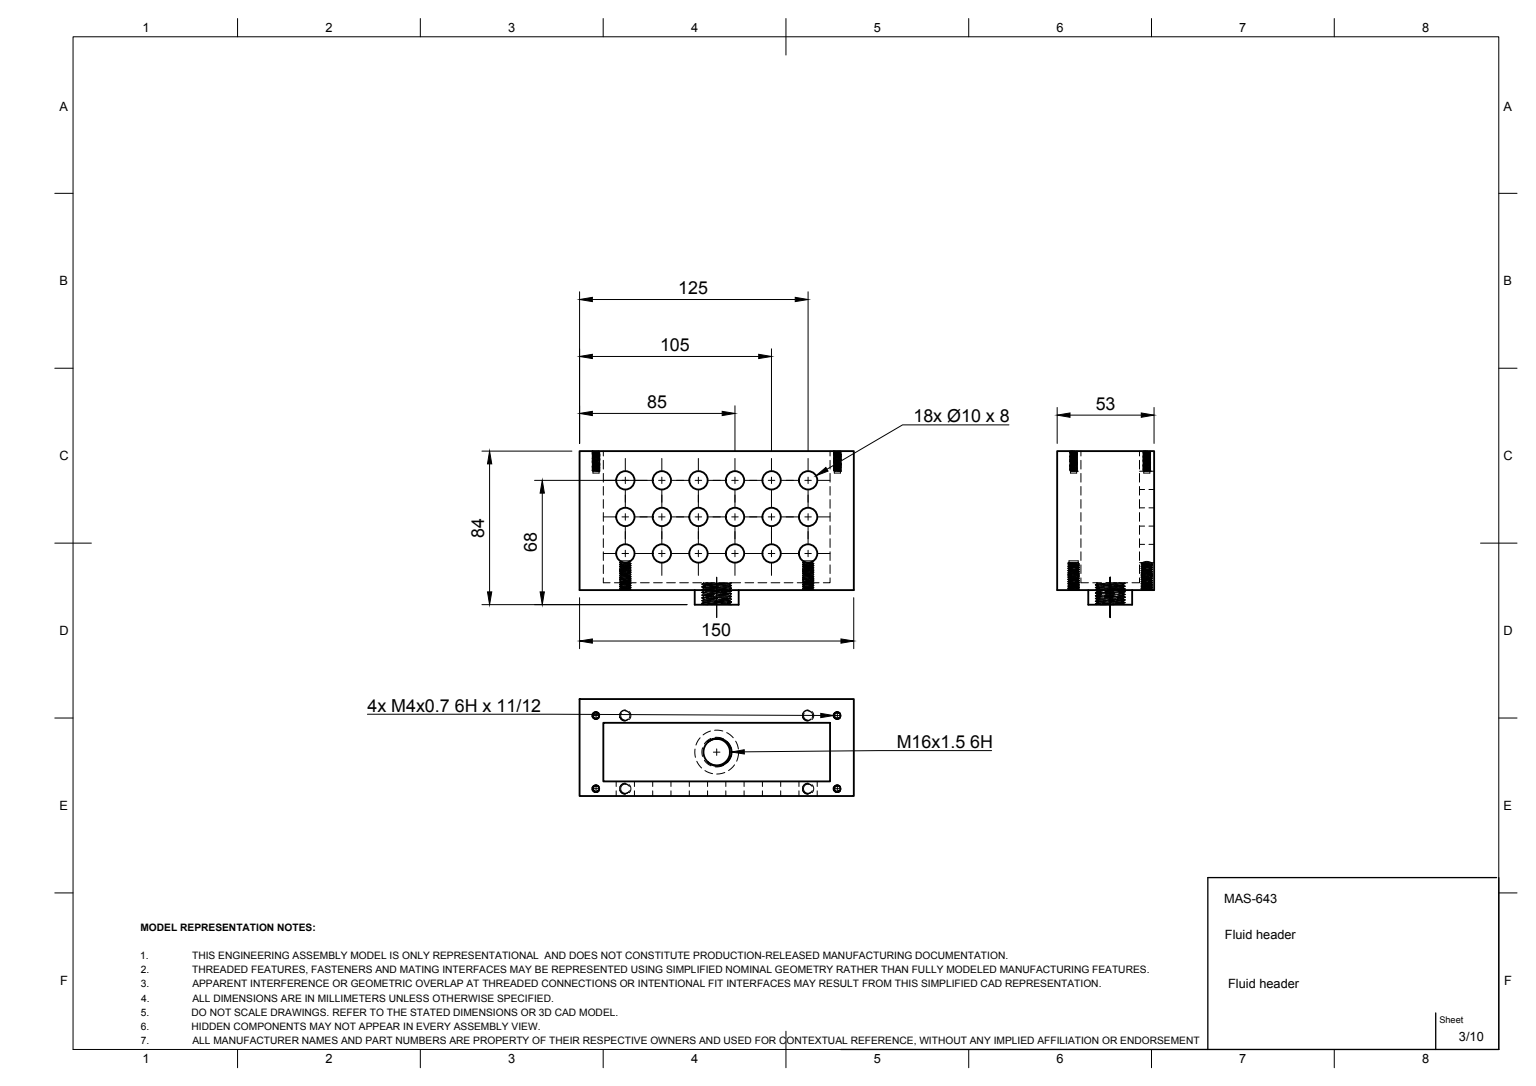
ISO-10303-21;
HEADER;
/* Generated by software containing ST-Developer
 * from STEP Tools, Inc. (www.steptools.com) 
 */

FILE_DESCRIPTION(
/* description */ ('Independent eighteen-tube parallel-flow evaporator geometry. Repeated
 machined headers and gasketed service covers, eighteen copper tubes, 
twenty-nine punched fins, threaded hose connections and bolted mountin
g feet. Native editable features and instanced parts. Braze details, w
orking fluid, pressure and thermal ratings require engineering selecti
on.'),
/* implementation_level */ '2;1');

FILE_NAME(
/* name */ 'Fluid header.step',
/* time_stamp */ '2026-11-08T20:53:59-08:00',
/* author */ (''),
/* organization */ (''),
/* preprocessor_version */ 'ST-DEVELOPER v20.2',
/* originating_system */ 'Autodesk Translation Framework v15.17.0.0',
/* authorisation */ '');

FILE_SCHEMA (('AUTOMOTIVE_DESIGN { 1 0 10303 214 3 1 1 }'));
ENDSEC;

DATA;
#10=MECHANICAL_DESIGN_GEOMETRIC_PRESENTATION_REPRESENTATION('',(#333),#42620);
#313=SHAPE_REPRESENTATION_RELATIONSHIP('SRR','None',#42723,#323);
#323=ADVANCED_BREP_SHAPE_REPRESENTATION('',(#343),#42610);
#333=STYLED_ITEM('',(#42782),#343);
#343=MANIFOLD_SOLID_BREP('Body1',#10383);
#353=FACE_BOUND('',#1411,.T.);
#354=FACE_BOUND('',#1415,.T.);
#355=FACE_BOUND('',#1416,.T.);
#356=FACE_BOUND('',#1417,.T.);
#357=FACE_BOUND('',#1418,.T.);
#358=FACE_BOUND('',#1419,.T.);
#359=FACE_BOUND('',#1492,.T.);
#360=FACE_BOUND('',#1493,.T.);
#361=FACE_BOUND('',#1494,.T.);
#362=FACE_BOUND('',#1495,.T.);
#363=FACE_BOUND('',#1496,.T.);
#364=FACE_BOUND('',#1497,.T.);
#365=FACE_BOUND('',#1498,.T.);
#366=FACE_BOUND('',#1499,.T.);
#367=FACE_BOUND('',#1500,.T.);
#368=FACE_BOUND('',#1501,.T.);
#369=FACE_BOUND('',#1502,.T.);
#370=FACE_BOUND('',#1503,.T.);
#371=FACE_BOUND('',#1504,.T.);
#372=FACE_BOUND('',#1505,.T.);
#373=FACE_BOUND('',#1506,.T.);
#374=FACE_BOUND('',#1507,.T.);
#375=FACE_BOUND('',#1508,.T.);
#376=FACE_BOUND('',#1509,.T.);
#377=FACE_BOUND('',#1513,.T.);
#378=FACE_BOUND('',#1516,.T.);
#379=FACE_BOUND('',#1517,.T.);
#380=FACE_BOUND('',#1518,.T.);
#381=FACE_BOUND('',#1519,.T.);
#382=FACE_BOUND('',#1520,.T.);
#383=FACE_BOUND('',#1521,.T.);
#384=FACE_BOUND('',#1522,.T.);
#385=FACE_BOUND('',#1523,.T.);
#386=FACE_BOUND('',#1524,.T.);
#387=FACE_BOUND('',#1525,.T.);
#388=FACE_BOUND('',#1526,.T.);
#389=FACE_BOUND('',#1527,.T.);
#390=FACE_BOUND('',#1528,.T.);
#391=FACE_BOUND('',#1529,.T.);
#392=FACE_BOUND('',#1530,.T.);
#393=FACE_BOUND('',#1531,.T.);
#394=FACE_BOUND('',#1532,.T.);
#395=FACE_BOUND('',#1533,.T.);
#396=FACE_BOUND('',#1537,.T.);
#397=FACE_BOUND('',#1538,.T.);
#398=FACE_BOUND('',#1539,.T.);
#399=FACE_BOUND('',#1540,.T.);
#400=FACE_BOUND('',#1541,.T.);
#487=PLANE('',#10813);
#488=PLANE('',#10818);
#489=PLANE('',#10819);
#490=PLANE('',#10822);
#491=PLANE('',#10825);
#492=PLANE('',#10826);
#493=PLANE('',#10828);
#494=PLANE('',#10831);
#495=PLANE('',#10832);
#496=PLANE('',#10834);
#497=PLANE('',#10838);
#498=PLANE('',#10839);
#499=PLANE('',#10841);
#500=PLANE('',#10844);
#501=PLANE('',#10847);
#502=PLANE('',#10850);
#503=PLANE('',#10853);
#504=PLANE('',#10854);
#505=PLANE('',#10855);
#506=PLANE('',#10856);
#507=PLANE('',#10911);
#508=PLANE('',#10912);
#509=PLANE('',#10913);
#510=PLANE('',#10914);
#511=PLANE('',#10915);
#512=PLANE('',#10916);
#513=PLANE('',#10917);
#514=PLANE('',#10918);
#515=PLANE('',#10919);
#516=PLANE('',#10920);
#579=B_SPLINE_SURFACE_WITH_KNOTS('',3,3,((#23222,#23223,#23224,#23225,#23226,
#23227,#23228,#23229,#23230,#23231,#23232,#23233,#23234,#23235,#23236,#23237,
#23238,#23239,#23240,#23241,#23242,#23243,#23244,#23245,#23246,#23247,#23248,
#23249,#23250,#23251,#23252,#23253,#23254,#23255,#23256,#23257,#23258,#23259,
#23260,#23261,#23262,#23263,#23264,#23265,#23266,#23267,#23268,#23269,#23270,
#23271,#23272,#23273,#23274,#23275,#23276,#23277,#23278,#23279,#23280,#23281,
#23282,#23283,#23284,#23285,#23286,#23287,#23288,#23289,#23290,#23291,#23292,
#23293,#23294,#23295,#23296,#23297,#23298,#23299,#23300,#23301,#23302,#23303,
#23304,#23305,#23306,#23307,#23308,#23309,#23310,#23311,#23312,#23313,#23314,
#23315,#23316,#23317,#23318,#23319,#23320,#23321,#23322,#23323,#23324,#23325,
#23326,#23327,#23328,#23329,#23330),(#23331,#23332,#23333,#23334,#23335,
#23336,#23337,#23338,#23339,#23340,#23341,#23342,#23343,#23344,#23345,#23346,
#23347,#23348,#23349,#23350,#23351,#23352,#23353,#23354,#23355,#23356,#23357,
#23358,#23359,#23360,#23361,#23362,#23363,#23364,#23365,#23366,#23367,#23368,
#23369,#23370,#23371,#23372,#23373,#23374,#23375,#23376,#23377,#23378,#23379,
#23380,#23381,#23382,#23383,#23384,#23385,#23386,#23387,#23388,#23389,#23390,
#23391,#23392,#23393,#23394,#23395,#23396,#23397,#23398,#23399,#23400,#23401,
#23402,#23403,#23404,#23405,#23406,#23407,#23408,#23409,#23410,#23411,#23412,
#23413,#23414,#23415,#23416,#23417,#23418,#23419,#23420,#23421,#23422,#23423,
#23424,#23425,#23426,#23427,#23428,#23429,#23430,#23431,#23432,#23433,#23434,
#23435,#23436,#23437,#23438,#23439),(#23440,#23441,#23442,#23443,#23444,
#23445,#23446,#23447,#23448,#23449,#23450,#23451,#23452,#23453,#23454,#23455,
#23456,#23457,#23458,#23459,#23460,#23461,#23462,#23463,#23464,#23465,#23466,
#23467,#23468,#23469,#23470,#23471,#23472,#23473,#23474,#23475,#23476,#23477,
#23478,#23479,#23480,#23481,#23482,#23483,#23484,#23485,#23486,#23487,#23488,
#23489,#23490,#23491,#23492,#23493,#23494,#23495,#23496,#23497,#23498,#23499,
#23500,#23501,#23502,#23503,#23504,#23505,#23506,#23507,#23508,#23509,#23510,
#23511,#23512,#23513,#23514,#23515,#23516,#23517,#23518,#23519,#23520,#23521,
#23522,#23523,#23524,#23525,#23526,#23527,#23528,#23529,#23530,#23531,#23532,
#23533,#23534,#23535,#23536,#23537,#23538,#23539,#23540,#23541,#23542,#23543,
#23544,#23545,#23546,#23547,#23548),(#23549,#23550,#23551,#23552,#23553,
#23554,#23555,#23556,#23557,#23558,#23559,#23560,#23561,#23562,#23563,#23564,
#23565,#23566,#23567,#23568,#23569,#23570,#23571,#23572,#23573,#23574,#23575,
#23576,#23577,#23578,#23579,#23580,#23581,#23582,#23583,#23584,#23585,#23586,
#23587,#23588,#23589,#23590,#23591,#23592,#23593,#23594,#23595,#23596,#23597,
#23598,#23599,#23600,#23601,#23602,#23603,#23604,#23605,#23606,#23607,#23608,
#23609,#23610,#23611,#23612,#23613,#23614,#23615,#23616,#23617,#23618,#23619,
#23620,#23621,#23622,#23623,#23624,#23625,#23626,#23627,#23628,#23629,#23630,
#23631,#23632,#23633,#23634,#23635,#23636,#23637,#23638,#23639,#23640,#23641,
#23642,#23643,#23644,#23645,#23646,#23647,#23648,#23649,#23650,#23651,#23652,
#23653,#23654,#23655,#23656,#23657)),.UNSPECIFIED.,.F.,.F.,.F.,(4,4),(4,
1,1,1,1,1,1,1,1,1,1,1,1,1,1,1,1,1,1,1,1,1,1,1,1,1,1,1,1,1,1,1,1,1,1,1,1,
1,1,1,1,1,1,1,1,1,1,1,1,1,1,1,1,1,1,1,1,1,1,1,1,1,1,1,1,1,1,1,1,1,1,1,1,
1,1,1,1,1,1,1,1,1,1,1,1,1,1,1,1,1,1,1,1,1,1,1,1,1,1,1,1,1,1,1,1,1,4),(0.,
0.0968216401431001),(11.8468968665462,12.3402299811373,12.8335630957283,
13.3268962103193,13.8202293249104,14.3135624395014,14.8068955540925,15.3002286686835,
15.7935617832746,16.2868948978656,16.7802280124566,17.2735611270477,17.7668942416387,
18.2602273562298,18.7535604708208,19.2468935854119,19.7402267000029,20.2335598145939,
20.726892929185,21.220226043776,21.7135591583671,22.2068922729581,22.7002253875492,
23.1935585021402,23.6868916167312,24.1802247313223,24.6735578459133,25.1668909605044,
25.6602240750954,26.1535571896865,26.6468903042775,27.1402234188686,27.6335565334596,
28.1268896480506,28.6202227626417,29.1135558772327,29.6068889918238,30.1002221064148,
30.5935552210059,31.0868883355969,31.5802214501879,32.073554564779,32.56688767937,
33.0602207939611,33.5535539085521,34.0468870231432,34.5402201377342,35.0335532523252,
35.5268863669163,36.0202194815073,36.5135525960984,37.0068857106894,37.5002188252805,
37.9935519398715,38.4868850544625,38.9802181690536,39.4735512836446,39.9668843982357,
40.4602175128267,40.9535506274178,41.4468837420088,41.9402168565998,42.4335499711909,
42.9268830857819,43.420216200373,43.913549314964,44.4068824295551,44.9002155441461,
45.3935486587371,45.8868817733282,46.3802148879192,46.8735480025103,47.3668811171013,
47.8602142316924,48.3535473462834,48.8468804608745,49.3402135754655,49.8335466900565,
50.3268798046476,50.8202129192386,51.3135460338297,51.8068791484207,52.3002122630117,
52.7935453776028,53.2868784921938,53.7802116067849,54.2735447213759,54.766877835967,
55.260210950558,55.7535440651491,56.2468771797401,56.7402102943311,57.2335434089222,
57.7268765235132,58.2202096381043,58.7135427526953,59.2068758672864,59.7002089818774,
60.1935420964684,60.6868752110595,61.1802083256505,61.6735414402416,62.1668745548326,
62.6602076694237,63.1535407840147,63.6468738986057,64.1402070131968),
 .UNSPECIFIED.);
#580=B_SPLINE_SURFACE_WITH_KNOTS('',3,3,((#23931,#23932,#23933,#23934,#23935,
#23936,#23937,#23938,#23939,#23940,#23941,#23942,#23943,#23944,#23945,#23946,
#23947,#23948,#23949,#23950,#23951,#23952,#23953,#23954,#23955,#23956,#23957,
#23958,#23959,#23960,#23961,#23962,#23963,#23964,#23965,#23966,#23967,#23968,
#23969,#23970,#23971,#23972,#23973,#23974,#23975,#23976,#23977,#23978,#23979,
#23980,#23981,#23982,#23983,#23984,#23985,#23986,#23987,#23988,#23989,#23990,
#23991,#23992,#23993,#23994,#23995,#23996,#23997,#23998,#23999,#24000,#24001,
#24002,#24003,#24004,#24005,#24006,#24007,#24008,#24009,#24010,#24011,#24012,
#24013,#24014,#24015,#24016,#24017,#24018,#24019,#24020,#24021,#24022,#24023,
#24024,#24025,#24026,#24027,#24028,#24029,#24030,#24031,#24032,#24033,#24034,
#24035,#24036,#24037,#24038,#24039),(#24040,#24041,#24042,#24043,#24044,
#24045,#24046,#24047,#24048,#24049,#24050,#24051,#24052,#24053,#24054,#24055,
#24056,#24057,#24058,#24059,#24060,#24061,#24062,#24063,#24064,#24065,#24066,
#24067,#24068,#24069,#24070,#24071,#24072,#24073,#24074,#24075,#24076,#24077,
#24078,#24079,#24080,#24081,#24082,#24083,#24084,#24085,#24086,#24087,#24088,
#24089,#24090,#24091,#24092,#24093,#24094,#24095,#24096,#24097,#24098,#24099,
#24100,#24101,#24102,#24103,#24104,#24105,#24106,#24107,#24108,#24109,#24110,
#24111,#24112,#24113,#24114,#24115,#24116,#24117,#24118,#24119,#24120,#24121,
#24122,#24123,#24124,#24125,#24126,#24127,#24128,#24129,#24130,#24131,#24132,
#24133,#24134,#24135,#24136,#24137,#24138,#24139,#24140,#24141,#24142,#24143,
#24144,#24145,#24146,#24147,#24148),(#24149,#24150,#24151,#24152,#24153,
#24154,#24155,#24156,#24157,#24158,#24159,#24160,#24161,#24162,#24163,#24164,
#24165,#24166,#24167,#24168,#24169,#24170,#24171,#24172,#24173,#24174,#24175,
#24176,#24177,#24178,#24179,#24180,#24181,#24182,#24183,#24184,#24185,#24186,
#24187,#24188,#24189,#24190,#24191,#24192,#24193,#24194,#24195,#24196,#24197,
#24198,#24199,#24200,#24201,#24202,#24203,#24204,#24205,#24206,#24207,#24208,
#24209,#24210,#24211,#24212,#24213,#24214,#24215,#24216,#24217,#24218,#24219,
#24220,#24221,#24222,#24223,#24224,#24225,#24226,#24227,#24228,#24229,#24230,
#24231,#24232,#24233,#24234,#24235,#24236,#24237,#24238,#24239,#24240,#24241,
#24242,#24243,#24244,#24245,#24246,#24247,#24248,#24249,#24250,#24251,#24252,
#24253,#24254,#24255,#24256,#24257),(#24258,#24259,#24260,#24261,#24262,
#24263,#24264,#24265,#24266,#24267,#24268,#24269,#24270,#24271,#24272,#24273,
#24274,#24275,#24276,#24277,#24278,#24279,#24280,#24281,#24282,#24283,#24284,
#24285,#24286,#24287,#24288,#24289,#24290,#24291,#24292,#24293,#24294,#24295,
#24296,#24297,#24298,#24299,#24300,#24301,#24302,#24303,#24304,#24305,#24306,
#24307,#24308,#24309,#24310,#24311,#24312,#24313,#24314,#24315,#24316,#24317,
#24318,#24319,#24320,#24321,#24322,#24323,#24324,#24325,#24326,#24327,#24328,
#24329,#24330,#24331,#24332,#24333,#24334,#24335,#24336,#24337,#24338,#24339,
#24340,#24341,#24342,#24343,#24344,#24345,#24346,#24347,#24348,#24349,#24350,
#24351,#24352,#24353,#24354,#24355,#24356,#24357,#24358,#24359,#24360,#24361,
#24362,#24363,#24364,#24365,#24366)),.UNSPECIFIED.,.F.,.F.,.F.,(4,4),(4,
1,1,1,1,1,1,1,1,1,1,1,1,1,1,1,1,1,1,1,1,1,1,1,1,1,1,1,1,1,1,1,1,1,1,1,1,
1,1,1,1,1,1,1,1,1,1,1,1,1,1,1,1,1,1,1,1,1,1,1,1,1,1,1,1,1,1,1,1,1,1,1,1,
1,1,1,1,1,1,1,1,1,1,1,1,1,1,1,1,1,1,1,1,1,1,1,1,1,1,1,1,1,1,1,1,1,4),(0.,
0.0968216401431001),(14.399609326548,14.892942441139,15.3862755557301,15.8796086703211,
16.3729417849122,16.8662748995032,17.3596080140942,17.8529411286853,18.3462742432763,
18.8396073578674,19.3329404724584,19.8262735870495,20.3196067016405,20.8129398162316,
21.3062729308226,21.7996060454136,22.2929391600047,22.7862722745957,23.2796053891868,
23.7729385037778,24.2662716183689,24.7596047329599,25.2529378475509,25.746270962142,
26.239604076733,26.7329371913241,27.2262703059151,27.7196034205062,28.2129365350972,
28.7062696496882,29.1996027642793,29.6929358788703,30.1862689934614,30.6796021080524,
31.1729352226435,31.6662683372345,32.1596014518255,32.6529345664166,33.1462676810076,
33.6396007955987,34.1329339101897,34.6262670247808,35.1196001393718,35.6129332539629,
36.1062663685539,36.5995994831449,37.092932597736,37.586265712327,38.0795988269181,
38.5729319415091,39.0662650561001,39.5595981706912,40.0529312852822,40.5462643998733,
41.0395975144643,41.5329306290554,42.0262637436464,42.5195968582374,43.0129299728285,
43.5062630874195,43.9995962020106,44.4929293166016,44.9862624311927,45.4795955457837,
45.9729286603748,46.4662617749658,46.9595948895568,47.4529280041479,47.9462611187389,
48.43959423333,48.932927347921,49.4262604625121,49.9195935771031,50.4129266916941,
50.9062598062852,51.3995929208762,51.8929260354673,52.3862591500583,52.8795922646494,
53.3729253792404,53.8662584938314,54.3595916084225,54.8529247230135,55.3462578376046,
55.8395909521956,56.3329240667867,56.8262571813777,57.3195902959688,57.8129234105598,
58.3062565251508,58.7995896397419,59.2929227543329,59.786255868924,60.279588983515,
60.7729220981061,61.2662552126971,61.7595883272881,62.2529214418792,62.7462545564702,
63.2395876710613,63.7329207856523,64.2262539002434,64.7195870148344,65.2129201294254,
65.7062532440165,66.1995863586075,66.6929194731986),.UNSPECIFIED.);
#581=B_SPLINE_SURFACE_WITH_KNOTS('',3,3,((#25611,#25612,#25613,#25614,#25615,
#25616,#25617,#25618,#25619,#25620,#25621,#25622,#25623,#25624,#25625,#25626,
#25627,#25628,#25629,#25630,#25631,#25632,#25633,#25634,#25635,#25636,#25637,
#25638,#25639,#25640,#25641,#25642,#25643,#25644,#25645,#25646,#25647,#25648,
#25649,#25650,#25651,#25652,#25653,#25654,#25655,#25656,#25657,#25658,#25659,
#25660,#25661,#25662,#25663,#25664,#25665,#25666,#25667,#25668,#25669,#25670,
#25671,#25672,#25673,#25674,#25675,#25676,#25677,#25678,#25679,#25680,#25681,
#25682,#25683,#25684,#25685,#25686,#25687,#25688,#25689,#25690,#25691,#25692,
#25693,#25694,#25695,#25696,#25697,#25698,#25699,#25700,#25701,#25702,#25703,
#25704,#25705,#25706,#25707,#25708,#25709,#25710),(#25711,#25712,#25713,
#25714,#25715,#25716,#25717,#25718,#25719,#25720,#25721,#25722,#25723,#25724,
#25725,#25726,#25727,#25728,#25729,#25730,#25731,#25732,#25733,#25734,#25735,
#25736,#25737,#25738,#25739,#25740,#25741,#25742,#25743,#25744,#25745,#25746,
#25747,#25748,#25749,#25750,#25751,#25752,#25753,#25754,#25755,#25756,#25757,
#25758,#25759,#25760,#25761,#25762,#25763,#25764,#25765,#25766,#25767,#25768,
#25769,#25770,#25771,#25772,#25773,#25774,#25775,#25776,#25777,#25778,#25779,
#25780,#25781,#25782,#25783,#25784,#25785,#25786,#25787,#25788,#25789,#25790,
#25791,#25792,#25793,#25794,#25795,#25796,#25797,#25798,#25799,#25800,#25801,
#25802,#25803,#25804,#25805,#25806,#25807,#25808,#25809,#25810),(#25811,
#25812,#25813,#25814,#25815,#25816,#25817,#25818,#25819,#25820,#25821,#25822,
#25823,#25824,#25825,#25826,#25827,#25828,#25829,#25830,#25831,#25832,#25833,
#25834,#25835,#25836,#25837,#25838,#25839,#25840,#25841,#25842,#25843,#25844,
#25845,#25846,#25847,#25848,#25849,#25850,#25851,#25852,#25853,#25854,#25855,
#25856,#25857,#25858,#25859,#25860,#25861,#25862,#25863,#25864,#25865,#25866,
#25867,#25868,#25869,#25870,#25871,#25872,#25873,#25874,#25875,#25876,#25877,
#25878,#25879,#25880,#25881,#25882,#25883,#25884,#25885,#25886,#25887,#25888,
#25889,#25890,#25891,#25892,#25893,#25894,#25895,#25896,#25897,#25898,#25899,
#25900,#25901,#25902,#25903,#25904,#25905,#25906,#25907,#25908,#25909,#25910),
(#25911,#25912,#25913,#25914,#25915,#25916,#25917,#25918,#25919,#25920,
#25921,#25922,#25923,#25924,#25925,#25926,#25927,#25928,#25929,#25930,#25931,
#25932,#25933,#25934,#25935,#25936,#25937,#25938,#25939,#25940,#25941,#25942,
#25943,#25944,#25945,#25946,#25947,#25948,#25949,#25950,#25951,#25952,#25953,
#25954,#25955,#25956,#25957,#25958,#25959,#25960,#25961,#25962,#25963,#25964,
#25965,#25966,#25967,#25968,#25969,#25970,#25971,#25972,#25973,#25974,#25975,
#25976,#25977,#25978,#25979,#25980,#25981,#25982,#25983,#25984,#25985,#25986,
#25987,#25988,#25989,#25990,#25991,#25992,#25993,#25994,#25995,#25996,#25997,
#25998,#25999,#26000,#26001,#26002,#26003,#26004,#26005,#26006,#26007,#26008,
#26009,#26010)),.UNSPECIFIED.,.F.,.F.,.F.,(4,4),(4,1,1,1,1,1,1,1,1,1,1,
1,1,1,1,1,1,1,1,1,1,1,1,1,1,1,1,1,1,1,1,1,1,1,1,1,1,1,1,1,1,1,1,1,1,1,1,
1,1,1,1,1,1,1,1,1,1,1,1,1,1,1,1,1,1,1,1,1,1,1,1,1,1,1,1,1,1,1,1,1,1,1,1,
1,1,1,1,1,1,1,1,1,1,1,1,1,1,4),(0.,0.0642013499338866),(11.8589888623077,
12.8514087025214,13.843828542735,14.8362483829486,15.8286682231623,16.8210880633759,
17.8135079035895,18.8059277438032,19.7983475840168,20.7907674242304,21.7831872644441,
22.7756071046577,23.7680269448713,24.7604467850849,25.7528666252986,26.7452864655122,
27.7377063057258,28.7301261459395,29.7225459861531,30.7149658263667,31.7073856665804,
32.699805506794,33.6922253470076,34.6846451872213,35.6770650274349,36.6694848676485,
37.6619047078622,38.6543245480758,39.6467443882894,40.639164228503,41.6315840687167,
42.6240039089303,43.6164237491439,44.6088435893576,45.6012634295712,46.5936832697848,
47.5861031099985,48.5785229502121,49.5709427904257,50.5633626306394,51.555782470853,
52.5482023110666,53.5406221512803,54.5330419914939,55.5254618317075,56.5178816719212,
57.5103015121348,58.5027213523484,59.4951411925621,60.4875610327757,61.4799808729893,
62.4724007132029,63.4648205534166,64.4572403936302,65.4496602338438,66.4420800740575,
67.4344999142711,68.4269197544847,69.4193395946984,70.411759434912,71.4041792751256,
72.3965991153393,73.3890189555529,74.3814387957665,75.3738586359802,76.3662784761938,
77.3586983164074,78.3511181566211,79.3435379968347,80.3359578370483,81.328377677262,
82.3207975174756,83.3132173576892,84.3056371979029,85.2980570381165,86.2904768783301,
87.2828967185437,88.2753165587574,89.267736398971,90.2601562391846,91.2525760793983,
92.2449959196119,93.2374157598255,94.2298356000392,95.2222554402528,96.2146752804664,
97.2070951206801,98.1995149608937,99.1919348011073,100.184354641321,101.176774481535,
102.169194321748,103.161614161962,104.154034002175,105.146453842389,106.138873682603,
107.131293522816,108.12371336303),.UNSPECIFIED.);
#582=B_SPLINE_SURFACE_WITH_KNOTS('',3,3,((#26036,#26037,#26038,#26039,#26040,
#26041,#26042,#26043,#26044,#26045,#26046,#26047,#26048,#26049,#26050,#26051,
#26052,#26053,#26054,#26055,#26056,#26057,#26058,#26059,#26060,#26061,#26062,
#26063,#26064,#26065,#26066,#26067,#26068,#26069,#26070,#26071,#26072,#26073,
#26074,#26075,#26076,#26077,#26078,#26079,#26080,#26081,#26082,#26083,#26084,
#26085,#26086,#26087,#26088,#26089,#26090,#26091,#26092,#26093,#26094,#26095,
#26096,#26097,#26098,#26099,#26100,#26101,#26102,#26103,#26104,#26105,#26106,
#26107,#26108,#26109,#26110,#26111,#26112,#26113,#26114,#26115,#26116,#26117,
#26118,#26119,#26120,#26121,#26122,#26123,#26124,#26125,#26126,#26127,#26128,
#26129,#26130,#26131,#26132,#26133,#26134,#26135),(#26136,#26137,#26138,
#26139,#26140,#26141,#26142,#26143,#26144,#26145,#26146,#26147,#26148,#26149,
#26150,#26151,#26152,#26153,#26154,#26155,#26156,#26157,#26158,#26159,#26160,
#26161,#26162,#26163,#26164,#26165,#26166,#26167,#26168,#26169,#26170,#26171,
#26172,#26173,#26174,#26175,#26176,#26177,#26178,#26179,#26180,#26181,#26182,
#26183,#26184,#26185,#26186,#26187,#26188,#26189,#26190,#26191,#26192,#26193,
#26194,#26195,#26196,#26197,#26198,#26199,#26200,#26201,#26202,#26203,#26204,
#26205,#26206,#26207,#26208,#26209,#26210,#26211,#26212,#26213,#26214,#26215,
#26216,#26217,#26218,#26219,#26220,#26221,#26222,#26223,#26224,#26225,#26226,
#26227,#26228,#26229,#26230,#26231,#26232,#26233,#26234,#26235),(#26236,
#26237,#26238,#26239,#26240,#26241,#26242,#26243,#26244,#26245,#26246,#26247,
#26248,#26249,#26250,#26251,#26252,#26253,#26254,#26255,#26256,#26257,#26258,
#26259,#26260,#26261,#26262,#26263,#26264,#26265,#26266,#26267,#26268,#26269,
#26270,#26271,#26272,#26273,#26274,#26275,#26276,#26277,#26278,#26279,#26280,
#26281,#26282,#26283,#26284,#26285,#26286,#26287,#26288,#26289,#26290,#26291,
#26292,#26293,#26294,#26295,#26296,#26297,#26298,#26299,#26300,#26301,#26302,
#26303,#26304,#26305,#26306,#26307,#26308,#26309,#26310,#26311,#26312,#26313,
#26314,#26315,#26316,#26317,#26318,#26319,#26320,#26321,#26322,#26323,#26324,
#26325,#26326,#26327,#26328,#26329,#26330,#26331,#26332,#26333,#26334,#26335),
(#26336,#26337,#26338,#26339,#26340,#26341,#26342,#26343,#26344,#26345,
#26346,#26347,#26348,#26349,#26350,#26351,#26352,#26353,#26354,#26355,#26356,
#26357,#26358,#26359,#26360,#26361,#26362,#26363,#26364,#26365,#26366,#26367,
#26368,#26369,#26370,#26371,#26372,#26373,#26374,#26375,#26376,#26377,#26378,
#26379,#26380,#26381,#26382,#26383,#26384,#26385,#26386,#26387,#26388,#26389,
#26390,#26391,#26392,#26393,#26394,#26395,#26396,#26397,#26398,#26399,#26400,
#26401,#26402,#26403,#26404,#26405,#26406,#26407,#26408,#26409,#26410,#26411,
#26412,#26413,#26414,#26415,#26416,#26417,#26418,#26419,#26420,#26421,#26422,
#26423,#26424,#26425,#26426,#26427,#26428,#26429,#26430,#26431,#26432,#26433,
#26434,#26435)),.UNSPECIFIED.,.F.,.F.,.F.,(4,4),(4,1,1,1,1,1,1,1,1,1,1,
1,1,1,1,1,1,1,1,1,1,1,1,1,1,1,1,1,1,1,1,1,1,1,1,1,1,1,1,1,1,1,1,1,1,1,1,
1,1,1,1,1,1,1,1,1,1,1,1,1,1,1,1,1,1,1,1,1,1,1,1,1,1,1,1,1,1,1,1,1,1,1,1,
1,1,1,1,1,1,1,1,1,1,1,1,1,1,4),(0.,0.0642013499338862),(14.3984001269718,
15.3908199671854,16.383239807399,17.3756596476127,18.3680794878263,19.3604993280399,
20.3529191682536,21.3453390084672,22.3377588486808,23.3301786888945,24.3225985291081,
25.3150183693217,26.3074382095353,27.299858049749,28.2922778899626,29.2846977301762,
30.2771175703899,31.2695374106035,32.2619572508171,33.2543770910308,34.2467969312444,
35.239216771458,36.2316366116717,37.2240564518853,38.2164762920989,39.2088961323126,
40.2013159725262,41.1937358127398,42.1861556529534,43.1785754931671,44.1709953333807,
45.1634151735943,46.155835013808,47.1482548540216,48.1406746942352,49.1330945344489,
50.1255143746625,51.1179342148761,52.1103540550898,53.1027738953034,54.095193735517,
55.0876135757306,56.0800334159443,57.0724532561579,58.0648730963715,59.0572929365852,
60.0497127767988,61.0421326170124,62.0345524572261,63.0269722974397,64.0193921376533,
65.011811977867,66.0042318180806,66.9966516582942,67.9890714985079,68.9814913387215,
69.9739111789351,70.9663310191488,71.9587508593624,72.951170699576,73.9435905397896,
74.9360103800033,75.9284302202169,76.9208500604305,77.9132699006442,78.9056897408578,
79.8981095810714,80.8905294212851,81.8829492614987,82.8753691017123,83.867788941926,
84.8602087821396,85.8526286223532,86.8450484625669,87.8374683027805,88.8298881429941,
89.8223079832078,90.8147278234214,91.807147663635,92.7995675038486,93.7919873440623,
94.7844071842759,95.7768270244895,96.7692468647032,97.7616667049168,98.7540865451304,
99.7465063853441,100.738926225558,101.731346065771,102.723765905985,103.716185746199,
104.708605586412,105.701025426626,106.693445266839,107.685865107053,108.678284947267,
109.67070478748,110.663124627694),.UNSPECIFIED.);
#583=B_SPLINE_SURFACE_WITH_KNOTS('',3,3,((#26670,#26671,#26672,#26673,#26674,
#26675,#26676,#26677,#26678,#26679,#26680,#26681,#26682,#26683,#26684,#26685,
#26686,#26687,#26688,#26689,#26690,#26691,#26692,#26693,#26694,#26695,#26696,
#26697,#26698,#26699,#26700,#26701,#26702,#26703,#26704,#26705,#26706,#26707,
#26708,#26709,#26710,#26711,#26712,#26713,#26714,#26715,#26716,#26717,#26718,
#26719,#26720,#26721,#26722,#26723,#26724,#26725,#26726,#26727,#26728,#26729,
#26730,#26731,#26732,#26733,#26734,#26735,#26736,#26737,#26738,#26739,#26740,
#26741,#26742,#26743,#26744,#26745,#26746,#26747,#26748,#26749,#26750,#26751,
#26752,#26753,#26754,#26755,#26756,#26757,#26758,#26759,#26760,#26761,#26762,
#26763,#26764,#26765,#26766,#26767,#26768,#26769),(#26770,#26771,#26772,
#26773,#26774,#26775,#26776,#26777,#26778,#26779,#26780,#26781,#26782,#26783,
#26784,#26785,#26786,#26787,#26788,#26789,#26790,#26791,#26792,#26793,#26794,
#26795,#26796,#26797,#26798,#26799,#26800,#26801,#26802,#26803,#26804,#26805,
#26806,#26807,#26808,#26809,#26810,#26811,#26812,#26813,#26814,#26815,#26816,
#26817,#26818,#26819,#26820,#26821,#26822,#26823,#26824,#26825,#26826,#26827,
#26828,#26829,#26830,#26831,#26832,#26833,#26834,#26835,#26836,#26837,#26838,
#26839,#26840,#26841,#26842,#26843,#26844,#26845,#26846,#26847,#26848,#26849,
#26850,#26851,#26852,#26853,#26854,#26855,#26856,#26857,#26858,#26859,#26860,
#26861,#26862,#26863,#26864,#26865,#26866,#26867,#26868,#26869),(#26870,
#26871,#26872,#26873,#26874,#26875,#26876,#26877,#26878,#26879,#26880,#26881,
#26882,#26883,#26884,#26885,#26886,#26887,#26888,#26889,#26890,#26891,#26892,
#26893,#26894,#26895,#26896,#26897,#26898,#26899,#26900,#26901,#26902,#26903,
#26904,#26905,#26906,#26907,#26908,#26909,#26910,#26911,#26912,#26913,#26914,
#26915,#26916,#26917,#26918,#26919,#26920,#26921,#26922,#26923,#26924,#26925,
#26926,#26927,#26928,#26929,#26930,#26931,#26932,#26933,#26934,#26935,#26936,
#26937,#26938,#26939,#26940,#26941,#26942,#26943,#26944,#26945,#26946,#26947,
#26948,#26949,#26950,#26951,#26952,#26953,#26954,#26955,#26956,#26957,#26958,
#26959,#26960,#26961,#26962,#26963,#26964,#26965,#26966,#26967,#26968,#26969),
(#26970,#26971,#26972,#26973,#26974,#26975,#26976,#26977,#26978,#26979,
#26980,#26981,#26982,#26983,#26984,#26985,#26986,#26987,#26988,#26989,#26990,
#26991,#26992,#26993,#26994,#26995,#26996,#26997,#26998,#26999,#27000,#27001,
#27002,#27003,#27004,#27005,#27006,#27007,#27008,#27009,#27010,#27011,#27012,
#27013,#27014,#27015,#27016,#27017,#27018,#27019,#27020,#27021,#27022,#27023,
#27024,#27025,#27026,#27027,#27028,#27029,#27030,#27031,#27032,#27033,#27034,
#27035,#27036,#27037,#27038,#27039,#27040,#27041,#27042,#27043,#27044,#27045,
#27046,#27047,#27048,#27049,#27050,#27051,#27052,#27053,#27054,#27055,#27056,
#27057,#27058,#27059,#27060,#27061,#27062,#27063,#27064,#27065,#27066,#27067,
#27068,#27069)),.UNSPECIFIED.,.F.,.F.,.F.,(4,4),(4,1,1,1,1,1,1,1,1,1,1,
1,1,1,1,1,1,1,1,1,1,1,1,1,1,1,1,1,1,1,1,1,1,1,1,1,1,1,1,1,1,1,1,1,1,1,1,
1,1,1,1,1,1,1,1,1,1,1,1,1,1,1,1,1,1,1,1,1,1,1,1,1,1,1,1,1,1,1,1,1,1,1,1,
1,1,1,1,1,1,1,1,1,1,1,1,1,1,4),(0.,0.0642013499338866),(11.8589888623077,
12.8514087025214,13.843828542735,14.8362483829486,15.8286682231623,16.8210880633759,
17.8135079035895,18.8059277438032,19.7983475840168,20.7907674242304,21.7831872644441,
22.7756071046577,23.7680269448713,24.7604467850849,25.7528666252986,26.7452864655122,
27.7377063057258,28.7301261459395,29.7225459861531,30.7149658263667,31.7073856665804,
32.699805506794,33.6922253470076,34.6846451872213,35.6770650274349,36.6694848676485,
37.6619047078622,38.6543245480758,39.6467443882894,40.639164228503,41.6315840687167,
42.6240039089303,43.6164237491439,44.6088435893576,45.6012634295712,46.5936832697848,
47.5861031099985,48.5785229502121,49.5709427904257,50.5633626306394,51.555782470853,
52.5482023110666,53.5406221512803,54.5330419914939,55.5254618317075,56.5178816719212,
57.5103015121348,58.5027213523484,59.4951411925621,60.4875610327757,61.4799808729893,
62.4724007132029,63.4648205534166,64.4572403936302,65.4496602338438,66.4420800740575,
67.4344999142711,68.4269197544847,69.4193395946984,70.411759434912,71.4041792751256,
72.3965991153393,73.3890189555529,74.3814387957665,75.3738586359802,76.3662784761938,
77.3586983164074,78.3511181566211,79.3435379968347,80.3359578370483,81.328377677262,
82.3207975174756,83.3132173576892,84.3056371979029,85.2980570381165,86.2904768783301,
87.2828967185437,88.2753165587574,89.267736398971,90.2601562391846,91.2525760793983,
92.2449959196119,93.2374157598255,94.2298356000392,95.2222554402528,96.2146752804664,
97.2070951206801,98.1995149608937,99.1919348011073,100.184354641321,101.176774481535,
102.169194321748,103.161614161962,104.154034002175,105.146453842389,106.138873682603,
107.131293522816,108.12371336303),.UNSPECIFIED.);
#584=B_SPLINE_SURFACE_WITH_KNOTS('',3,3,((#27095,#27096,#27097,#27098,#27099,
#27100,#27101,#27102,#27103,#27104,#27105,#27106,#27107,#27108,#27109,#27110,
#27111,#27112,#27113,#27114,#27115,#27116,#27117,#27118,#27119,#27120,#27121,
#27122,#27123,#27124,#27125,#27126,#27127,#27128,#27129,#27130,#27131,#27132,
#27133,#27134,#27135,#27136,#27137,#27138,#27139,#27140,#27141,#27142,#27143,
#27144,#27145,#27146,#27147,#27148,#27149,#27150,#27151,#27152,#27153,#27154,
#27155,#27156,#27157,#27158,#27159,#27160,#27161,#27162,#27163,#27164,#27165,
#27166,#27167,#27168,#27169,#27170,#27171,#27172,#27173,#27174,#27175,#27176,
#27177,#27178,#27179,#27180,#27181,#27182,#27183,#27184,#27185,#27186,#27187,
#27188,#27189,#27190,#27191,#27192,#27193,#27194),(#27195,#27196,#27197,
#27198,#27199,#27200,#27201,#27202,#27203,#27204,#27205,#27206,#27207,#27208,
#27209,#27210,#27211,#27212,#27213,#27214,#27215,#27216,#27217,#27218,#27219,
#27220,#27221,#27222,#27223,#27224,#27225,#27226,#27227,#27228,#27229,#27230,
#27231,#27232,#27233,#27234,#27235,#27236,#27237,#27238,#27239,#27240,#27241,
#27242,#27243,#27244,#27245,#27246,#27247,#27248,#27249,#27250,#27251,#27252,
#27253,#27254,#27255,#27256,#27257,#27258,#27259,#27260,#27261,#27262,#27263,
#27264,#27265,#27266,#27267,#27268,#27269,#27270,#27271,#27272,#27273,#27274,
#27275,#27276,#27277,#27278,#27279,#27280,#27281,#27282,#27283,#27284,#27285,
#27286,#27287,#27288,#27289,#27290,#27291,#27292,#27293,#27294),(#27295,
#27296,#27297,#27298,#27299,#27300,#27301,#27302,#27303,#27304,#27305,#27306,
#27307,#27308,#27309,#27310,#27311,#27312,#27313,#27314,#27315,#27316,#27317,
#27318,#27319,#27320,#27321,#27322,#27323,#27324,#27325,#27326,#27327,#27328,
#27329,#27330,#27331,#27332,#27333,#27334,#27335,#27336,#27337,#27338,#27339,
#27340,#27341,#27342,#27343,#27344,#27345,#27346,#27347,#27348,#27349,#27350,
#27351,#27352,#27353,#27354,#27355,#27356,#27357,#27358,#27359,#27360,#27361,
#27362,#27363,#27364,#27365,#27366,#27367,#27368,#27369,#27370,#27371,#27372,
#27373,#27374,#27375,#27376,#27377,#27378,#27379,#27380,#27381,#27382,#27383,
#27384,#27385,#27386,#27387,#27388,#27389,#27390,#27391,#27392,#27393,#27394),
(#27395,#27396,#27397,#27398,#27399,#27400,#27401,#27402,#27403,#27404,
#27405,#27406,#27407,#27408,#27409,#27410,#27411,#27412,#27413,#27414,#27415,
#27416,#27417,#27418,#27419,#27420,#27421,#27422,#27423,#27424,#27425,#27426,
#27427,#27428,#27429,#27430,#27431,#27432,#27433,#27434,#27435,#27436,#27437,
#27438,#27439,#27440,#27441,#27442,#27443,#27444,#27445,#27446,#27447,#27448,
#27449,#27450,#27451,#27452,#27453,#27454,#27455,#27456,#27457,#27458,#27459,
#27460,#27461,#27462,#27463,#27464,#27465,#27466,#27467,#27468,#27469,#27470,
#27471,#27472,#27473,#27474,#27475,#27476,#27477,#27478,#27479,#27480,#27481,
#27482,#27483,#27484,#27485,#27486,#27487,#27488,#27489,#27490,#27491,#27492,
#27493,#27494)),.UNSPECIFIED.,.F.,.F.,.F.,(4,4),(4,1,1,1,1,1,1,1,1,1,1,
1,1,1,1,1,1,1,1,1,1,1,1,1,1,1,1,1,1,1,1,1,1,1,1,1,1,1,1,1,1,1,1,1,1,1,1,
1,1,1,1,1,1,1,1,1,1,1,1,1,1,1,1,1,1,1,1,1,1,1,1,1,1,1,1,1,1,1,1,1,1,1,1,
1,1,1,1,1,1,1,1,1,1,1,1,1,1,4),(0.,0.0642013499338862),(14.3984001269718,
15.3908199671854,16.383239807399,17.3756596476127,18.3680794878263,19.3604993280399,
20.3529191682536,21.3453390084672,22.3377588486808,23.3301786888945,24.3225985291081,
25.3150183693217,26.3074382095353,27.299858049749,28.2922778899626,29.2846977301762,
30.2771175703899,31.2695374106035,32.2619572508171,33.2543770910308,34.2467969312444,
35.239216771458,36.2316366116717,37.2240564518853,38.2164762920989,39.2088961323126,
40.2013159725262,41.1937358127398,42.1861556529534,43.1785754931671,44.1709953333807,
45.1634151735943,46.155835013808,47.1482548540216,48.1406746942352,49.1330945344489,
50.1255143746625,51.1179342148761,52.1103540550898,53.1027738953034,54.095193735517,
55.0876135757306,56.0800334159443,57.0724532561579,58.0648730963715,59.0572929365852,
60.0497127767988,61.0421326170124,62.0345524572261,63.0269722974397,64.0193921376533,
65.011811977867,66.0042318180806,66.9966516582942,67.9890714985079,68.9814913387215,
69.9739111789351,70.9663310191488,71.9587508593624,72.951170699576,73.9435905397896,
74.9360103800033,75.9284302202169,76.9208500604305,77.9132699006442,78.9056897408578,
79.8981095810714,80.8905294212851,81.8829492614987,82.8753691017123,83.867788941926,
84.8602087821396,85.8526286223532,86.8450484625669,87.8374683027805,88.8298881429941,
89.8223079832078,90.8147278234214,91.807147663635,92.7995675038486,93.7919873440623,
94.7844071842759,95.7768270244895,96.7692468647032,97.7616667049168,98.7540865451304,
99.7465063853441,100.738926225558,101.731346065771,102.723765905985,103.716185746199,
104.708605586412,105.701025426626,106.693445266839,107.685865107053,108.678284947267,
109.67070478748,110.663124627694),.UNSPECIFIED.);
#585=B_SPLINE_SURFACE_WITH_KNOTS('',3,3,((#27743,#27744,#27745,#27746,#27747,
#27748,#27749,#27750,#27751,#27752,#27753,#27754,#27755,#27756,#27757,#27758,
#27759,#27760,#27761,#27762,#27763,#27764,#27765,#27766,#27767,#27768,#27769,
#27770,#27771,#27772,#27773,#27774,#27775,#27776,#27777,#27778,#27779,#27780,
#27781,#27782,#27783,#27784,#27785,#27786,#27787,#27788,#27789,#27790,#27791,
#27792,#27793,#27794,#27795,#27796,#27797,#27798,#27799,#27800,#27801,#27802,
#27803,#27804,#27805,#27806,#27807,#27808,#27809,#27810,#27811,#27812,#27813,
#27814,#27815,#27816,#27817,#27818,#27819,#27820,#27821,#27822,#27823,#27824,
#27825,#27826,#27827,#27828,#27829,#27830,#27831,#27832,#27833,#27834,#27835,
#27836,#27837,#27838,#27839,#27840,#27841,#27842),(#27843,#27844,#27845,
#27846,#27847,#27848,#27849,#27850,#27851,#27852,#27853,#27854,#27855,#27856,
#27857,#27858,#27859,#27860,#27861,#27862,#27863,#27864,#27865,#27866,#27867,
#27868,#27869,#27870,#27871,#27872,#27873,#27874,#27875,#27876,#27877,#27878,
#27879,#27880,#27881,#27882,#27883,#27884,#27885,#27886,#27887,#27888,#27889,
#27890,#27891,#27892,#27893,#27894,#27895,#27896,#27897,#27898,#27899,#27900,
#27901,#27902,#27903,#27904,#27905,#27906,#27907,#27908,#27909,#27910,#27911,
#27912,#27913,#27914,#27915,#27916,#27917,#27918,#27919,#27920,#27921,#27922,
#27923,#27924,#27925,#27926,#27927,#27928,#27929,#27930,#27931,#27932,#27933,
#27934,#27935,#27936,#27937,#27938,#27939,#27940,#27941,#27942),(#27943,
#27944,#27945,#27946,#27947,#27948,#27949,#27950,#27951,#27952,#27953,#27954,
#27955,#27956,#27957,#27958,#27959,#27960,#27961,#27962,#27963,#27964,#27965,
#27966,#27967,#27968,#27969,#27970,#27971,#27972,#27973,#27974,#27975,#27976,
#27977,#27978,#27979,#27980,#27981,#27982,#27983,#27984,#27985,#27986,#27987,
#27988,#27989,#27990,#27991,#27992,#27993,#27994,#27995,#27996,#27997,#27998,
#27999,#28000,#28001,#28002,#28003,#28004,#28005,#28006,#28007,#28008,#28009,
#28010,#28011,#28012,#28013,#28014,#28015,#28016,#28017,#28018,#28019,#28020,
#28021,#28022,#28023,#28024,#28025,#28026,#28027,#28028,#28029,#28030,#28031,
#28032,#28033,#28034,#28035,#28036,#28037,#28038,#28039,#28040,#28041,#28042),
(#28043,#28044,#28045,#28046,#28047,#28048,#28049,#28050,#28051,#28052,
#28053,#28054,#28055,#28056,#28057,#28058,#28059,#28060,#28061,#28062,#28063,
#28064,#28065,#28066,#28067,#28068,#28069,#28070,#28071,#28072,#28073,#28074,
#28075,#28076,#28077,#28078,#28079,#28080,#28081,#28082,#28083,#28084,#28085,
#28086,#28087,#28088,#28089,#28090,#28091,#28092,#28093,#28094,#28095,#28096,
#28097,#28098,#28099,#28100,#28101,#28102,#28103,#28104,#28105,#28106,#28107,
#28108,#28109,#28110,#28111,#28112,#28113,#28114,#28115,#28116,#28117,#28118,
#28119,#28120,#28121,#28122,#28123,#28124,#28125,#28126,#28127,#28128,#28129,
#28130,#28131,#28132,#28133,#28134,#28135,#28136,#28137,#28138,#28139,#28140,
#28141,#28142)),.UNSPECIFIED.,.F.,.F.,.F.,(4,4),(4,1,1,1,1,1,1,1,1,1,1,
1,1,1,1,1,1,1,1,1,1,1,1,1,1,1,1,1,1,1,1,1,1,1,1,1,1,1,1,1,1,1,1,1,1,1,1,
1,1,1,1,1,1,1,1,1,1,1,1,1,1,1,1,1,1,1,1,1,1,1,1,1,1,1,1,1,1,1,1,1,1,1,1,
1,1,1,1,1,1,1,1,1,1,1,1,1,1,4),(0.,0.0642013499338866),(11.8589888623077,
12.8514087025214,13.843828542735,14.8362483829486,15.8286682231623,16.8210880633759,
17.8135079035895,18.8059277438032,19.7983475840168,20.7907674242304,21.7831872644441,
22.7756071046577,23.7680269448713,24.7604467850849,25.7528666252986,26.7452864655122,
27.7377063057258,28.7301261459395,29.7225459861531,30.7149658263667,31.7073856665804,
32.699805506794,33.6922253470076,34.6846451872213,35.6770650274349,36.6694848676485,
37.6619047078622,38.6543245480758,39.6467443882894,40.639164228503,41.6315840687167,
42.6240039089303,43.6164237491439,44.6088435893576,45.6012634295712,46.5936832697848,
47.5861031099985,48.5785229502121,49.5709427904257,50.5633626306394,51.555782470853,
52.5482023110666,53.5406221512803,54.5330419914939,55.5254618317075,56.5178816719212,
57.5103015121348,58.5027213523484,59.4951411925621,60.4875610327757,61.4799808729893,
62.4724007132029,63.4648205534166,64.4572403936302,65.4496602338438,66.4420800740575,
67.4344999142711,68.4269197544847,69.4193395946984,70.411759434912,71.4041792751256,
72.3965991153393,73.3890189555529,74.3814387957665,75.3738586359802,76.3662784761938,
77.3586983164074,78.3511181566211,79.3435379968347,80.3359578370483,81.328377677262,
82.3207975174756,83.3132173576892,84.3056371979029,85.2980570381165,86.2904768783301,
87.2828967185437,88.2753165587574,89.267736398971,90.2601562391846,91.2525760793983,
92.2449959196119,93.2374157598255,94.2298356000392,95.2222554402528,96.2146752804664,
97.2070951206801,98.1995149608937,99.1919348011073,100.184354641321,101.176774481535,
102.169194321748,103.161614161962,104.154034002175,105.146453842389,106.138873682603,
107.131293522816,108.12371336303),.UNSPECIFIED.);
#586=B_SPLINE_SURFACE_WITH_KNOTS('',3,3,((#28168,#28169,#28170,#28171,#28172,
#28173,#28174,#28175,#28176,#28177,#28178,#28179,#28180,#28181,#28182,#28183,
#28184,#28185,#28186,#28187,#28188,#28189,#28190,#28191,#28192,#28193,#28194,
#28195,#28196,#28197,#28198,#28199,#28200,#28201,#28202,#28203,#28204,#28205,
#28206,#28207,#28208,#28209,#28210,#28211,#28212,#28213,#28214,#28215,#28216,
#28217,#28218,#28219,#28220,#28221,#28222,#28223,#28224,#28225,#28226,#28227,
#28228,#28229,#28230,#28231,#28232,#28233,#28234,#28235,#28236,#28237,#28238,
#28239,#28240,#28241,#28242,#28243,#28244,#28245,#28246,#28247,#28248,#28249,
#28250,#28251,#28252,#28253,#28254,#28255,#28256,#28257,#28258,#28259,#28260,
#28261,#28262,#28263,#28264,#28265,#28266,#28267),(#28268,#28269,#28270,
#28271,#28272,#28273,#28274,#28275,#28276,#28277,#28278,#28279,#28280,#28281,
#28282,#28283,#28284,#28285,#28286,#28287,#28288,#28289,#28290,#28291,#28292,
#28293,#28294,#28295,#28296,#28297,#28298,#28299,#28300,#28301,#28302,#28303,
#28304,#28305,#28306,#28307,#28308,#28309,#28310,#28311,#28312,#28313,#28314,
#28315,#28316,#28317,#28318,#28319,#28320,#28321,#28322,#28323,#28324,#28325,
#28326,#28327,#28328,#28329,#28330,#28331,#28332,#28333,#28334,#28335,#28336,
#28337,#28338,#28339,#28340,#28341,#28342,#28343,#28344,#28345,#28346,#28347,
#28348,#28349,#28350,#28351,#28352,#28353,#28354,#28355,#28356,#28357,#28358,
#28359,#28360,#28361,#28362,#28363,#28364,#28365,#28366,#28367),(#28368,
#28369,#28370,#28371,#28372,#28373,#28374,#28375,#28376,#28377,#28378,#28379,
#28380,#28381,#28382,#28383,#28384,#28385,#28386,#28387,#28388,#28389,#28390,
#28391,#28392,#28393,#28394,#28395,#28396,#28397,#28398,#28399,#28400,#28401,
#28402,#28403,#28404,#28405,#28406,#28407,#28408,#28409,#28410,#28411,#28412,
#28413,#28414,#28415,#28416,#28417,#28418,#28419,#28420,#28421,#28422,#28423,
#28424,#28425,#28426,#28427,#28428,#28429,#28430,#28431,#28432,#28433,#28434,
#28435,#28436,#28437,#28438,#28439,#28440,#28441,#28442,#28443,#28444,#28445,
#28446,#28447,#28448,#28449,#28450,#28451,#28452,#28453,#28454,#28455,#28456,
#28457,#28458,#28459,#28460,#28461,#28462,#28463,#28464,#28465,#28466,#28467),
(#28468,#28469,#28470,#28471,#28472,#28473,#28474,#28475,#28476,#28477,
#28478,#28479,#28480,#28481,#28482,#28483,#28484,#28485,#28486,#28487,#28488,
#28489,#28490,#28491,#28492,#28493,#28494,#28495,#28496,#28497,#28498,#28499,
#28500,#28501,#28502,#28503,#28504,#28505,#28506,#28507,#28508,#28509,#28510,
#28511,#28512,#28513,#28514,#28515,#28516,#28517,#28518,#28519,#28520,#28521,
#28522,#28523,#28524,#28525,#28526,#28527,#28528,#28529,#28530,#28531,#28532,
#28533,#28534,#28535,#28536,#28537,#28538,#28539,#28540,#28541,#28542,#28543,
#28544,#28545,#28546,#28547,#28548,#28549,#28550,#28551,#28552,#28553,#28554,
#28555,#28556,#28557,#28558,#28559,#28560,#28561,#28562,#28563,#28564,#28565,
#28566,#28567)),.UNSPECIFIED.,.F.,.F.,.F.,(4,4),(4,1,1,1,1,1,1,1,1,1,1,
1,1,1,1,1,1,1,1,1,1,1,1,1,1,1,1,1,1,1,1,1,1,1,1,1,1,1,1,1,1,1,1,1,1,1,1,
1,1,1,1,1,1,1,1,1,1,1,1,1,1,1,1,1,1,1,1,1,1,1,1,1,1,1,1,1,1,1,1,1,1,1,1,
1,1,1,1,1,1,1,1,1,1,1,1,1,1,4),(0.,0.0642013499338862),(14.3984001269718,
15.3908199671854,16.383239807399,17.3756596476127,18.3680794878263,19.3604993280399,
20.3529191682536,21.3453390084672,22.3377588486808,23.3301786888945,24.3225985291081,
25.3150183693217,26.3074382095353,27.299858049749,28.2922778899626,29.2846977301762,
30.2771175703899,31.2695374106035,32.2619572508171,33.2543770910308,34.2467969312444,
35.239216771458,36.2316366116717,37.2240564518853,38.2164762920989,39.2088961323126,
40.2013159725262,41.1937358127398,42.1861556529534,43.1785754931671,44.1709953333807,
45.1634151735943,46.155835013808,47.1482548540216,48.1406746942352,49.1330945344489,
50.1255143746625,51.1179342148761,52.1103540550898,53.1027738953034,54.095193735517,
55.0876135757306,56.0800334159443,57.0724532561579,58.0648730963715,59.0572929365852,
60.0497127767988,61.0421326170124,62.0345524572261,63.0269722974397,64.0193921376533,
65.011811977867,66.0042318180806,66.9966516582942,67.9890714985079,68.9814913387215,
69.9739111789351,70.9663310191488,71.9587508593624,72.951170699576,73.9435905397896,
74.9360103800033,75.9284302202169,76.9208500604305,77.9132699006442,78.9056897408578,
79.8981095810714,80.8905294212851,81.8829492614987,82.8753691017123,83.867788941926,
84.8602087821396,85.8526286223532,86.8450484625669,87.8374683027805,88.8298881429941,
89.8223079832078,90.8147278234214,91.807147663635,92.7995675038486,93.7919873440623,
94.7844071842759,95.7768270244895,96.7692468647032,97.7616667049168,98.7540865451304,
99.7465063853441,100.738926225558,101.731346065771,102.723765905985,103.716185746199,
104.708605586412,105.701025426626,106.693445266839,107.685865107053,108.678284947267,
109.67070478748,110.663124627694),.UNSPECIFIED.);
#587=B_SPLINE_SURFACE_WITH_KNOTS('',3,3,((#28837,#28838,#28839,#28840,#28841,
#28842,#28843,#28844,#28845,#28846,#28847,#28848,#28849,#28850,#28851,#28852,
#28853,#28854,#28855,#28856,#28857,#28858,#28859,#28860,#28861,#28862,#28863,
#28864,#28865,#28866,#28867,#28868,#28869,#28870,#28871,#28872,#28873,#28874,
#28875,#28876,#28877,#28878,#28879,#28880,#28881,#28882,#28883,#28884,#28885,
#28886,#28887,#28888,#28889,#28890,#28891,#28892,#28893,#28894,#28895,#28896,
#28897,#28898,#28899,#28900,#28901,#28902,#28903,#28904,#28905,#28906,#28907,
#28908,#28909,#28910,#28911,#28912,#28913,#28914,#28915,#28916,#28917,#28918,
#28919,#28920,#28921,#28922,#28923,#28924,#28925,#28926,#28927,#28928,#28929,
#28930,#28931,#28932,#28933,#28934,#28935,#28936),(#28937,#28938,#28939,
#28940,#28941,#28942,#28943,#28944,#28945,#28946,#28947,#28948,#28949,#28950,
#28951,#28952,#28953,#28954,#28955,#28956,#28957,#28958,#28959,#28960,#28961,
#28962,#28963,#28964,#28965,#28966,#28967,#28968,#28969,#28970,#28971,#28972,
#28973,#28974,#28975,#28976,#28977,#28978,#28979,#28980,#28981,#28982,#28983,
#28984,#28985,#28986,#28987,#28988,#28989,#28990,#28991,#28992,#28993,#28994,
#28995,#28996,#28997,#28998,#28999,#29000,#29001,#29002,#29003,#29004,#29005,
#29006,#29007,#29008,#29009,#29010,#29011,#29012,#29013,#29014,#29015,#29016,
#29017,#29018,#29019,#29020,#29021,#29022,#29023,#29024,#29025,#29026,#29027,
#29028,#29029,#29030,#29031,#29032,#29033,#29034,#29035,#29036),(#29037,
#29038,#29039,#29040,#29041,#29042,#29043,#29044,#29045,#29046,#29047,#29048,
#29049,#29050,#29051,#29052,#29053,#29054,#29055,#29056,#29057,#29058,#29059,
#29060,#29061,#29062,#29063,#29064,#29065,#29066,#29067,#29068,#29069,#29070,
#29071,#29072,#29073,#29074,#29075,#29076,#29077,#29078,#29079,#29080,#29081,
#29082,#29083,#29084,#29085,#29086,#29087,#29088,#29089,#29090,#29091,#29092,
#29093,#29094,#29095,#29096,#29097,#29098,#29099,#29100,#29101,#29102,#29103,
#29104,#29105,#29106,#29107,#29108,#29109,#29110,#29111,#29112,#29113,#29114,
#29115,#29116,#29117,#29118,#29119,#29120,#29121,#29122,#29123,#29124,#29125,
#29126,#29127,#29128,#29129,#29130,#29131,#29132,#29133,#29134,#29135,#29136),
(#29137,#29138,#29139,#29140,#29141,#29142,#29143,#29144,#29145,#29146,
#29147,#29148,#29149,#29150,#29151,#29152,#29153,#29154,#29155,#29156,#29157,
#29158,#29159,#29160,#29161,#29162,#29163,#29164,#29165,#29166,#29167,#29168,
#29169,#29170,#29171,#29172,#29173,#29174,#29175,#29176,#29177,#29178,#29179,
#29180,#29181,#29182,#29183,#29184,#29185,#29186,#29187,#29188,#29189,#29190,
#29191,#29192,#29193,#29194,#29195,#29196,#29197,#29198,#29199,#29200,#29201,
#29202,#29203,#29204,#29205,#29206,#29207,#29208,#29209,#29210,#29211,#29212,
#29213,#29214,#29215,#29216,#29217,#29218,#29219,#29220,#29221,#29222,#29223,
#29224,#29225,#29226,#29227,#29228,#29229,#29230,#29231,#29232,#29233,#29234,
#29235,#29236)),.UNSPECIFIED.,.F.,.F.,.F.,(4,4),(4,1,1,1,1,1,1,1,1,1,1,
1,1,1,1,1,1,1,1,1,1,1,1,1,1,1,1,1,1,1,1,1,1,1,1,1,1,1,1,1,1,1,1,1,1,1,1,
1,1,1,1,1,1,1,1,1,1,1,1,1,1,1,1,1,1,1,1,1,1,1,1,1,1,1,1,1,1,1,1,1,1,1,1,
1,1,1,1,1,1,1,1,1,1,1,1,1,1,4),(0.,0.0642013499338866),(11.8589888623077,
12.8514087025214,13.843828542735,14.8362483829486,15.8286682231623,16.8210880633759,
17.8135079035895,18.8059277438032,19.7983475840168,20.7907674242304,21.7831872644441,
22.7756071046577,23.7680269448713,24.7604467850849,25.7528666252986,26.7452864655122,
27.7377063057258,28.7301261459395,29.7225459861531,30.7149658263667,31.7073856665804,
32.699805506794,33.6922253470076,34.6846451872213,35.6770650274349,36.6694848676485,
37.6619047078622,38.6543245480758,39.6467443882894,40.639164228503,41.6315840687167,
42.6240039089303,43.6164237491439,44.6088435893576,45.6012634295712,46.5936832697848,
47.5861031099985,48.5785229502121,49.5709427904257,50.5633626306394,51.555782470853,
52.5482023110666,53.5406221512803,54.5330419914939,55.5254618317075,56.5178816719212,
57.5103015121348,58.5027213523484,59.4951411925621,60.4875610327757,61.4799808729893,
62.4724007132029,63.4648205534166,64.4572403936302,65.4496602338438,66.4420800740575,
67.4344999142711,68.4269197544847,69.4193395946984,70.411759434912,71.4041792751256,
72.3965991153393,73.3890189555529,74.3814387957665,75.3738586359802,76.3662784761938,
77.3586983164074,78.3511181566211,79.3435379968347,80.3359578370483,81.328377677262,
82.3207975174756,83.3132173576892,84.3056371979029,85.2980570381165,86.2904768783301,
87.2828967185437,88.2753165587574,89.267736398971,90.2601562391846,91.2525760793983,
92.2449959196119,93.2374157598255,94.2298356000392,95.2222554402528,96.2146752804664,
97.2070951206801,98.1995149608937,99.1919348011073,100.184354641321,101.176774481535,
102.169194321748,103.161614161962,104.154034002175,105.146453842389,106.138873682603,
107.131293522816,108.12371336303),.UNSPECIFIED.);
#588=B_SPLINE_SURFACE_WITH_KNOTS('',3,3,((#29262,#29263,#29264,#29265,#29266,
#29267,#29268,#29269,#29270,#29271,#29272,#29273,#29274,#29275,#29276,#29277,
#29278,#29279,#29280,#29281,#29282,#29283,#29284,#29285,#29286,#29287,#29288,
#29289,#29290,#29291,#29292,#29293,#29294,#29295,#29296,#29297,#29298,#29299,
#29300,#29301,#29302,#29303,#29304,#29305,#29306,#29307,#29308,#29309,#29310,
#29311,#29312,#29313,#29314,#29315,#29316,#29317,#29318,#29319,#29320,#29321,
#29322,#29323,#29324,#29325,#29326,#29327,#29328,#29329,#29330,#29331,#29332,
#29333,#29334,#29335,#29336,#29337,#29338,#29339,#29340,#29341,#29342,#29343,
#29344,#29345,#29346,#29347,#29348,#29349,#29350,#29351,#29352,#29353,#29354,
#29355,#29356,#29357,#29358,#29359,#29360,#29361),(#29362,#29363,#29364,
#29365,#29366,#29367,#29368,#29369,#29370,#29371,#29372,#29373,#29374,#29375,
#29376,#29377,#29378,#29379,#29380,#29381,#29382,#29383,#29384,#29385,#29386,
#29387,#29388,#29389,#29390,#29391,#29392,#29393,#29394,#29395,#29396,#29397,
#29398,#29399,#29400,#29401,#29402,#29403,#29404,#29405,#29406,#29407,#29408,
#29409,#29410,#29411,#29412,#29413,#29414,#29415,#29416,#29417,#29418,#29419,
#29420,#29421,#29422,#29423,#29424,#29425,#29426,#29427,#29428,#29429,#29430,
#29431,#29432,#29433,#29434,#29435,#29436,#29437,#29438,#29439,#29440,#29441,
#29442,#29443,#29444,#29445,#29446,#29447,#29448,#29449,#29450,#29451,#29452,
#29453,#29454,#29455,#29456,#29457,#29458,#29459,#29460,#29461),(#29462,
#29463,#29464,#29465,#29466,#29467,#29468,#29469,#29470,#29471,#29472,#29473,
#29474,#29475,#29476,#29477,#29478,#29479,#29480,#29481,#29482,#29483,#29484,
#29485,#29486,#29487,#29488,#29489,#29490,#29491,#29492,#29493,#29494,#29495,
#29496,#29497,#29498,#29499,#29500,#29501,#29502,#29503,#29504,#29505,#29506,
#29507,#29508,#29509,#29510,#29511,#29512,#29513,#29514,#29515,#29516,#29517,
#29518,#29519,#29520,#29521,#29522,#29523,#29524,#29525,#29526,#29527,#29528,
#29529,#29530,#29531,#29532,#29533,#29534,#29535,#29536,#29537,#29538,#29539,
#29540,#29541,#29542,#29543,#29544,#29545,#29546,#29547,#29548,#29549,#29550,
#29551,#29552,#29553,#29554,#29555,#29556,#29557,#29558,#29559,#29560,#29561),
(#29562,#29563,#29564,#29565,#29566,#29567,#29568,#29569,#29570,#29571,
#29572,#29573,#29574,#29575,#29576,#29577,#29578,#29579,#29580,#29581,#29582,
#29583,#29584,#29585,#29586,#29587,#29588,#29589,#29590,#29591,#29592,#29593,
#29594,#29595,#29596,#29597,#29598,#29599,#29600,#29601,#29602,#29603,#29604,
#29605,#29606,#29607,#29608,#29609,#29610,#29611,#29612,#29613,#29614,#29615,
#29616,#29617,#29618,#29619,#29620,#29621,#29622,#29623,#29624,#29625,#29626,
#29627,#29628,#29629,#29630,#29631,#29632,#29633,#29634,#29635,#29636,#29637,
#29638,#29639,#29640,#29641,#29642,#29643,#29644,#29645,#29646,#29647,#29648,
#29649,#29650,#29651,#29652,#29653,#29654,#29655,#29656,#29657,#29658,#29659,
#29660,#29661)),.UNSPECIFIED.,.F.,.F.,.F.,(4,4),(4,1,1,1,1,1,1,1,1,1,1,
1,1,1,1,1,1,1,1,1,1,1,1,1,1,1,1,1,1,1,1,1,1,1,1,1,1,1,1,1,1,1,1,1,1,1,1,
1,1,1,1,1,1,1,1,1,1,1,1,1,1,1,1,1,1,1,1,1,1,1,1,1,1,1,1,1,1,1,1,1,1,1,1,
1,1,1,1,1,1,1,1,1,1,1,1,1,1,4),(0.,0.0642013499338862),(14.3984001269718,
15.3908199671854,16.383239807399,17.3756596476127,18.3680794878263,19.3604993280399,
20.3529191682536,21.3453390084672,22.3377588486808,23.3301786888945,24.3225985291081,
25.3150183693217,26.3074382095353,27.299858049749,28.2922778899626,29.2846977301762,
30.2771175703899,31.2695374106035,32.2619572508171,33.2543770910308,34.2467969312444,
35.239216771458,36.2316366116717,37.2240564518853,38.2164762920989,39.2088961323126,
40.2013159725262,41.1937358127398,42.1861556529534,43.1785754931671,44.1709953333807,
45.1634151735943,46.155835013808,47.1482548540216,48.1406746942352,49.1330945344489,
50.1255143746625,51.1179342148761,52.1103540550898,53.1027738953034,54.095193735517,
55.0876135757306,56.0800334159443,57.0724532561579,58.0648730963715,59.0572929365852,
60.0497127767988,61.0421326170124,62.0345524572261,63.0269722974397,64.0193921376533,
65.011811977867,66.0042318180806,66.9966516582942,67.9890714985079,68.9814913387215,
69.9739111789351,70.9663310191488,71.9587508593624,72.951170699576,73.9435905397896,
74.9360103800033,75.9284302202169,76.9208500604305,77.9132699006442,78.9056897408578,
79.8981095810714,80.8905294212851,81.8829492614987,82.8753691017123,83.867788941926,
84.8602087821396,85.8526286223532,86.8450484625669,87.8374683027805,88.8298881429941,
89.8223079832078,90.8147278234214,91.807147663635,92.7995675038486,93.7919873440623,
94.7844071842759,95.7768270244895,96.7692468647032,97.7616667049168,98.7540865451304,
99.7465063853441,100.738926225558,101.731346065771,102.723765905985,103.716185746199,
104.708605586412,105.701025426626,106.693445266839,107.685865107053,108.678284947267,
109.67070478748,110.663124627694),.UNSPECIFIED.);
#589=B_SPLINE_SURFACE_WITH_KNOTS('',3,3,((#29906,#29907,#29908,#29909,#29910,
#29911,#29912,#29913,#29914,#29915,#29916,#29917,#29918,#29919,#29920,#29921,
#29922,#29923,#29924,#29925,#29926,#29927,#29928,#29929,#29930,#29931,#29932,
#29933,#29934,#29935,#29936,#29937,#29938,#29939,#29940,#29941,#29942,#29943,
#29944,#29945,#29946,#29947,#29948,#29949,#29950,#29951,#29952,#29953,#29954,
#29955,#29956,#29957,#29958,#29959,#29960,#29961,#29962,#29963,#29964,#29965,
#29966,#29967,#29968,#29969,#29970,#29971,#29972,#29973,#29974,#29975,#29976,
#29977,#29978,#29979,#29980,#29981,#29982,#29983,#29984,#29985,#29986,#29987,
#29988,#29989,#29990,#29991,#29992,#29993,#29994,#29995,#29996,#29997,#29998,
#29999,#30000,#30001,#30002,#30003,#30004,#30005,#30006,#30007,#30008,#30009),
(#30010,#30011,#30012,#30013,#30014,#30015,#30016,#30017,#30018,#30019,
#30020,#30021,#30022,#30023,#30024,#30025,#30026,#30027,#30028,#30029,#30030,
#30031,#30032,#30033,#30034,#30035,#30036,#30037,#30038,#30039,#30040,#30041,
#30042,#30043,#30044,#30045,#30046,#30047,#30048,#30049,#30050,#30051,#30052,
#30053,#30054,#30055,#30056,#30057,#30058,#30059,#30060,#30061,#30062,#30063,
#30064,#30065,#30066,#30067,#30068,#30069,#30070,#30071,#30072,#30073,#30074,
#30075,#30076,#30077,#30078,#30079,#30080,#30081,#30082,#30083,#30084,#30085,
#30086,#30087,#30088,#30089,#30090,#30091,#30092,#30093,#30094,#30095,#30096,
#30097,#30098,#30099,#30100,#30101,#30102,#30103,#30104,#30105,#30106,#30107,
#30108,#30109,#30110,#30111,#30112,#30113),(#30114,#30115,#30116,#30117,
#30118,#30119,#30120,#30121,#30122,#30123,#30124,#30125,#30126,#30127,#30128,
#30129,#30130,#30131,#30132,#30133,#30134,#30135,#30136,#30137,#30138,#30139,
#30140,#30141,#30142,#30143,#30144,#30145,#30146,#30147,#30148,#30149,#30150,
#30151,#30152,#30153,#30154,#30155,#30156,#30157,#30158,#30159,#30160,#30161,
#30162,#30163,#30164,#30165,#30166,#30167,#30168,#30169,#30170,#30171,#30172,
#30173,#30174,#30175,#30176,#30177,#30178,#30179,#30180,#30181,#30182,#30183,
#30184,#30185,#30186,#30187,#30188,#30189,#30190,#30191,#30192,#30193,#30194,
#30195,#30196,#30197,#30198,#30199,#30200,#30201,#30202,#30203,#30204,#30205,
#30206,#30207,#30208,#30209,#30210,#30211,#30212,#30213,#30214,#30215,#30216,
#30217),(#30218,#30219,#30220,#30221,#30222,#30223,#30224,#30225,#30226,
#30227,#30228,#30229,#30230,#30231,#30232,#30233,#30234,#30235,#30236,#30237,
#30238,#30239,#30240,#30241,#30242,#30243,#30244,#30245,#30246,#30247,#30248,
#30249,#30250,#30251,#30252,#30253,#30254,#30255,#30256,#30257,#30258,#30259,
#30260,#30261,#30262,#30263,#30264,#30265,#30266,#30267,#30268,#30269,#30270,
#30271,#30272,#30273,#30274,#30275,#30276,#30277,#30278,#30279,#30280,#30281,
#30282,#30283,#30284,#30285,#30286,#30287,#30288,#30289,#30290,#30291,#30292,
#30293,#30294,#30295,#30296,#30297,#30298,#30299,#30300,#30301,#30302,#30303,
#30304,#30305,#30306,#30307,#30308,#30309,#30310,#30311,#30312,#30313,#30314,
#30315,#30316,#30317,#30318,#30319,#30320,#30321)),.UNSPECIFIED.,.F.,.F.,
 .F.,(4,4),(4,1,1,1,1,1,1,1,1,1,1,1,1,1,1,1,1,1,1,1,1,1,1,1,1,1,1,1,1,1,
1,1,1,1,1,1,1,1,1,1,1,1,1,1,1,1,1,1,1,1,1,1,1,1,1,1,1,1,1,1,1,1,1,1,1,1,
1,1,1,1,1,1,1,1,1,1,1,1,1,1,1,1,1,1,1,1,1,1,1,1,1,1,1,1,1,1,1,1,1,1,1,4),
(0.,0.0448889834294935),(11.8615800042566,12.8591085386932,13.8566370731298,
14.8541656075664,15.851694142003,16.8492226764396,17.8467512108762,18.8442797453128,
19.8418082797494,20.839336814186,21.8368653486226,22.8343938830591,23.8319224174958,
24.8294509519324,25.8269794863689,26.8245080208056,27.8220365552421,28.8195650896787,
29.8170936241154,30.8146221585519,31.8121506929885,32.8096792274251,33.8072077618617,
34.8047362962984,35.8022648307349,36.7997933651715,37.7973218996081,38.7948504340447,
39.7923789684813,40.7899075029179,41.7874360373545,42.7849645717911,43.7824931062277,
44.7800216406643,45.7775501751009,46.7750787095375,47.7726072439741,48.7701357784107,
49.7676643128473,50.7651928472839,51.7627213817205,52.7602499161571,53.7577784505937,
54.7553069850303,55.7528355194669,56.7503640539035,57.7478925883401,58.7454211227767,
59.7429496572133,60.7404781916499,61.7380067260865,62.7355352605231,63.7330637949597,
64.7305923293963,65.7281208638329,66.7256493982695,67.7231779327061,68.7207064671427,
69.7182350015793,70.7157635360159,71.7132920704525,72.7108206048891,73.7083491393257,
74.7058776737623,75.7034062081989,76.7009347426355,77.6984632770721,78.6959918115087,
79.6935203459453,80.6910488803819,81.6885774148185,82.6861059492551,83.6836344836917,
84.6811630181283,85.6786915525649,86.6762200870015,87.6737486214381,88.6712771558747,
89.6688056903113,90.6663342247479,91.6638627591845,92.6613912936211,93.6589198280577,
94.6564483624943,95.6539768969309,96.6515054313675,97.6490339658041,98.6465625002407,
99.6440910346773,100.641619569114,101.639148103551,102.636676637987,103.634205172424,
104.63173370686,105.629262241297,106.626790775734,107.62431931017,108.621847844607,
109.619376379043,110.61690491348,111.614433447917,112.611961982353),
 .UNSPECIFIED.);
#590=B_SPLINE_SURFACE_WITH_KNOTS('',3,3,((#30429,#30430,#30431,#30432,#30433,
#30434,#30435,#30436,#30437,#30438,#30439,#30440,#30441,#30442,#30443,#30444,
#30445,#30446,#30447,#30448,#30449,#30450,#30451,#30452,#30453,#30454,#30455,
#30456,#30457,#30458,#30459,#30460,#30461,#30462,#30463,#30464,#30465,#30466,
#30467,#30468,#30469,#30470,#30471,#30472,#30473,#30474,#30475,#30476,#30477,
#30478,#30479,#30480,#30481,#30482,#30483,#30484,#30485,#30486,#30487,#30488,
#30489,#30490,#30491,#30492,#30493,#30494,#30495,#30496,#30497,#30498,#30499,
#30500,#30501,#30502,#30503,#30504,#30505,#30506,#30507,#30508,#30509,#30510,
#30511,#30512,#30513,#30514,#30515,#30516,#30517,#30518,#30519,#30520,#30521,
#30522,#30523,#30524,#30525,#30526,#30527,#30528,#30529,#30530,#30531,#30532),
(#30533,#30534,#30535,#30536,#30537,#30538,#30539,#30540,#30541,#30542,
#30543,#30544,#30545,#30546,#30547,#30548,#30549,#30550,#30551,#30552,#30553,
#30554,#30555,#30556,#30557,#30558,#30559,#30560,#30561,#30562,#30563,#30564,
#30565,#30566,#30567,#30568,#30569,#30570,#30571,#30572,#30573,#30574,#30575,
#30576,#30577,#30578,#30579,#30580,#30581,#30582,#30583,#30584,#30585,#30586,
#30587,#30588,#30589,#30590,#30591,#30592,#30593,#30594,#30595,#30596,#30597,
#30598,#30599,#30600,#30601,#30602,#30603,#30604,#30605,#30606,#30607,#30608,
#30609,#30610,#30611,#30612,#30613,#30614,#30615,#30616,#30617,#30618,#30619,
#30620,#30621,#30622,#30623,#30624,#30625,#30626,#30627,#30628,#30629,#30630,
#30631,#30632,#30633,#30634,#30635,#30636),(#30637,#30638,#30639,#30640,
#30641,#30642,#30643,#30644,#30645,#30646,#30647,#30648,#30649,#30650,#30651,
#30652,#30653,#30654,#30655,#30656,#30657,#30658,#30659,#30660,#30661,#30662,
#30663,#30664,#30665,#30666,#30667,#30668,#30669,#30670,#30671,#30672,#30673,
#30674,#30675,#30676,#30677,#30678,#30679,#30680,#30681,#30682,#30683,#30684,
#30685,#30686,#30687,#30688,#30689,#30690,#30691,#30692,#30693,#30694,#30695,
#30696,#30697,#30698,#30699,#30700,#30701,#30702,#30703,#30704,#30705,#30706,
#30707,#30708,#30709,#30710,#30711,#30712,#30713,#30714,#30715,#30716,#30717,
#30718,#30719,#30720,#30721,#30722,#30723,#30724,#30725,#30726,#30727,#30728,
#30729,#30730,#30731,#30732,#30733,#30734,#30735,#30736,#30737,#30738,#30739,
#30740),(#30741,#30742,#30743,#30744,#30745,#30746,#30747,#30748,#30749,
#30750,#30751,#30752,#30753,#30754,#30755,#30756,#30757,#30758,#30759,#30760,
#30761,#30762,#30763,#30764,#30765,#30766,#30767,#30768,#30769,#30770,#30771,
#30772,#30773,#30774,#30775,#30776,#30777,#30778,#30779,#30780,#30781,#30782,
#30783,#30784,#30785,#30786,#30787,#30788,#30789,#30790,#30791,#30792,#30793,
#30794,#30795,#30796,#30797,#30798,#30799,#30800,#30801,#30802,#30803,#30804,
#30805,#30806,#30807,#30808,#30809,#30810,#30811,#30812,#30813,#30814,#30815,
#30816,#30817,#30818,#30819,#30820,#30821,#30822,#30823,#30824,#30825,#30826,
#30827,#30828,#30829,#30830,#30831,#30832,#30833,#30834,#30835,#30836,#30837,
#30838,#30839,#30840,#30841,#30842,#30843,#30844)),.UNSPECIFIED.,.F.,.F.,
 .F.,(4,4),(4,1,1,1,1,1,1,1,1,1,1,1,1,1,1,1,1,1,1,1,1,1,1,1,1,1,1,1,1,1,
1,1,1,1,1,1,1,1,1,1,1,1,1,1,1,1,1,1,1,1,1,1,1,1,1,1,1,1,1,1,1,1,1,1,1,1,
1,1,1,1,1,1,1,1,1,1,1,1,1,1,1,1,1,1,1,1,1,1,1,1,1,1,1,1,1,1,1,1,1,1,1,4),
(0.,0.0448889834294935),(14.3981410127768,15.3956695472134,16.39319808165,
17.3907266160866,18.3882551505232,19.3857836849598,20.3833122193964,21.380840753833,
22.3783692882696,23.3758978227062,24.3734263571428,25.3709548915794,26.368483426016,
27.3660119604526,28.3635404948892,29.3610690293258,30.3585975637624,31.356126098199,
32.3536546326356,33.3511831670722,34.3487117015088,35.3462402359454,36.343768770382,
37.3412973048186,38.3388258392552,39.3363543736918,40.3338829081284,41.331411442565,
42.3289399770016,43.3264685114382,44.3239970458748,45.3215255803114,46.319054114748,
47.3165826491846,48.3141111836212,49.3116397180578,50.3091682524944,51.306696786931,
52.3042253213676,53.3017538558042,54.2992823902408,55.2968109246774,56.294339459114,
57.2918679935506,58.2893965279872,59.2869250624238,60.2844535968604,61.281982131297,
62.2795106657336,63.2770392001702,64.2745677346068,65.2720962690434,66.26962480348,
67.2671533379166,68.2646818723532,69.2622104067898,70.2597389412264,71.257267475663,
72.2547960100996,73.2523245445362,74.2498530789728,75.2473816134094,76.244910147846,
77.2424386822826,78.2399672167192,79.2374957511558,80.2350242855924,81.232552820029,
82.2300813544656,83.2276098889022,84.2251384233388,85.2226669577754,86.220195492212,
87.2177240266486,88.2152525610852,89.2127810955218,90.2103096299584,91.207838164395,
92.2053666988316,93.2028952332682,94.2004237677048,95.1979523021414,96.195480836578,
97.1930093710146,98.1905379054512,99.1880664398878,100.185594974324,101.183123508761,
102.180652043198,103.178180577634,104.175709112071,105.173237646507,106.170766180944,
107.168294715381,108.165823249817,109.163351784254,110.16088031869,111.158408853127,
112.155937387564,113.153465922,114.150994456437,115.148522990873),
 .UNSPECIFIED.);
#591=B_SPLINE_SURFACE_WITH_KNOTS('',3,3,((#31149,#31150,#31151,#31152,#31153,
#31154,#31155,#31156,#31157,#31158,#31159,#31160,#31161,#31162,#31163,#31164,
#31165,#31166,#31167,#31168,#31169,#31170,#31171,#31172,#31173,#31174,#31175,
#31176,#31177,#31178,#31179,#31180,#31181,#31182,#31183,#31184,#31185,#31186,
#31187,#31188,#31189,#31190,#31191,#31192,#31193,#31194,#31195,#31196,#31197,
#31198,#31199,#31200,#31201,#31202,#31203,#31204,#31205,#31206,#31207,#31208,
#31209,#31210,#31211,#31212,#31213,#31214,#31215,#31216,#31217,#31218,#31219,
#31220,#31221,#31222,#31223,#31224,#31225,#31226,#31227,#31228,#31229,#31230,
#31231,#31232,#31233,#31234,#31235,#31236,#31237,#31238,#31239,#31240,#31241,
#31242,#31243,#31244,#31245,#31246,#31247,#31248,#31249,#31250,#31251,#31252),
(#31253,#31254,#31255,#31256,#31257,#31258,#31259,#31260,#31261,#31262,
#31263,#31264,#31265,#31266,#31267,#31268,#31269,#31270,#31271,#31272,#31273,
#31274,#31275,#31276,#31277,#31278,#31279,#31280,#31281,#31282,#31283,#31284,
#31285,#31286,#31287,#31288,#31289,#31290,#31291,#31292,#31293,#31294,#31295,
#31296,#31297,#31298,#31299,#31300,#31301,#31302,#31303,#31304,#31305,#31306,
#31307,#31308,#31309,#31310,#31311,#31312,#31313,#31314,#31315,#31316,#31317,
#31318,#31319,#31320,#31321,#31322,#31323,#31324,#31325,#31326,#31327,#31328,
#31329,#31330,#31331,#31332,#31333,#31334,#31335,#31336,#31337,#31338,#31339,
#31340,#31341,#31342,#31343,#31344,#31345,#31346,#31347,#31348,#31349,#31350,
#31351,#31352,#31353,#31354,#31355,#31356),(#31357,#31358,#31359,#31360,
#31361,#31362,#31363,#31364,#31365,#31366,#31367,#31368,#31369,#31370,#31371,
#31372,#31373,#31374,#31375,#31376,#31377,#31378,#31379,#31380,#31381,#31382,
#31383,#31384,#31385,#31386,#31387,#31388,#31389,#31390,#31391,#31392,#31393,
#31394,#31395,#31396,#31397,#31398,#31399,#31400,#31401,#31402,#31403,#31404,
#31405,#31406,#31407,#31408,#31409,#31410,#31411,#31412,#31413,#31414,#31415,
#31416,#31417,#31418,#31419,#31420,#31421,#31422,#31423,#31424,#31425,#31426,
#31427,#31428,#31429,#31430,#31431,#31432,#31433,#31434,#31435,#31436,#31437,
#31438,#31439,#31440,#31441,#31442,#31443,#31444,#31445,#31446,#31447,#31448,
#31449,#31450,#31451,#31452,#31453,#31454,#31455,#31456,#31457,#31458,#31459,
#31460),(#31461,#31462,#31463,#31464,#31465,#31466,#31467,#31468,#31469,
#31470,#31471,#31472,#31473,#31474,#31475,#31476,#31477,#31478,#31479,#31480,
#31481,#31482,#31483,#31484,#31485,#31486,#31487,#31488,#31489,#31490,#31491,
#31492,#31493,#31494,#31495,#31496,#31497,#31498,#31499,#31500,#31501,#31502,
#31503,#31504,#31505,#31506,#31507,#31508,#31509,#31510,#31511,#31512,#31513,
#31514,#31515,#31516,#31517,#31518,#31519,#31520,#31521,#31522,#31523,#31524,
#31525,#31526,#31527,#31528,#31529,#31530,#31531,#31532,#31533,#31534,#31535,
#31536,#31537,#31538,#31539,#31540,#31541,#31542,#31543,#31544,#31545,#31546,
#31547,#31548,#31549,#31550,#31551,#31552,#31553,#31554,#31555,#31556,#31557,
#31558,#31559,#31560,#31561,#31562,#31563,#31564)),.UNSPECIFIED.,.F.,.F.,
 .F.,(4,4),(4,1,1,1,1,1,1,1,1,1,1,1,1,1,1,1,1,1,1,1,1,1,1,1,1,1,1,1,1,1,
1,1,1,1,1,1,1,1,1,1,1,1,1,1,1,1,1,1,1,1,1,1,1,1,1,1,1,1,1,1,1,1,1,1,1,1,
1,1,1,1,1,1,1,1,1,1,1,1,1,1,1,1,1,1,1,1,1,1,1,1,1,1,1,1,1,1,1,1,1,1,1,4),
(0.,0.0448889834294935),(11.8615800042566,12.8591085386932,13.8566370731298,
14.8541656075664,15.851694142003,16.8492226764396,17.8467512108762,18.8442797453128,
19.8418082797494,20.839336814186,21.8368653486226,22.8343938830592,23.8319224174958,
24.8294509519324,25.826979486369,26.8245080208056,27.8220365552422,28.8195650896788,
29.8170936241154,30.814622158552,31.8121506929886,32.8096792274252,33.8072077618618,
34.8047362962984,35.802264830735,36.7997933651716,37.7973218996082,38.7948504340448,
39.7923789684814,40.789907502918,41.7874360373546,42.7849645717912,43.7824931062278,
44.7800216406644,45.777550175101,46.7750787095376,47.7726072439742,48.7701357784108,
49.7676643128474,50.765192847284,51.7627213817206,52.7602499161572,53.7577784505938,
54.7553069850304,55.752835519467,56.7503640539036,57.7478925883402,58.7454211227768,
59.7429496572134,60.74047819165,61.7380067260866,62.7355352605232,63.7330637949598,
64.7305923293964,65.728120863833,66.7256493982696,67.7231779327062,68.7207064671428,
69.7182350015794,70.715763536016,71.7132920704526,72.7108206048892,73.7083491393258,
74.7058776737624,75.703406208199,76.7009347426356,77.6984632770722,78.6959918115088,
79.6935203459454,80.691048880382,81.6885774148186,82.6861059492552,83.6836344836918,
84.6811630181284,85.678691552565,86.6762200870016,87.6737486214382,88.6712771558748,
89.6688056903114,90.666334224748,91.6638627591846,92.6613912936212,93.6589198280578,
94.6564483624944,95.653976896931,96.6515054313676,97.6490339658042,98.6465625002408,
99.6440910346774,100.641619569114,101.639148103551,102.636676637987,103.634205172424,
104.63173370686,105.629262241297,106.626790775734,107.62431931017,108.621847844607,
109.619376379043,110.61690491348,111.614433447917,112.611961982353),
 .UNSPECIFIED.);
#592=B_SPLINE_SURFACE_WITH_KNOTS('',3,3,((#31672,#31673,#31674,#31675,#31676,
#31677,#31678,#31679,#31680,#31681,#31682,#31683,#31684,#31685,#31686,#31687,
#31688,#31689,#31690,#31691,#31692,#31693,#31694,#31695,#31696,#31697,#31698,
#31699,#31700,#31701,#31702,#31703,#31704,#31705,#31706,#31707,#31708,#31709,
#31710,#31711,#31712,#31713,#31714,#31715,#31716,#31717,#31718,#31719,#31720,
#31721,#31722,#31723,#31724,#31725,#31726,#31727,#31728,#31729,#31730,#31731,
#31732,#31733,#31734,#31735,#31736,#31737,#31738,#31739,#31740,#31741,#31742,
#31743,#31744,#31745,#31746,#31747,#31748,#31749,#31750,#31751,#31752,#31753,
#31754,#31755,#31756,#31757,#31758,#31759,#31760,#31761,#31762,#31763,#31764,
#31765,#31766,#31767,#31768,#31769,#31770,#31771,#31772,#31773,#31774,#31775),
(#31776,#31777,#31778,#31779,#31780,#31781,#31782,#31783,#31784,#31785,
#31786,#31787,#31788,#31789,#31790,#31791,#31792,#31793,#31794,#31795,#31796,
#31797,#31798,#31799,#31800,#31801,#31802,#31803,#31804,#31805,#31806,#31807,
#31808,#31809,#31810,#31811,#31812,#31813,#31814,#31815,#31816,#31817,#31818,
#31819,#31820,#31821,#31822,#31823,#31824,#31825,#31826,#31827,#31828,#31829,
#31830,#31831,#31832,#31833,#31834,#31835,#31836,#31837,#31838,#31839,#31840,
#31841,#31842,#31843,#31844,#31845,#31846,#31847,#31848,#31849,#31850,#31851,
#31852,#31853,#31854,#31855,#31856,#31857,#31858,#31859,#31860,#31861,#31862,
#31863,#31864,#31865,#31866,#31867,#31868,#31869,#31870,#31871,#31872,#31873,
#31874,#31875,#31876,#31877,#31878,#31879),(#31880,#31881,#31882,#31883,
#31884,#31885,#31886,#31887,#31888,#31889,#31890,#31891,#31892,#31893,#31894,
#31895,#31896,#31897,#31898,#31899,#31900,#31901,#31902,#31903,#31904,#31905,
#31906,#31907,#31908,#31909,#31910,#31911,#31912,#31913,#31914,#31915,#31916,
#31917,#31918,#31919,#31920,#31921,#31922,#31923,#31924,#31925,#31926,#31927,
#31928,#31929,#31930,#31931,#31932,#31933,#31934,#31935,#31936,#31937,#31938,
#31939,#31940,#31941,#31942,#31943,#31944,#31945,#31946,#31947,#31948,#31949,
#31950,#31951,#31952,#31953,#31954,#31955,#31956,#31957,#31958,#31959,#31960,
#31961,#31962,#31963,#31964,#31965,#31966,#31967,#31968,#31969,#31970,#31971,
#31972,#31973,#31974,#31975,#31976,#31977,#31978,#31979,#31980,#31981,#31982,
#31983),(#31984,#31985,#31986,#31987,#31988,#31989,#31990,#31991,#31992,
#31993,#31994,#31995,#31996,#31997,#31998,#31999,#32000,#32001,#32002,#32003,
#32004,#32005,#32006,#32007,#32008,#32009,#32010,#32011,#32012,#32013,#32014,
#32015,#32016,#32017,#32018,#32019,#32020,#32021,#32022,#32023,#32024,#32025,
#32026,#32027,#32028,#32029,#32030,#32031,#32032,#32033,#32034,#32035,#32036,
#32037,#32038,#32039,#32040,#32041,#32042,#32043,#32044,#32045,#32046,#32047,
#32048,#32049,#32050,#32051,#32052,#32053,#32054,#32055,#32056,#32057,#32058,
#32059,#32060,#32061,#32062,#32063,#32064,#32065,#32066,#32067,#32068,#32069,
#32070,#32071,#32072,#32073,#32074,#32075,#32076,#32077,#32078,#32079,#32080,
#32081,#32082,#32083,#32084,#32085,#32086,#32087)),.UNSPECIFIED.,.F.,.F.,
 .F.,(4,4),(4,1,1,1,1,1,1,1,1,1,1,1,1,1,1,1,1,1,1,1,1,1,1,1,1,1,1,1,1,1,
1,1,1,1,1,1,1,1,1,1,1,1,1,1,1,1,1,1,1,1,1,1,1,1,1,1,1,1,1,1,1,1,1,1,1,1,
1,1,1,1,1,1,1,1,1,1,1,1,1,1,1,1,1,1,1,1,1,1,1,1,1,1,1,1,1,1,1,1,1,1,1,4),
(0.,0.0448889834294935),(14.3981410127769,15.3956695472135,16.3931980816501,
17.3907266160867,18.3882551505233,19.3857836849599,20.3833122193965,21.3808407538331,
22.3783692882697,23.3758978227063,24.3734263571429,25.3709548915795,26.3684834260161,
27.3660119604527,28.3635404948893,29.3610690293259,30.3585975637625,31.3561260981991,
32.3536546326357,33.3511831670723,34.3487117015089,35.3462402359455,36.3437687703821,
37.3412973048187,38.3388258392553,39.3363543736919,40.3338829081285,41.3314114425651,
42.3289399770017,43.3264685114383,44.3239970458749,45.3215255803115,46.3190541147481,
47.3165826491847,48.3141111836213,49.3116397180578,50.3091682524944,51.3066967869311,
52.3042253213677,53.3017538558043,54.2992823902408,55.2968109246774,56.294339459114,
57.2918679935507,58.2893965279873,59.2869250624238,60.2844535968604,61.281982131297,
62.2795106657336,63.2770392001703,64.2745677346068,65.2720962690434,66.26962480348,
67.2671533379166,68.2646818723533,69.2622104067898,70.2597389412264,71.257267475663,
72.2547960100996,73.2523245445362,74.2498530789728,75.2473816134094,76.244910147846,
77.2424386822826,78.2399672167192,79.2374957511558,80.2350242855924,81.232552820029,
82.2300813544656,83.2276098889022,84.2251384233388,85.2226669577754,86.220195492212,
87.2177240266486,88.2152525610852,89.2127810955218,90.2103096299584,91.207838164395,
92.2053666988316,93.2028952332682,94.2004237677048,95.1979523021414,96.195480836578,
97.1930093710146,98.1905379054512,99.1880664398878,100.185594974324,101.183123508761,
102.180652043198,103.178180577634,104.175709112071,105.173237646507,106.170766180944,
107.168294715381,108.165823249817,109.163351784254,110.16088031869,111.158408853127,
112.155937387564,113.153465922,114.150994456437,115.148522990873),
 .UNSPECIFIED.);
#593=B_SPLINE_SURFACE_WITH_KNOTS('',3,3,((#32392,#32393,#32394,#32395,#32396,
#32397,#32398,#32399,#32400,#32401,#32402,#32403,#32404,#32405,#32406,#32407,
#32408,#32409,#32410,#32411,#32412,#32413,#32414,#32415,#32416,#32417,#32418,
#32419,#32420,#32421,#32422,#32423,#32424,#32425,#32426,#32427,#32428,#32429,
#32430,#32431,#32432,#32433,#32434,#32435,#32436,#32437,#32438,#32439,#32440,
#32441,#32442,#32443,#32444,#32445,#32446,#32447,#32448,#32449,#32450,#32451,
#32452,#32453,#32454,#32455,#32456,#32457,#32458,#32459,#32460,#32461,#32462,
#32463,#32464,#32465,#32466,#32467,#32468,#32469,#32470,#32471,#32472,#32473,
#32474,#32475,#32476,#32477,#32478,#32479,#32480,#32481,#32482,#32483,#32484,
#32485,#32486,#32487,#32488,#32489,#32490,#32491,#32492,#32493,#32494,#32495),
(#32496,#32497,#32498,#32499,#32500,#32501,#32502,#32503,#32504,#32505,
#32506,#32507,#32508,#32509,#32510,#32511,#32512,#32513,#32514,#32515,#32516,
#32517,#32518,#32519,#32520,#32521,#32522,#32523,#32524,#32525,#32526,#32527,
#32528,#32529,#32530,#32531,#32532,#32533,#32534,#32535,#32536,#32537,#32538,
#32539,#32540,#32541,#32542,#32543,#32544,#32545,#32546,#32547,#32548,#32549,
#32550,#32551,#32552,#32553,#32554,#32555,#32556,#32557,#32558,#32559,#32560,
#32561,#32562,#32563,#32564,#32565,#32566,#32567,#32568,#32569,#32570,#32571,
#32572,#32573,#32574,#32575,#32576,#32577,#32578,#32579,#32580,#32581,#32582,
#32583,#32584,#32585,#32586,#32587,#32588,#32589,#32590,#32591,#32592,#32593,
#32594,#32595,#32596,#32597,#32598,#32599),(#32600,#32601,#32602,#32603,
#32604,#32605,#32606,#32607,#32608,#32609,#32610,#32611,#32612,#32613,#32614,
#32615,#32616,#32617,#32618,#32619,#32620,#32621,#32622,#32623,#32624,#32625,
#32626,#32627,#32628,#32629,#32630,#32631,#32632,#32633,#32634,#32635,#32636,
#32637,#32638,#32639,#32640,#32641,#32642,#32643,#32644,#32645,#32646,#32647,
#32648,#32649,#32650,#32651,#32652,#32653,#32654,#32655,#32656,#32657,#32658,
#32659,#32660,#32661,#32662,#32663,#32664,#32665,#32666,#32667,#32668,#32669,
#32670,#32671,#32672,#32673,#32674,#32675,#32676,#32677,#32678,#32679,#32680,
#32681,#32682,#32683,#32684,#32685,#32686,#32687,#32688,#32689,#32690,#32691,
#32692,#32693,#32694,#32695,#32696,#32697,#32698,#32699,#32700,#32701,#32702,
#32703),(#32704,#32705,#32706,#32707,#32708,#32709,#32710,#32711,#32712,
#32713,#32714,#32715,#32716,#32717,#32718,#32719,#32720,#32721,#32722,#32723,
#32724,#32725,#32726,#32727,#32728,#32729,#32730,#32731,#32732,#32733,#32734,
#32735,#32736,#32737,#32738,#32739,#32740,#32741,#32742,#32743,#32744,#32745,
#32746,#32747,#32748,#32749,#32750,#32751,#32752,#32753,#32754,#32755,#32756,
#32757,#32758,#32759,#32760,#32761,#32762,#32763,#32764,#32765,#32766,#32767,
#32768,#32769,#32770,#32771,#32772,#32773,#32774,#32775,#32776,#32777,#32778,
#32779,#32780,#32781,#32782,#32783,#32784,#32785,#32786,#32787,#32788,#32789,
#32790,#32791,#32792,#32793,#32794,#32795,#32796,#32797,#32798,#32799,#32800,
#32801,#32802,#32803,#32804,#32805,#32806,#32807)),.UNSPECIFIED.,.F.,.F.,
 .F.,(4,4),(4,1,1,1,1,1,1,1,1,1,1,1,1,1,1,1,1,1,1,1,1,1,1,1,1,1,1,1,1,1,
1,1,1,1,1,1,1,1,1,1,1,1,1,1,1,1,1,1,1,1,1,1,1,1,1,1,1,1,1,1,1,1,1,1,1,1,
1,1,1,1,1,1,1,1,1,1,1,1,1,1,1,1,1,1,1,1,1,1,1,1,1,1,1,1,1,1,1,1,1,1,1,4),
(0.,0.0448889834294935),(11.8615800042566,12.8591085386932,13.8566370731298,
14.8541656075664,15.851694142003,16.8492226764396,17.8467512108762,18.8442797453128,
19.8418082797494,20.839336814186,21.8368653486226,22.8343938830592,23.8319224174958,
24.8294509519324,25.826979486369,26.8245080208056,27.8220365552422,28.8195650896788,
29.8170936241154,30.814622158552,31.8121506929886,32.8096792274252,33.8072077618618,
34.8047362962984,35.802264830735,36.7997933651716,37.7973218996082,38.7948504340448,
39.7923789684814,40.789907502918,41.7874360373546,42.7849645717912,43.7824931062278,
44.7800216406644,45.777550175101,46.7750787095376,47.7726072439742,48.7701357784108,
49.7676643128474,50.765192847284,51.7627213817206,52.7602499161572,53.7577784505938,
54.7553069850304,55.752835519467,56.7503640539036,57.7478925883402,58.7454211227768,
59.7429496572134,60.74047819165,61.7380067260866,62.7355352605232,63.7330637949598,
64.7305923293964,65.728120863833,66.7256493982696,67.7231779327062,68.7207064671428,
69.7182350015794,70.715763536016,71.7132920704526,72.7108206048892,73.7083491393258,
74.7058776737624,75.703406208199,76.7009347426356,77.6984632770722,78.6959918115088,
79.6935203459454,80.691048880382,81.6885774148186,82.6861059492552,83.6836344836918,
84.6811630181284,85.678691552565,86.6762200870016,87.6737486214382,88.6712771558748,
89.6688056903114,90.666334224748,91.6638627591846,92.6613912936212,93.6589198280578,
94.6564483624944,95.653976896931,96.6515054313676,97.6490339658042,98.6465625002408,
99.6440910346774,100.641619569114,101.639148103551,102.636676637987,103.634205172424,
104.63173370686,105.629262241297,106.626790775734,107.62431931017,108.621847844607,
109.619376379043,110.61690491348,111.614433447917,112.611961982353),
 .UNSPECIFIED.);
#594=B_SPLINE_SURFACE_WITH_KNOTS('',3,3,((#32915,#32916,#32917,#32918,#32919,
#32920,#32921,#32922,#32923,#32924,#32925,#32926,#32927,#32928,#32929,#32930,
#32931,#32932,#32933,#32934,#32935,#32936,#32937,#32938,#32939,#32940,#32941,
#32942,#32943,#32944,#32945,#32946,#32947,#32948,#32949,#32950,#32951,#32952,
#32953,#32954,#32955,#32956,#32957,#32958,#32959,#32960,#32961,#32962,#32963,
#32964,#32965,#32966,#32967,#32968,#32969,#32970,#32971,#32972,#32973,#32974,
#32975,#32976,#32977,#32978,#32979,#32980,#32981,#32982,#32983,#32984,#32985,
#32986,#32987,#32988,#32989,#32990,#32991,#32992,#32993,#32994,#32995,#32996,
#32997,#32998,#32999,#33000,#33001,#33002,#33003,#33004,#33005,#33006,#33007,
#33008,#33009,#33010,#33011,#33012,#33013,#33014,#33015,#33016,#33017,#33018),
(#33019,#33020,#33021,#33022,#33023,#33024,#33025,#33026,#33027,#33028,
#33029,#33030,#33031,#33032,#33033,#33034,#33035,#33036,#33037,#33038,#33039,
#33040,#33041,#33042,#33043,#33044,#33045,#33046,#33047,#33048,#33049,#33050,
#33051,#33052,#33053,#33054,#33055,#33056,#33057,#33058,#33059,#33060,#33061,
#33062,#33063,#33064,#33065,#33066,#33067,#33068,#33069,#33070,#33071,#33072,
#33073,#33074,#33075,#33076,#33077,#33078,#33079,#33080,#33081,#33082,#33083,
#33084,#33085,#33086,#33087,#33088,#33089,#33090,#33091,#33092,#33093,#33094,
#33095,#33096,#33097,#33098,#33099,#33100,#33101,#33102,#33103,#33104,#33105,
#33106,#33107,#33108,#33109,#33110,#33111,#33112,#33113,#33114,#33115,#33116,
#33117,#33118,#33119,#33120,#33121,#33122),(#33123,#33124,#33125,#33126,
#33127,#33128,#33129,#33130,#33131,#33132,#33133,#33134,#33135,#33136,#33137,
#33138,#33139,#33140,#33141,#33142,#33143,#33144,#33145,#33146,#33147,#33148,
#33149,#33150,#33151,#33152,#33153,#33154,#33155,#33156,#33157,#33158,#33159,
#33160,#33161,#33162,#33163,#33164,#33165,#33166,#33167,#33168,#33169,#33170,
#33171,#33172,#33173,#33174,#33175,#33176,#33177,#33178,#33179,#33180,#33181,
#33182,#33183,#33184,#33185,#33186,#33187,#33188,#33189,#33190,#33191,#33192,
#33193,#33194,#33195,#33196,#33197,#33198,#33199,#33200,#33201,#33202,#33203,
#33204,#33205,#33206,#33207,#33208,#33209,#33210,#33211,#33212,#33213,#33214,
#33215,#33216,#33217,#33218,#33219,#33220,#33221,#33222,#33223,#33224,#33225,
#33226),(#33227,#33228,#33229,#33230,#33231,#33232,#33233,#33234,#33235,
#33236,#33237,#33238,#33239,#33240,#33241,#33242,#33243,#33244,#33245,#33246,
#33247,#33248,#33249,#33250,#33251,#33252,#33253,#33254,#33255,#33256,#33257,
#33258,#33259,#33260,#33261,#33262,#33263,#33264,#33265,#33266,#33267,#33268,
#33269,#33270,#33271,#33272,#33273,#33274,#33275,#33276,#33277,#33278,#33279,
#33280,#33281,#33282,#33283,#33284,#33285,#33286,#33287,#33288,#33289,#33290,
#33291,#33292,#33293,#33294,#33295,#33296,#33297,#33298,#33299,#33300,#33301,
#33302,#33303,#33304,#33305,#33306,#33307,#33308,#33309,#33310,#33311,#33312,
#33313,#33314,#33315,#33316,#33317,#33318,#33319,#33320,#33321,#33322,#33323,
#33324,#33325,#33326,#33327,#33328,#33329,#33330)),.UNSPECIFIED.,.F.,.F.,
 .F.,(4,4),(4,1,1,1,1,1,1,1,1,1,1,1,1,1,1,1,1,1,1,1,1,1,1,1,1,1,1,1,1,1,
1,1,1,1,1,1,1,1,1,1,1,1,1,1,1,1,1,1,1,1,1,1,1,1,1,1,1,1,1,1,1,1,1,1,1,1,
1,1,1,1,1,1,1,1,1,1,1,1,1,1,1,1,1,1,1,1,1,1,1,1,1,1,1,1,1,1,1,1,1,1,1,4),
(0.,0.0448889834294935),(14.3981410127769,15.3956695472135,16.3931980816501,
17.3907266160867,18.3882551505233,19.3857836849599,20.3833122193965,21.3808407538331,
22.3783692882697,23.3758978227063,24.3734263571429,25.3709548915795,26.3684834260161,
27.3660119604527,28.3635404948893,29.3610690293259,30.3585975637625,31.3561260981991,
32.3536546326357,33.3511831670723,34.3487117015089,35.3462402359455,36.3437687703821,
37.3412973048187,38.3388258392553,39.3363543736919,40.3338829081285,41.3314114425651,
42.3289399770017,43.3264685114383,44.3239970458749,45.3215255803115,46.3190541147481,
47.3165826491847,48.3141111836213,49.3116397180579,50.3091682524945,51.3066967869311,
52.3042253213677,53.3017538558043,54.2992823902409,55.2968109246775,56.2943394591141,
57.2918679935507,58.2893965279873,59.2869250624239,60.2844535968605,61.2819821312971,
62.2795106657337,63.2770392001703,64.2745677346069,65.2720962690435,66.2696248034801,
67.2671533379167,68.2646818723533,69.2622104067899,70.2597389412265,71.2572674756631,
72.2547960100997,73.2523245445363,74.2498530789729,75.2473816134095,76.2449101478461,
77.2424386822827,78.2399672167193,79.2374957511559,80.2350242855925,81.2325528200291,
82.2300813544657,83.2276098889023,84.2251384233389,85.2226669577755,86.2201954922121,
87.2177240266487,88.2152525610853,89.2127810955219,90.2103096299585,91.2078381643951,
92.2053666988317,93.2028952332683,94.2004237677049,95.1979523021415,96.1954808365781,
97.1930093710147,98.1905379054513,99.1880664398879,100.185594974324,101.183123508761,
102.180652043198,103.178180577634,104.175709112071,105.173237646507,106.170766180944,
107.168294715381,108.165823249817,109.163351784254,110.16088031869,111.158408853127,
112.155937387564,113.153465922,114.150994456437,115.148522990873),
 .UNSPECIFIED.);
#595=B_SPLINE_SURFACE_WITH_KNOTS('',3,3,((#33635,#33636,#33637,#33638,#33639,
#33640,#33641,#33642,#33643,#33644,#33645,#33646,#33647,#33648,#33649,#33650,
#33651,#33652,#33653,#33654,#33655,#33656,#33657,#33658,#33659,#33660,#33661,
#33662,#33663,#33664,#33665,#33666,#33667,#33668,#33669,#33670,#33671,#33672,
#33673,#33674,#33675,#33676,#33677,#33678,#33679,#33680,#33681,#33682,#33683,
#33684,#33685,#33686,#33687,#33688,#33689,#33690,#33691,#33692,#33693,#33694,
#33695,#33696,#33697,#33698,#33699,#33700,#33701,#33702,#33703,#33704,#33705,
#33706,#33707,#33708,#33709,#33710,#33711,#33712,#33713,#33714,#33715,#33716,
#33717,#33718,#33719,#33720,#33721,#33722,#33723,#33724,#33725,#33726,#33727,
#33728,#33729,#33730,#33731,#33732,#33733,#33734,#33735,#33736,#33737,#33738),
(#33739,#33740,#33741,#33742,#33743,#33744,#33745,#33746,#33747,#33748,
#33749,#33750,#33751,#33752,#33753,#33754,#33755,#33756,#33757,#33758,#33759,
#33760,#33761,#33762,#33763,#33764,#33765,#33766,#33767,#33768,#33769,#33770,
#33771,#33772,#33773,#33774,#33775,#33776,#33777,#33778,#33779,#33780,#33781,
#33782,#33783,#33784,#33785,#33786,#33787,#33788,#33789,#33790,#33791,#33792,
#33793,#33794,#33795,#33796,#33797,#33798,#33799,#33800,#33801,#33802,#33803,
#33804,#33805,#33806,#33807,#33808,#33809,#33810,#33811,#33812,#33813,#33814,
#33815,#33816,#33817,#33818,#33819,#33820,#33821,#33822,#33823,#33824,#33825,
#33826,#33827,#33828,#33829,#33830,#33831,#33832,#33833,#33834,#33835,#33836,
#33837,#33838,#33839,#33840,#33841,#33842),(#33843,#33844,#33845,#33846,
#33847,#33848,#33849,#33850,#33851,#33852,#33853,#33854,#33855,#33856,#33857,
#33858,#33859,#33860,#33861,#33862,#33863,#33864,#33865,#33866,#33867,#33868,
#33869,#33870,#33871,#33872,#33873,#33874,#33875,#33876,#33877,#33878,#33879,
#33880,#33881,#33882,#33883,#33884,#33885,#33886,#33887,#33888,#33889,#33890,
#33891,#33892,#33893,#33894,#33895,#33896,#33897,#33898,#33899,#33900,#33901,
#33902,#33903,#33904,#33905,#33906,#33907,#33908,#33909,#33910,#33911,#33912,
#33913,#33914,#33915,#33916,#33917,#33918,#33919,#33920,#33921,#33922,#33923,
#33924,#33925,#33926,#33927,#33928,#33929,#33930,#33931,#33932,#33933,#33934,
#33935,#33936,#33937,#33938,#33939,#33940,#33941,#33942,#33943,#33944,#33945,
#33946),(#33947,#33948,#33949,#33950,#33951,#33952,#33953,#33954,#33955,
#33956,#33957,#33958,#33959,#33960,#33961,#33962,#33963,#33964,#33965,#33966,
#33967,#33968,#33969,#33970,#33971,#33972,#33973,#33974,#33975,#33976,#33977,
#33978,#33979,#33980,#33981,#33982,#33983,#33984,#33985,#33986,#33987,#33988,
#33989,#33990,#33991,#33992,#33993,#33994,#33995,#33996,#33997,#33998,#33999,
#34000,#34001,#34002,#34003,#34004,#34005,#34006,#34007,#34008,#34009,#34010,
#34011,#34012,#34013,#34014,#34015,#34016,#34017,#34018,#34019,#34020,#34021,
#34022,#34023,#34024,#34025,#34026,#34027,#34028,#34029,#34030,#34031,#34032,
#34033,#34034,#34035,#34036,#34037,#34038,#34039,#34040,#34041,#34042,#34043,
#34044,#34045,#34046,#34047,#34048,#34049,#34050)),.UNSPECIFIED.,.F.,.F.,
 .F.,(4,4),(4,1,1,1,1,1,1,1,1,1,1,1,1,1,1,1,1,1,1,1,1,1,1,1,1,1,1,1,1,1,
1,1,1,1,1,1,1,1,1,1,1,1,1,1,1,1,1,1,1,1,1,1,1,1,1,1,1,1,1,1,1,1,1,1,1,1,
1,1,1,1,1,1,1,1,1,1,1,1,1,1,1,1,1,1,1,1,1,1,1,1,1,1,1,1,1,1,1,1,1,1,1,4),
(0.,0.0448889834294935),(11.8615800042566,12.8591085386932,13.8566370731298,
14.8541656075664,15.851694142003,16.8492226764396,17.8467512108762,18.8442797453128,
19.8418082797494,20.839336814186,21.8368653486226,22.8343938830592,23.8319224174958,
24.8294509519324,25.826979486369,26.8245080208056,27.8220365552422,28.8195650896788,
29.8170936241154,30.814622158552,31.8121506929886,32.8096792274252,33.8072077618618,
34.8047362962984,35.802264830735,36.7997933651716,37.7973218996082,38.7948504340448,
39.7923789684814,40.789907502918,41.7874360373546,42.7849645717912,43.7824931062278,
44.7800216406644,45.777550175101,46.7750787095376,47.7726072439742,48.7701357784108,
49.7676643128474,50.765192847284,51.7627213817206,52.7602499161572,53.7577784505938,
54.7553069850304,55.752835519467,56.7503640539036,57.7478925883402,58.7454211227768,
59.7429496572134,60.74047819165,61.7380067260866,62.7355352605232,63.7330637949598,
64.7305923293964,65.728120863833,66.7256493982696,67.7231779327062,68.7207064671428,
69.7182350015794,70.715763536016,71.7132920704526,72.7108206048892,73.7083491393258,
74.7058776737624,75.703406208199,76.7009347426356,77.6984632770722,78.6959918115088,
79.6935203459454,80.691048880382,81.6885774148186,82.6861059492552,83.6836344836918,
84.6811630181284,85.678691552565,86.6762200870016,87.6737486214382,88.6712771558748,
89.6688056903114,90.666334224748,91.6638627591846,92.6613912936212,93.6589198280578,
94.6564483624944,95.653976896931,96.6515054313676,97.6490339658042,98.6465625002408,
99.6440910346774,100.641619569114,101.639148103551,102.636676637987,103.634205172424,
104.63173370686,105.629262241297,106.626790775734,107.62431931017,108.621847844607,
109.619376379043,110.61690491348,111.614433447917,112.611961982353),
 .UNSPECIFIED.);
#596=B_SPLINE_SURFACE_WITH_KNOTS('',3,3,((#34158,#34159,#34160,#34161,#34162,
#34163,#34164,#34165,#34166,#34167,#34168,#34169,#34170,#34171,#34172,#34173,
#34174,#34175,#34176,#34177,#34178,#34179,#34180,#34181,#34182,#34183,#34184,
#34185,#34186,#34187,#34188,#34189,#34190,#34191,#34192,#34193,#34194,#34195,
#34196,#34197,#34198,#34199,#34200,#34201,#34202,#34203,#34204,#34205,#34206,
#34207,#34208,#34209,#34210,#34211,#34212,#34213,#34214,#34215,#34216,#34217,
#34218,#34219,#34220,#34221,#34222,#34223,#34224,#34225,#34226,#34227,#34228,
#34229,#34230,#34231,#34232,#34233,#34234,#34235,#34236,#34237,#34238,#34239,
#34240,#34241,#34242,#34243,#34244,#34245,#34246,#34247,#34248,#34249,#34250,
#34251,#34252,#34253,#34254,#34255,#34256,#34257,#34258,#34259,#34260,#34261),
(#34262,#34263,#34264,#34265,#34266,#34267,#34268,#34269,#34270,#34271,
#34272,#34273,#34274,#34275,#34276,#34277,#34278,#34279,#34280,#34281,#34282,
#34283,#34284,#34285,#34286,#34287,#34288,#34289,#34290,#34291,#34292,#34293,
#34294,#34295,#34296,#34297,#34298,#34299,#34300,#34301,#34302,#34303,#34304,
#34305,#34306,#34307,#34308,#34309,#34310,#34311,#34312,#34313,#34314,#34315,
#34316,#34317,#34318,#34319,#34320,#34321,#34322,#34323,#34324,#34325,#34326,
#34327,#34328,#34329,#34330,#34331,#34332,#34333,#34334,#34335,#34336,#34337,
#34338,#34339,#34340,#34341,#34342,#34343,#34344,#34345,#34346,#34347,#34348,
#34349,#34350,#34351,#34352,#34353,#34354,#34355,#34356,#34357,#34358,#34359,
#34360,#34361,#34362,#34363,#34364,#34365),(#34366,#34367,#34368,#34369,
#34370,#34371,#34372,#34373,#34374,#34375,#34376,#34377,#34378,#34379,#34380,
#34381,#34382,#34383,#34384,#34385,#34386,#34387,#34388,#34389,#34390,#34391,
#34392,#34393,#34394,#34395,#34396,#34397,#34398,#34399,#34400,#34401,#34402,
#34403,#34404,#34405,#34406,#34407,#34408,#34409,#34410,#34411,#34412,#34413,
#34414,#34415,#34416,#34417,#34418,#34419,#34420,#34421,#34422,#34423,#34424,
#34425,#34426,#34427,#34428,#34429,#34430,#34431,#34432,#34433,#34434,#34435,
#34436,#34437,#34438,#34439,#34440,#34441,#34442,#34443,#34444,#34445,#34446,
#34447,#34448,#34449,#34450,#34451,#34452,#34453,#34454,#34455,#34456,#34457,
#34458,#34459,#34460,#34461,#34462,#34463,#34464,#34465,#34466,#34467,#34468,
#34469),(#34470,#34471,#34472,#34473,#34474,#34475,#34476,#34477,#34478,
#34479,#34480,#34481,#34482,#34483,#34484,#34485,#34486,#34487,#34488,#34489,
#34490,#34491,#34492,#34493,#34494,#34495,#34496,#34497,#34498,#34499,#34500,
#34501,#34502,#34503,#34504,#34505,#34506,#34507,#34508,#34509,#34510,#34511,
#34512,#34513,#34514,#34515,#34516,#34517,#34518,#34519,#34520,#34521,#34522,
#34523,#34524,#34525,#34526,#34527,#34528,#34529,#34530,#34531,#34532,#34533,
#34534,#34535,#34536,#34537,#34538,#34539,#34540,#34541,#34542,#34543,#34544,
#34545,#34546,#34547,#34548,#34549,#34550,#34551,#34552,#34553,#34554,#34555,
#34556,#34557,#34558,#34559,#34560,#34561,#34562,#34563,#34564,#34565,#34566,
#34567,#34568,#34569,#34570,#34571,#34572,#34573)),.UNSPECIFIED.,.F.,.F.,
 .F.,(4,4),(4,1,1,1,1,1,1,1,1,1,1,1,1,1,1,1,1,1,1,1,1,1,1,1,1,1,1,1,1,1,
1,1,1,1,1,1,1,1,1,1,1,1,1,1,1,1,1,1,1,1,1,1,1,1,1,1,1,1,1,1,1,1,1,1,1,1,
1,1,1,1,1,1,1,1,1,1,1,1,1,1,1,1,1,1,1,1,1,1,1,1,1,1,1,1,1,1,1,1,1,1,1,4),
(0.,0.0448889834294935),(14.3981410127769,15.3956695472135,16.3931980816501,
17.3907266160867,18.3882551505233,19.3857836849599,20.3833122193965,21.3808407538331,
22.3783692882697,23.3758978227063,24.3734263571429,25.3709548915795,26.3684834260161,
27.3660119604527,28.3635404948893,29.3610690293259,30.3585975637625,31.3561260981991,
32.3536546326357,33.3511831670723,34.3487117015089,35.3462402359455,36.3437687703821,
37.3412973048187,38.3388258392553,39.3363543736919,40.3338829081285,41.3314114425651,
42.3289399770017,43.3264685114383,44.3239970458749,45.3215255803115,46.3190541147481,
47.3165826491847,48.3141111836213,49.3116397180578,50.3091682524944,51.3066967869311,
52.3042253213677,53.3017538558043,54.2992823902408,55.2968109246774,56.294339459114,
57.2918679935507,58.2893965279873,59.2869250624238,60.2844535968604,61.281982131297,
62.2795106657336,63.2770392001703,64.2745677346068,65.2720962690434,66.26962480348,
67.2671533379166,68.2646818723533,69.2622104067898,70.2597389412264,71.257267475663,
72.2547960100996,73.2523245445362,74.2498530789728,75.2473816134094,76.244910147846,
77.2424386822826,78.2399672167192,79.2374957511558,80.2350242855924,81.232552820029,
82.2300813544656,83.2276098889022,84.2251384233388,85.2226669577754,86.220195492212,
87.2177240266486,88.2152525610852,89.2127810955218,90.2103096299584,91.207838164395,
92.2053666988316,93.2028952332682,94.2004237677048,95.1979523021414,96.195480836578,
97.1930093710146,98.1905379054512,99.1880664398878,100.185594974324,101.183123508761,
102.180652043198,103.178180577634,104.175709112071,105.173237646507,106.170766180944,
107.168294715381,108.165823249817,109.163351784254,110.16088031869,111.158408853127,
112.155937387564,113.153465922,114.150994456437,115.148522990873),
 .UNSPECIFIED.);
#603=FACE_OUTER_BOUND('',#1147,.T.);
#604=FACE_OUTER_BOUND('',#1148,.T.);
#605=FACE_OUTER_BOUND('',#1149,.T.);
#606=FACE_OUTER_BOUND('',#1150,.T.);
#607=FACE_OUTER_BOUND('',#1151,.T.);
#608=FACE_OUTER_BOUND('',#1152,.T.);
#609=FACE_OUTER_BOUND('',#1153,.T.);
#610=FACE_OUTER_BOUND('',#1154,.T.);
#611=FACE_OUTER_BOUND('',#1155,.T.);
#612=FACE_OUTER_BOUND('',#1156,.T.);
#613=FACE_OUTER_BOUND('',#1157,.T.);
#614=FACE_OUTER_BOUND('',#1158,.T.);
#615=FACE_OUTER_BOUND('',#1159,.T.);
#616=FACE_OUTER_BOUND('',#1160,.T.);
#617=FACE_OUTER_BOUND('',#1161,.T.);
#618=FACE_OUTER_BOUND('',#1162,.T.);
#619=FACE_OUTER_BOUND('',#1163,.T.);
#620=FACE_OUTER_BOUND('',#1164,.T.);
#621=FACE_OUTER_BOUND('',#1165,.T.);
#622=FACE_OUTER_BOUND('',#1166,.T.);
#623=FACE_OUTER_BOUND('',#1167,.T.);
#624=FACE_OUTER_BOUND('',#1168,.T.);
#625=FACE_OUTER_BOUND('',#1169,.T.);
#626=FACE_OUTER_BOUND('',#1170,.T.);
#627=FACE_OUTER_BOUND('',#1171,.T.);
#628=FACE_OUTER_BOUND('',#1172,.T.);
#629=FACE_OUTER_BOUND('',#1173,.T.);
#630=FACE_OUTER_BOUND('',#1174,.T.);
#631=FACE_OUTER_BOUND('',#1175,.T.);
#632=FACE_OUTER_BOUND('',#1176,.T.);
#633=FACE_OUTER_BOUND('',#1177,.T.);
#634=FACE_OUTER_BOUND('',#1178,.T.);
#635=FACE_OUTER_BOUND('',#1179,.T.);
#636=FACE_OUTER_BOUND('',#1180,.T.);
#637=FACE_OUTER_BOUND('',#1181,.T.);
#638=FACE_OUTER_BOUND('',#1182,.T.);
#639=FACE_OUTER_BOUND('',#1183,.T.);
#640=FACE_OUTER_BOUND('',#1184,.T.);
#641=FACE_OUTER_BOUND('',#1185,.T.);
#642=FACE_OUTER_BOUND('',#1186,.T.);
#643=FACE_OUTER_BOUND('',#1187,.T.);
#644=FACE_OUTER_BOUND('',#1188,.T.);
#645=FACE_OUTER_BOUND('',#1189,.T.);
#646=FACE_OUTER_BOUND('',#1190,.T.);
#647=FACE_OUTER_BOUND('',#1191,.T.);
#648=FACE_OUTER_BOUND('',#1192,.T.);
#649=FACE_OUTER_BOUND('',#1193,.T.);
#650=FACE_OUTER_BOUND('',#1194,.T.);
#651=FACE_OUTER_BOUND('',#1195,.T.);
#652=FACE_OUTER_BOUND('',#1196,.T.);
#653=FACE_OUTER_BOUND('',#1197,.T.);
#654=FACE_OUTER_BOUND('',#1198,.T.);
#655=FACE_OUTER_BOUND('',#1199,.T.);
#656=FACE_OUTER_BOUND('',#1200,.T.);
#657=FACE_OUTER_BOUND('',#1201,.T.);
#658=FACE_OUTER_BOUND('',#1202,.T.);
#659=FACE_OUTER_BOUND('',#1203,.T.);
#660=FACE_OUTER_BOUND('',#1204,.T.);
#661=FACE_OUTER_BOUND('',#1205,.T.);
#662=FACE_OUTER_BOUND('',#1206,.T.);
#663=FACE_OUTER_BOUND('',#1207,.T.);
#664=FACE_OUTER_BOUND('',#1208,.T.);
#665=FACE_OUTER_BOUND('',#1209,.T.);
#666=FACE_OUTER_BOUND('',#1210,.T.);
#667=FACE_OUTER_BOUND('',#1211,.T.);
#668=FACE_OUTER_BOUND('',#1212,.T.);
#669=FACE_OUTER_BOUND('',#1213,.T.);
#670=FACE_OUTER_BOUND('',#1214,.T.);
#671=FACE_OUTER_BOUND('',#1215,.T.);
#672=FACE_OUTER_BOUND('',#1216,.T.);
#673=FACE_OUTER_BOUND('',#1217,.T.);
#674=FACE_OUTER_BOUND('',#1218,.T.);
#675=FACE_OUTER_BOUND('',#1219,.T.);
#676=FACE_OUTER_BOUND('',#1220,.T.);
#677=FACE_OUTER_BOUND('',#1221,.T.);
#678=FACE_OUTER_BOUND('',#1222,.T.);
#679=FACE_OUTER_BOUND('',#1223,.T.);
#680=FACE_OUTER_BOUND('',#1224,.T.);
#681=FACE_OUTER_BOUND('',#1225,.T.);
#682=FACE_OUTER_BOUND('',#1226,.T.);
#683=FACE_OUTER_BOUND('',#1227,.T.);
#684=FACE_OUTER_BOUND('',#1228,.T.);
#685=FACE_OUTER_BOUND('',#1229,.T.);
#686=FACE_OUTER_BOUND('',#1230,.T.);
#687=FACE_OUTER_BOUND('',#1231,.T.);
#688=FACE_OUTER_BOUND('',#1232,.T.);
#689=FACE_OUTER_BOUND('',#1233,.T.);
#690=FACE_OUTER_BOUND('',#1234,.T.);
#691=FACE_OUTER_BOUND('',#1235,.T.);
#692=FACE_OUTER_BOUND('',#1236,.T.);
#693=FACE_OUTER_BOUND('',#1237,.T.);
#694=FACE_OUTER_BOUND('',#1238,.T.);
#695=FACE_OUTER_BOUND('',#1239,.T.);
#696=FACE_OUTER_BOUND('',#1240,.T.);
#697=FACE_OUTER_BOUND('',#1241,.T.);
#698=FACE_OUTER_BOUND('',#1242,.T.);
#699=FACE_OUTER_BOUND('',#1243,.T.);
#700=FACE_OUTER_BOUND('',#1244,.T.);
#701=FACE_OUTER_BOUND('',#1245,.T.);
#702=FACE_OUTER_BOUND('',#1246,.T.);
#703=FACE_OUTER_BOUND('',#1247,.T.);
#704=FACE_OUTER_BOUND('',#1248,.T.);
#705=FACE_OUTER_BOUND('',#1249,.T.);
#706=FACE_OUTER_BOUND('',#1250,.T.);
#707=FACE_OUTER_BOUND('',#1251,.T.);
#708=FACE_OUTER_BOUND('',#1252,.T.);
#709=FACE_OUTER_BOUND('',#1253,.T.);
#710=FACE_OUTER_BOUND('',#1254,.T.);
#711=FACE_OUTER_BOUND('',#1255,.T.);
#712=FACE_OUTER_BOUND('',#1256,.T.);
#713=FACE_OUTER_BOUND('',#1257,.T.);
#714=FACE_OUTER_BOUND('',#1258,.T.);
#715=FACE_OUTER_BOUND('',#1259,.T.);
#716=FACE_OUTER_BOUND('',#1260,.T.);
#717=FACE_OUTER_BOUND('',#1261,.T.);
#718=FACE_OUTER_BOUND('',#1262,.T.);
#719=FACE_OUTER_BOUND('',#1263,.T.);
#720=FACE_OUTER_BOUND('',#1264,.T.);
#721=FACE_OUTER_BOUND('',#1265,.T.);
#722=FACE_OUTER_BOUND('',#1266,.T.);
#723=FACE_OUTER_BOUND('',#1267,.T.);
#724=FACE_OUTER_BOUND('',#1268,.T.);
#725=FACE_OUTER_BOUND('',#1269,.T.);
#726=FACE_OUTER_BOUND('',#1270,.T.);
#727=FACE_OUTER_BOUND('',#1271,.T.);
#728=FACE_OUTER_BOUND('',#1272,.T.);
#729=FACE_OUTER_BOUND('',#1273,.T.);
#730=FACE_OUTER_BOUND('',#1274,.T.);
#731=FACE_OUTER_BOUND('',#1275,.T.);
#732=FACE_OUTER_BOUND('',#1276,.T.);
#733=FACE_OUTER_BOUND('',#1277,.T.);
#734=FACE_OUTER_BOUND('',#1278,.T.);
#735=FACE_OUTER_BOUND('',#1279,.T.);
#736=FACE_OUTER_BOUND('',#1280,.T.);
#737=FACE_OUTER_BOUND('',#1281,.T.);
#738=FACE_OUTER_BOUND('',#1282,.T.);
#739=FACE_OUTER_BOUND('',#1283,.T.);
#740=FACE_OUTER_BOUND('',#1284,.T.);
#741=FACE_OUTER_BOUND('',#1285,.T.);
#742=FACE_OUTER_BOUND('',#1286,.T.);
#743=FACE_OUTER_BOUND('',#1287,.T.);
#744=FACE_OUTER_BOUND('',#1288,.T.);
#745=FACE_OUTER_BOUND('',#1289,.T.);
#746=FACE_OUTER_BOUND('',#1290,.T.);
#747=FACE_OUTER_BOUND('',#1291,.T.);
#748=FACE_OUTER_BOUND('',#1292,.T.);
#749=FACE_OUTER_BOUND('',#1293,.T.);
#750=FACE_OUTER_BOUND('',#1294,.T.);
#751=FACE_OUTER_BOUND('',#1295,.T.);
#752=FACE_OUTER_BOUND('',#1296,.T.);
#753=FACE_OUTER_BOUND('',#1297,.T.);
#754=FACE_OUTER_BOUND('',#1298,.T.);
#755=FACE_OUTER_BOUND('',#1299,.T.);
#756=FACE_OUTER_BOUND('',#1300,.T.);
#757=FACE_OUTER_BOUND('',#1301,.T.);
#758=FACE_OUTER_BOUND('',#1302,.T.);
#759=FACE_OUTER_BOUND('',#1303,.T.);
#760=FACE_OUTER_BOUND('',#1304,.T.);
#761=FACE_OUTER_BOUND('',#1305,.T.);
#762=FACE_OUTER_BOUND('',#1306,.T.);
#763=FACE_OUTER_BOUND('',#1307,.T.);
#764=FACE_OUTER_BOUND('',#1308,.T.);
#765=FACE_OUTER_BOUND('',#1309,.T.);
#766=FACE_OUTER_BOUND('',#1310,.T.);
#767=FACE_OUTER_BOUND('',#1311,.T.);
#768=FACE_OUTER_BOUND('',#1312,.T.);
#769=FACE_OUTER_BOUND('',#1313,.T.);
#770=FACE_OUTER_BOUND('',#1314,.T.);
#771=FACE_OUTER_BOUND('',#1315,.T.);
#772=FACE_OUTER_BOUND('',#1316,.T.);
#773=FACE_OUTER_BOUND('',#1317,.T.);
#774=FACE_OUTER_BOUND('',#1318,.T.);
#775=FACE_OUTER_BOUND('',#1319,.T.);
#776=FACE_OUTER_BOUND('',#1320,.T.);
#777=FACE_OUTER_BOUND('',#1321,.T.);
#778=FACE_OUTER_BOUND('',#1322,.T.);
#779=FACE_OUTER_BOUND('',#1323,.T.);
#780=FACE_OUTER_BOUND('',#1324,.T.);
#781=FACE_OUTER_BOUND('',#1325,.T.);
#782=FACE_OUTER_BOUND('',#1326,.T.);
#783=FACE_OUTER_BOUND('',#1327,.T.);
#784=FACE_OUTER_BOUND('',#1328,.T.);
#785=FACE_OUTER_BOUND('',#1329,.T.);
#786=FACE_OUTER_BOUND('',#1330,.T.);
#787=FACE_OUTER_BOUND('',#1331,.T.);
#788=FACE_OUTER_BOUND('',#1332,.T.);
#789=FACE_OUTER_BOUND('',#1333,.T.);
#790=FACE_OUTER_BOUND('',#1334,.T.);
#791=FACE_OUTER_BOUND('',#1335,.T.);
#792=FACE_OUTER_BOUND('',#1336,.T.);
#793=FACE_OUTER_BOUND('',#1337,.T.);
#794=FACE_OUTER_BOUND('',#1338,.T.);
#795=FACE_OUTER_BOUND('',#1339,.T.);
#796=FACE_OUTER_BOUND('',#1340,.T.);
#797=FACE_OUTER_BOUND('',#1341,.T.);
#798=FACE_OUTER_BOUND('',#1342,.T.);
#799=FACE_OUTER_BOUND('',#1343,.T.);
#800=FACE_OUTER_BOUND('',#1344,.T.);
#801=FACE_OUTER_BOUND('',#1345,.T.);
#802=FACE_OUTER_BOUND('',#1346,.T.);
#803=FACE_OUTER_BOUND('',#1347,.T.);
#804=FACE_OUTER_BOUND('',#1348,.T.);
#805=FACE_OUTER_BOUND('',#1349,.T.);
#806=FACE_OUTER_BOUND('',#1350,.T.);
#807=FACE_OUTER_BOUND('',#1351,.T.);
#808=FACE_OUTER_BOUND('',#1352,.T.);
#809=FACE_OUTER_BOUND('',#1353,.T.);
#810=FACE_OUTER_BOUND('',#1354,.T.);
#811=FACE_OUTER_BOUND('',#1355,.T.);
#812=FACE_OUTER_BOUND('',#1356,.T.);
#813=FACE_OUTER_BOUND('',#1357,.T.);
#814=FACE_OUTER_BOUND('',#1358,.T.);
#815=FACE_OUTER_BOUND('',#1359,.T.);
#816=FACE_OUTER_BOUND('',#1360,.T.);
#817=FACE_OUTER_BOUND('',#1361,.T.);
#818=FACE_OUTER_BOUND('',#1362,.T.);
#819=FACE_OUTER_BOUND('',#1363,.T.);
#820=FACE_OUTER_BOUND('',#1364,.T.);
#821=FACE_OUTER_BOUND('',#1365,.T.);
#822=FACE_OUTER_BOUND('',#1366,.T.);
#823=FACE_OUTER_BOUND('',#1367,.T.);
#824=FACE_OUTER_BOUND('',#1368,.T.);
#825=FACE_OUTER_BOUND('',#1369,.T.);
#826=FACE_OUTER_BOUND('',#1370,.T.);
#827=FACE_OUTER_BOUND('',#1371,.T.);
#828=FACE_OUTER_BOUND('',#1372,.T.);
#829=FACE_OUTER_BOUND('',#1373,.T.);
#830=FACE_OUTER_BOUND('',#1374,.T.);
#831=FACE_OUTER_BOUND('',#1375,.T.);
#832=FACE_OUTER_BOUND('',#1376,.T.);
#833=FACE_OUTER_BOUND('',#1377,.T.);
#834=FACE_OUTER_BOUND('',#1378,.T.);
#835=FACE_OUTER_BOUND('',#1379,.T.);
#836=FACE_OUTER_BOUND('',#1380,.T.);
#837=FACE_OUTER_BOUND('',#1381,.T.);
#838=FACE_OUTER_BOUND('',#1382,.T.);
#839=FACE_OUTER_BOUND('',#1383,.T.);
#840=FACE_OUTER_BOUND('',#1384,.T.);
#841=FACE_OUTER_BOUND('',#1385,.T.);
#842=FACE_OUTER_BOUND('',#1386,.T.);
#843=FACE_OUTER_BOUND('',#1387,.T.);
#844=FACE_OUTER_BOUND('',#1388,.T.);
#845=FACE_OUTER_BOUND('',#1389,.T.);
#846=FACE_OUTER_BOUND('',#1390,.T.);
#847=FACE_OUTER_BOUND('',#1391,.T.);
#848=FACE_OUTER_BOUND('',#1392,.T.);
#849=FACE_OUTER_BOUND('',#1393,.T.);
#850=FACE_OUTER_BOUND('',#1394,.T.);
#851=FACE_OUTER_BOUND('',#1395,.T.);
#852=FACE_OUTER_BOUND('',#1396,.T.);
#853=FACE_OUTER_BOUND('',#1397,.T.);
#854=FACE_OUTER_BOUND('',#1398,.T.);
#855=FACE_OUTER_BOUND('',#1399,.T.);
#856=FACE_OUTER_BOUND('',#1400,.T.);
#857=FACE_OUTER_BOUND('',#1401,.T.);
#858=FACE_OUTER_BOUND('',#1402,.T.);
#859=FACE_OUTER_BOUND('',#1403,.T.);
#860=FACE_OUTER_BOUND('',#1404,.T.);
#861=FACE_OUTER_BOUND('',#1405,.T.);
#862=FACE_OUTER_BOUND('',#1406,.T.);
#863=FACE_OUTER_BOUND('',#1407,.T.);
#864=FACE_OUTER_BOUND('',#1408,.T.);
#865=FACE_OUTER_BOUND('',#1409,.T.);
#866=FACE_OUTER_BOUND('',#1410,.T.);
#867=FACE_OUTER_BOUND('',#1412,.T.);
#868=FACE_OUTER_BOUND('',#1413,.T.);
#869=FACE_OUTER_BOUND('',#1414,.T.);
#870=FACE_OUTER_BOUND('',#1420,.T.);
#871=FACE_OUTER_BOUND('',#1421,.T.);
#872=FACE_OUTER_BOUND('',#1422,.T.);
#873=FACE_OUTER_BOUND('',#1423,.T.);
#874=FACE_OUTER_BOUND('',#1424,.T.);
#875=FACE_OUTER_BOUND('',#1425,.T.);
#876=FACE_OUTER_BOUND('',#1426,.T.);
#877=FACE_OUTER_BOUND('',#1427,.T.);
#878=FACE_OUTER_BOUND('',#1428,.T.);
#879=FACE_OUTER_BOUND('',#1429,.T.);
#880=FACE_OUTER_BOUND('',#1430,.T.);
#881=FACE_OUTER_BOUND('',#1431,.T.);
#882=FACE_OUTER_BOUND('',#1432,.T.);
#883=FACE_OUTER_BOUND('',#1433,.T.);
#884=FACE_OUTER_BOUND('',#1434,.T.);
#885=FACE_OUTER_BOUND('',#1435,.T.);
#886=FACE_OUTER_BOUND('',#1436,.T.);
#887=FACE_OUTER_BOUND('',#1437,.T.);
#888=FACE_OUTER_BOUND('',#1438,.T.);
#889=FACE_OUTER_BOUND('',#1439,.T.);
#890=FACE_OUTER_BOUND('',#1440,.T.);
#891=FACE_OUTER_BOUND('',#1441,.T.);
#892=FACE_OUTER_BOUND('',#1442,.T.);
#893=FACE_OUTER_BOUND('',#1443,.T.);
#894=FACE_OUTER_BOUND('',#1444,.T.);
#895=FACE_OUTER_BOUND('',#1445,.T.);
#896=FACE_OUTER_BOUND('',#1446,.T.);
#897=FACE_OUTER_BOUND('',#1447,.T.);
#898=FACE_OUTER_BOUND('',#1448,.T.);
#899=FACE_OUTER_BOUND('',#1449,.T.);
#900=FACE_OUTER_BOUND('',#1450,.T.);
#901=FACE_OUTER_BOUND('',#1451,.T.);
#902=FACE_OUTER_BOUND('',#1452,.T.);
#903=FACE_OUTER_BOUND('',#1453,.T.);
#904=FACE_OUTER_BOUND('',#1454,.T.);
#905=FACE_OUTER_BOUND('',#1455,.T.);
#906=FACE_OUTER_BOUND('',#1456,.T.);
#907=FACE_OUTER_BOUND('',#1457,.T.);
#908=FACE_OUTER_BOUND('',#1458,.T.);
#909=FACE_OUTER_BOUND('',#1459,.T.);
#910=FACE_OUTER_BOUND('',#1460,.T.);
#911=FACE_OUTER_BOUND('',#1461,.T.);
#912=FACE_OUTER_BOUND('',#1462,.T.);
#913=FACE_OUTER_BOUND('',#1463,.T.);
#914=FACE_OUTER_BOUND('',#1464,.T.);
#915=FACE_OUTER_BOUND('',#1465,.T.);
#916=FACE_OUTER_BOUND('',#1466,.T.);
#917=FACE_OUTER_BOUND('',#1467,.T.);
#918=FACE_OUTER_BOUND('',#1468,.T.);
#919=FACE_OUTER_BOUND('',#1469,.T.);
#920=FACE_OUTER_BOUND('',#1470,.T.);
#921=FACE_OUTER_BOUND('',#1471,.T.);
#922=FACE_OUTER_BOUND('',#1472,.T.);
#923=FACE_OUTER_BOUND('',#1473,.T.);
#924=FACE_OUTER_BOUND('',#1474,.T.);
#925=FACE_OUTER_BOUND('',#1475,.T.);
#926=FACE_OUTER_BOUND('',#1476,.T.);
#927=FACE_OUTER_BOUND('',#1477,.T.);
#928=FACE_OUTER_BOUND('',#1478,.T.);
#929=FACE_OUTER_BOUND('',#1479,.T.);
#930=FACE_OUTER_BOUND('',#1480,.T.);
#931=FACE_OUTER_BOUND('',#1481,.T.);
#932=FACE_OUTER_BOUND('',#1482,.T.);
#933=FACE_OUTER_BOUND('',#1483,.T.);
#934=FACE_OUTER_BOUND('',#1484,.T.);
#935=FACE_OUTER_BOUND('',#1485,.T.);
#936=FACE_OUTER_BOUND('',#1486,.T.);
#937=FACE_OUTER_BOUND('',#1487,.T.);
#938=FACE_OUTER_BOUND('',#1488,.T.);
#939=FACE_OUTER_BOUND('',#1489,.T.);
#940=FACE_OUTER_BOUND('',#1490,.T.);
#941=FACE_OUTER_BOUND('',#1491,.T.);
#942=FACE_OUTER_BOUND('',#1510,.T.);
#943=FACE_OUTER_BOUND('',#1511,.T.);
#944=FACE_OUTER_BOUND('',#1512,.T.);
#945=FACE_OUTER_BOUND('',#1514,.T.);
#946=FACE_OUTER_BOUND('',#1515,.T.);
#947=FACE_OUTER_BOUND('',#1534,.T.);
#948=FACE_OUTER_BOUND('',#1535,.T.);
#949=FACE_OUTER_BOUND('',#1536,.T.);
#1147=EDGE_LOOP('',(#6389,#6390,#6391,#6392,#6393,#6394,#6395,#6396));
#1148=EDGE_LOOP('',(#6397,#6398,#6399,#6400));
#1149=EDGE_LOOP('',(#6401,#6402,#6403,#6404));
#1150=EDGE_LOOP('',(#6405,#6406,#6407,#6408));
#1151=EDGE_LOOP('',(#6409,#6410,#6411,#6412));
#1152=EDGE_LOOP('',(#6413,#6414,#6415,#6416));
#1153=EDGE_LOOP('',(#6417,#6418,#6419,#6420));
#1154=EDGE_LOOP('',(#6421,#6422,#6423,#6424));
#1155=EDGE_LOOP('',(#6425,#6426,#6427,#6428));
#1156=EDGE_LOOP('',(#6429,#6430,#6431,#6432));
#1157=EDGE_LOOP('',(#6433,#6434,#6435,#6436));
#1158=EDGE_LOOP('',(#6437,#6438,#6439,#6440));
#1159=EDGE_LOOP('',(#6441,#6442,#6443,#6444));
#1160=EDGE_LOOP('',(#6445,#6446,#6447,#6448));
#1161=EDGE_LOOP('',(#6449,#6450,#6451,#6452));
#1162=EDGE_LOOP('',(#6453,#6454,#6455,#6456));
#1163=EDGE_LOOP('',(#6457,#6458,#6459,#6460));
#1164=EDGE_LOOP('',(#6461,#6462,#6463,#6464));
#1165=EDGE_LOOP('',(#6465,#6466,#6467,#6468));
#1166=EDGE_LOOP('',(#6469,#6470,#6471,#6472));
#1167=EDGE_LOOP('',(#6473,#6474,#6475,#6476));
#1168=EDGE_LOOP('',(#6477,#6478,#6479,#6480));
#1169=EDGE_LOOP('',(#6481,#6482,#6483,#6484));
#1170=EDGE_LOOP('',(#6485,#6486,#6487,#6488));
#1171=EDGE_LOOP('',(#6489,#6490,#6491,#6492));
#1172=EDGE_LOOP('',(#6493,#6494,#6495,#6496));
#1173=EDGE_LOOP('',(#6497,#6498,#6499,#6500));
#1174=EDGE_LOOP('',(#6501,#6502,#6503,#6504));
#1175=EDGE_LOOP('',(#6505,#6506,#6507,#6508));
#1176=EDGE_LOOP('',(#6509,#6510,#6511,#6512));
#1177=EDGE_LOOP('',(#6513,#6514,#6515,#6516));
#1178=EDGE_LOOP('',(#6517,#6518,#6519,#6520,#6521,#6522,#6523,#6524));
#1179=EDGE_LOOP('',(#6525,#6526,#6527,#6528));
#1180=EDGE_LOOP('',(#6529,#6530,#6531,#6532));
#1181=EDGE_LOOP('',(#6533,#6534,#6535,#6536));
#1182=EDGE_LOOP('',(#6537,#6538,#6539,#6540));
#1183=EDGE_LOOP('',(#6541,#6542,#6543,#6544));
#1184=EDGE_LOOP('',(#6545,#6546,#6547,#6548));
#1185=EDGE_LOOP('',(#6549,#6550,#6551,#6552));
#1186=EDGE_LOOP('',(#6553,#6554,#6555,#6556));
#1187=EDGE_LOOP('',(#6557,#6558,#6559,#6560));
#1188=EDGE_LOOP('',(#6561,#6562,#6563,#6564));
#1189=EDGE_LOOP('',(#6565,#6566,#6567,#6568));
#1190=EDGE_LOOP('',(#6569,#6570,#6571,#6572));
#1191=EDGE_LOOP('',(#6573,#6574,#6575,#6576));
#1192=EDGE_LOOP('',(#6577,#6578,#6579,#6580));
#1193=EDGE_LOOP('',(#6581,#6582,#6583,#6584));
#1194=EDGE_LOOP('',(#6585,#6586,#6587,#6588));
#1195=EDGE_LOOP('',(#6589,#6590,#6591,#6592));
#1196=EDGE_LOOP('',(#6593,#6594,#6595,#6596));
#1197=EDGE_LOOP('',(#6597,#6598,#6599,#6600));
#1198=EDGE_LOOP('',(#6601,#6602,#6603,#6604));
#1199=EDGE_LOOP('',(#6605,#6606,#6607,#6608));
#1200=EDGE_LOOP('',(#6609,#6610,#6611,#6612));
#1201=EDGE_LOOP('',(#6613,#6614,#6615,#6616));
#1202=EDGE_LOOP('',(#6617,#6618,#6619,#6620));
#1203=EDGE_LOOP('',(#6621,#6622,#6623,#6624));
#1204=EDGE_LOOP('',(#6625,#6626,#6627,#6628));
#1205=EDGE_LOOP('',(#6629,#6630,#6631,#6632));
#1206=EDGE_LOOP('',(#6633,#6634,#6635,#6636));
#1207=EDGE_LOOP('',(#6637,#6638,#6639,#6640));
#1208=EDGE_LOOP('',(#6641,#6642,#6643,#6644));
#1209=EDGE_LOOP('',(#6645,#6646,#6647,#6648,#6649,#6650,#6651,#6652));
#1210=EDGE_LOOP('',(#6653,#6654,#6655,#6656));
#1211=EDGE_LOOP('',(#6657,#6658,#6659,#6660));
#1212=EDGE_LOOP('',(#6661,#6662,#6663,#6664));
#1213=EDGE_LOOP('',(#6665,#6666,#6667,#6668));
#1214=EDGE_LOOP('',(#6669,#6670,#6671,#6672));
#1215=EDGE_LOOP('',(#6673,#6674,#6675,#6676));
#1216=EDGE_LOOP('',(#6677,#6678,#6679,#6680));
#1217=EDGE_LOOP('',(#6681,#6682,#6683,#6684));
#1218=EDGE_LOOP('',(#6685,#6686,#6687,#6688));
#1219=EDGE_LOOP('',(#6689,#6690,#6691,#6692));
#1220=EDGE_LOOP('',(#6693,#6694,#6695,#6696));
#1221=EDGE_LOOP('',(#6697,#6698,#6699,#6700));
#1222=EDGE_LOOP('',(#6701,#6702,#6703,#6704));
#1223=EDGE_LOOP('',(#6705,#6706,#6707,#6708));
#1224=EDGE_LOOP('',(#6709,#6710,#6711,#6712));
#1225=EDGE_LOOP('',(#6713,#6714,#6715,#6716));
#1226=EDGE_LOOP('',(#6717,#6718,#6719,#6720));
#1227=EDGE_LOOP('',(#6721,#6722,#6723,#6724));
#1228=EDGE_LOOP('',(#6725,#6726,#6727,#6728));
#1229=EDGE_LOOP('',(#6729,#6730,#6731,#6732));
#1230=EDGE_LOOP('',(#6733,#6734,#6735,#6736));
#1231=EDGE_LOOP('',(#6737,#6738,#6739,#6740));
#1232=EDGE_LOOP('',(#6741,#6742,#6743,#6744));
#1233=EDGE_LOOP('',(#6745,#6746,#6747,#6748));
#1234=EDGE_LOOP('',(#6749,#6750,#6751,#6752));
#1235=EDGE_LOOP('',(#6753,#6754,#6755,#6756));
#1236=EDGE_LOOP('',(#6757,#6758,#6759,#6760));
#1237=EDGE_LOOP('',(#6761,#6762,#6763,#6764));
#1238=EDGE_LOOP('',(#6765,#6766,#6767,#6768));
#1239=EDGE_LOOP('',(#6769,#6770,#6771,#6772));
#1240=EDGE_LOOP('',(#6773,#6774,#6775,#6776,#6777,#6778,#6779,#6780));
#1241=EDGE_LOOP('',(#6781,#6782,#6783,#6784));
#1242=EDGE_LOOP('',(#6785,#6786,#6787,#6788));
#1243=EDGE_LOOP('',(#6789,#6790,#6791,#6792));
#1244=EDGE_LOOP('',(#6793,#6794,#6795,#6796));
#1245=EDGE_LOOP('',(#6797,#6798,#6799,#6800));
#1246=EDGE_LOOP('',(#6801,#6802,#6803,#6804));
#1247=EDGE_LOOP('',(#6805,#6806,#6807,#6808));
#1248=EDGE_LOOP('',(#6809,#6810,#6811,#6812));
#1249=EDGE_LOOP('',(#6813,#6814,#6815,#6816));
#1250=EDGE_LOOP('',(#6817,#6818,#6819,#6820));
#1251=EDGE_LOOP('',(#6821,#6822,#6823,#6824));
#1252=EDGE_LOOP('',(#6825,#6826,#6827,#6828));
#1253=EDGE_LOOP('',(#6829,#6830,#6831,#6832));
#1254=EDGE_LOOP('',(#6833,#6834,#6835,#6836));
#1255=EDGE_LOOP('',(#6837,#6838,#6839,#6840));
#1256=EDGE_LOOP('',(#6841,#6842,#6843,#6844));
#1257=EDGE_LOOP('',(#6845,#6846,#6847,#6848));
#1258=EDGE_LOOP('',(#6849,#6850,#6851,#6852));
#1259=EDGE_LOOP('',(#6853,#6854,#6855,#6856));
#1260=EDGE_LOOP('',(#6857,#6858,#6859,#6860));
#1261=EDGE_LOOP('',(#6861,#6862,#6863,#6864));
#1262=EDGE_LOOP('',(#6865,#6866,#6867,#6868));
#1263=EDGE_LOOP('',(#6869,#6870,#6871,#6872));
#1264=EDGE_LOOP('',(#6873,#6874,#6875,#6876));
#1265=EDGE_LOOP('',(#6877,#6878,#6879,#6880));
#1266=EDGE_LOOP('',(#6881,#6882,#6883,#6884));
#1267=EDGE_LOOP('',(#6885,#6886,#6887,#6888));
#1268=EDGE_LOOP('',(#6889,#6890,#6891,#6892));
#1269=EDGE_LOOP('',(#6893,#6894,#6895,#6896));
#1270=EDGE_LOOP('',(#6897,#6898,#6899,#6900));
#1271=EDGE_LOOP('',(#6901,#6902,#6903,#6904,#6905,#6906));
#1272=EDGE_LOOP('',(#6907,#6908,#6909,#6910));
#1273=EDGE_LOOP('',(#6911,#6912,#6913,#6914));
#1274=EDGE_LOOP('',(#6915,#6916,#6917,#6918));
#1275=EDGE_LOOP('',(#6919,#6920,#6921,#6922));
#1276=EDGE_LOOP('',(#6923,#6924,#6925,#6926));
#1277=EDGE_LOOP('',(#6927,#6928,#6929,#6930));
#1278=EDGE_LOOP('',(#6931,#6932,#6933,#6934));
#1279=EDGE_LOOP('',(#6935,#6936,#6937,#6938));
#1280=EDGE_LOOP('',(#6939,#6940,#6941,#6942));
#1281=EDGE_LOOP('',(#6943,#6944,#6945,#6946));
#1282=EDGE_LOOP('',(#6947,#6948,#6949,#6950));
#1283=EDGE_LOOP('',(#6951,#6952,#6953,#6954));
#1284=EDGE_LOOP('',(#6955,#6956,#6957,#6958));
#1285=EDGE_LOOP('',(#6959,#6960,#6961,#6962));
#1286=EDGE_LOOP('',(#6963,#6964,#6965,#6966,#6967,#6968));
#1287=EDGE_LOOP('',(#6969,#6970,#6971,#6972));
#1288=EDGE_LOOP('',(#6973,#6974,#6975,#6976));
#1289=EDGE_LOOP('',(#6977,#6978,#6979,#6980));
#1290=EDGE_LOOP('',(#6981,#6982,#6983,#6984));
#1291=EDGE_LOOP('',(#6985,#6986,#6987,#6988));
#1292=EDGE_LOOP('',(#6989,#6990,#6991,#6992));
#1293=EDGE_LOOP('',(#6993,#6994,#6995,#6996));
#1294=EDGE_LOOP('',(#6997,#6998,#6999,#7000));
#1295=EDGE_LOOP('',(#7001,#7002,#7003,#7004));
#1296=EDGE_LOOP('',(#7005,#7006,#7007,#7008));
#1297=EDGE_LOOP('',(#7009,#7010,#7011,#7012));
#1298=EDGE_LOOP('',(#7013,#7014,#7015,#7016));
#1299=EDGE_LOOP('',(#7017,#7018,#7019,#7020));
#1300=EDGE_LOOP('',(#7021,#7022,#7023,#7024));
#1301=EDGE_LOOP('',(#7025,#7026,#7027,#7028));
#1302=EDGE_LOOP('',(#7029,#7030,#7031,#7032));
#1303=EDGE_LOOP('',(#7033,#7034,#7035,#7036));
#1304=EDGE_LOOP('',(#7037,#7038,#7039,#7040));
#1305=EDGE_LOOP('',(#7041,#7042,#7043,#7044));
#1306=EDGE_LOOP('',(#7045,#7046,#7047,#7048));
#1307=EDGE_LOOP('',(#7049,#7050,#7051,#7052));
#1308=EDGE_LOOP('',(#7053,#7054,#7055,#7056));
#1309=EDGE_LOOP('',(#7057,#7058,#7059,#7060));
#1310=EDGE_LOOP('',(#7061,#7062,#7063,#7064));
#1311=EDGE_LOOP('',(#7065,#7066,#7067,#7068));
#1312=EDGE_LOOP('',(#7069,#7070,#7071,#7072));
#1313=EDGE_LOOP('',(#7073,#7074,#7075,#7076));
#1314=EDGE_LOOP('',(#7077,#7078,#7079,#7080));
#1315=EDGE_LOOP('',(#7081,#7082,#7083,#7084));
#1316=EDGE_LOOP('',(#7085,#7086,#7087,#7088));
#1317=EDGE_LOOP('',(#7089,#7090,#7091,#7092));
#1318=EDGE_LOOP('',(#7093,#7094,#7095,#7096));
#1319=EDGE_LOOP('',(#7097,#7098,#7099,#7100));
#1320=EDGE_LOOP('',(#7101,#7102,#7103,#7104));
#1321=EDGE_LOOP('',(#7105,#7106,#7107,#7108));
#1322=EDGE_LOOP('',(#7109,#7110,#7111,#7112));
#1323=EDGE_LOOP('',(#7113,#7114,#7115,#7116));
#1324=EDGE_LOOP('',(#7117,#7118,#7119,#7120));
#1325=EDGE_LOOP('',(#7121,#7122,#7123,#7124));
#1326=EDGE_LOOP('',(#7125,#7126,#7127,#7128));
#1327=EDGE_LOOP('',(#7129,#7130,#7131,#7132));
#1328=EDGE_LOOP('',(#7133,#7134,#7135,#7136));
#1329=EDGE_LOOP('',(#7137,#7138,#7139,#7140));
#1330=EDGE_LOOP('',(#7141,#7142,#7143,#7144));
#1331=EDGE_LOOP('',(#7145,#7146,#7147,#7148,#7149,#7150,#7151,#7152));
#1332=EDGE_LOOP('',(#7153,#7154,#7155,#7156));
#1333=EDGE_LOOP('',(#7157,#7158,#7159,#7160));
#1334=EDGE_LOOP('',(#7161,#7162,#7163,#7164));
#1335=EDGE_LOOP('',(#7165,#7166,#7167,#7168));
#1336=EDGE_LOOP('',(#7169,#7170,#7171,#7172));
#1337=EDGE_LOOP('',(#7173,#7174,#7175,#7176));
#1338=EDGE_LOOP('',(#7177,#7178,#7179,#7180));
#1339=EDGE_LOOP('',(#7181,#7182,#7183,#7184));
#1340=EDGE_LOOP('',(#7185,#7186,#7187,#7188));
#1341=EDGE_LOOP('',(#7189,#7190,#7191,#7192));
#1342=EDGE_LOOP('',(#7193,#7194,#7195,#7196));
#1343=EDGE_LOOP('',(#7197,#7198,#7199,#7200));
#1344=EDGE_LOOP('',(#7201,#7202,#7203,#7204));
#1345=EDGE_LOOP('',(#7205,#7206,#7207,#7208));
#1346=EDGE_LOOP('',(#7209,#7210,#7211,#7212));
#1347=EDGE_LOOP('',(#7213,#7214,#7215,#7216));
#1348=EDGE_LOOP('',(#7217,#7218,#7219,#7220));
#1349=EDGE_LOOP('',(#7221,#7222,#7223,#7224));
#1350=EDGE_LOOP('',(#7225,#7226,#7227,#7228));
#1351=EDGE_LOOP('',(#7229,#7230,#7231,#7232));
#1352=EDGE_LOOP('',(#7233,#7234,#7235,#7236));
#1353=EDGE_LOOP('',(#7237,#7238,#7239,#7240));
#1354=EDGE_LOOP('',(#7241,#7242,#7243,#7244));
#1355=EDGE_LOOP('',(#7245,#7246,#7247,#7248));
#1356=EDGE_LOOP('',(#7249,#7250,#7251,#7252));
#1357=EDGE_LOOP('',(#7253,#7254,#7255,#7256));
#1358=EDGE_LOOP('',(#7257,#7258,#7259,#7260));
#1359=EDGE_LOOP('',(#7261,#7262,#7263,#7264));
#1360=EDGE_LOOP('',(#7265,#7266,#7267,#7268));
#1361=EDGE_LOOP('',(#7269,#7270,#7271,#7272,#7273,#7274,#7275,#7276));
#1362=EDGE_LOOP('',(#7277,#7278,#7279,#7280));
#1363=EDGE_LOOP('',(#7281,#7282,#7283,#7284));
#1364=EDGE_LOOP('',(#7285,#7286,#7287,#7288));
#1365=EDGE_LOOP('',(#7289,#7290,#7291,#7292));
#1366=EDGE_LOOP('',(#7293,#7294,#7295,#7296));
#1367=EDGE_LOOP('',(#7297,#7298,#7299,#7300));
#1368=EDGE_LOOP('',(#7301,#7302,#7303,#7304));
#1369=EDGE_LOOP('',(#7305,#7306,#7307,#7308));
#1370=EDGE_LOOP('',(#7309,#7310,#7311,#7312));
#1371=EDGE_LOOP('',(#7313,#7314,#7315,#7316));
#1372=EDGE_LOOP('',(#7317,#7318,#7319,#7320));
#1373=EDGE_LOOP('',(#7321,#7322,#7323,#7324));
#1374=EDGE_LOOP('',(#7325,#7326,#7327,#7328));
#1375=EDGE_LOOP('',(#7329,#7330,#7331,#7332));
#1376=EDGE_LOOP('',(#7333,#7334,#7335,#7336));
#1377=EDGE_LOOP('',(#7337,#7338,#7339,#7340));
#1378=EDGE_LOOP('',(#7341,#7342,#7343,#7344));
#1379=EDGE_LOOP('',(#7345,#7346,#7347,#7348));
#1380=EDGE_LOOP('',(#7349,#7350,#7351,#7352));
#1381=EDGE_LOOP('',(#7353,#7354,#7355,#7356));
#1382=EDGE_LOOP('',(#7357,#7358,#7359,#7360));
#1383=EDGE_LOOP('',(#7361,#7362,#7363,#7364));
#1384=EDGE_LOOP('',(#7365,#7366,#7367,#7368));
#1385=EDGE_LOOP('',(#7369,#7370,#7371,#7372));
#1386=EDGE_LOOP('',(#7373,#7374,#7375,#7376));
#1387=EDGE_LOOP('',(#7377,#7378,#7379,#7380));
#1388=EDGE_LOOP('',(#7381,#7382,#7383,#7384));
#1389=EDGE_LOOP('',(#7385,#7386,#7387,#7388));
#1390=EDGE_LOOP('',(#7389,#7390,#7391,#7392));
#1391=EDGE_LOOP('',(#7393,#7394,#7395,#7396));
#1392=EDGE_LOOP('',(#7397,#7398,#7399,#7400));
#1393=EDGE_LOOP('',(#7401,#7402,#7403,#7404));
#1394=EDGE_LOOP('',(#7405,#7406,#7407,#7408));
#1395=EDGE_LOOP('',(#7409,#7410,#7411,#7412));
#1396=EDGE_LOOP('',(#7413,#7414,#7415,#7416));
#1397=EDGE_LOOP('',(#7417,#7418,#7419,#7420));
#1398=EDGE_LOOP('',(#7421,#7422,#7423,#7424));
#1399=EDGE_LOOP('',(#7425,#7426,#7427,#7428));
#1400=EDGE_LOOP('',(#7429,#7430,#7431,#7432));
#1401=EDGE_LOOP('',(#7433,#7434,#7435,#7436));
#1402=EDGE_LOOP('',(#7437,#7438,#7439,#7440));
#1403=EDGE_LOOP('',(#7441,#7442,#7443,#7444));
#1404=EDGE_LOOP('',(#7445,#7446,#7447,#7448));
#1405=EDGE_LOOP('',(#7449,#7450,#7451,#7452));
#1406=EDGE_LOOP('',(#7453,#7454,#7455,#7456));
#1407=EDGE_LOOP('',(#7457,#7458,#7459,#7460));
#1408=EDGE_LOOP('',(#7461,#7462,#7463,#7464,#7465,#7466,#7467,#7468,#7469,
#7470,#7471,#7472,#7473,#7474,#7475,#7476,#7477,#7478,#7479,#7480));
#1409=EDGE_LOOP('',(#7481,#7482,#7483,#7484,#7485,#7486,#7487,#7488,#7489,
#7490,#7491,#7492,#7493,#7494,#7495,#7496,#7497,#7498,#7499,#7500));
#1410=EDGE_LOOP('',(#7501));
#1411=EDGE_LOOP('',(#7502,#7503,#7504,#7505));
#1412=EDGE_LOOP('',(#7506,#7507,#7508,#7509));
#1413=EDGE_LOOP('',(#7510,#7511,#7512,#7513));
#1414=EDGE_LOOP('',(#7514,#7515,#7516,#7517));
#1415=EDGE_LOOP('',(#7518,#7519,#7520,#7521));
#1416=EDGE_LOOP('',(#7522,#7523,#7524,#7525));
#1417=EDGE_LOOP('',(#7526,#7527,#7528,#7529));
#1418=EDGE_LOOP('',(#7530,#7531,#7532,#7533));
#1419=EDGE_LOOP('',(#7534));
#1420=EDGE_LOOP('',(#7535,#7536,#7537,#7538,#7539));
#1421=EDGE_LOOP('',(#7540,#7541,#7542,#7543));
#1422=EDGE_LOOP('',(#7544,#7545,#7546,#7547,#7548,#7549,#7550,#7551,#7552,
#7553,#7554,#7555,#7556,#7557,#7558,#7559,#7560,#7561,#7562,#7563,#7564,
#7565,#7566,#7567,#7568,#7569,#7570,#7571,#7572,#7573,#7574,#7575,#7576,
#7577));
#1423=EDGE_LOOP('',(#7578,#7579,#7580,#7581,#7582,#7583,#7584,#7585,#7586,
#7587,#7588,#7589,#7590,#7591,#7592,#7593,#7594,#7595,#7596,#7597,#7598,
#7599,#7600,#7601,#7602,#7603,#7604,#7605,#7606,#7607,#7608,#7609,#7610,
#7611));
#1424=EDGE_LOOP('',(#7612,#7613,#7614,#7615));
#1425=EDGE_LOOP('',(#7616,#7617,#7618,#7619,#7620));
#1426=EDGE_LOOP('',(#7621,#7622,#7623,#7624));
#1427=EDGE_LOOP('',(#7625,#7626,#7627,#7628,#7629,#7630,#7631,#7632,#7633,
#7634,#7635,#7636,#7637,#7638,#7639,#7640,#7641,#7642,#7643,#7644,#7645,
#7646,#7647,#7648,#7649,#7650,#7651,#7652,#7653,#7654,#7655,#7656,#7657,
#7658));
#1428=EDGE_LOOP('',(#7659,#7660,#7661,#7662,#7663,#7664,#7665,#7666,#7667,
#7668,#7669,#7670,#7671,#7672,#7673,#7674,#7675,#7676,#7677,#7678,#7679,
#7680,#7681,#7682,#7683,#7684,#7685,#7686,#7687,#7688,#7689,#7690,#7691,
#7692));
#1429=EDGE_LOOP('',(#7693,#7694,#7695,#7696));
#1430=EDGE_LOOP('',(#7697,#7698,#7699));
#1431=EDGE_LOOP('',(#7700,#7701,#7702,#7703,#7704,#7705));
#1432=EDGE_LOOP('',(#7706,#7707,#7708));
#1433=EDGE_LOOP('',(#7709,#7710,#7711,#7712));
#1434=EDGE_LOOP('',(#7713,#7714,#7715,#7716,#7717,#7718,#7719,#7720,#7721,
#7722,#7723,#7724,#7725,#7726,#7727,#7728,#7729,#7730,#7731,#7732,#7733,
#7734,#7735,#7736,#7737,#7738,#7739,#7740,#7741,#7742,#7743,#7744,#7745,
#7746,#7747));
#1435=EDGE_LOOP('',(#7748,#7749,#7750,#7751,#7752,#7753,#7754,#7755,#7756,
#7757,#7758,#7759,#7760,#7761,#7762,#7763,#7764,#7765,#7766,#7767,#7768,
#7769,#7770,#7771,#7772,#7773,#7774,#7775,#7776,#7777,#7778,#7779,#7780,
#7781,#7782));
#1436=EDGE_LOOP('',(#7783,#7784,#7785));
#1437=EDGE_LOOP('',(#7786,#7787,#7788));
#1438=EDGE_LOOP('',(#7789,#7790,#7791,#7792,#7793,#7794));
#1439=EDGE_LOOP('',(#7795,#7796,#7797));
#1440=EDGE_LOOP('',(#7798,#7799,#7800,#7801));
#1441=EDGE_LOOP('',(#7802,#7803,#7804,#7805,#7806,#7807,#7808,#7809,#7810,
#7811,#7812,#7813,#7814,#7815,#7816,#7817,#7818,#7819,#7820,#7821,#7822,
#7823,#7824,#7825,#7826,#7827,#7828,#7829,#7830,#7831,#7832,#7833,#7834,
#7835,#7836));
#1442=EDGE_LOOP('',(#7837,#7838,#7839,#7840,#7841,#7842,#7843,#7844,#7845,
#7846,#7847,#7848,#7849,#7850,#7851,#7852,#7853,#7854,#7855,#7856,#7857,
#7858,#7859,#7860,#7861,#7862,#7863,#7864,#7865,#7866,#7867,#7868,#7869,
#7870,#7871));
#1443=EDGE_LOOP('',(#7872,#7873,#7874));
#1444=EDGE_LOOP('',(#7875,#7876,#7877,#7878));
#1445=EDGE_LOOP('',(#7879));
#1446=EDGE_LOOP('',(#7880));
#1447=EDGE_LOOP('',(#7881,#7882,#7883,#7884));
#1448=EDGE_LOOP('',(#7885,#7886,#7887,#7888));
#1449=EDGE_LOOP('',(#7889,#7890,#7891,#7892));
#1450=EDGE_LOOP('',(#7893,#7894,#7895,#7896,#7897,#7898,#7899,#7900,#7901,
#7902,#7903,#7904,#7905,#7906,#7907,#7908,#7909,#7910,#7911,#7912,#7913,
#7914,#7915,#7916,#7917,#7918,#7919,#7920,#7921,#7922,#7923,#7924,#7925,
#7926,#7927,#7928));
#1451=EDGE_LOOP('',(#7929,#7930,#7931,#7932,#7933,#7934,#7935,#7936,#7937,
#7938,#7939,#7940,#7941,#7942,#7943,#7944,#7945,#7946,#7947,#7948,#7949,
#7950,#7951,#7952,#7953,#7954,#7955,#7956,#7957,#7958,#7959,#7960,#7961,
#7962,#7963));
#1452=EDGE_LOOP('',(#7964,#7965,#7966,#7967));
#1453=EDGE_LOOP('',(#7968,#7969,#7970,#7971));
#1454=EDGE_LOOP('',(#7972,#7973,#7974,#7975));
#1455=EDGE_LOOP('',(#7976,#7977,#7978,#7979,#7980,#7981,#7982,#7983,#7984,
#7985,#7986,#7987,#7988,#7989,#7990,#7991,#7992,#7993,#7994,#7995,#7996,
#7997,#7998,#7999,#8000,#8001,#8002,#8003,#8004,#8005,#8006,#8007,#8008,
#8009,#8010,#8011));
#1456=EDGE_LOOP('',(#8012,#8013,#8014,#8015,#8016,#8017,#8018,#8019,#8020,
#8021,#8022,#8023,#8024,#8025,#8026,#8027,#8028,#8029,#8030,#8031,#8032,
#8033,#8034,#8035,#8036,#8037,#8038,#8039,#8040,#8041,#8042,#8043,#8044,
#8045,#8046));
#1457=EDGE_LOOP('',(#8047,#8048,#8049,#8050));
#1458=EDGE_LOOP('',(#8051,#8052,#8053,#8054));
#1459=EDGE_LOOP('',(#8055,#8056,#8057,#8058));
#1460=EDGE_LOOP('',(#8059,#8060,#8061,#8062,#8063,#8064,#8065,#8066,#8067,
#8068,#8069,#8070,#8071,#8072,#8073,#8074,#8075,#8076,#8077,#8078,#8079,
#8080,#8081,#8082,#8083,#8084,#8085,#8086,#8087,#8088,#8089,#8090,#8091,
#8092,#8093,#8094));
#1461=EDGE_LOOP('',(#8095,#8096,#8097,#8098,#8099,#8100,#8101,#8102,#8103,
#8104,#8105,#8106,#8107,#8108,#8109,#8110,#8111,#8112,#8113,#8114,#8115,
#8116,#8117,#8118,#8119,#8120,#8121,#8122,#8123,#8124,#8125,#8126,#8127,
#8128,#8129));
#1462=EDGE_LOOP('',(#8130,#8131,#8132,#8133));
#1463=EDGE_LOOP('',(#8134,#8135,#8136,#8137));
#1464=EDGE_LOOP('',(#8138,#8139,#8140,#8141));
#1465=EDGE_LOOP('',(#8142,#8143,#8144,#8145,#8146,#8147,#8148,#8149,#8150,
#8151,#8152,#8153,#8154,#8155,#8156,#8157,#8158,#8159,#8160,#8161,#8162,
#8163,#8164,#8165,#8166,#8167,#8168,#8169,#8170,#8171,#8172,#8173,#8174,
#8175,#8176,#8177));
#1466=EDGE_LOOP('',(#8178,#8179,#8180,#8181,#8182,#8183,#8184,#8185,#8186,
#8187,#8188,#8189,#8190,#8191,#8192,#8193,#8194,#8195,#8196,#8197,#8198,
#8199,#8200,#8201,#8202,#8203,#8204,#8205,#8206,#8207,#8208,#8209,#8210,
#8211,#8212));
#1467=EDGE_LOOP('',(#8213,#8214,#8215,#8216));
#1468=EDGE_LOOP('',(#8217));
#1469=EDGE_LOOP('',(#8218));
#1470=EDGE_LOOP('',(#8219));
#1471=EDGE_LOOP('',(#8220));
#1472=EDGE_LOOP('',(#8221,#8222,#8223,#8224));
#1473=EDGE_LOOP('',(#8225,#8226,#8227,#8228));
#1474=EDGE_LOOP('',(#8229,#8230,#8231,#8232));
#1475=EDGE_LOOP('',(#8233,#8234,#8235,#8236));
#1476=EDGE_LOOP('',(#8237,#8238,#8239,#8240));
#1477=EDGE_LOOP('',(#8241,#8242,#8243,#8244));
#1478=EDGE_LOOP('',(#8245,#8246,#8247,#8248));
#1479=EDGE_LOOP('',(#8249,#8250,#8251,#8252));
#1480=EDGE_LOOP('',(#8253,#8254,#8255,#8256,#8257,#8258,#8259,#8260,#8261,
#8262,#8263,#8264,#8265));
#1481=EDGE_LOOP('',(#8266,#8267,#8268,#8269));
#1482=EDGE_LOOP('',(#8270,#8271,#8272,#8273));
#1483=EDGE_LOOP('',(#8274,#8275,#8276,#8277));
#1484=EDGE_LOOP('',(#8278,#8279,#8280,#8281));
#1485=EDGE_LOOP('',(#8282,#8283,#8284,#8285));
#1486=EDGE_LOOP('',(#8286,#8287,#8288,#8289));
#1487=EDGE_LOOP('',(#8290,#8291,#8292,#8293));
#1488=EDGE_LOOP('',(#8294,#8295,#8296,#8297,#8298,#8299,#8300,#8301,#8302,
#8303,#8304,#8305,#8306));
#1489=EDGE_LOOP('',(#8307,#8308,#8309,#8310));
#1490=EDGE_LOOP('',(#8311,#8312,#8313,#8314));
#1491=EDGE_LOOP('',(#8315,#8316,#8317,#8318));
#1492=EDGE_LOOP('',(#8319));
#1493=EDGE_LOOP('',(#8320));
#1494=EDGE_LOOP('',(#8321));
#1495=EDGE_LOOP('',(#8322));
#1496=EDGE_LOOP('',(#8323));
#1497=EDGE_LOOP('',(#8324));
#1498=EDGE_LOOP('',(#8325));
#1499=EDGE_LOOP('',(#8326));
#1500=EDGE_LOOP('',(#8327));
#1501=EDGE_LOOP('',(#8328));
#1502=EDGE_LOOP('',(#8329));
#1503=EDGE_LOOP('',(#8330));
#1504=EDGE_LOOP('',(#8331));
#1505=EDGE_LOOP('',(#8332));
#1506=EDGE_LOOP('',(#8333));
#1507=EDGE_LOOP('',(#8334));
#1508=EDGE_LOOP('',(#8335));
#1509=EDGE_LOOP('',(#8336));
#1510=EDGE_LOOP('',(#8337,#8338,#8339,#8340));
#1511=EDGE_LOOP('',(#8341,#8342,#8343,#8344));
#1512=EDGE_LOOP('',(#8345,#8346,#8347,#8348));
#1513=EDGE_LOOP('',(#8349,#8350,#8351,#8352));
#1514=EDGE_LOOP('',(#8353,#8354,#8355,#8356));
#1515=EDGE_LOOP('',(#8357,#8358,#8359,#8360));
#1516=EDGE_LOOP('',(#8361));
#1517=EDGE_LOOP('',(#8362));
#1518=EDGE_LOOP('',(#8363));
#1519=EDGE_LOOP('',(#8364));
#1520=EDGE_LOOP('',(#8365));
#1521=EDGE_LOOP('',(#8366));
#1522=EDGE_LOOP('',(#8367));
#1523=EDGE_LOOP('',(#8368));
#1524=EDGE_LOOP('',(#8369));
#1525=EDGE_LOOP('',(#8370));
#1526=EDGE_LOOP('',(#8371));
#1527=EDGE_LOOP('',(#8372));
#1528=EDGE_LOOP('',(#8373));
#1529=EDGE_LOOP('',(#8374));
#1530=EDGE_LOOP('',(#8375));
#1531=EDGE_LOOP('',(#8376));
#1532=EDGE_LOOP('',(#8377));
#1533=EDGE_LOOP('',(#8378));
#1534=EDGE_LOOP('',(#8379,#8380,#8381,#8382));
#1535=EDGE_LOOP('',(#8383,#8384,#8385,#8386));
#1536=EDGE_LOOP('',(#8387,#8388,#8389,#8390));
#1537=EDGE_LOOP('',(#8391,#8392,#8393,#8394));
#1538=EDGE_LOOP('',(#8395,#8396,#8397,#8398));
#1539=EDGE_LOOP('',(#8399,#8400,#8401,#8402));
#1540=EDGE_LOOP('',(#8403,#8404,#8405,#8406));
#1541=EDGE_LOOP('',(#8407,#8408,#8409,#8410));
#1825=CIRCLE('',#10507,1.666);
#1826=CIRCLE('',#10508,1.666);
#1827=CIRCLE('',#10523,1.666);
#1828=CIRCLE('',#10525,2.05475000000001);
#1829=CIRCLE('',#10541,2.05475000000001);
#1830=CIRCLE('',#10543,1.666);
#1831=CIRCLE('',#10544,1.666);
#1832=CIRCLE('',#10559,1.666);
#1833=CIRCLE('',#10561,2.05475);
#1834=CIRCLE('',#10577,2.05475);
#1835=CIRCLE('',#10579,1.666);
#1836=CIRCLE('',#10580,1.666);
#1837=CIRCLE('',#10595,1.666);
#1838=CIRCLE('',#10597,2.05475000000001);
#1839=CIRCLE('',#10613,2.05475000000001);
#1840=CIRCLE('',#10615,1.666);
#1841=CIRCLE('',#10616,1.666);
#1842=CIRCLE('',#10631,1.666);
#1843=CIRCLE('',#10633,2.05475);
#1844=CIRCLE('',#10649,2.05475);
#1845=CIRCLE('',#10651,2.5175);
#1846=CIRCLE('',#10652,2.5175);
#1847=CIRCLE('',#10667,2.5175);
#1848=CIRCLE('',#10669,2.5175);
#1849=CIRCLE('',#10670,2.5175);
#1850=CIRCLE('',#10685,2.5175);
#1851=CIRCLE('',#10687,3.0735);
#1852=CIRCLE('',#10702,3.0735);
#1853=CIRCLE('',#10704,3.0735);
#1854=CIRCLE('',#10719,3.0735);
#1855=CIRCLE('',#10721,2.5175);
#1856=CIRCLE('',#10722,2.5175);
#1857=CIRCLE('',#10723,2.5175);
#1858=CIRCLE('',#10738,2.5175);
#1859=CIRCLE('',#10740,3.0735);
#1860=CIRCLE('',#10755,3.0735);
#1861=CIRCLE('',#10757,2.5175);
#1862=CIRCLE('',#10758,2.5175);
#1863=CIRCLE('',#10759,2.5175);
#1864=CIRCLE('',#10774,2.5175);
#1865=CIRCLE('',#10776,3.0735);
#1866=CIRCLE('',#10791,3.0735);
#1867=CIRCLE('',#10793,7.263);
#1868=CIRCLE('',#10801,7.263);
#1869=CIRCLE('',#10803,8.1015);
#1870=CIRCLE('',#10811,8.1015);
#1871=CIRCLE('',#10814,12.);
#1872=CIRCLE('',#10817,12.);
#1873=CIRCLE('',#10827,2.5175);
#1874=CIRCLE('',#10833,2.5175);
#1875=CIRCLE('',#10858,5.);
#1876=CIRCLE('',#10859,5.);
#1877=CIRCLE('',#10861,5.);
#1878=CIRCLE('',#10862,5.);
#1879=CIRCLE('',#10864,5.);
#1880=CIRCLE('',#10865,5.);
#1881=CIRCLE('',#10867,5.);
#1882=CIRCLE('',#10868,5.);
#1883=CIRCLE('',#10870,5.);
#1884=CIRCLE('',#10871,5.);
#1885=CIRCLE('',#10873,5.);
#1886=CIRCLE('',#10874,5.);
#1887=CIRCLE('',#10876,5.);
#1888=CIRCLE('',#10877,5.);
#1889=CIRCLE('',#10879,5.);
#1890=CIRCLE('',#10880,5.);
#1891=CIRCLE('',#10882,5.);
#1892=CIRCLE('',#10883,5.);
#1893=CIRCLE('',#10885,5.);
#1894=CIRCLE('',#10886,5.);
#1895=CIRCLE('',#10888,5.);
#1896=CIRCLE('',#10889,5.);
#1897=CIRCLE('',#10891,5.);
#1898=CIRCLE('',#10892,5.);
#1899=CIRCLE('',#10894,5.);
#1900=CIRCLE('',#10895,5.);
#1901=CIRCLE('',#10897,5.);
#1902=CIRCLE('',#10898,5.);
#1903=CIRCLE('',#10900,5.);
#1904=CIRCLE('',#10901,5.);
#1905=CIRCLE('',#10903,5.);
#1906=CIRCLE('',#10904,5.);
#1907=CIRCLE('',#10906,5.);
#1908=CIRCLE('',#10907,5.);
#1909=CIRCLE('',#10909,5.);
#1910=CIRCLE('',#10910,5.);
#2021=B_SPLINE_CURVE_WITH_KNOTS('',3,(#13455,#13456,#13457,#13458,#13459,
#13460,#13461,#13462,#13463,#13464,#13465,#13466,#13467,#13468,#13469,#13470,
#13471,#13472,#13473),.UNSPECIFIED.,.F.,.F.,(4,3,3,3,3,3,4),(95.5576018628658,
95.7627393059135,96.7602678403502,97.7577963747867,98.7553249092233,99.75285344366,
100.750381978097),.UNSPECIFIED.);
#2022=B_SPLINE_CURVE_WITH_KNOTS('',3,(#13477,#13478,#13479,#13480),
 .UNSPECIFIED.,.F.,.F.,(4,4),(-98.735769112822,-98.0941628713862),
 .UNSPECIFIED.);
#2023=B_SPLINE_CURVE_WITH_KNOTS('',3,(#13484,#13485,#13486,#13487,#13488,
#13489,#13490,#13491,#13492,#13493,#13494,#13495,#13496,#13497,#13498,#13499,
#13500,#13501,#13502,#13503,#13504,#13505),.UNSPECIFIED.,.F.,.F.,(4,3,3,
3,3,3,3,4),(-98.0941628713862,-97.7577963747868,-96.7602678403502,-95.7627393059136,
-94.765210771477,-93.7676822370404,-92.7701537026038,-91.8109775642066),
 .UNSPECIFIED.);
#2024=B_SPLINE_CURVE_WITH_KNOTS('',3,(#13510,#13511,#13512,#13513,#13514,
#13515,#13516,#13517,#13518,#13519,#13520,#13521,#13522,#13523,#13524,#13525,
#13526,#13527,#13528,#13529,#13530,#13531),.UNSPECIFIED.,.F.,.F.,(4,3,3,
3,3,3,3,4),(89.2744165556862,89.777568099294,90.7750966337306,91.7726251681672,
92.7701537026037,93.7676822370404,94.7652107714769,95.5576018628658),
 .UNSPECIFIED.);
#2025=B_SPLINE_CURVE_WITH_KNOTS('',3,(#13532,#13533,#13534,#13535,#13536,
#13537,#13538,#13539,#13540,#13541,#13542,#13543,#13544,#13545,#13546,#13547,
#13548,#13549,#13550,#13551,#13552,#13553,#13554,#13555,#13556),
 .UNSPECIFIED.,.F.,.F.,(4,3,3,3,3,3,3,3,4),(-91.8109775642066,-91.7726251681672,
-90.7750966337306,-89.777568099294,-88.7800395648574,-87.7825110304208,
-86.7849824959842,-85.7874539615476,-85.527792257027),.UNSPECIFIED.);
#2026=B_SPLINE_CURVE_WITH_KNOTS('',3,(#13561,#13562,#13563,#13564,#13565,
#13566,#13567,#13568,#13569,#13570,#13571,#13572,#13573,#13574,#13575,#13576,
#13577,#13578,#13579,#13580,#13581,#13582),.UNSPECIFIED.,.F.,.F.,(4,3,3,
3,3,3,3,4),(82.9912312485066,83.7923968926744,84.789925427111,85.7874539615476,
86.7849824959842,87.7825110304208,88.7800395648573,89.2744165556862),
 .UNSPECIFIED.);
#2027=B_SPLINE_CURVE_WITH_KNOTS('',3,(#13583,#13584,#13585,#13586,#13587,
#13588,#13589,#13590,#13591,#13592,#13593,#13594,#13595,#13596,#13597,#13598,
#13599,#13600,#13601,#13602,#13603,#13604),.UNSPECIFIED.,.F.,.F.,(4,3,3,
3,3,3,3,4),(-85.527792257027,-84.789925427111,-83.7923968926744,-82.7948683582378,
-81.7973398238012,-80.7998112893646,-79.802282754928,-79.2446069498474),
 .UNSPECIFIED.);
#2028=B_SPLINE_CURVE_WITH_KNOTS('',3,(#13609,#13610,#13611,#13612,#13613,
#13614,#13615,#13616,#13617,#13618,#13619,#13620,#13621,#13622,#13623,#13624,
#13625,#13626,#13627,#13628,#13629,#13630,#13631,#13632,#13633),
 .UNSPECIFIED.,.F.,.F.,(4,3,3,3,3,3,3,3,4),(76.7080459413271,76.8096971516182,
77.8072256860548,78.8047542204914,79.802282754928,80.7998112893646,81.7973398238012,
82.7948683582378,82.9912312485066),.UNSPECIFIED.);
#2029=B_SPLINE_CURVE_WITH_KNOTS('',3,(#13634,#13635,#13636,#13637,#13638,
#13639,#13640,#13641,#13642,#13643,#13644,#13645,#13646,#13647,#13648,#13649,
#13650,#13651,#13652,#13653,#13654,#13655),.UNSPECIFIED.,.F.,.F.,(4,3,3,
3,3,3,3,4),(-79.2446069498474,-78.8047542204914,-77.8072256860548,-76.8096971516182,
-75.8121686171816,-74.814640082745,-73.8171115483084,-72.9614216426678),
 .UNSPECIFIED.);
#2030=B_SPLINE_CURVE_WITH_KNOTS('',3,(#13660,#13661,#13662,#13663,#13664,
#13665,#13666,#13667,#13668,#13669,#13670,#13671,#13672,#13673,#13674,#13675,
#13676,#13677,#13678,#13679,#13680,#13681),.UNSPECIFIED.,.F.,.F.,(4,3,3,
3,3,3,3,4),(70.4248606341475,70.8245259449986,71.8220544794352,72.8195830138718,
73.8171115483084,74.814640082745,75.8121686171816,76.7080459413271),
 .UNSPECIFIED.);
#2031=B_SPLINE_CURVE_WITH_KNOTS('',3,(#13682,#13683,#13684,#13685,#13686,
#13687,#13688,#13689,#13690,#13691,#13692,#13693,#13694,#13695,#13696,#13697,
#13698,#13699,#13700,#13701,#13702,#13703,#13704,#13705,#13706),
 .UNSPECIFIED.,.F.,.F.,(4,3,3,3,3,3,3,3,4),(-72.9614216426678,-72.8195830138718,
-71.8220544794352,-70.8245259449986,-69.826997410562,-68.8294688761254,
-67.8319403416888,-66.8344118072522,-66.6782363354882),.UNSPECIFIED.);
#2032=B_SPLINE_CURVE_WITH_KNOTS('',3,(#13711,#13712,#13713,#13714,#13715,
#13716,#13717,#13718,#13719,#13720,#13721,#13722,#13723,#13724,#13725,#13726,
#13727,#13728,#13729,#13730,#13731,#13732),.UNSPECIFIED.,.F.,.F.,(4,3,3,
3,3,3,3,4),(64.1416753269678,64.839354738379,65.8368832728156,66.8344118072522,
67.8319403416888,68.8294688761254,69.826997410562,70.4248606341475),
 .UNSPECIFIED.);
#2033=B_SPLINE_CURVE_WITH_KNOTS('',3,(#13733,#13734,#13735,#13736,#13737,
#13738,#13739,#13740,#13741,#13742,#13743,#13744,#13745,#13746,#13747,#13748,
#13749,#13750,#13751,#13752,#13753,#13754),.UNSPECIFIED.,.F.,.F.,(4,3,3,
3,3,3,3,4),(-66.6782363354882,-65.8368832728156,-64.839354738379,-63.8418262039424,
-62.8442976695058,-61.8467691350692,-60.8492406006326,-60.3950510283086),
 .UNSPECIFIED.);
#2034=B_SPLINE_CURVE_WITH_KNOTS('',3,(#13759,#13760,#13761,#13762,#13763,
#13764,#13765,#13766,#13767,#13768,#13769,#13770,#13771,#13772,#13773,#13774,
#13775,#13776,#13777,#13778,#13779,#13780),.UNSPECIFIED.,.F.,.F.,(4,3,3,
3,3,3,3,4),(57.8584900197883,58.8541835317594,59.851712066196,60.8492406006326,
61.8467691350692,62.8442976695058,63.8418262039424,64.1416753269678),
 .UNSPECIFIED.);
#2035=B_SPLINE_CURVE_WITH_KNOTS('',3,(#13781,#13782,#13783,#13784,#13785,
#13786,#13787,#13788,#13789,#13790,#13791,#13792,#13793,#13794,#13795,#13796,
#13797,#13798,#13799,#13800,#13801,#13802),.UNSPECIFIED.,.F.,.F.,(4,3,3,
3,3,3,3,4),(-60.3950510283086,-59.851712066196,-58.8541835317594,-57.8566549973228,
-56.8591264628862,-55.8615979284496,-54.864069394013,-54.111865721129),
 .UNSPECIFIED.);
#2036=B_SPLINE_CURVE_WITH_KNOTS('',3,(#13807,#13808,#13809,#13810,#13811,
#13812,#13813,#13814,#13815,#13816,#13817,#13818,#13819,#13820,#13821,#13822,
#13823,#13824,#13825,#13826,#13827,#13828),.UNSPECIFIED.,.F.,.F.,(4,3,3,
3,3,3,3,4),(51.5753047126087,51.8714837907032,52.8690123251398,53.8665408595764,
54.864069394013,55.8615979284496,56.8591264628862,57.8584900197883),
 .UNSPECIFIED.);
#2037=B_SPLINE_CURVE_WITH_KNOTS('',3,(#13829,#13830,#13831,#13832,#13833,
#13834,#13835,#13836,#13837,#13838,#13839,#13840,#13841,#13842,#13843,#13844,
#13845,#13846,#13847,#13848,#13849,#13850,#13851,#13852,#13853),
 .UNSPECIFIED.,.F.,.F.,(4,3,3,3,3,3,3,3,4),(-54.111865721129,-53.8665408595764,
-52.8690123251398,-51.8714837907032,-50.8739552562666,-49.87642672183,-48.8788981873934,
-47.8813696529568,-47.8286804139494),.UNSPECIFIED.);
#2038=B_SPLINE_CURVE_WITH_KNOTS('',3,(#13858,#13859,#13860,#13861,#13862,
#13863,#13864,#13865,#13866,#13867,#13868,#13869,#13870,#13871,#13872,#13873,
#13874,#13875,#13876,#13877,#13878,#13879),.UNSPECIFIED.,.F.,.F.,(4,3,3,
3,3,3,3,4),(45.2921194054291,45.8863125840836,46.8838411185202,47.8813696529568,
48.8788981873934,49.87642672183,50.8739552562666,51.5753047126087),
 .UNSPECIFIED.);
#2039=B_SPLINE_CURVE_WITH_KNOTS('',3,(#13880,#13881,#13882,#13883,#13884,
#13885,#13886,#13887,#13888,#13889,#13890,#13891,#13892,#13893,#13894,#13895,
#13896,#13897,#13898,#13899,#13900,#13901),.UNSPECIFIED.,.F.,.F.,(4,3,3,
3,3,3,3,4),(-47.8286804139494,-46.8838411185202,-45.8863125840836,-44.888784049647,
-43.8912555152104,-42.8937269807738,-41.8961984463372,-41.5454951067698),
 .UNSPECIFIED.);
#2040=B_SPLINE_CURVE_WITH_KNOTS('',3,(#13906,#13907,#13908,#13909,#13910,
#13911,#13912,#13913,#13914,#13915,#13916,#13917,#13918,#13919,#13920,#13921,
#13922,#13923,#13924,#13925,#13926,#13927),.UNSPECIFIED.,.F.,.F.,(4,3,3,
3,3,3,3,4),(39.0089340982495,39.901141377464,40.8986699119006,41.8961984463372,
42.8937269807738,43.8912555152104,44.888784049647,45.2921194054291),
 .UNSPECIFIED.);
#2041=B_SPLINE_CURVE_WITH_KNOTS('',3,(#13928,#13929,#13930,#13931,#13932,
#13933,#13934,#13935,#13936,#13937,#13938,#13939,#13940,#13941,#13942,#13943,
#13944,#13945,#13946,#13947,#13948,#13949),.UNSPECIFIED.,.F.,.F.,(4,3,3,
3,3,3,3,4),(-41.5454951067698,-40.8986699119006,-39.901141377464,-38.9036128430274,
-37.9060843085908,-36.9085557741542,-35.9110272397176,-35.2623097995902),
 .UNSPECIFIED.);
#2042=B_SPLINE_CURVE_WITH_KNOTS('',3,(#13954,#13955,#13956,#13957,#13958,
#13959,#13960,#13961,#13962,#13963,#13964,#13965,#13966,#13967,#13968,#13969,
#13970,#13971,#13972,#13973,#13974,#13975,#13976,#13977,#13978),
 .UNSPECIFIED.,.F.,.F.,(4,3,3,3,3,3,3,3,4),(32.7257487910699,32.9184416364078,
33.9159701708444,34.913498705281,35.9110272397176,36.9085557741542,37.9060843085908,
38.9036128430274,39.0089340982495),.UNSPECIFIED.);
#2043=B_SPLINE_CURVE_WITH_KNOTS('',3,(#13979,#13980,#13981,#13982,#13983,
#13984,#13985,#13986,#13987,#13988,#13989,#13990,#13991,#13992,#13993,#13994,
#13995,#13996,#13997,#13998,#13999,#14000),.UNSPECIFIED.,.F.,.F.,(4,3,3,
3,3,3,3,4),(-35.2623097995902,-34.913498705281,-33.9159701708444,-32.9184416364078,
-31.9209131019712,-30.9233845675346,-29.925856033098,-28.9791244924106),
 .UNSPECIFIED.);
#2044=B_SPLINE_CURVE_WITH_KNOTS('',3,(#14005,#14006,#14007,#14008,#14009,
#14010,#14011,#14012,#14013,#14014,#14015,#14016,#14017,#14018,#14019,#14020,
#14021,#14022,#14023,#14024,#14025,#14026),.UNSPECIFIED.,.F.,.F.,(4,3,3,
3,3,3,3,4),(26.4425634838903,26.9332704297882,27.9307989642248,28.9283274986614,
29.925856033098,30.9233845675346,31.9209131019712,32.7257487910699),
 .UNSPECIFIED.);
#2045=B_SPLINE_CURVE_WITH_KNOTS('',3,(#14027,#14028,#14029,#14030,#14031,
#14032,#14033,#14034,#14035,#14036,#14037,#14038,#14039,#14040,#14041,#14042,
#14043,#14044,#14045,#14046,#14047,#14048,#14049,#14050,#14051),
 .UNSPECIFIED.,.F.,.F.,(4,3,3,3,3,3,3,3,4),(-28.9791244924106,-28.9283274986614,
-27.9307989642248,-26.9332704297882,-25.9357418953516,-24.938213360915,
-23.9406848264784,-22.9431562920418,-22.6959391852311),.UNSPECIFIED.);
#2046=B_SPLINE_CURVE_WITH_KNOTS('',3,(#14056,#14057,#14058,#14059,#14060,
#14061,#14062,#14063,#14064,#14065,#14066,#14067,#14068,#14069,#14070,#14071,
#14072,#14073,#14074,#14075,#14076,#14077),.UNSPECIFIED.,.F.,.F.,(4,3,3,
3,3,3,3,4),(20.1593781767107,20.9480992231686,21.9456277576052,22.9431562920418,
23.9406848264784,24.938213360915,25.9357418953516,26.4425634838903),
 .UNSPECIFIED.);
#2047=B_SPLINE_CURVE_WITH_KNOTS('',3,(#14078,#14079,#14080,#14081,#14082,
#14083,#14084,#14085,#14086,#14087,#14088,#14089,#14090,#14091,#14092,#14093,
#14094,#14095,#14096,#14097,#14098,#14099),.UNSPECIFIED.,.F.,.F.,(4,3,3,
3,3,3,3,4),(-22.6959391852311,-21.9456277576052,-20.9480992231686,-19.950570688732,
-18.9530421542954,-17.9555136198588,-16.9579850854222,-16.4127538780515),
 .UNSPECIFIED.);
#2048=B_SPLINE_CURVE_WITH_KNOTS('',3,(#14104,#14105,#14106,#14107,#14108,
#14109,#14110,#14111,#14112,#14113,#14114,#14115,#14116,#14117,#14118,#14119,
#14120,#14121,#14122,#14123,#14124,#14125,#14126,#14127,#14128),
 .UNSPECIFIED.,.F.,.F.,(4,3,3,3,3,3,3,3,4),(13.8761928695311,13.9653994821124,
14.962928016549,15.9604565509856,16.9579850854222,17.9555136198588,18.9530421542954,
19.950570688732,20.1593781767107),.UNSPECIFIED.);
#2049=B_SPLINE_CURVE_WITH_KNOTS('',3,(#14129,#14130,#14131,#14132,#14133,
#14134,#14135,#14136,#14137,#14138,#14139,#14140,#14141,#14142,#14143,#14144,
#14145,#14146,#14147,#14148,#14149,#14150),.UNSPECIFIED.,.F.,.F.,(4,3,3,
3,3,3,3,4),(-16.4127538780515,-15.9604565509856,-14.962928016549,-13.9653994821124,
-12.9678709476758,-11.9703424132392,-10.9728138788026,-10.1295685708719),
 .UNSPECIFIED.);
#2050=B_SPLINE_CURVE_WITH_KNOTS('',3,(#14156,#14157,#14158,#14159,#14160,
#14161,#14162,#14163,#14164,#14165,#14166,#14167,#14168),.UNSPECIFIED.,
 .F.,.F.,(4,3,3,3,4),(-3.8463832636923,-2.9925856033098,-1.9950570688732,
-0.997528534436598,0.),.UNSPECIFIED.);
#2051=B_SPLINE_CURVE_WITH_KNOTS('',3,(#14171,#14172,#14173,#14174,#14175,
#14176,#14177,#14178,#14179,#14180,#14181,#14182,#14183,#14184,#14185,#14186,
#14187,#14188,#14189),.UNSPECIFIED.,.F.,.F.,(4,3,3,3,3,3,4),(2.01461286527445,
2.9925856033098,3.9901141377464,4.987642672183,5.9851712066196,6.9826997410562,
7.59300756235153),.UNSPECIFIED.);
#2052=B_SPLINE_CURVE_WITH_KNOTS('',3,(#14195,#14196,#14197,#14198,#14199,
#14200),.UNSPECIFIED.,.F.,.F.,(4,1,1,4),(109.955742875643,110.61690491348,
111.614433447917,112.611961982353),.UNSPECIFIED.);
#2053=B_SPLINE_CURVE_WITH_KNOTS('',3,(#14203,#14204,#14205,#14206,#14207,
#14208,#14209),.UNSPECIFIED.,.F.,.F.,(4,1,1,1,4),(109.955742875643,110.16088031869,
111.158408853127,112.155937387564,113.133910125599),.UNSPECIFIED.);
#2054=B_SPLINE_CURVE_WITH_KNOTS('',3,(#14214,#14215,#14216,#14217,#14218,
#14219,#14220,#14221,#14222,#14223),.UNSPECIFIED.,.F.,.F.,(4,1,1,1,1,1,
1,4),(103.672557568463,104.63173370686,105.629262241297,106.626790775734,
107.62431931017,108.621847844607,109.619376379043,109.955742875643),
 .UNSPECIFIED.);
#2055=B_SPLINE_CURVE_WITH_KNOTS('',3,(#14224,#14225,#14226,#14227,#14228,
#14229,#14230,#14231,#14232,#14233),.UNSPECIFIED.,.F.,.F.,(4,1,1,1,1,1,
1,4),(103.672557568463,104.175709112071,105.173237646507,106.170766180944,
107.168294715381,108.165823249817,109.163351784254,109.955742875643),
 .UNSPECIFIED.);
#2056=B_SPLINE_CURVE_WITH_KNOTS('',3,(#14238,#14239,#14240,#14241,#14242,
#14243,#14244,#14245,#14246,#14247,#14248),.UNSPECIFIED.,.F.,.F.,(4,1,1,
1,1,1,1,1,4),(97.3893722612836,97.6490339658042,98.6465625002408,99.6440910346774,
100.641619569114,101.639148103551,102.636676637987,103.634205172424,103.672557568463),
 .UNSPECIFIED.);
#2057=B_SPLINE_CURVE_WITH_KNOTS('',3,(#14249,#14250,#14251,#14252,#14253,
#14254,#14255,#14256,#14257,#14258),.UNSPECIFIED.,.F.,.F.,(4,1,1,1,1,1,
1,4),(97.3893722612836,98.1905379054512,99.1880664398878,100.185594974324,
101.183123508761,102.180652043198,103.178180577634,103.672557568463),
 .UNSPECIFIED.);
#2058=B_SPLINE_CURVE_WITH_KNOTS('',3,(#14263,#14264,#14265,#14266,#14267,
#14268,#14269,#14270,#14271,#14272),.UNSPECIFIED.,.F.,.F.,(4,1,1,1,1,1,
1,4),(91.106186954104,91.6638627591846,92.6613912936212,93.6589198280578,
94.6564483624944,95.653976896931,96.6515054313676,97.3893722612836),
 .UNSPECIFIED.);
#2059=B_SPLINE_CURVE_WITH_KNOTS('',3,(#14273,#14274,#14275,#14276,#14277,
#14278,#14279,#14280,#14281,#14282,#14283),.UNSPECIFIED.,.F.,.F.,(4,1,1,
1,1,1,1,1,4),(91.106186954104,91.207838164395,92.2053666988316,93.2028952332682,
94.2004237677048,95.1979523021414,96.195480836578,97.1930093710146,97.3893722612836),
 .UNSPECIFIED.);
#2060=B_SPLINE_CURVE_WITH_KNOTS('',3,(#14288,#14289,#14290,#14291,#14292,
#14293,#14294,#14295,#14296,#14297),.UNSPECIFIED.,.F.,.F.,(4,1,1,1,1,1,
1,4),(84.8230016469244,85.678691552565,86.6762200870016,87.6737486214382,
88.6712771558748,89.6688056903114,90.666334224748,91.106186954104),
 .UNSPECIFIED.);
#2061=B_SPLINE_CURVE_WITH_KNOTS('',3,(#14298,#14299,#14300,#14301,#14302,
#14303,#14304,#14305,#14306,#14307),.UNSPECIFIED.,.F.,.F.,(4,1,1,1,1,1,
1,4),(84.8230016469244,85.2226669577754,86.220195492212,87.2177240266486,
88.2152525610852,89.2127810955218,90.2103096299584,91.106186954104),
 .UNSPECIFIED.);
#2062=B_SPLINE_CURVE_WITH_KNOTS('',3,(#14312,#14313,#14314,#14315,#14316,
#14317,#14318,#14319,#14320,#14321,#14322),.UNSPECIFIED.,.F.,.F.,(4,1,1,
1,1,1,1,1,4),(78.5398163397448,78.6959918115088,79.6935203459454,80.691048880382,
81.6885774148186,82.6861059492552,83.6836344836918,84.6811630181284,84.8230016469244),
 .UNSPECIFIED.);
#2063=B_SPLINE_CURVE_WITH_KNOTS('',3,(#14323,#14324,#14325,#14326,#14327,
#14328,#14329,#14330,#14331,#14332),.UNSPECIFIED.,.F.,.F.,(4,1,1,1,1,1,
1,4),(78.5398163397448,79.2374957511558,80.2350242855924,81.232552820029,
82.2300813544656,83.2276098889022,84.2251384233388,84.8230016469244),
 .UNSPECIFIED.);
#2064=B_SPLINE_CURVE_WITH_KNOTS('',3,(#14337,#14338,#14339,#14340,#14341,
#14342,#14343,#14344,#14345,#14346),.UNSPECIFIED.,.F.,.F.,(4,1,1,1,1,1,
1,4),(72.2566310325652,72.7108206048892,73.7083491393258,74.7058776737624,
75.703406208199,76.7009347426356,77.6984632770722,78.5398163397448),
 .UNSPECIFIED.);
#2065=B_SPLINE_CURVE_WITH_KNOTS('',3,(#14347,#14348,#14349,#14350,#14351,
#14352,#14353,#14354,#14355,#14356),.UNSPECIFIED.,.F.,.F.,(4,1,1,1,1,1,
1,4),(72.2566310325652,73.2523245445362,74.2498530789728,75.2473816134094,
76.244910147846,77.2424386822826,78.2399672167192,78.5398163397448),
 .UNSPECIFIED.);
#2066=B_SPLINE_CURVE_WITH_KNOTS('',3,(#14361,#14362,#14363,#14364,#14365,
#14366,#14367,#14368,#14369,#14370),.UNSPECIFIED.,.F.,.F.,(4,1,1,1,1,1,
1,4),(65.9734457253856,66.7256493982696,67.7231779327062,68.7207064671428,
69.7182350015794,70.715763536016,71.7132920704526,72.2566310325652),
 .UNSPECIFIED.);
#2067=B_SPLINE_CURVE_WITH_KNOTS('',3,(#14371,#14372,#14373,#14374,#14375,
#14376,#14377,#14378,#14379,#14380,#14381),.UNSPECIFIED.,.F.,.F.,(4,1,1,
1,1,1,1,1,4),(65.9734457253856,66.26962480348,67.2671533379166,68.2646818723533,
69.2622104067898,70.2597389412264,71.257267475663,72.2547960100996,72.2566310325652),
 .UNSPECIFIED.);
#2068=B_SPLINE_CURVE_WITH_KNOTS('',3,(#14386,#14387,#14388,#14389,#14390,
#14391,#14392,#14393,#14394,#14395,#14396),.UNSPECIFIED.,.F.,.F.,(4,1,1,
1,1,1,1,1,4),(59.690260418206,59.7429496572134,60.74047819165,61.7380067260866,
62.7355352605232,63.7330637949598,64.7305923293964,65.728120863833,65.9734457253856),
 .UNSPECIFIED.);
#2069=B_SPLINE_CURVE_WITH_KNOTS('',3,(#14397,#14398,#14399,#14400,#14401,
#14402,#14403,#14404,#14405,#14406),.UNSPECIFIED.,.F.,.F.,(4,1,1,1,1,1,
1,4),(59.690260418206,60.2844535968604,61.281982131297,62.2795106657336,
63.2770392001703,64.2745677346068,65.2720962690434,65.9734457253856),
 .UNSPECIFIED.);
#2070=B_SPLINE_CURVE_WITH_KNOTS('',3,(#14411,#14412,#14413,#14414,#14415,
#14416,#14417,#14418,#14419,#14420),.UNSPECIFIED.,.F.,.F.,(4,1,1,1,1,1,
1,4),(53.4070751110264,53.7577784505938,54.7553069850304,55.752835519467,
56.7503640539036,57.7478925883402,58.7454211227768,59.690260418206),
 .UNSPECIFIED.);
#2071=B_SPLINE_CURVE_WITH_KNOTS('',3,(#14421,#14422,#14423,#14424,#14425,
#14426,#14427,#14428,#14429,#14430),.UNSPECIFIED.,.F.,.F.,(4,1,1,1,1,1,
1,4),(53.4070751110264,54.2992823902408,55.2968109246774,56.294339459114,
57.2918679935507,58.2893965279873,59.2869250624238,59.690260418206),
 .UNSPECIFIED.);
#2072=B_SPLINE_CURVE_WITH_KNOTS('',3,(#14435,#14436,#14437,#14438,#14439,
#14440,#14441,#14442,#14443,#14444),.UNSPECIFIED.,.F.,.F.,(4,1,1,1,1,1,
1,4),(47.1238898038469,47.7726072439742,48.7701357784108,49.7676643128474,
50.765192847284,51.7627213817206,52.7602499161572,53.4070751110264),
 .UNSPECIFIED.);
#2073=B_SPLINE_CURVE_WITH_KNOTS('',3,(#14445,#14446,#14447,#14448,#14449,
#14450,#14451,#14452,#14453,#14454,#14455),.UNSPECIFIED.,.F.,.F.,(4,1,1,
1,1,1,1,1,4),(47.1238898038469,47.3165826491847,48.3141111836213,49.3116397180578,
50.3091682524944,51.3066967869311,52.3042253213677,53.3017538558043,53.4070751110264),
 .UNSPECIFIED.);
#2074=B_SPLINE_CURVE_WITH_KNOTS('',3,(#14460,#14461,#14462,#14463,#14464,
#14465,#14466,#14467,#14468,#14469),.UNSPECIFIED.,.F.,.F.,(4,1,1,1,1,1,
1,4),(40.8407044966673,41.7874360373546,42.7849645717912,43.7824931062278,
44.7800216406644,45.777550175101,46.7750787095376,47.1238898038469),
 .UNSPECIFIED.);
#2075=B_SPLINE_CURVE_WITH_KNOTS('',3,(#14470,#14471,#14472,#14473,#14474,
#14475,#14476,#14477,#14478,#14479),.UNSPECIFIED.,.F.,.F.,(4,1,1,1,1,1,
1,4),(40.8407044966673,41.3314114425651,42.3289399770017,43.3264685114383,
44.3239970458749,45.3215255803115,46.3190541147481,47.1238898038469),
 .UNSPECIFIED.);
#2076=B_SPLINE_CURVE_WITH_KNOTS('',3,(#14484,#14485,#14486,#14487,#14488,
#14489,#14490,#14491,#14492,#14493,#14494),.UNSPECIFIED.,.F.,.F.,(4,1,1,
1,1,1,1,1,4),(34.5575191894876,34.8047362962984,35.802264830735,36.7997933651716,
37.7973218996082,38.7948504340448,39.7923789684814,40.789907502918,40.8407044966673),
 .UNSPECIFIED.);
#2077=B_SPLINE_CURVE_WITH_KNOTS('',3,(#14495,#14496,#14497,#14498,#14499,
#14500,#14501,#14502,#14503,#14504),.UNSPECIFIED.,.F.,.F.,(4,1,1,1,1,1,
1,4),(34.5575191894876,35.3462402359455,36.3437687703821,37.3412973048187,
38.3388258392553,39.3363543736919,40.3338829081285,40.8407044966673),
 .UNSPECIFIED.);
#2078=B_SPLINE_CURVE_WITH_KNOTS('',3,(#14509,#14510,#14511,#14512,#14513,
#14514,#14515,#14516,#14517,#14518),.UNSPECIFIED.,.F.,.F.,(4,1,1,1,1,1,
1,4),(28.2743338823081,28.8195650896788,29.8170936241154,30.814622158552,
31.8121506929886,32.8096792274252,33.8072077618618,34.5575191894876),
 .UNSPECIFIED.);
#2079=B_SPLINE_CURVE_WITH_KNOTS('',3,(#14519,#14520,#14521,#14522,#14523,
#14524,#14525,#14526,#14527,#14528,#14529),.UNSPECIFIED.,.F.,.F.,(4,1,1,
1,1,1,1,1,4),(28.2743338823081,28.3635404948893,29.3610690293259,30.3585975637625,
31.3561260981991,32.3536546326357,33.3511831670723,34.3487117015089,34.5575191894876),
 .UNSPECIFIED.);
#2080=B_SPLINE_CURVE_WITH_KNOTS('',3,(#14534,#14535,#14536,#14537,#14538,
#14539,#14540,#14541,#14542,#14543),.UNSPECIFIED.,.F.,.F.,(4,1,1,1,1,1,
1,4),(21.9911485751285,22.8343938830592,23.8319224174958,24.8294509519324,
25.826979486369,26.8245080208056,27.8220365552422,28.2743338823081),
 .UNSPECIFIED.);
#2081=B_SPLINE_CURVE_WITH_KNOTS('',3,(#14544,#14545,#14546,#14547,#14548,
#14549,#14550,#14551,#14552,#14553),.UNSPECIFIED.,.F.,.F.,(4,1,1,1,1,1,
1,4),(21.9911485751285,22.3783692882697,23.3758978227063,24.3734263571429,
25.3709548915795,26.3684834260161,27.3660119604527,28.2743338823081),
 .UNSPECIFIED.);
#2082=B_SPLINE_CURVE_WITH_KNOTS('',3,(#14559,#14560,#14561,#14562,#14563),
 .UNSPECIFIED.,.F.,.F.,(4,1,4),(14.3981410127769,15.3956695472135,15.7079632679489),
 .UNSPECIFIED.);
#2083=B_SPLINE_CURVE_WITH_KNOTS('',3,(#14566,#14567,#14568,#14569,#14570),
 .UNSPECIFIED.,.F.,.F.,(4,1,4),(13.8761928695311,14.8541656075664,15.7079632679489),
 .UNSPECIFIED.);
#2084=B_SPLINE_CURVE_WITH_KNOTS('',3,(#14576,#14577,#14578,#14579,#14580,
#14581,#14582,#14583,#14584,#14585,#14586,#14587,#14588,#14589,#14590,#14591,
#14592,#14593,#14594),.UNSPECIFIED.,.F.,.F.,(4,3,3,3,3,3,4),(95.5576018628658,
95.7627393059136,96.7602678403502,97.7577963747868,98.7553249092234,99.75285344366,
100.750381978097),.UNSPECIFIED.);
#2085=B_SPLINE_CURVE_WITH_KNOTS('',3,(#14598,#14599,#14600,#14601),
 .UNSPECIFIED.,.F.,.F.,(4,4),(-98.735769112822,-98.0941628713861),
 .UNSPECIFIED.);
#2086=B_SPLINE_CURVE_WITH_KNOTS('',3,(#14605,#14606,#14607,#14608,#14609,
#14610,#14611,#14612,#14613,#14614,#14615,#14616,#14617,#14618,#14619,#14620,
#14621,#14622,#14623,#14624,#14625,#14626),.UNSPECIFIED.,.F.,.F.,(4,3,3,
3,3,3,3,4),(-98.0941628713861,-97.7577963747867,-96.7602678403501,-95.7627393059135,
-94.7652107714769,-93.7676822370404,-92.7701537026037,-91.8109775642065),
 .UNSPECIFIED.);
#2087=B_SPLINE_CURVE_WITH_KNOTS('',3,(#14631,#14632,#14633,#14634,#14635,
#14636,#14637,#14638,#14639,#14640,#14641,#14642,#14643,#14644,#14645,#14646,
#14647,#14648,#14649,#14650,#14651,#14652),.UNSPECIFIED.,.F.,.F.,(4,3,3,
3,3,3,3,4),(89.2744165556862,89.777568099294,90.7750966337306,91.7726251681672,
92.7701537026038,93.7676822370404,94.765210771477,95.5576018628658),
 .UNSPECIFIED.);
#2088=B_SPLINE_CURVE_WITH_KNOTS('',3,(#14653,#14654,#14655,#14656,#14657,
#14658,#14659,#14660,#14661,#14662,#14663,#14664,#14665,#14666,#14667,#14668,
#14669,#14670,#14671,#14672,#14673,#14674,#14675,#14676,#14677),
 .UNSPECIFIED.,.F.,.F.,(4,3,3,3,3,3,3,3,4),(-91.8109775642065,-91.7726251681671,
-90.7750966337306,-89.7775680992939,-88.7800395648573,-87.7825110304207,
-86.7849824959842,-85.7874539615475,-85.527792257027),.UNSPECIFIED.);
#2089=B_SPLINE_CURVE_WITH_KNOTS('',3,(#14682,#14683,#14684,#14685,#14686,
#14687,#14688,#14689,#14690,#14691,#14692,#14693,#14694,#14695,#14696,#14697,
#14698,#14699,#14700,#14701,#14702,#14703),.UNSPECIFIED.,.F.,.F.,(4,3,3,
3,3,3,3,4),(82.9912312485066,83.7923968926744,84.789925427111,85.7874539615476,
86.7849824959842,87.7825110304208,88.7800395648574,89.2744165556862),
 .UNSPECIFIED.);
#2090=B_SPLINE_CURVE_WITH_KNOTS('',3,(#14704,#14705,#14706,#14707,#14708,
#14709,#14710,#14711,#14712,#14713,#14714,#14715,#14716,#14717,#14718,#14719,
#14720,#14721,#14722,#14723,#14724,#14725),.UNSPECIFIED.,.F.,.F.,(4,3,3,
3,3,3,3,4),(-85.527792257027,-84.7899254271109,-83.7923968926744,-82.7948683582377,
-81.7973398238012,-80.7998112893646,-79.802282754928,-79.2446069498474),
 .UNSPECIFIED.);
#2091=B_SPLINE_CURVE_WITH_KNOTS('',3,(#14730,#14731,#14732,#14733,#14734,
#14735,#14736,#14737,#14738,#14739,#14740,#14741,#14742,#14743,#14744,#14745,
#14746,#14747,#14748,#14749,#14750,#14751,#14752,#14753,#14754),
 .UNSPECIFIED.,.F.,.F.,(4,3,3,3,3,3,3,3,4),(76.708045941327,76.8096971516182,
77.8072256860548,78.8047542204914,79.802282754928,80.7998112893646,81.7973398238012,
82.7948683582378,82.9912312485066),.UNSPECIFIED.);
#2092=B_SPLINE_CURVE_WITH_KNOTS('',3,(#14755,#14756,#14757,#14758,#14759,
#14760,#14761,#14762,#14763,#14764,#14765,#14766,#14767,#14768,#14769,#14770,
#14771,#14772,#14773,#14774,#14775,#14776),.UNSPECIFIED.,.F.,.F.,(4,3,3,
3,3,3,3,4),(-79.2446069498474,-78.8047542204914,-77.8072256860548,-76.8096971516182,
-75.8121686171816,-74.814640082745,-73.8171115483084,-72.9614216426678),
 .UNSPECIFIED.);
#2093=B_SPLINE_CURVE_WITH_KNOTS('',3,(#14781,#14782,#14783,#14784,#14785,
#14786,#14787,#14788,#14789,#14790,#14791,#14792,#14793,#14794,#14795,#14796,
#14797,#14798,#14799,#14800,#14801,#14802),.UNSPECIFIED.,.F.,.F.,(4,3,3,
3,3,3,3,4),(70.4248606341474,70.8245259449986,71.8220544794352,72.8195830138718,
73.8171115483084,74.814640082745,75.8121686171816,76.708045941327),
 .UNSPECIFIED.);
#2094=B_SPLINE_CURVE_WITH_KNOTS('',3,(#14803,#14804,#14805,#14806,#14807,
#14808,#14809,#14810,#14811,#14812,#14813,#14814,#14815,#14816,#14817,#14818,
#14819,#14820,#14821,#14822,#14823,#14824,#14825,#14826,#14827),
 .UNSPECIFIED.,.F.,.F.,(4,3,3,3,3,3,3,3,4),(-72.9614216426678,-72.8195830138717,
-71.8220544794352,-70.8245259449986,-69.826997410562,-68.8294688761254,
-67.8319403416887,-66.8344118072522,-66.6782363354882),.UNSPECIFIED.);
#2095=B_SPLINE_CURVE_WITH_KNOTS('',3,(#14832,#14833,#14834,#14835,#14836,
#14837,#14838,#14839,#14840,#14841,#14842,#14843,#14844,#14845,#14846,#14847,
#14848,#14849,#14850,#14851,#14852,#14853),.UNSPECIFIED.,.F.,.F.,(4,3,3,
3,3,3,3,4),(64.1416753269678,64.839354738379,65.8368832728156,66.8344118072522,
67.8319403416888,68.8294688761254,69.826997410562,70.4248606341474),
 .UNSPECIFIED.);
#2096=B_SPLINE_CURVE_WITH_KNOTS('',3,(#14854,#14855,#14856,#14857,#14858,
#14859,#14860,#14861,#14862,#14863,#14864,#14865,#14866,#14867,#14868,#14869,
#14870,#14871,#14872,#14873,#14874,#14875),.UNSPECIFIED.,.F.,.F.,(4,3,3,
3,3,3,3,4),(-66.6782363354882,-65.8368832728156,-64.839354738379,-63.8418262039424,
-62.8442976695058,-61.8467691350692,-60.8492406006326,-60.3950510283086),
 .UNSPECIFIED.);
#2097=B_SPLINE_CURVE_WITH_KNOTS('',3,(#14880,#14881,#14882,#14883,#14884,
#14885,#14886,#14887,#14888,#14889,#14890,#14891,#14892,#14893,#14894,#14895,
#14896,#14897,#14898,#14899,#14900,#14901),.UNSPECIFIED.,.F.,.F.,(4,3,3,
3,3,3,3,4),(57.8584900197882,58.8541835317594,59.851712066196,60.8492406006326,
61.8467691350692,62.8442976695058,63.8418262039424,64.1416753269678),
 .UNSPECIFIED.);
#2098=B_SPLINE_CURVE_WITH_KNOTS('',3,(#14902,#14903,#14904,#14905,#14906,
#14907,#14908,#14909,#14910,#14911,#14912,#14913,#14914,#14915,#14916,#14917,
#14918,#14919,#14920,#14921,#14922,#14923),.UNSPECIFIED.,.F.,.F.,(4,3,3,
3,3,3,3,4),(-60.3950510283086,-59.851712066196,-58.8541835317594,-57.8566549973228,
-56.8591264628862,-55.8615979284496,-54.864069394013,-54.111865721129),
 .UNSPECIFIED.);
#2099=B_SPLINE_CURVE_WITH_KNOTS('',3,(#14928,#14929,#14930,#14931,#14932,
#14933,#14934,#14935,#14936,#14937,#14938,#14939,#14940,#14941,#14942,#14943,
#14944,#14945,#14946,#14947,#14948,#14949),.UNSPECIFIED.,.F.,.F.,(4,3,3,
3,3,3,3,4),(51.5753047126086,51.8714837907032,52.8690123251398,53.8665408595764,
54.864069394013,55.8615979284496,56.8591264628862,57.8584900197882),
 .UNSPECIFIED.);
#2100=B_SPLINE_CURVE_WITH_KNOTS('',3,(#14950,#14951,#14952,#14953,#14954,
#14955,#14956,#14957,#14958,#14959,#14960,#14961,#14962,#14963,#14964,#14965,
#14966,#14967,#14968,#14969,#14970,#14971,#14972,#14973,#14974),
 .UNSPECIFIED.,.F.,.F.,(4,3,3,3,3,3,3,3,4),(-54.111865721129,-53.8665408595764,
-52.8690123251398,-51.8714837907032,-50.8739552562666,-49.87642672183,-48.8788981873934,
-47.8813696529568,-47.8286804139494),.UNSPECIFIED.);
#2101=B_SPLINE_CURVE_WITH_KNOTS('',3,(#14979,#14980,#14981,#14982,#14983,
#14984,#14985,#14986,#14987,#14988,#14989,#14990,#14991,#14992,#14993,#14994,
#14995,#14996,#14997,#14998,#14999,#15000),.UNSPECIFIED.,.F.,.F.,(4,3,3,
3,3,3,3,4),(45.292119405429,45.8863125840836,46.8838411185202,47.8813696529568,
48.8788981873934,49.87642672183,50.8739552562666,51.5753047126086),
 .UNSPECIFIED.);
#2102=B_SPLINE_CURVE_WITH_KNOTS('',3,(#15001,#15002,#15003,#15004,#15005,
#15006,#15007,#15008,#15009,#15010,#15011,#15012,#15013,#15014,#15015,#15016,
#15017,#15018,#15019,#15020,#15021,#15022),.UNSPECIFIED.,.F.,.F.,(4,3,3,
3,3,3,3,4),(-47.8286804139494,-46.8838411185202,-45.8863125840836,-44.888784049647,
-43.8912555152104,-42.8937269807738,-41.8961984463372,-41.5454951067698),
 .UNSPECIFIED.);
#2103=B_SPLINE_CURVE_WITH_KNOTS('',3,(#15027,#15028,#15029,#15030,#15031,
#15032,#15033,#15034,#15035,#15036,#15037,#15038,#15039,#15040,#15041,#15042,
#15043,#15044,#15045,#15046,#15047,#15048),.UNSPECIFIED.,.F.,.F.,(4,3,3,
3,3,3,3,4),(39.0089340982494,39.901141377464,40.8986699119006,41.8961984463372,
42.8937269807738,43.8912555152104,44.888784049647,45.292119405429),
 .UNSPECIFIED.);
#2104=B_SPLINE_CURVE_WITH_KNOTS('',3,(#15049,#15050,#15051,#15052,#15053,
#15054,#15055,#15056,#15057,#15058,#15059,#15060,#15061,#15062,#15063,#15064,
#15065,#15066,#15067,#15068,#15069,#15070),.UNSPECIFIED.,.F.,.F.,(4,3,3,
3,3,3,3,4),(-41.5454951067698,-40.8986699119006,-39.901141377464,-38.9036128430274,
-37.9060843085908,-36.9085557741542,-35.9110272397176,-35.2623097995902),
 .UNSPECIFIED.);
#2105=B_SPLINE_CURVE_WITH_KNOTS('',3,(#15075,#15076,#15077,#15078,#15079,
#15080,#15081,#15082,#15083,#15084,#15085,#15086,#15087,#15088,#15089,#15090,
#15091,#15092,#15093,#15094,#15095,#15096,#15097,#15098,#15099),
 .UNSPECIFIED.,.F.,.F.,(4,3,3,3,3,3,3,3,4),(32.7257487910699,32.9184416364078,
33.9159701708444,34.913498705281,35.9110272397176,36.9085557741542,37.9060843085908,
38.9036128430274,39.0089340982494),.UNSPECIFIED.);
#2106=B_SPLINE_CURVE_WITH_KNOTS('',3,(#15100,#15101,#15102,#15103,#15104,
#15105,#15106,#15107,#15108,#15109,#15110,#15111,#15112,#15113,#15114,#15115,
#15116,#15117,#15118,#15119,#15120,#15121),.UNSPECIFIED.,.F.,.F.,(4,3,3,
3,3,3,3,4),(-35.2623097995902,-34.913498705281,-33.9159701708444,-32.9184416364078,
-31.9209131019712,-30.9233845675346,-29.925856033098,-28.9791244924106),
 .UNSPECIFIED.);
#2107=B_SPLINE_CURVE_WITH_KNOTS('',3,(#15126,#15127,#15128,#15129,#15130,
#15131,#15132,#15133,#15134,#15135,#15136,#15137,#15138,#15139,#15140,#15141,
#15142,#15143,#15144,#15145,#15146,#15147),.UNSPECIFIED.,.F.,.F.,(4,3,3,
3,3,3,3,4),(26.4425634838902,26.9332704297882,27.9307989642248,28.9283274986614,
29.925856033098,30.9233845675346,31.9209131019712,32.7257487910699),
 .UNSPECIFIED.);
#2108=B_SPLINE_CURVE_WITH_KNOTS('',3,(#15148,#15149,#15150,#15151,#15152,
#15153,#15154,#15155,#15156,#15157,#15158,#15159,#15160,#15161,#15162,#15163,
#15164,#15165,#15166,#15167,#15168,#15169,#15170,#15171,#15172),
 .UNSPECIFIED.,.F.,.F.,(4,3,3,3,3,3,3,3,4),(-28.9791244924106,-28.9283274986614,
-27.9307989642248,-26.9332704297882,-25.9357418953516,-24.938213360915,
-23.9406848264784,-22.9431562920418,-22.695939185231),.UNSPECIFIED.);
#2109=B_SPLINE_CURVE_WITH_KNOTS('',3,(#15177,#15178,#15179,#15180,#15181,
#15182,#15183,#15184,#15185,#15186,#15187,#15188,#15189,#15190,#15191,#15192,
#15193,#15194,#15195,#15196,#15197,#15198),.UNSPECIFIED.,.F.,.F.,(4,3,3,
3,3,3,3,4),(20.1593781767107,20.9480992231686,21.9456277576052,22.9431562920418,
23.9406848264784,24.938213360915,25.9357418953516,26.4425634838902),
 .UNSPECIFIED.);
#2110=B_SPLINE_CURVE_WITH_KNOTS('',3,(#15199,#15200,#15201,#15202,#15203,
#15204,#15205,#15206,#15207,#15208,#15209,#15210,#15211,#15212,#15213,#15214,
#15215,#15216,#15217,#15218,#15219,#15220),.UNSPECIFIED.,.F.,.F.,(4,3,3,
3,3,3,3,4),(-22.695939185231,-21.9456277576052,-20.9480992231686,-19.950570688732,
-18.9530421542954,-17.9555136198588,-16.9579850854222,-16.4127538780514),
 .UNSPECIFIED.);
#2111=B_SPLINE_CURVE_WITH_KNOTS('',3,(#15225,#15226,#15227,#15228,#15229,
#15230,#15231,#15232,#15233,#15234,#15235,#15236,#15237,#15238,#15239,#15240,
#15241,#15242,#15243,#15244,#15245,#15246,#15247,#15248,#15249),
 .UNSPECIFIED.,.F.,.F.,(4,3,3,3,3,3,3,3,4),(13.8761928695311,13.9653994821124,
14.962928016549,15.9604565509856,16.9579850854222,17.9555136198588,18.9530421542954,
19.950570688732,20.1593781767107),.UNSPECIFIED.);
#2112=B_SPLINE_CURVE_WITH_KNOTS('',3,(#15250,#15251,#15252,#15253,#15254,
#15255,#15256,#15257,#15258,#15259,#15260,#15261,#15262,#15263,#15264,#15265,
#15266,#15267,#15268,#15269,#15270,#15271),.UNSPECIFIED.,.F.,.F.,(4,3,3,
3,3,3,3,4),(-16.4127538780514,-15.9604565509856,-14.962928016549,-13.9653994821124,
-12.9678709476758,-11.9703424132392,-10.9728138788026,-10.1295685708719),
 .UNSPECIFIED.);
#2113=B_SPLINE_CURVE_WITH_KNOTS('',3,(#15277,#15278,#15279,#15280,#15281,
#15282,#15283,#15284,#15285,#15286,#15287,#15288,#15289),.UNSPECIFIED.,
 .F.,.F.,(4,3,3,3,4),(-3.84638326369226,-2.9925856033098,-1.9950570688732,
-0.997528534436601,0.),.UNSPECIFIED.);
#2114=B_SPLINE_CURVE_WITH_KNOTS('',3,(#15292,#15293,#15294,#15295,#15296,
#15297,#15298,#15299,#15300,#15301,#15302,#15303,#15304,#15305,#15306,#15307,
#15308,#15309,#15310),.UNSPECIFIED.,.F.,.F.,(4,3,3,3,3,3,4),(2.01461286527449,
2.9925856033098,3.9901141377464,4.987642672183,5.9851712066196,6.9826997410562,
7.59300756235149),.UNSPECIFIED.);
#2115=B_SPLINE_CURVE_WITH_KNOTS('',3,(#15316,#15317,#15318,#15319,#15320,
#15321),.UNSPECIFIED.,.F.,.F.,(4,1,1,4),(109.955742875643,110.61690491348,
111.614433447917,112.611961982353),.UNSPECIFIED.);
#2116=B_SPLINE_CURVE_WITH_KNOTS('',3,(#15324,#15325,#15326,#15327,#15328,
#15329,#15330),.UNSPECIFIED.,.F.,.F.,(4,1,1,1,4),(109.955742875643,110.16088031869,
111.158408853127,112.155937387564,113.133910125599),.UNSPECIFIED.);
#2117=B_SPLINE_CURVE_WITH_KNOTS('',3,(#15335,#15336,#15337,#15338,#15339,
#15340,#15341,#15342,#15343,#15344),.UNSPECIFIED.,.F.,.F.,(4,1,1,1,1,1,
1,4),(103.672557568463,104.63173370686,105.629262241297,106.626790775734,
107.62431931017,108.621847844607,109.619376379043,109.955742875643),
 .UNSPECIFIED.);
#2118=B_SPLINE_CURVE_WITH_KNOTS('',3,(#15345,#15346,#15347,#15348,#15349,
#15350,#15351,#15352,#15353,#15354),.UNSPECIFIED.,.F.,.F.,(4,1,1,1,1,1,
1,4),(103.672557568463,104.175709112071,105.173237646507,106.170766180944,
107.168294715381,108.165823249817,109.163351784254,109.955742875643),
 .UNSPECIFIED.);
#2119=B_SPLINE_CURVE_WITH_KNOTS('',3,(#15359,#15360,#15361,#15362,#15363,
#15364,#15365,#15366,#15367,#15368,#15369),.UNSPECIFIED.,.F.,.F.,(4,1,1,
1,1,1,1,1,4),(97.3893722612835,97.6490339658042,98.6465625002408,99.6440910346774,
100.641619569114,101.639148103551,102.636676637987,103.634205172424,103.672557568463),
 .UNSPECIFIED.);
#2120=B_SPLINE_CURVE_WITH_KNOTS('',3,(#15370,#15371,#15372,#15373,#15374,
#15375,#15376,#15377,#15378,#15379),.UNSPECIFIED.,.F.,.F.,(4,1,1,1,1,1,
1,4),(97.3893722612835,98.1905379054513,99.1880664398879,100.185594974324,
101.183123508761,102.180652043198,103.178180577634,103.672557568463),
 .UNSPECIFIED.);
#2121=B_SPLINE_CURVE_WITH_KNOTS('',3,(#15384,#15385,#15386,#15387,#15388,
#15389,#15390,#15391,#15392,#15393),.UNSPECIFIED.,.F.,.F.,(4,1,1,1,1,1,
1,4),(91.106186954104,91.6638627591846,92.6613912936212,93.6589198280578,
94.6564483624944,95.653976896931,96.6515054313676,97.3893722612835),
 .UNSPECIFIED.);
#2122=B_SPLINE_CURVE_WITH_KNOTS('',3,(#15394,#15395,#15396,#15397,#15398,
#15399,#15400,#15401,#15402,#15403,#15404),.UNSPECIFIED.,.F.,.F.,(4,1,1,
1,1,1,1,1,4),(91.106186954104,91.2078381643951,92.2053666988317,93.2028952332683,
94.2004237677049,95.1979523021415,96.1954808365781,97.1930093710147,97.3893722612835),
 .UNSPECIFIED.);
#2123=B_SPLINE_CURVE_WITH_KNOTS('',3,(#15409,#15410,#15411,#15412,#15413,
#15414,#15415,#15416,#15417,#15418),.UNSPECIFIED.,.F.,.F.,(4,1,1,1,1,1,
1,4),(84.8230016469244,85.678691552565,86.6762200870016,87.6737486214382,
88.6712771558748,89.6688056903114,90.666334224748,91.106186954104),
 .UNSPECIFIED.);
#2124=B_SPLINE_CURVE_WITH_KNOTS('',3,(#15419,#15420,#15421,#15422,#15423,
#15424,#15425,#15426,#15427,#15428),.UNSPECIFIED.,.F.,.F.,(4,1,1,1,1,1,
1,4),(84.8230016469244,85.2226669577755,86.2201954922121,87.2177240266487,
88.2152525610853,89.2127810955219,90.2103096299585,91.106186954104),
 .UNSPECIFIED.);
#2125=B_SPLINE_CURVE_WITH_KNOTS('',3,(#15433,#15434,#15435,#15436,#15437,
#15438,#15439,#15440,#15441,#15442,#15443),.UNSPECIFIED.,.F.,.F.,(4,1,1,
1,1,1,1,1,4),(78.5398163397448,78.6959918115088,79.6935203459454,80.691048880382,
81.6885774148186,82.6861059492552,83.6836344836918,84.6811630181284,84.8230016469244),
 .UNSPECIFIED.);
#2126=B_SPLINE_CURVE_WITH_KNOTS('',3,(#15444,#15445,#15446,#15447,#15448,
#15449,#15450,#15451,#15452,#15453),.UNSPECIFIED.,.F.,.F.,(4,1,1,1,1,1,
1,4),(78.5398163397448,79.2374957511559,80.2350242855925,81.2325528200291,
82.2300813544657,83.2276098889023,84.2251384233389,84.8230016469244),
 .UNSPECIFIED.);
#2127=B_SPLINE_CURVE_WITH_KNOTS('',3,(#15458,#15459,#15460,#15461,#15462,
#15463,#15464,#15465,#15466,#15467),.UNSPECIFIED.,.F.,.F.,(4,1,1,1,1,1,
1,4),(72.2566310325652,72.7108206048892,73.7083491393258,74.7058776737624,
75.703406208199,76.7009347426356,77.6984632770722,78.5398163397448),
 .UNSPECIFIED.);
#2128=B_SPLINE_CURVE_WITH_KNOTS('',3,(#15468,#15469,#15470,#15471,#15472,
#15473,#15474,#15475,#15476,#15477),.UNSPECIFIED.,.F.,.F.,(4,1,1,1,1,1,
1,4),(72.2566310325652,73.2523245445363,74.2498530789729,75.2473816134095,
76.2449101478461,77.2424386822827,78.2399672167193,78.5398163397448),
 .UNSPECIFIED.);
#2129=B_SPLINE_CURVE_WITH_KNOTS('',3,(#15482,#15483,#15484,#15485,#15486,
#15487,#15488,#15489,#15490,#15491),.UNSPECIFIED.,.F.,.F.,(4,1,1,1,1,1,
1,4),(65.9734457253856,66.7256493982696,67.7231779327062,68.7207064671428,
69.7182350015794,70.715763536016,71.7132920704526,72.2566310325652),
 .UNSPECIFIED.);
#2130=B_SPLINE_CURVE_WITH_KNOTS('',3,(#15492,#15493,#15494,#15495,#15496,
#15497,#15498,#15499,#15500,#15501,#15502),.UNSPECIFIED.,.F.,.F.,(4,1,1,
1,1,1,1,1,4),(65.9734457253856,66.2696248034801,67.2671533379167,68.2646818723533,
69.2622104067899,70.2597389412265,71.2572674756631,72.2547960100997,72.2566310325652),
 .UNSPECIFIED.);
#2131=B_SPLINE_CURVE_WITH_KNOTS('',3,(#15507,#15508,#15509,#15510,#15511,
#15512,#15513,#15514,#15515,#15516,#15517),.UNSPECIFIED.,.F.,.F.,(4,1,1,
1,1,1,1,1,4),(59.690260418206,59.7429496572134,60.74047819165,61.7380067260866,
62.7355352605232,63.7330637949598,64.7305923293964,65.728120863833,65.9734457253856),
 .UNSPECIFIED.);
#2132=B_SPLINE_CURVE_WITH_KNOTS('',3,(#15518,#15519,#15520,#15521,#15522,
#15523,#15524,#15525,#15526,#15527),.UNSPECIFIED.,.F.,.F.,(4,1,1,1,1,1,
1,4),(59.690260418206,60.2844535968605,61.2819821312971,62.2795106657337,
63.2770392001703,64.2745677346069,65.2720962690435,65.9734457253856),
 .UNSPECIFIED.);
#2133=B_SPLINE_CURVE_WITH_KNOTS('',3,(#15532,#15533,#15534,#15535,#15536,
#15537,#15538,#15539,#15540,#15541),.UNSPECIFIED.,.F.,.F.,(4,1,1,1,1,1,
1,4),(53.4070751110264,53.7577784505938,54.7553069850304,55.752835519467,
56.7503640539036,57.7478925883402,58.7454211227768,59.690260418206),
 .UNSPECIFIED.);
#2134=B_SPLINE_CURVE_WITH_KNOTS('',3,(#15542,#15543,#15544,#15545,#15546,
#15547,#15548,#15549,#15550,#15551),.UNSPECIFIED.,.F.,.F.,(4,1,1,1,1,1,
1,4),(53.4070751110264,54.2992823902409,55.2968109246775,56.2943394591141,
57.2918679935507,58.2893965279873,59.2869250624239,59.690260418206),
 .UNSPECIFIED.);
#2135=B_SPLINE_CURVE_WITH_KNOTS('',3,(#15556,#15557,#15558,#15559,#15560,
#15561,#15562,#15563,#15564,#15565),.UNSPECIFIED.,.F.,.F.,(4,1,1,1,1,1,
1,4),(47.1238898038468,47.7726072439742,48.7701357784108,49.7676643128474,
50.765192847284,51.7627213817206,52.7602499161572,53.4070751110264),
 .UNSPECIFIED.);
#2136=B_SPLINE_CURVE_WITH_KNOTS('',3,(#15566,#15567,#15568,#15569,#15570,
#15571,#15572,#15573,#15574,#15575,#15576),.UNSPECIFIED.,.F.,.F.,(4,1,1,
1,1,1,1,1,4),(47.1238898038468,47.3165826491847,48.3141111836213,49.3116397180579,
50.3091682524945,51.3066967869311,52.3042253213677,53.3017538558043,53.4070751110264),
 .UNSPECIFIED.);
#2137=B_SPLINE_CURVE_WITH_KNOTS('',3,(#15581,#15582,#15583,#15584,#15585,
#15586,#15587,#15588,#15589,#15590),.UNSPECIFIED.,.F.,.F.,(4,1,1,1,1,1,
1,4),(40.8407044966673,41.7874360373546,42.7849645717912,43.7824931062278,
44.7800216406644,45.777550175101,46.7750787095376,47.1238898038468),
 .UNSPECIFIED.);
#2138=B_SPLINE_CURVE_WITH_KNOTS('',3,(#15591,#15592,#15593,#15594,#15595,
#15596,#15597,#15598,#15599,#15600),.UNSPECIFIED.,.F.,.F.,(4,1,1,1,1,1,
1,4),(40.8407044966673,41.3314114425651,42.3289399770017,43.3264685114383,
44.3239970458749,45.3215255803115,46.3190541147481,47.1238898038468),
 .UNSPECIFIED.);
#2139=B_SPLINE_CURVE_WITH_KNOTS('',3,(#15605,#15606,#15607,#15608,#15609,
#15610,#15611,#15612,#15613,#15614,#15615),.UNSPECIFIED.,.F.,.F.,(4,1,1,
1,1,1,1,1,4),(34.5575191894876,34.8047362962984,35.802264830735,36.7997933651716,
37.7973218996082,38.7948504340448,39.7923789684814,40.789907502918,40.8407044966673),
 .UNSPECIFIED.);
#2140=B_SPLINE_CURVE_WITH_KNOTS('',3,(#15616,#15617,#15618,#15619,#15620,
#15621,#15622,#15623,#15624,#15625),.UNSPECIFIED.,.F.,.F.,(4,1,1,1,1,1,
1,4),(34.5575191894876,35.3462402359455,36.3437687703821,37.3412973048187,
38.3388258392553,39.3363543736919,40.3338829081285,40.8407044966673),
 .UNSPECIFIED.);
#2141=B_SPLINE_CURVE_WITH_KNOTS('',3,(#15630,#15631,#15632,#15633,#15634,
#15635,#15636,#15637,#15638,#15639),.UNSPECIFIED.,.F.,.F.,(4,1,1,1,1,1,
1,4),(28.2743338823081,28.8195650896788,29.8170936241154,30.814622158552,
31.8121506929886,32.8096792274252,33.8072077618618,34.5575191894876),
 .UNSPECIFIED.);
#2142=B_SPLINE_CURVE_WITH_KNOTS('',3,(#15640,#15641,#15642,#15643,#15644,
#15645,#15646,#15647,#15648,#15649,#15650),.UNSPECIFIED.,.F.,.F.,(4,1,1,
1,1,1,1,1,4),(28.2743338823081,28.3635404948893,29.3610690293259,30.3585975637625,
31.3561260981991,32.3536546326357,33.3511831670723,34.3487117015089,34.5575191894876),
 .UNSPECIFIED.);
#2143=B_SPLINE_CURVE_WITH_KNOTS('',3,(#15655,#15656,#15657,#15658,#15659,
#15660,#15661,#15662,#15663,#15664),.UNSPECIFIED.,.F.,.F.,(4,1,1,1,1,1,
1,4),(21.9911485751284,22.8343938830592,23.8319224174958,24.8294509519324,
25.826979486369,26.8245080208056,27.8220365552422,28.2743338823081),
 .UNSPECIFIED.);
#2144=B_SPLINE_CURVE_WITH_KNOTS('',3,(#15665,#15666,#15667,#15668,#15669,
#15670,#15671,#15672,#15673,#15674),.UNSPECIFIED.,.F.,.F.,(4,1,1,1,1,1,
1,4),(21.9911485751284,22.3783692882697,23.3758978227063,24.3734263571429,
25.3709548915795,26.3684834260161,27.3660119604527,28.2743338823081),
 .UNSPECIFIED.);
#2145=B_SPLINE_CURVE_WITH_KNOTS('',3,(#15680,#15681,#15682,#15683,#15684),
 .UNSPECIFIED.,.F.,.F.,(4,1,4),(14.3981410127769,15.3956695472135,15.7079632679489),
 .UNSPECIFIED.);
#2146=B_SPLINE_CURVE_WITH_KNOTS('',3,(#15687,#15688,#15689,#15690,#15691),
 .UNSPECIFIED.,.F.,.F.,(4,1,4),(13.8761928695311,14.8541656075664,15.7079632679489),
 .UNSPECIFIED.);
#2147=B_SPLINE_CURVE_WITH_KNOTS('',3,(#15697,#15698,#15699,#15700,#15701,
#15702,#15703,#15704,#15705,#15706,#15707,#15708,#15709,#15710,#15711,#15712,
#15713,#15714,#15715),.UNSPECIFIED.,.F.,.F.,(4,3,3,3,3,3,4),(95.5576018628658,
95.7627393059135,96.7602678403502,97.7577963747867,98.7553249092234,99.75285344366,
100.750381978096),.UNSPECIFIED.);
#2148=B_SPLINE_CURVE_WITH_KNOTS('',3,(#15719,#15720,#15721,#15722),
 .UNSPECIFIED.,.F.,.F.,(4,4),(-98.735769112822,-98.0941628713861),
 .UNSPECIFIED.);
#2149=B_SPLINE_CURVE_WITH_KNOTS('',3,(#15726,#15727,#15728,#15729,#15730,
#15731,#15732,#15733,#15734,#15735,#15736,#15737,#15738,#15739,#15740,#15741,
#15742,#15743,#15744,#15745,#15746,#15747),.UNSPECIFIED.,.F.,.F.,(4,3,3,
3,3,3,3,4),(-98.0941628713861,-97.7577963747868,-96.7602678403502,-95.7627393059136,
-94.765210771477,-93.7676822370404,-92.7701537026038,-91.8109775642066),
 .UNSPECIFIED.);
#2150=B_SPLINE_CURVE_WITH_KNOTS('',3,(#15752,#15753,#15754,#15755,#15756,
#15757,#15758,#15759,#15760,#15761,#15762,#15763,#15764,#15765,#15766,#15767,
#15768,#15769,#15770,#15771,#15772,#15773),.UNSPECIFIED.,.F.,.F.,(4,3,3,
3,3,3,3,4),(89.2744165556862,89.777568099294,90.7750966337306,91.7726251681672,
92.7701537026037,93.7676822370404,94.7652107714769,95.5576018628658),
 .UNSPECIFIED.);
#2151=B_SPLINE_CURVE_WITH_KNOTS('',3,(#15774,#15775,#15776,#15777,#15778,
#15779,#15780,#15781,#15782,#15783,#15784,#15785,#15786,#15787,#15788,#15789,
#15790,#15791,#15792,#15793,#15794,#15795,#15796,#15797,#15798),
 .UNSPECIFIED.,.F.,.F.,(4,3,3,3,3,3,3,3,4),(-91.8109775642066,-91.7726251681672,
-90.7750966337306,-89.777568099294,-88.7800395648574,-87.7825110304208,
-86.7849824959842,-85.7874539615476,-85.527792257027),.UNSPECIFIED.);
#2152=B_SPLINE_CURVE_WITH_KNOTS('',3,(#15803,#15804,#15805,#15806,#15807,
#15808,#15809,#15810,#15811,#15812,#15813,#15814,#15815,#15816,#15817,#15818,
#15819,#15820,#15821,#15822,#15823,#15824),.UNSPECIFIED.,.F.,.F.,(4,3,3,
3,3,3,3,4),(82.9912312485066,83.7923968926744,84.789925427111,85.7874539615476,
86.7849824959842,87.7825110304208,88.7800395648573,89.2744165556862),
 .UNSPECIFIED.);
#2153=B_SPLINE_CURVE_WITH_KNOTS('',3,(#15825,#15826,#15827,#15828,#15829,
#15830,#15831,#15832,#15833,#15834,#15835,#15836,#15837,#15838,#15839,#15840,
#15841,#15842,#15843,#15844,#15845,#15846),.UNSPECIFIED.,.F.,.F.,(4,3,3,
3,3,3,3,4),(-85.527792257027,-84.789925427111,-83.7923968926744,-82.7948683582378,
-81.7973398238012,-80.7998112893646,-79.802282754928,-79.2446069498474),
 .UNSPECIFIED.);
#2154=B_SPLINE_CURVE_WITH_KNOTS('',3,(#15851,#15852,#15853,#15854,#15855,
#15856,#15857,#15858,#15859,#15860,#15861,#15862,#15863,#15864,#15865,#15866,
#15867,#15868,#15869,#15870,#15871,#15872,#15873,#15874,#15875),
 .UNSPECIFIED.,.F.,.F.,(4,3,3,3,3,3,3,3,4),(76.708045941327,76.8096971516182,
77.8072256860548,78.8047542204914,79.802282754928,80.7998112893646,81.7973398238012,
82.7948683582378,82.9912312485066),.UNSPECIFIED.);
#2155=B_SPLINE_CURVE_WITH_KNOTS('',3,(#15876,#15877,#15878,#15879,#15880,
#15881,#15882,#15883,#15884,#15885,#15886,#15887,#15888,#15889,#15890,#15891,
#15892,#15893,#15894,#15895,#15896,#15897),.UNSPECIFIED.,.F.,.F.,(4,3,3,
3,3,3,3,4),(-79.2446069498474,-78.8047542204914,-77.8072256860548,-76.8096971516182,
-75.8121686171816,-74.814640082745,-73.8171115483084,-72.9614216426678),
 .UNSPECIFIED.);
#2156=B_SPLINE_CURVE_WITH_KNOTS('',3,(#15902,#15903,#15904,#15905,#15906,
#15907,#15908,#15909,#15910,#15911,#15912,#15913,#15914,#15915,#15916,#15917,
#15918,#15919,#15920,#15921,#15922,#15923),.UNSPECIFIED.,.F.,.F.,(4,3,3,
3,3,3,3,4),(70.4248606341474,70.8245259449986,71.8220544794352,72.8195830138718,
73.8171115483084,74.814640082745,75.8121686171816,76.708045941327),
 .UNSPECIFIED.);
#2157=B_SPLINE_CURVE_WITH_KNOTS('',3,(#15924,#15925,#15926,#15927,#15928,
#15929,#15930,#15931,#15932,#15933,#15934,#15935,#15936,#15937,#15938,#15939,
#15940,#15941,#15942,#15943,#15944,#15945,#15946,#15947,#15948),
 .UNSPECIFIED.,.F.,.F.,(4,3,3,3,3,3,3,3,4),(-72.9614216426678,-72.8195830138718,
-71.8220544794352,-70.8245259449986,-69.826997410562,-68.8294688761254,
-67.8319403416888,-66.8344118072522,-66.6782363354882),.UNSPECIFIED.);
#2158=B_SPLINE_CURVE_WITH_KNOTS('',3,(#15953,#15954,#15955,#15956,#15957,
#15958,#15959,#15960,#15961,#15962,#15963,#15964,#15965,#15966,#15967,#15968,
#15969,#15970,#15971,#15972,#15973,#15974),.UNSPECIFIED.,.F.,.F.,(4,3,3,
3,3,3,3,4),(64.1416753269678,64.839354738379,65.8368832728156,66.8344118072522,
67.8319403416888,68.8294688761254,69.826997410562,70.4248606341474),
 .UNSPECIFIED.);
#2159=B_SPLINE_CURVE_WITH_KNOTS('',3,(#15975,#15976,#15977,#15978,#15979,
#15980,#15981,#15982,#15983,#15984,#15985,#15986,#15987,#15988,#15989,#15990,
#15991,#15992,#15993,#15994,#15995,#15996),.UNSPECIFIED.,.F.,.F.,(4,3,3,
3,3,3,3,4),(-66.6782363354882,-65.8368832728156,-64.839354738379,-63.8418262039424,
-62.8442976695058,-61.8467691350692,-60.8492406006326,-60.3950510283086),
 .UNSPECIFIED.);
#2160=B_SPLINE_CURVE_WITH_KNOTS('',3,(#16001,#16002,#16003,#16004,#16005,
#16006,#16007,#16008,#16009,#16010,#16011,#16012,#16013,#16014,#16015,#16016,
#16017,#16018,#16019,#16020,#16021,#16022),.UNSPECIFIED.,.F.,.F.,(4,3,3,
3,3,3,3,4),(57.8584900197883,58.8541835317594,59.851712066196,60.8492406006326,
61.8467691350692,62.8442976695058,63.8418262039424,64.1416753269678),
 .UNSPECIFIED.);
#2161=B_SPLINE_CURVE_WITH_KNOTS('',3,(#16023,#16024,#16025,#16026,#16027,
#16028,#16029,#16030,#16031,#16032,#16033,#16034,#16035,#16036,#16037,#16038,
#16039,#16040,#16041,#16042,#16043,#16044),.UNSPECIFIED.,.F.,.F.,(4,3,3,
3,3,3,3,4),(-60.3950510283086,-59.851712066196,-58.8541835317594,-57.8566549973228,
-56.8591264628862,-55.8615979284496,-54.864069394013,-54.111865721129),
 .UNSPECIFIED.);
#2162=B_SPLINE_CURVE_WITH_KNOTS('',3,(#16049,#16050,#16051,#16052,#16053,
#16054,#16055,#16056,#16057,#16058,#16059,#16060,#16061,#16062,#16063,#16064,
#16065,#16066,#16067,#16068,#16069,#16070),.UNSPECIFIED.,.F.,.F.,(4,3,3,
3,3,3,3,4),(51.5753047126087,51.8714837907032,52.8690123251398,53.8665408595764,
54.864069394013,55.8615979284496,56.8591264628862,57.8584900197883),
 .UNSPECIFIED.);
#2163=B_SPLINE_CURVE_WITH_KNOTS('',3,(#16071,#16072,#16073,#16074,#16075,
#16076,#16077,#16078,#16079,#16080,#16081,#16082,#16083,#16084,#16085,#16086,
#16087,#16088,#16089,#16090,#16091,#16092,#16093,#16094,#16095),
 .UNSPECIFIED.,.F.,.F.,(4,3,3,3,3,3,3,3,4),(-54.111865721129,-53.8665408595764,
-52.8690123251398,-51.8714837907032,-50.8739552562666,-49.87642672183,-48.8788981873934,
-47.8813696529568,-47.8286804139494),.UNSPECIFIED.);
#2164=B_SPLINE_CURVE_WITH_KNOTS('',3,(#16100,#16101,#16102,#16103,#16104,
#16105,#16106,#16107,#16108,#16109,#16110,#16111,#16112,#16113,#16114,#16115,
#16116,#16117,#16118,#16119,#16120,#16121),.UNSPECIFIED.,.F.,.F.,(4,3,3,
3,3,3,3,4),(45.292119405429,45.8863125840836,46.8838411185202,47.8813696529568,
48.8788981873934,49.87642672183,50.8739552562666,51.5753047126087),
 .UNSPECIFIED.);
#2165=B_SPLINE_CURVE_WITH_KNOTS('',3,(#16122,#16123,#16124,#16125,#16126,
#16127,#16128,#16129,#16130,#16131,#16132,#16133,#16134,#16135,#16136,#16137,
#16138,#16139,#16140,#16141,#16142,#16143),.UNSPECIFIED.,.F.,.F.,(4,3,3,
3,3,3,3,4),(-47.8286804139494,-46.8838411185202,-45.8863125840836,-44.888784049647,
-43.8912555152104,-42.8937269807738,-41.8961984463372,-41.5454951067698),
 .UNSPECIFIED.);
#2166=B_SPLINE_CURVE_WITH_KNOTS('',3,(#16148,#16149,#16150,#16151,#16152,
#16153,#16154,#16155,#16156,#16157,#16158,#16159,#16160,#16161,#16162,#16163,
#16164,#16165,#16166,#16167,#16168,#16169),.UNSPECIFIED.,.F.,.F.,(4,3,3,
3,3,3,3,4),(39.0089340982495,39.901141377464,40.8986699119006,41.8961984463372,
42.8937269807738,43.8912555152104,44.888784049647,45.292119405429),
 .UNSPECIFIED.);
#2167=B_SPLINE_CURVE_WITH_KNOTS('',3,(#16170,#16171,#16172,#16173,#16174,
#16175,#16176,#16177,#16178,#16179,#16180,#16181,#16182,#16183,#16184,#16185,
#16186,#16187,#16188,#16189,#16190,#16191),.UNSPECIFIED.,.F.,.F.,(4,3,3,
3,3,3,3,4),(-41.5454951067698,-40.8986699119006,-39.901141377464,-38.9036128430274,
-37.9060843085908,-36.9085557741542,-35.9110272397176,-35.2623097995902),
 .UNSPECIFIED.);
#2168=B_SPLINE_CURVE_WITH_KNOTS('',3,(#16196,#16197,#16198,#16199,#16200,
#16201,#16202,#16203,#16204,#16205,#16206,#16207,#16208,#16209,#16210,#16211,
#16212,#16213,#16214,#16215,#16216,#16217,#16218,#16219,#16220),
 .UNSPECIFIED.,.F.,.F.,(4,3,3,3,3,3,3,3,4),(32.7257487910699,32.9184416364078,
33.9159701708444,34.913498705281,35.9110272397176,36.9085557741542,37.9060843085908,
38.9036128430274,39.0089340982495),.UNSPECIFIED.);
#2169=B_SPLINE_CURVE_WITH_KNOTS('',3,(#16221,#16222,#16223,#16224,#16225,
#16226,#16227,#16228,#16229,#16230,#16231,#16232,#16233,#16234,#16235,#16236,
#16237,#16238,#16239,#16240,#16241,#16242),.UNSPECIFIED.,.F.,.F.,(4,3,3,
3,3,3,3,4),(-35.2623097995902,-34.913498705281,-33.9159701708444,-32.9184416364078,
-31.9209131019712,-30.9233845675346,-29.925856033098,-28.9791244924106),
 .UNSPECIFIED.);
#2170=B_SPLINE_CURVE_WITH_KNOTS('',3,(#16247,#16248,#16249,#16250,#16251,
#16252,#16253,#16254,#16255,#16256,#16257,#16258,#16259,#16260,#16261,#16262,
#16263,#16264,#16265,#16266,#16267,#16268),.UNSPECIFIED.,.F.,.F.,(4,3,3,
3,3,3,3,4),(26.4425634838903,26.9332704297882,27.9307989642248,28.9283274986614,
29.925856033098,30.9233845675346,31.9209131019712,32.7257487910699),
 .UNSPECIFIED.);
#2171=B_SPLINE_CURVE_WITH_KNOTS('',3,(#16269,#16270,#16271,#16272,#16273,
#16274,#16275,#16276,#16277,#16278,#16279,#16280,#16281,#16282,#16283,#16284,
#16285,#16286,#16287,#16288,#16289,#16290,#16291,#16292,#16293),
 .UNSPECIFIED.,.F.,.F.,(4,3,3,3,3,3,3,3,4),(-28.9791244924106,-28.9283274986614,
-27.9307989642248,-26.9332704297882,-25.9357418953516,-24.938213360915,
-23.9406848264784,-22.9431562920418,-22.6959391852311),.UNSPECIFIED.);
#2172=B_SPLINE_CURVE_WITH_KNOTS('',3,(#16298,#16299,#16300,#16301,#16302,
#16303,#16304,#16305,#16306,#16307,#16308,#16309,#16310,#16311,#16312,#16313,
#16314,#16315,#16316,#16317,#16318,#16319),.UNSPECIFIED.,.F.,.F.,(4,3,3,
3,3,3,3,4),(20.1593781767107,20.9480992231686,21.9456277576052,22.9431562920418,
23.9406848264784,24.938213360915,25.9357418953516,26.4425634838903),
 .UNSPECIFIED.);
#2173=B_SPLINE_CURVE_WITH_KNOTS('',3,(#16320,#16321,#16322,#16323,#16324,
#16325,#16326,#16327,#16328,#16329,#16330,#16331,#16332,#16333,#16334,#16335,
#16336,#16337,#16338,#16339,#16340,#16341),.UNSPECIFIED.,.F.,.F.,(4,3,3,
3,3,3,3,4),(-22.6959391852311,-21.9456277576052,-20.9480992231686,-19.950570688732,
-18.9530421542954,-17.9555136198588,-16.9579850854222,-16.4127538780514),
 .UNSPECIFIED.);
#2174=B_SPLINE_CURVE_WITH_KNOTS('',3,(#16346,#16347,#16348,#16349,#16350,
#16351,#16352,#16353,#16354,#16355,#16356,#16357,#16358,#16359,#16360,#16361,
#16362,#16363,#16364,#16365,#16366,#16367,#16368,#16369,#16370),
 .UNSPECIFIED.,.F.,.F.,(4,3,3,3,3,3,3,3,4),(13.8761928695311,13.9653994821124,
14.962928016549,15.9604565509856,16.9579850854222,17.9555136198588,18.9530421542954,
19.950570688732,20.1593781767107),.UNSPECIFIED.);
#2175=B_SPLINE_CURVE_WITH_KNOTS('',3,(#16371,#16372,#16373,#16374,#16375,
#16376,#16377,#16378,#16379,#16380,#16381,#16382,#16383,#16384,#16385,#16386,
#16387,#16388,#16389,#16390,#16391,#16392),.UNSPECIFIED.,.F.,.F.,(4,3,3,
3,3,3,3,4),(-16.4127538780514,-15.9604565509856,-14.962928016549,-13.9653994821124,
-12.9678709476758,-11.9703424132392,-10.9728138788026,-10.1295685708719),
 .UNSPECIFIED.);
#2176=B_SPLINE_CURVE_WITH_KNOTS('',3,(#16398,#16399,#16400,#16401,#16402,
#16403,#16404,#16405,#16406,#16407,#16408,#16409,#16410),.UNSPECIFIED.,
 .F.,.F.,(4,3,3,3,4),(-3.8463832636923,-2.9925856033098,-1.9950570688732,
-0.997528534436595,0.),.UNSPECIFIED.);
#2177=B_SPLINE_CURVE_WITH_KNOTS('',3,(#16413,#16414,#16415,#16416,#16417,
#16418,#16419,#16420,#16421,#16422,#16423,#16424,#16425,#16426,#16427,#16428,
#16429,#16430,#16431),.UNSPECIFIED.,.F.,.F.,(4,3,3,3,3,3,4),(2.01461286527449,
2.9925856033098,3.9901141377464,4.98764267218299,5.98517120661959,6.98269974105619,
7.59300756235153),.UNSPECIFIED.);
#2178=B_SPLINE_CURVE_WITH_KNOTS('',3,(#16437,#16438,#16439,#16440,#16441,
#16442),.UNSPECIFIED.,.F.,.F.,(4,1,1,4),(109.955742875643,110.61690491348,
111.614433447917,112.611961982353),.UNSPECIFIED.);
#2179=B_SPLINE_CURVE_WITH_KNOTS('',3,(#16445,#16446,#16447,#16448,#16449,
#16450,#16451),.UNSPECIFIED.,.F.,.F.,(4,1,1,1,4),(109.955742875643,110.16088031869,
111.158408853127,112.155937387564,113.133910125599),.UNSPECIFIED.);
#2180=B_SPLINE_CURVE_WITH_KNOTS('',3,(#16456,#16457,#16458,#16459,#16460,
#16461,#16462,#16463,#16464,#16465),.UNSPECIFIED.,.F.,.F.,(4,1,1,1,1,1,
1,4),(103.672557568463,104.63173370686,105.629262241297,106.626790775734,
107.62431931017,108.621847844607,109.619376379043,109.955742875643),
 .UNSPECIFIED.);
#2181=B_SPLINE_CURVE_WITH_KNOTS('',3,(#16466,#16467,#16468,#16469,#16470,
#16471,#16472,#16473,#16474,#16475),.UNSPECIFIED.,.F.,.F.,(4,1,1,1,1,1,
1,4),(103.672557568463,104.175709112071,105.173237646507,106.170766180944,
107.168294715381,108.165823249817,109.163351784254,109.955742875643),
 .UNSPECIFIED.);
#2182=B_SPLINE_CURVE_WITH_KNOTS('',3,(#16480,#16481,#16482,#16483,#16484,
#16485,#16486,#16487,#16488,#16489,#16490),.UNSPECIFIED.,.F.,.F.,(4,1,1,
1,1,1,1,1,4),(97.3893722612836,97.6490339658042,98.6465625002408,99.6440910346774,
100.641619569114,101.639148103551,102.636676637987,103.634205172424,103.672557568463),
 .UNSPECIFIED.);
#2183=B_SPLINE_CURVE_WITH_KNOTS('',3,(#16491,#16492,#16493,#16494,#16495,
#16496,#16497,#16498,#16499,#16500),.UNSPECIFIED.,.F.,.F.,(4,1,1,1,1,1,
1,4),(97.3893722612836,98.1905379054512,99.1880664398878,100.185594974324,
101.183123508761,102.180652043198,103.178180577634,103.672557568463),
 .UNSPECIFIED.);
#2184=B_SPLINE_CURVE_WITH_KNOTS('',3,(#16505,#16506,#16507,#16508,#16509,
#16510,#16511,#16512,#16513,#16514),.UNSPECIFIED.,.F.,.F.,(4,1,1,1,1,1,
1,4),(91.106186954104,91.6638627591846,92.6613912936212,93.6589198280578,
94.6564483624944,95.653976896931,96.6515054313676,97.3893722612836),
 .UNSPECIFIED.);
#2185=B_SPLINE_CURVE_WITH_KNOTS('',3,(#16515,#16516,#16517,#16518,#16519,
#16520,#16521,#16522,#16523,#16524,#16525),.UNSPECIFIED.,.F.,.F.,(4,1,1,
1,1,1,1,1,4),(91.106186954104,91.207838164395,92.2053666988316,93.2028952332682,
94.2004237677048,95.1979523021414,96.195480836578,97.1930093710146,97.3893722612836),
 .UNSPECIFIED.);
#2186=B_SPLINE_CURVE_WITH_KNOTS('',3,(#16530,#16531,#16532,#16533,#16534,
#16535,#16536,#16537,#16538,#16539),.UNSPECIFIED.,.F.,.F.,(4,1,1,1,1,1,
1,4),(84.8230016469244,85.678691552565,86.6762200870016,87.6737486214382,
88.6712771558748,89.6688056903114,90.666334224748,91.106186954104),
 .UNSPECIFIED.);
#2187=B_SPLINE_CURVE_WITH_KNOTS('',3,(#16540,#16541,#16542,#16543,#16544,
#16545,#16546,#16547,#16548,#16549),.UNSPECIFIED.,.F.,.F.,(4,1,1,1,1,1,
1,4),(84.8230016469244,85.2226669577754,86.220195492212,87.2177240266486,
88.2152525610852,89.2127810955218,90.2103096299584,91.106186954104),
 .UNSPECIFIED.);
#2188=B_SPLINE_CURVE_WITH_KNOTS('',3,(#16554,#16555,#16556,#16557,#16558,
#16559,#16560,#16561,#16562,#16563,#16564),.UNSPECIFIED.,.F.,.F.,(4,1,1,
1,1,1,1,1,4),(78.5398163397448,78.6959918115088,79.6935203459454,80.691048880382,
81.6885774148186,82.6861059492552,83.6836344836918,84.6811630181284,84.8230016469244),
 .UNSPECIFIED.);
#2189=B_SPLINE_CURVE_WITH_KNOTS('',3,(#16565,#16566,#16567,#16568,#16569,
#16570,#16571,#16572,#16573,#16574),.UNSPECIFIED.,.F.,.F.,(4,1,1,1,1,1,
1,4),(78.5398163397448,79.2374957511558,80.2350242855924,81.232552820029,
82.2300813544656,83.2276098889022,84.2251384233388,84.8230016469244),
 .UNSPECIFIED.);
#2190=B_SPLINE_CURVE_WITH_KNOTS('',3,(#16579,#16580,#16581,#16582,#16583,
#16584,#16585,#16586,#16587,#16588),.UNSPECIFIED.,.F.,.F.,(4,1,1,1,1,1,
1,4),(72.2566310325652,72.7108206048892,73.7083491393258,74.7058776737624,
75.703406208199,76.7009347426356,77.6984632770722,78.5398163397448),
 .UNSPECIFIED.);
#2191=B_SPLINE_CURVE_WITH_KNOTS('',3,(#16589,#16590,#16591,#16592,#16593,
#16594,#16595,#16596,#16597,#16598),.UNSPECIFIED.,.F.,.F.,(4,1,1,1,1,1,
1,4),(72.2566310325652,73.2523245445362,74.2498530789728,75.2473816134094,
76.244910147846,77.2424386822826,78.2399672167192,78.5398163397448),
 .UNSPECIFIED.);
#2192=B_SPLINE_CURVE_WITH_KNOTS('',3,(#16603,#16604,#16605,#16606,#16607,
#16608,#16609,#16610,#16611,#16612),.UNSPECIFIED.,.F.,.F.,(4,1,1,1,1,1,
1,4),(65.9734457253856,66.7256493982696,67.7231779327062,68.7207064671428,
69.7182350015794,70.715763536016,71.7132920704526,72.2566310325652),
 .UNSPECIFIED.);
#2193=B_SPLINE_CURVE_WITH_KNOTS('',3,(#16613,#16614,#16615,#16616,#16617,
#16618,#16619,#16620,#16621,#16622,#16623),.UNSPECIFIED.,.F.,.F.,(4,1,1,
1,1,1,1,1,4),(65.9734457253856,66.26962480348,67.2671533379166,68.2646818723533,
69.2622104067898,70.2597389412264,71.257267475663,72.2547960100996,72.2566310325652),
 .UNSPECIFIED.);
#2194=B_SPLINE_CURVE_WITH_KNOTS('',3,(#16628,#16629,#16630,#16631,#16632,
#16633,#16634,#16635,#16636,#16637,#16638),.UNSPECIFIED.,.F.,.F.,(4,1,1,
1,1,1,1,1,4),(59.690260418206,59.7429496572134,60.74047819165,61.7380067260866,
62.7355352605232,63.7330637949598,64.7305923293964,65.728120863833,65.9734457253856),
 .UNSPECIFIED.);
#2195=B_SPLINE_CURVE_WITH_KNOTS('',3,(#16639,#16640,#16641,#16642,#16643,
#16644,#16645,#16646,#16647,#16648),.UNSPECIFIED.,.F.,.F.,(4,1,1,1,1,1,
1,4),(59.690260418206,60.2844535968604,61.281982131297,62.2795106657336,
63.2770392001703,64.2745677346068,65.2720962690434,65.9734457253856),
 .UNSPECIFIED.);
#2196=B_SPLINE_CURVE_WITH_KNOTS('',3,(#16653,#16654,#16655,#16656,#16657,
#16658,#16659,#16660,#16661,#16662),.UNSPECIFIED.,.F.,.F.,(4,1,1,1,1,1,
1,4),(53.4070751110264,53.7577784505938,54.7553069850304,55.752835519467,
56.7503640539036,57.7478925883402,58.7454211227768,59.690260418206),
 .UNSPECIFIED.);
#2197=B_SPLINE_CURVE_WITH_KNOTS('',3,(#16663,#16664,#16665,#16666,#16667,
#16668,#16669,#16670,#16671,#16672),.UNSPECIFIED.,.F.,.F.,(4,1,1,1,1,1,
1,4),(53.4070751110264,54.2992823902408,55.2968109246774,56.294339459114,
57.2918679935507,58.2893965279873,59.2869250624238,59.690260418206),
 .UNSPECIFIED.);
#2198=B_SPLINE_CURVE_WITH_KNOTS('',3,(#16677,#16678,#16679,#16680,#16681,
#16682,#16683,#16684,#16685,#16686),.UNSPECIFIED.,.F.,.F.,(4,1,1,1,1,1,
1,4),(47.1238898038469,47.7726072439742,48.7701357784108,49.7676643128474,
50.765192847284,51.7627213817206,52.7602499161572,53.4070751110264),
 .UNSPECIFIED.);
#2199=B_SPLINE_CURVE_WITH_KNOTS('',3,(#16687,#16688,#16689,#16690,#16691,
#16692,#16693,#16694,#16695,#16696,#16697),.UNSPECIFIED.,.F.,.F.,(4,1,1,
1,1,1,1,1,4),(47.1238898038469,47.3165826491847,48.3141111836213,49.3116397180578,
50.3091682524944,51.3066967869311,52.3042253213677,53.3017538558043,53.4070751110264),
 .UNSPECIFIED.);
#2200=B_SPLINE_CURVE_WITH_KNOTS('',3,(#16702,#16703,#16704,#16705,#16706,
#16707,#16708,#16709,#16710,#16711),.UNSPECIFIED.,.F.,.F.,(4,1,1,1,1,1,
1,4),(40.8407044966673,41.7874360373546,42.7849645717912,43.7824931062278,
44.7800216406644,45.777550175101,46.7750787095376,47.1238898038469),
 .UNSPECIFIED.);
#2201=B_SPLINE_CURVE_WITH_KNOTS('',3,(#16712,#16713,#16714,#16715,#16716,
#16717,#16718,#16719,#16720,#16721),.UNSPECIFIED.,.F.,.F.,(4,1,1,1,1,1,
1,4),(40.8407044966673,41.3314114425651,42.3289399770017,43.3264685114383,
44.3239970458749,45.3215255803115,46.3190541147481,47.1238898038469),
 .UNSPECIFIED.);
#2202=B_SPLINE_CURVE_WITH_KNOTS('',3,(#16726,#16727,#16728,#16729,#16730,
#16731,#16732,#16733,#16734,#16735,#16736),.UNSPECIFIED.,.F.,.F.,(4,1,1,
1,1,1,1,1,4),(34.5575191894876,34.8047362962984,35.802264830735,36.7997933651716,
37.7973218996082,38.7948504340448,39.7923789684814,40.789907502918,40.8407044966673),
 .UNSPECIFIED.);
#2203=B_SPLINE_CURVE_WITH_KNOTS('',3,(#16737,#16738,#16739,#16740,#16741,
#16742,#16743,#16744,#16745,#16746),.UNSPECIFIED.,.F.,.F.,(4,1,1,1,1,1,
1,4),(34.5575191894876,35.3462402359455,36.3437687703821,37.3412973048187,
38.3388258392553,39.3363543736919,40.3338829081285,40.8407044966673),
 .UNSPECIFIED.);
#2204=B_SPLINE_CURVE_WITH_KNOTS('',3,(#16751,#16752,#16753,#16754,#16755,
#16756,#16757,#16758,#16759,#16760),.UNSPECIFIED.,.F.,.F.,(4,1,1,1,1,1,
1,4),(28.2743338823081,28.8195650896788,29.8170936241154,30.814622158552,
31.8121506929886,32.8096792274252,33.8072077618618,34.5575191894876),
 .UNSPECIFIED.);
#2205=B_SPLINE_CURVE_WITH_KNOTS('',3,(#16761,#16762,#16763,#16764,#16765,
#16766,#16767,#16768,#16769,#16770,#16771),.UNSPECIFIED.,.F.,.F.,(4,1,1,
1,1,1,1,1,4),(28.2743338823081,28.3635404948893,29.3610690293259,30.3585975637625,
31.3561260981991,32.3536546326357,33.3511831670723,34.3487117015089,34.5575191894876),
 .UNSPECIFIED.);
#2206=B_SPLINE_CURVE_WITH_KNOTS('',3,(#16776,#16777,#16778,#16779,#16780,
#16781,#16782,#16783,#16784,#16785),.UNSPECIFIED.,.F.,.F.,(4,1,1,1,1,1,
1,4),(21.9911485751285,22.8343938830592,23.8319224174958,24.8294509519324,
25.826979486369,26.8245080208056,27.8220365552422,28.2743338823081),
 .UNSPECIFIED.);
#2207=B_SPLINE_CURVE_WITH_KNOTS('',3,(#16786,#16787,#16788,#16789,#16790,
#16791,#16792,#16793,#16794,#16795),.UNSPECIFIED.,.F.,.F.,(4,1,1,1,1,1,
1,4),(21.9911485751285,22.3783692882697,23.3758978227063,24.3734263571429,
25.3709548915795,26.3684834260161,27.3660119604527,28.2743338823081),
 .UNSPECIFIED.);
#2208=B_SPLINE_CURVE_WITH_KNOTS('',3,(#16801,#16802,#16803,#16804,#16805),
 .UNSPECIFIED.,.F.,.F.,(4,1,4),(14.3981410127769,15.3956695472135,15.7079632679489),
 .UNSPECIFIED.);
#2209=B_SPLINE_CURVE_WITH_KNOTS('',3,(#16808,#16809,#16810,#16811,#16812),
 .UNSPECIFIED.,.F.,.F.,(4,1,4),(13.8761928695311,14.8541656075664,15.7079632679489),
 .UNSPECIFIED.);
#2210=B_SPLINE_CURVE_WITH_KNOTS('',3,(#16818,#16819,#16820,#16821,#16822,
#16823,#16824,#16825,#16826,#16827,#16828,#16829,#16830,#16831,#16832,#16833,
#16834,#16835,#16836),.UNSPECIFIED.,.F.,.F.,(4,3,3,3,3,3,4),(95.5576018628658,
95.7627393059136,96.7602678403502,97.7577963747868,98.7553249092234,99.75285344366,
100.750381978097),.UNSPECIFIED.);
#2211=B_SPLINE_CURVE_WITH_KNOTS('',3,(#16840,#16841,#16842,#16843),
 .UNSPECIFIED.,.F.,.F.,(4,4),(-98.7357691128221,-98.0941628713862),
 .UNSPECIFIED.);
#2212=B_SPLINE_CURVE_WITH_KNOTS('',3,(#16847,#16848,#16849,#16850,#16851,
#16852,#16853,#16854,#16855,#16856,#16857,#16858,#16859,#16860,#16861,#16862,
#16863,#16864,#16865,#16866,#16867,#16868),.UNSPECIFIED.,.F.,.F.,(4,3,3,
3,3,3,3,4),(-98.0941628713862,-97.7577963747868,-96.7602678403502,-95.7627393059136,
-94.765210771477,-93.7676822370404,-92.7701537026038,-91.8109775642066),
 .UNSPECIFIED.);
#2213=B_SPLINE_CURVE_WITH_KNOTS('',3,(#16873,#16874,#16875,#16876,#16877,
#16878,#16879,#16880,#16881,#16882,#16883,#16884,#16885,#16886,#16887,#16888,
#16889,#16890,#16891,#16892,#16893,#16894),.UNSPECIFIED.,.F.,.F.,(4,3,3,
3,3,3,3,4),(89.2744165556863,89.777568099294,90.7750966337306,91.7726251681672,
92.7701537026038,93.7676822370404,94.765210771477,95.5576018628658),
 .UNSPECIFIED.);
#2214=B_SPLINE_CURVE_WITH_KNOTS('',3,(#16895,#16896,#16897,#16898,#16899,
#16900,#16901,#16902,#16903,#16904,#16905,#16906,#16907,#16908,#16909,#16910,
#16911,#16912,#16913,#16914,#16915,#16916,#16917,#16918,#16919),
 .UNSPECIFIED.,.F.,.F.,(4,3,3,3,3,3,3,3,4),(-91.8109775642066,-91.7726251681672,
-90.7750966337306,-89.777568099294,-88.7800395648574,-87.7825110304208,
-86.7849824959842,-85.7874539615476,-85.527792257027),.UNSPECIFIED.);
#2215=B_SPLINE_CURVE_WITH_KNOTS('',3,(#16924,#16925,#16926,#16927,#16928,
#16929,#16930,#16931,#16932,#16933,#16934,#16935,#16936,#16937,#16938,#16939,
#16940,#16941,#16942,#16943,#16944,#16945),.UNSPECIFIED.,.F.,.F.,(4,3,3,
3,3,3,3,4),(82.9912312485067,83.7923968926744,84.789925427111,85.7874539615476,
86.7849824959842,87.7825110304208,88.7800395648574,89.2744165556863),
 .UNSPECIFIED.);
#2216=B_SPLINE_CURVE_WITH_KNOTS('',3,(#16946,#16947,#16948,#16949,#16950,
#16951,#16952,#16953,#16954,#16955,#16956,#16957,#16958,#16959,#16960,#16961,
#16962,#16963,#16964,#16965,#16966,#16967),.UNSPECIFIED.,.F.,.F.,(4,3,3,
3,3,3,3,4),(-85.527792257027,-84.789925427111,-83.7923968926744,-82.7948683582378,
-81.7973398238012,-80.7998112893646,-79.802282754928,-79.2446069498474),
 .UNSPECIFIED.);
#2217=B_SPLINE_CURVE_WITH_KNOTS('',3,(#16972,#16973,#16974,#16975,#16976,
#16977,#16978,#16979,#16980,#16981,#16982,#16983,#16984,#16985,#16986,#16987,
#16988,#16989,#16990,#16991,#16992,#16993,#16994,#16995,#16996),
 .UNSPECIFIED.,.F.,.F.,(4,3,3,3,3,3,3,3,4),(76.7080459413271,76.8096971516182,
77.8072256860548,78.8047542204914,79.802282754928,80.7998112893646,81.7973398238012,
82.7948683582378,82.9912312485067),.UNSPECIFIED.);
#2218=B_SPLINE_CURVE_WITH_KNOTS('',3,(#16997,#16998,#16999,#17000,#17001,
#17002,#17003,#17004,#17005,#17006,#17007,#17008,#17009,#17010,#17011,#17012,
#17013,#17014,#17015,#17016,#17017,#17018),.UNSPECIFIED.,.F.,.F.,(4,3,3,
3,3,3,3,4),(-79.2446069498474,-78.8047542204914,-77.8072256860548,-76.8096971516182,
-75.8121686171816,-74.814640082745,-73.8171115483084,-72.9614216426678),
 .UNSPECIFIED.);
#2219=B_SPLINE_CURVE_WITH_KNOTS('',3,(#17023,#17024,#17025,#17026,#17027,
#17028,#17029,#17030,#17031,#17032,#17033,#17034,#17035,#17036,#17037,#17038,
#17039,#17040,#17041,#17042,#17043,#17044),.UNSPECIFIED.,.F.,.F.,(4,3,3,
3,3,3,3,4),(70.4248606341475,70.8245259449986,71.8220544794352,72.8195830138718,
73.8171115483084,74.814640082745,75.8121686171816,76.7080459413271),
 .UNSPECIFIED.);
#2220=B_SPLINE_CURVE_WITH_KNOTS('',3,(#17045,#17046,#17047,#17048,#17049,
#17050,#17051,#17052,#17053,#17054,#17055,#17056,#17057,#17058,#17059,#17060,
#17061,#17062,#17063,#17064,#17065,#17066,#17067,#17068,#17069),
 .UNSPECIFIED.,.F.,.F.,(4,3,3,3,3,3,3,3,4),(-72.9614216426678,-72.8195830138718,
-71.8220544794352,-70.8245259449986,-69.826997410562,-68.8294688761254,
-67.8319403416888,-66.8344118072522,-66.6782363354882),.UNSPECIFIED.);
#2221=B_SPLINE_CURVE_WITH_KNOTS('',3,(#17074,#17075,#17076,#17077,#17078,
#17079,#17080,#17081,#17082,#17083,#17084,#17085,#17086,#17087,#17088,#17089,
#17090,#17091,#17092,#17093,#17094,#17095),.UNSPECIFIED.,.F.,.F.,(4,3,3,
3,3,3,3,4),(64.1416753269679,64.839354738379,65.8368832728156,66.8344118072522,
67.8319403416888,68.8294688761254,69.826997410562,70.4248606341475),
 .UNSPECIFIED.);
#2222=B_SPLINE_CURVE_WITH_KNOTS('',3,(#17096,#17097,#17098,#17099,#17100,
#17101,#17102,#17103,#17104,#17105,#17106,#17107,#17108,#17109,#17110,#17111,
#17112,#17113,#17114,#17115,#17116,#17117),.UNSPECIFIED.,.F.,.F.,(4,3,3,
3,3,3,3,4),(-66.6782363354882,-65.8368832728156,-64.839354738379,-63.8418262039424,
-62.8442976695058,-61.8467691350692,-60.8492406006326,-60.3950510283086),
 .UNSPECIFIED.);
#2223=B_SPLINE_CURVE_WITH_KNOTS('',3,(#17122,#17123,#17124,#17125,#17126,
#17127,#17128,#17129,#17130,#17131,#17132,#17133,#17134,#17135,#17136,#17137,
#17138,#17139,#17140,#17141,#17142,#17143),.UNSPECIFIED.,.F.,.F.,(4,3,3,
3,3,3,3,4),(57.8584900197883,58.8541835317594,59.851712066196,60.8492406006326,
61.8467691350692,62.8442976695058,63.8418262039424,64.1416753269679),
 .UNSPECIFIED.);
#2224=B_SPLINE_CURVE_WITH_KNOTS('',3,(#17144,#17145,#17146,#17147,#17148,
#17149,#17150,#17151,#17152,#17153,#17154,#17155,#17156,#17157,#17158,#17159,
#17160,#17161,#17162,#17163,#17164,#17165),.UNSPECIFIED.,.F.,.F.,(4,3,3,
3,3,3,3,4),(-60.3950510283086,-59.851712066196,-58.8541835317594,-57.8566549973228,
-56.8591264628862,-55.8615979284496,-54.864069394013,-54.111865721129),
 .UNSPECIFIED.);
#2225=B_SPLINE_CURVE_WITH_KNOTS('',3,(#17170,#17171,#17172,#17173,#17174,
#17175,#17176,#17177,#17178,#17179,#17180,#17181,#17182,#17183,#17184,#17185,
#17186,#17187,#17188,#17189,#17190,#17191),.UNSPECIFIED.,.F.,.F.,(4,3,3,
3,3,3,3,4),(51.5753047126087,51.8714837907032,52.8690123251398,53.8665408595764,
54.864069394013,55.8615979284496,56.8591264628862,57.8584900197883),
 .UNSPECIFIED.);
#2226=B_SPLINE_CURVE_WITH_KNOTS('',3,(#17192,#17193,#17194,#17195,#17196,
#17197,#17198,#17199,#17200,#17201,#17202,#17203,#17204,#17205,#17206,#17207,
#17208,#17209,#17210,#17211,#17212,#17213,#17214,#17215,#17216),
 .UNSPECIFIED.,.F.,.F.,(4,3,3,3,3,3,3,3,4),(-54.111865721129,-53.8665408595764,
-52.8690123251398,-51.8714837907032,-50.8739552562666,-49.87642672183,-48.8788981873934,
-47.8813696529568,-47.8286804139494),.UNSPECIFIED.);
#2227=B_SPLINE_CURVE_WITH_KNOTS('',3,(#17221,#17222,#17223,#17224,#17225,
#17226,#17227,#17228,#17229,#17230,#17231,#17232,#17233,#17234,#17235,#17236,
#17237,#17238,#17239,#17240,#17241,#17242),.UNSPECIFIED.,.F.,.F.,(4,3,3,
3,3,3,3,4),(45.2921194054291,45.8863125840836,46.8838411185202,47.8813696529568,
48.8788981873934,49.87642672183,50.8739552562666,51.5753047126087),
 .UNSPECIFIED.);
#2228=B_SPLINE_CURVE_WITH_KNOTS('',3,(#17243,#17244,#17245,#17246,#17247,
#17248,#17249,#17250,#17251,#17252,#17253,#17254,#17255,#17256,#17257,#17258,
#17259,#17260,#17261,#17262,#17263,#17264),.UNSPECIFIED.,.F.,.F.,(4,3,3,
3,3,3,3,4),(-47.8286804139494,-46.8838411185202,-45.8863125840836,-44.888784049647,
-43.8912555152104,-42.8937269807738,-41.8961984463372,-41.5454951067699),
 .UNSPECIFIED.);
#2229=B_SPLINE_CURVE_WITH_KNOTS('',3,(#17269,#17270,#17271,#17272,#17273,
#17274,#17275,#17276,#17277,#17278,#17279,#17280,#17281,#17282,#17283,#17284,
#17285,#17286,#17287,#17288,#17289,#17290),.UNSPECIFIED.,.F.,.F.,(4,3,3,
3,3,3,3,4),(39.0089340982495,39.901141377464,40.8986699119006,41.8961984463372,
42.8937269807738,43.8912555152104,44.888784049647,45.2921194054291),
 .UNSPECIFIED.);
#2230=B_SPLINE_CURVE_WITH_KNOTS('',3,(#17291,#17292,#17293,#17294,#17295,
#17296,#17297,#17298,#17299,#17300,#17301,#17302,#17303,#17304,#17305,#17306,
#17307,#17308,#17309,#17310,#17311,#17312),.UNSPECIFIED.,.F.,.F.,(4,3,3,
3,3,3,3,4),(-41.5454951067699,-40.8986699119006,-39.901141377464,-38.9036128430274,
-37.9060843085908,-36.9085557741542,-35.9110272397176,-35.2623097995902),
 .UNSPECIFIED.);
#2231=B_SPLINE_CURVE_WITH_KNOTS('',3,(#17317,#17318,#17319,#17320,#17321,
#17322,#17323,#17324,#17325,#17326,#17327,#17328,#17329,#17330,#17331,#17332,
#17333,#17334,#17335,#17336,#17337,#17338,#17339,#17340,#17341),
 .UNSPECIFIED.,.F.,.F.,(4,3,3,3,3,3,3,3,4),(32.7257487910699,32.9184416364078,
33.9159701708444,34.913498705281,35.9110272397176,36.9085557741542,37.9060843085908,
38.9036128430274,39.0089340982495),.UNSPECIFIED.);
#2232=B_SPLINE_CURVE_WITH_KNOTS('',3,(#17342,#17343,#17344,#17345,#17346,
#17347,#17348,#17349,#17350,#17351,#17352,#17353,#17354,#17355,#17356,#17357,
#17358,#17359,#17360,#17361,#17362,#17363),.UNSPECIFIED.,.F.,.F.,(4,3,3,
3,3,3,3,4),(-35.2623097995902,-34.913498705281,-33.9159701708444,-32.9184416364078,
-31.9209131019712,-30.9233845675346,-29.925856033098,-28.9791244924107),
 .UNSPECIFIED.);
#2233=B_SPLINE_CURVE_WITH_KNOTS('',3,(#17368,#17369,#17370,#17371,#17372,
#17373,#17374,#17375,#17376,#17377,#17378,#17379,#17380,#17381,#17382,#17383,
#17384,#17385,#17386,#17387,#17388,#17389),.UNSPECIFIED.,.F.,.F.,(4,3,3,
3,3,3,3,4),(26.4425634838903,26.9332704297882,27.9307989642248,28.9283274986614,
29.925856033098,30.9233845675346,31.9209131019712,32.7257487910699),
 .UNSPECIFIED.);
#2234=B_SPLINE_CURVE_WITH_KNOTS('',3,(#17390,#17391,#17392,#17393,#17394,
#17395,#17396,#17397,#17398,#17399,#17400,#17401,#17402,#17403,#17404,#17405,
#17406,#17407,#17408,#17409,#17410,#17411,#17412,#17413,#17414),
 .UNSPECIFIED.,.F.,.F.,(4,3,3,3,3,3,3,3,4),(-28.9791244924107,-28.9283274986614,
-27.9307989642248,-26.9332704297882,-25.9357418953516,-24.938213360915,
-23.9406848264784,-22.9431562920418,-22.6959391852311),.UNSPECIFIED.);
#2235=B_SPLINE_CURVE_WITH_KNOTS('',3,(#17419,#17420,#17421,#17422,#17423,
#17424,#17425,#17426,#17427,#17428,#17429,#17430,#17431,#17432,#17433,#17434,
#17435,#17436,#17437,#17438,#17439,#17440),.UNSPECIFIED.,.F.,.F.,(4,3,3,
3,3,3,3,4),(20.1593781767108,20.9480992231686,21.9456277576052,22.9431562920418,
23.9406848264784,24.938213360915,25.9357418953516,26.4425634838903),
 .UNSPECIFIED.);
#2236=B_SPLINE_CURVE_WITH_KNOTS('',3,(#17441,#17442,#17443,#17444,#17445,
#17446,#17447,#17448,#17449,#17450,#17451,#17452,#17453,#17454,#17455,#17456,
#17457,#17458,#17459,#17460,#17461,#17462),.UNSPECIFIED.,.F.,.F.,(4,3,3,
3,3,3,3,4),(-22.6959391852311,-21.9456277576052,-20.9480992231686,-19.950570688732,
-18.9530421542954,-17.9555136198588,-16.9579850854222,-16.4127538780515),
 .UNSPECIFIED.);
#2237=B_SPLINE_CURVE_WITH_KNOTS('',3,(#17467,#17468,#17469,#17470,#17471,
#17472,#17473,#17474,#17475,#17476,#17477,#17478,#17479,#17480,#17481,#17482,
#17483,#17484,#17485,#17486,#17487,#17488,#17489,#17490,#17491),
 .UNSPECIFIED.,.F.,.F.,(4,3,3,3,3,3,3,3,4),(13.8761928695312,13.9653994821124,
14.962928016549,15.9604565509856,16.9579850854222,17.9555136198588,18.9530421542954,
19.950570688732,20.1593781767108),.UNSPECIFIED.);
#2238=B_SPLINE_CURVE_WITH_KNOTS('',3,(#17492,#17493,#17494,#17495,#17496,
#17497,#17498,#17499,#17500,#17501,#17502,#17503,#17504,#17505,#17506,#17507,
#17508,#17509,#17510,#17511,#17512,#17513),.UNSPECIFIED.,.F.,.F.,(4,3,3,
3,3,3,3,4),(-16.4127538780515,-15.9604565509856,-14.962928016549,-13.9653994821124,
-12.9678709476758,-11.9703424132392,-10.9728138788026,-10.1295685708719),
 .UNSPECIFIED.);
#2239=B_SPLINE_CURVE_WITH_KNOTS('',3,(#17519,#17520,#17521,#17522,#17523,
#17524,#17525,#17526,#17527,#17528,#17529,#17530,#17531),.UNSPECIFIED.,
 .F.,.F.,(4,3,3,3,4),(-3.84638326369234,-2.99258560330979,-1.9950570688732,
-0.997528534436597,0.),.UNSPECIFIED.);
#2240=B_SPLINE_CURVE_WITH_KNOTS('',3,(#17534,#17535,#17536,#17537,#17538,
#17539,#17540,#17541,#17542,#17543,#17544,#17545,#17546,#17547,#17548,#17549,
#17550,#17551,#17552),.UNSPECIFIED.,.F.,.F.,(4,3,3,3,3,3,4),(2.01461286527445,
2.9925856033098,3.9901141377464,4.987642672183,5.9851712066196,6.98269974105621,
7.59300756235157),.UNSPECIFIED.);
#2241=B_SPLINE_CURVE_WITH_KNOTS('',3,(#17558,#17559,#17560,#17561,#17562,
#17563),.UNSPECIFIED.,.F.,.F.,(4,1,1,4),(109.955742875643,110.61690491348,
111.614433447917,112.611961982353),.UNSPECIFIED.);
#2242=B_SPLINE_CURVE_WITH_KNOTS('',3,(#17566,#17567,#17568,#17569,#17570,
#17571,#17572),.UNSPECIFIED.,.F.,.F.,(4,1,1,1,4),(109.955742875643,110.16088031869,
111.158408853127,112.155937387564,113.133910125599),.UNSPECIFIED.);
#2243=B_SPLINE_CURVE_WITH_KNOTS('',3,(#17577,#17578,#17579,#17580,#17581,
#17582,#17583,#17584,#17585,#17586),.UNSPECIFIED.,.F.,.F.,(4,1,1,1,1,1,
1,4),(103.672557568463,104.63173370686,105.629262241297,106.626790775734,
107.62431931017,108.621847844607,109.619376379043,109.955742875643),
 .UNSPECIFIED.);
#2244=B_SPLINE_CURVE_WITH_KNOTS('',3,(#17587,#17588,#17589,#17590,#17591,
#17592,#17593,#17594,#17595,#17596),.UNSPECIFIED.,.F.,.F.,(4,1,1,1,1,1,
1,4),(103.672557568463,104.175709112071,105.173237646507,106.170766180944,
107.168294715381,108.165823249817,109.163351784254,109.955742875643),
 .UNSPECIFIED.);
#2245=B_SPLINE_CURVE_WITH_KNOTS('',3,(#17601,#17602,#17603,#17604,#17605,
#17606,#17607,#17608,#17609,#17610,#17611),.UNSPECIFIED.,.F.,.F.,(4,1,1,
1,1,1,1,1,4),(97.3893722612835,97.6490339658041,98.6465625002407,99.6440910346773,
100.641619569114,101.639148103551,102.636676637987,103.634205172424,103.672557568463),
 .UNSPECIFIED.);
#2246=B_SPLINE_CURVE_WITH_KNOTS('',3,(#17612,#17613,#17614,#17615,#17616,
#17617,#17618,#17619,#17620,#17621),.UNSPECIFIED.,.F.,.F.,(4,1,1,1,1,1,
1,4),(97.3893722612835,98.1905379054512,99.1880664398878,100.185594974324,
101.183123508761,102.180652043198,103.178180577634,103.672557568463),
 .UNSPECIFIED.);
#2247=B_SPLINE_CURVE_WITH_KNOTS('',3,(#17626,#17627,#17628,#17629,#17630,
#17631,#17632,#17633,#17634,#17635),.UNSPECIFIED.,.F.,.F.,(4,1,1,1,1,1,
1,4),(91.106186954104,91.6638627591845,92.6613912936211,93.6589198280577,
94.6564483624943,95.6539768969309,96.6515054313675,97.3893722612835),
 .UNSPECIFIED.);
#2248=B_SPLINE_CURVE_WITH_KNOTS('',3,(#17636,#17637,#17638,#17639,#17640,
#17641,#17642,#17643,#17644,#17645,#17646),.UNSPECIFIED.,.F.,.F.,(4,1,1,
1,1,1,1,1,4),(91.106186954104,91.207838164395,92.2053666988316,93.2028952332682,
94.2004237677048,95.1979523021414,96.195480836578,97.1930093710146,97.3893722612835),
 .UNSPECIFIED.);
#2249=B_SPLINE_CURVE_WITH_KNOTS('',3,(#17651,#17652,#17653,#17654,#17655,
#17656,#17657,#17658,#17659,#17660),.UNSPECIFIED.,.F.,.F.,(4,1,1,1,1,1,
1,4),(84.8230016469244,85.6786915525649,86.6762200870015,87.6737486214381,
88.6712771558747,89.6688056903113,90.6663342247479,91.106186954104),
 .UNSPECIFIED.);
#2250=B_SPLINE_CURVE_WITH_KNOTS('',3,(#17661,#17662,#17663,#17664,#17665,
#17666,#17667,#17668,#17669,#17670),.UNSPECIFIED.,.F.,.F.,(4,1,1,1,1,1,
1,4),(84.8230016469244,85.2226669577754,86.220195492212,87.2177240266486,
88.2152525610852,89.2127810955218,90.2103096299584,91.106186954104),
 .UNSPECIFIED.);
#2251=B_SPLINE_CURVE_WITH_KNOTS('',3,(#17675,#17676,#17677,#17678,#17679,
#17680,#17681,#17682,#17683,#17684,#17685),.UNSPECIFIED.,.F.,.F.,(4,1,1,
1,1,1,1,1,4),(78.5398163397448,78.6959918115087,79.6935203459453,80.6910488803819,
81.6885774148185,82.6861059492551,83.6836344836917,84.6811630181283,84.8230016469244),
 .UNSPECIFIED.);
#2252=B_SPLINE_CURVE_WITH_KNOTS('',3,(#17686,#17687,#17688,#17689,#17690,
#17691,#17692,#17693,#17694,#17695),.UNSPECIFIED.,.F.,.F.,(4,1,1,1,1,1,
1,4),(78.5398163397448,79.2374957511558,80.2350242855924,81.232552820029,
82.2300813544656,83.2276098889022,84.2251384233388,84.8230016469244),
 .UNSPECIFIED.);
#2253=B_SPLINE_CURVE_WITH_KNOTS('',3,(#17700,#17701,#17702,#17703,#17704,
#17705,#17706,#17707,#17708,#17709),.UNSPECIFIED.,.F.,.F.,(4,1,1,1,1,1,
1,4),(72.2566310325652,72.7108206048891,73.7083491393257,74.7058776737623,
75.7034062081989,76.7009347426355,77.6984632770721,78.5398163397448),
 .UNSPECIFIED.);
#2254=B_SPLINE_CURVE_WITH_KNOTS('',3,(#17710,#17711,#17712,#17713,#17714,
#17715,#17716,#17717,#17718,#17719),.UNSPECIFIED.,.F.,.F.,(4,1,1,1,1,1,
1,4),(72.2566310325652,73.2523245445362,74.2498530789728,75.2473816134094,
76.244910147846,77.2424386822826,78.2399672167192,78.5398163397448),
 .UNSPECIFIED.);
#2255=B_SPLINE_CURVE_WITH_KNOTS('',3,(#17724,#17725,#17726,#17727,#17728,
#17729,#17730,#17731,#17732,#17733),.UNSPECIFIED.,.F.,.F.,(4,1,1,1,1,1,
1,4),(65.9734457253856,66.7256493982695,67.7231779327061,68.7207064671427,
69.7182350015793,70.7157635360159,71.7132920704525,72.2566310325652),
 .UNSPECIFIED.);
#2256=B_SPLINE_CURVE_WITH_KNOTS('',3,(#17734,#17735,#17736,#17737,#17738,
#17739,#17740,#17741,#17742,#17743,#17744),.UNSPECIFIED.,.F.,.F.,(4,1,1,
1,1,1,1,1,4),(65.9734457253856,66.26962480348,67.2671533379166,68.2646818723532,
69.2622104067898,70.2597389412264,71.257267475663,72.2547960100996,72.2566310325652),
 .UNSPECIFIED.);
#2257=B_SPLINE_CURVE_WITH_KNOTS('',3,(#17749,#17750,#17751,#17752,#17753,
#17754,#17755,#17756,#17757,#17758,#17759),.UNSPECIFIED.,.F.,.F.,(4,1,1,
1,1,1,1,1,4),(59.690260418206,59.7429496572133,60.7404781916499,61.7380067260865,
62.7355352605231,63.7330637949597,64.7305923293963,65.7281208638329,65.9734457253856),
 .UNSPECIFIED.);
#2258=B_SPLINE_CURVE_WITH_KNOTS('',3,(#17760,#17761,#17762,#17763,#17764,
#17765,#17766,#17767,#17768,#17769),.UNSPECIFIED.,.F.,.F.,(4,1,1,1,1,1,
1,4),(59.690260418206,60.2844535968604,61.281982131297,62.2795106657336,
63.2770392001702,64.2745677346068,65.2720962690434,65.9734457253856),
 .UNSPECIFIED.);
#2259=B_SPLINE_CURVE_WITH_KNOTS('',3,(#17774,#17775,#17776,#17777,#17778,
#17779,#17780,#17781,#17782,#17783),.UNSPECIFIED.,.F.,.F.,(4,1,1,1,1,1,
1,4),(53.4070751110264,53.7577784505937,54.7553069850303,55.7528355194669,
56.7503640539035,57.7478925883401,58.7454211227767,59.690260418206),
 .UNSPECIFIED.);
#2260=B_SPLINE_CURVE_WITH_KNOTS('',3,(#17784,#17785,#17786,#17787,#17788,
#17789,#17790,#17791,#17792,#17793),.UNSPECIFIED.,.F.,.F.,(4,1,1,1,1,1,
1,4),(53.4070751110264,54.2992823902408,55.2968109246774,56.294339459114,
57.2918679935506,58.2893965279872,59.2869250624238,59.690260418206),
 .UNSPECIFIED.);
#2261=B_SPLINE_CURVE_WITH_KNOTS('',3,(#17798,#17799,#17800,#17801,#17802,
#17803,#17804,#17805,#17806,#17807),.UNSPECIFIED.,.F.,.F.,(4,1,1,1,1,1,
1,4),(47.1238898038468,47.7726072439741,48.7701357784107,49.7676643128473,
50.7651928472839,51.7627213817205,52.7602499161571,53.4070751110264),
 .UNSPECIFIED.);
#2262=B_SPLINE_CURVE_WITH_KNOTS('',3,(#17808,#17809,#17810,#17811,#17812,
#17813,#17814,#17815,#17816,#17817,#17818),.UNSPECIFIED.,.F.,.F.,(4,1,1,
1,1,1,1,1,4),(47.1238898038468,47.3165826491846,48.3141111836212,49.3116397180578,
50.3091682524944,51.306696786931,52.3042253213676,53.3017538558042,53.4070751110264),
 .UNSPECIFIED.);
#2263=B_SPLINE_CURVE_WITH_KNOTS('',3,(#17823,#17824,#17825,#17826,#17827,
#17828,#17829,#17830,#17831,#17832),.UNSPECIFIED.,.F.,.F.,(4,1,1,1,1,1,
1,4),(40.8407044966673,41.7874360373545,42.7849645717911,43.7824931062277,
44.7800216406643,45.7775501751009,46.7750787095375,47.1238898038468),
 .UNSPECIFIED.);
#2264=B_SPLINE_CURVE_WITH_KNOTS('',3,(#17833,#17834,#17835,#17836,#17837,
#17838,#17839,#17840,#17841,#17842),.UNSPECIFIED.,.F.,.F.,(4,1,1,1,1,1,
1,4),(40.8407044966673,41.331411442565,42.3289399770016,43.3264685114382,
44.3239970458748,45.3215255803114,46.319054114748,47.1238898038468),
 .UNSPECIFIED.);
#2265=B_SPLINE_CURVE_WITH_KNOTS('',3,(#17847,#17848,#17849,#17850,#17851,
#17852,#17853,#17854,#17855,#17856,#17857),.UNSPECIFIED.,.F.,.F.,(4,1,1,
1,1,1,1,1,4),(34.5575191894877,34.8047362962984,35.8022648307349,36.7997933651715,
37.7973218996081,38.7948504340447,39.7923789684813,40.7899075029179,40.8407044966673),
 .UNSPECIFIED.);
#2266=B_SPLINE_CURVE_WITH_KNOTS('',3,(#17858,#17859,#17860,#17861,#17862,
#17863,#17864,#17865,#17866,#17867),.UNSPECIFIED.,.F.,.F.,(4,1,1,1,1,1,
1,4),(34.5575191894876,35.3462402359454,36.343768770382,37.3412973048186,
38.3388258392552,39.3363543736918,40.3338829081284,40.8407044966673),
 .UNSPECIFIED.);
#2267=B_SPLINE_CURVE_WITH_KNOTS('',3,(#17872,#17873,#17874,#17875,#17876,
#17877,#17878,#17879,#17880,#17881),.UNSPECIFIED.,.F.,.F.,(4,1,1,1,1,1,
1,4),(28.2743338823081,28.8195650896787,29.8170936241154,30.8146221585519,
31.8121506929885,32.8096792274251,33.8072077618617,34.5575191894877),
 .UNSPECIFIED.);
#2268=B_SPLINE_CURVE_WITH_KNOTS('',3,(#17882,#17883,#17884,#17885,#17886,
#17887,#17888,#17889,#17890,#17891,#17892),.UNSPECIFIED.,.F.,.F.,(4,1,1,
1,1,1,1,1,4),(28.2743338823081,28.3635404948892,29.3610690293258,30.3585975637624,
31.356126098199,32.3536546326356,33.3511831670722,34.3487117015088,34.5575191894876),
 .UNSPECIFIED.);
#2269=B_SPLINE_CURVE_WITH_KNOTS('',3,(#17897,#17898,#17899,#17900,#17901,
#17902,#17903,#17904,#17905,#17906),.UNSPECIFIED.,.F.,.F.,(4,1,1,1,1,1,
1,4),(21.9911485751285,22.8343938830591,23.8319224174958,24.8294509519324,
25.8269794863689,26.8245080208056,27.8220365552421,28.2743338823081),
 .UNSPECIFIED.);
#2270=B_SPLINE_CURVE_WITH_KNOTS('',3,(#17907,#17908,#17909,#17910,#17911,
#17912,#17913,#17914,#17915,#17916),.UNSPECIFIED.,.F.,.F.,(4,1,1,1,1,1,
1,4),(21.9911485751284,22.3783692882696,23.3758978227062,24.3734263571428,
25.3709548915794,26.368483426016,27.3660119604526,28.2743338823081),
 .UNSPECIFIED.);
#2271=B_SPLINE_CURVE_WITH_KNOTS('',3,(#17922,#17923,#17924,#17925,#17926),
 .UNSPECIFIED.,.F.,.F.,(4,1,4),(14.3981410127768,15.3956695472134,15.7079632679489),
 .UNSPECIFIED.);
#2272=B_SPLINE_CURVE_WITH_KNOTS('',3,(#17929,#17930,#17931,#17932,#17933),
 .UNSPECIFIED.,.F.,.F.,(4,1,4),(13.876192869531,14.8541656075664,15.7079632679489),
 .UNSPECIFIED.);
#2273=B_SPLINE_CURVE_WITH_KNOTS('',3,(#17939,#17940,#17941,#17942),
 .UNSPECIFIED.,.F.,.F.,(4,4),(95.5573427486709,96.2647245007222),
 .UNSPECIFIED.);
#2274=B_SPLINE_CURVE_WITH_KNOTS('',3,(#17946,#17947,#17948,#17949,#17950,
#17951,#17952,#17953,#17954,#17955,#17956,#17957,#17958,#17959,#17960,#17961,
#17962,#17963,#17964),.UNSPECIFIED.,.F.,.F.,(4,2,2,2,3,2,2,2,4),(1.16162179993387,
1.25828720239456,1.35495260485525,1.45189083571687,1.54882906657849,1.64576729744011,
1.74270552830173,1.83937093076242,1.93603633322311),.UNSPECIFIED.);
#2275=B_SPLINE_CURVE_WITH_KNOTS('',3,(#17967,#17968,#17969,#17970,#17971,
#17972,#17973,#17974,#17975,#17976),.UNSPECIFIED.,.F.,.F.,(4,3,3,4),(-94.2477796076938,
-93.2874649800814,-92.2950451398677,-91.8135687061554),.UNSPECIFIED.);
#2276=B_SPLINE_CURVE_WITH_KNOTS('',3,(#17981,#17982,#17983,#17984,#17985,
#17986,#17987,#17988,#17989,#17990,#17991,#17992,#17993,#17994,#17995,#17996,
#17997,#17998,#17999,#18000,#18001,#18002,#18003,#18004,#18005),
 .UNSPECIFIED.,.F.,.F.,(4,3,3,3,3,3,3,3,4),(89.2741574414913,89.3177856192268,
90.3102054594404,91.3026252996541,92.2950451398677,93.2874649800813,94.279884820295,
95.2723046605086,95.5573427486709),.UNSPECIFIED.);
#2277=B_SPLINE_CURVE_WITH_KNOTS('',3,(#18006,#18007,#18008,#18009,#18010,
#18011,#18012,#18013,#18014,#18015,#18016,#18017,#18018,#18019,#18020,#18021,
#18022,#18023,#18024,#18025,#18026,#18027),.UNSPECIFIED.,.F.,.F.,(4,3,3,
3,3,3,3,4),(-91.8135687061554,-91.3026252996541,-90.3102054594405,-89.3177856192269,
-88.3253657790132,-87.3329459387996,-86.340526098586,-85.5303833989758),
 .UNSPECIFIED.);
#2278=B_SPLINE_CURVE_WITH_KNOTS('',3,(#18032,#18033,#18034,#18035,#18036,
#18037,#18038,#18039,#18040,#18041,#18042,#18043,#18044,#18045,#18046,#18047,
#18048,#18049,#18050,#18051,#18052,#18053),.UNSPECIFIED.,.F.,.F.,(4,3,3,
3,3,3,3,4),(82.9909721343117,83.363266577945,84.3556864181587,85.3481062583723,
86.3405260985859,87.3329459387996,88.3253657790132,89.2741574414913),
 .UNSPECIFIED.);
#2279=B_SPLINE_CURVE_WITH_KNOTS('',3,(#18054,#18055,#18056,#18057,#18058,
#18059,#18060,#18061,#18062,#18063,#18064,#18065,#18066,#18067,#18068,#18069,
#18070,#18071,#18072,#18073,#18074,#18075,#18076,#18077,#18078),
 .UNSPECIFIED.,.F.,.F.,(4,3,3,3,3,3,3,3,4),(-85.5303833989758,-85.3481062583723,
-84.3556864181587,-83.3632665779451,-82.3708467377314,-81.3784268975178,
-80.3860070573042,-79.3935872170905,-79.2471980917962),.UNSPECIFIED.);
#2280=B_SPLINE_CURVE_WITH_KNOTS('',3,(#18083,#18084,#18085,#18086,#18087,
#18088,#18089,#18090,#18091,#18092,#18093,#18094,#18095,#18096,#18097,#18098,
#18099,#18100,#18101,#18102,#18103,#18104),.UNSPECIFIED.,.F.,.F.,(4,3,3,
3,3,3,3,4),(76.7077868271321,77.4087475366632,78.4011673768769,79.3935872170905,
80.3860070573041,81.3784268975178,82.3708467377314,82.9909721343117),
 .UNSPECIFIED.);
#2281=B_SPLINE_CURVE_WITH_KNOTS('',3,(#18105,#18106,#18107,#18108,#18109,
#18110,#18111,#18112,#18113,#18114,#18115,#18116,#18117,#18118,#18119,#18120,
#18121,#18122,#18123,#18124,#18125,#18126),.UNSPECIFIED.,.F.,.F.,(4,3,3,
3,3,3,3,4),(-79.2471980917962,-78.4011673768769,-77.4087475366633,-76.4163276964496,
-75.423907856236,-74.4314880160224,-73.4390681758088,-72.9640127846167),
 .UNSPECIFIED.);
#2282=B_SPLINE_CURVE_WITH_KNOTS('',3,(#18131,#18132,#18133,#18134,#18135,
#18136,#18137,#18138,#18139,#18140,#18141,#18142,#18143,#18144,#18145,#18146,
#18147,#18148,#18149,#18150,#18151,#18152,#18153,#18154,#18155),
 .UNSPECIFIED.,.F.,.F.,(4,3,3,3,3,3,3,3,4),(70.4246015199525,70.4618086551678,
71.4542284953814,72.4466483355951,73.4390681758087,74.4314880160223,75.423907856236,
76.4163276964496,76.7077868271321),.UNSPECIFIED.);
#2283=B_SPLINE_CURVE_WITH_KNOTS('',3,(#18156,#18157,#18158,#18159,#18160,
#18161,#18162,#18163,#18164,#18165,#18166,#18167,#18168,#18169,#18170,#18171,
#18172,#18173,#18174,#18175,#18176,#18177),.UNSPECIFIED.,.F.,.F.,(4,3,3,
3,3,3,3,4),(-72.9640127846167,-72.4466483355951,-71.4542284953815,-70.4618086551678,
-69.4693888149542,-68.4769689747406,-67.4845491345269,-66.680827477437),
 .UNSPECIFIED.);
#2284=B_SPLINE_CURVE_WITH_KNOTS('',3,(#18182,#18183,#18184,#18185,#18186,
#18187,#18188,#18189,#18190,#18191,#18192,#18193,#18194,#18195,#18196,#18197,
#18198,#18199,#18200,#18201,#18202,#18203),.UNSPECIFIED.,.F.,.F.,(4,3,3,
3,3,3,3,4),(64.1414162127729,64.507289613886,65.4997094540997,66.4921292943133,
67.4845491345269,68.4769689747405,69.4693888149542,70.4246015199525),
 .UNSPECIFIED.);
#2285=B_SPLINE_CURVE_WITH_KNOTS('',3,(#18204,#18205,#18206,#18207,#18208,
#18209,#18210,#18211,#18212,#18213,#18214,#18215,#18216,#18217,#18218,#18219,
#18220,#18221,#18222,#18223,#18224,#18225,#18226,#18227,#18228),
 .UNSPECIFIED.,.F.,.F.,(4,3,3,3,3,3,3,3,4),(-66.680827477437,-66.4921292943133,
-65.4997094540997,-64.5072896138861,-63.5148697736724,-62.5224499334588,
-61.5300300932452,-60.5376102530315,-60.3976421702575),.UNSPECIFIED.);
#2286=B_SPLINE_CURVE_WITH_KNOTS('',3,(#18233,#18234,#18235,#18236,#18237,
#18238,#18239,#18240,#18241,#18242,#18243,#18244,#18245,#18246,#18247,#18248,
#18249,#18250,#18251,#18252,#18253,#18254),.UNSPECIFIED.,.F.,.F.,(4,3,3,
3,3,3,3,4),(57.8582309055933,58.5527705726042,59.5451904128179,60.5376102530315,
61.5300300932451,62.5224499334588,63.5148697736724,64.1414162127729),
 .UNSPECIFIED.);
#2287=B_SPLINE_CURVE_WITH_KNOTS('',3,(#18255,#18256,#18257,#18258,#18259,
#18260,#18261,#18262,#18263,#18264,#18265,#18266,#18267,#18268,#18269,#18270,
#18271,#18272,#18273,#18274,#18275,#18276),.UNSPECIFIED.,.F.,.F.,(4,3,3,
3,3,3,3,4),(-60.3976421702575,-59.5451904128179,-58.5527705726043,-57.5603507323906,
-56.567930892177,-55.5755110519634,-54.5830912117497,-54.1144568630778),
 .UNSPECIFIED.);
#2288=B_SPLINE_CURVE_WITH_KNOTS('',3,(#18281,#18282,#18283,#18284,#18285,
#18286,#18287,#18288,#18289,#18290,#18291,#18292,#18293,#18294,#18295,#18296,
#18297,#18298,#18299,#18300,#18301,#18302,#18303,#18304,#18305),
 .UNSPECIFIED.,.F.,.F.,(4,3,3,3,3,3,3,3,4),(51.5750455984138,51.6058316911088,
52.5982515313225,53.5906713715361,54.5830912117497,55.5755110519634,56.567930892177,
57.5603507323906,57.8582309055933),.UNSPECIFIED.);
#2289=B_SPLINE_CURVE_WITH_KNOTS('',3,(#18306,#18307,#18308,#18309,#18310,
#18311,#18312,#18313,#18314,#18315,#18316,#18317,#18318,#18319,#18320,#18321,
#18322,#18323,#18324,#18325,#18326,#18327),.UNSPECIFIED.,.F.,.F.,(4,3,3,
3,3,3,3,4),(-54.1144568630778,-53.5906713715361,-52.5982515313225,-51.6058316911089,
-50.6134118508952,-49.6209920106816,-48.6285721704679,-47.8312715558983),
 .UNSPECIFIED.);
#2290=B_SPLINE_CURVE_WITH_KNOTS('',3,(#18332,#18333,#18334,#18335,#18336,
#18337,#18338,#18339,#18340,#18341,#18342,#18343,#18344,#18345,#18346,#18347,
#18348,#18349,#18350,#18351,#18352,#18353),.UNSPECIFIED.,.F.,.F.,(4,3,3,
3,3,3,3,4),(45.2918602912342,45.651312649827,46.6437324900407,47.6361523302543,
48.6285721704679,49.6209920106816,50.6134118508952,51.5750455984138),
 .UNSPECIFIED.);
#2291=B_SPLINE_CURVE_WITH_KNOTS('',3,(#18354,#18355,#18356,#18357,#18358,
#18359,#18360,#18361,#18362,#18363,#18364,#18365,#18366,#18367,#18368,#18369,
#18370,#18371,#18372,#18373,#18374,#18375,#18376,#18377,#18378),
 .UNSPECIFIED.,.F.,.F.,(4,3,3,3,3,3,3,3,4),(-47.8312715558983,-47.6361523302543,
-46.6437324900407,-45.651312649827,-44.6588928096134,-43.6664729693998,
-42.6740531291861,-41.6816332889725,-41.5480862487187),.UNSPECIFIED.);
#2292=B_SPLINE_CURVE_WITH_KNOTS('',3,(#18383,#18384,#18385,#18386,#18387,
#18388,#18389,#18390,#18391,#18392,#18393,#18394,#18395,#18396,#18397,#18398,
#18399,#18400,#18401,#18402,#18403,#18404),.UNSPECIFIED.,.F.,.F.,(4,3,3,
3,3,3,3,4),(39.0086749840546,39.6967936085453,40.6892134487589,41.6816332889725,
42.6740531291861,43.6664729693998,44.6588928096134,45.2918602912342),
 .UNSPECIFIED.);
#2293=B_SPLINE_CURVE_WITH_KNOTS('',3,(#18405,#18406,#18407,#18408,#18409,
#18410,#18411,#18412,#18413,#18414,#18415,#18416,#18417,#18418,#18419,#18420,
#18421,#18422,#18423,#18424,#18425,#18426),.UNSPECIFIED.,.F.,.F.,(4,3,3,
3,3,3,3,4),(-41.5480862487187,-40.6892134487589,-39.6967936085453,-38.7043737683316,
-37.711953928118,-36.7195340879044,-35.7271142476907,-35.2649009415391),
 .UNSPECIFIED.);
#2294=B_SPLINE_CURVE_WITH_KNOTS('',3,(#18431,#18432,#18433,#18434,#18435,
#18436,#18437,#18438,#18439,#18440,#18441,#18442,#18443,#18444,#18445,#18446,
#18447,#18448,#18449,#18450,#18451,#18452,#18453,#18454,#18455),
 .UNSPECIFIED.,.F.,.F.,(4,3,3,3,3,3,3,3,4),(32.725489676875,32.7498547270498,
33.7422745672635,34.7346944074771,35.7271142476907,36.7195340879043,37.711953928118,
38.7043737683316,39.0086749840546),.UNSPECIFIED.);
#2295=B_SPLINE_CURVE_WITH_KNOTS('',3,(#18456,#18457,#18458,#18459,#18460,
#18461,#18462,#18463,#18464,#18465,#18466,#18467,#18468,#18469,#18470,#18471,
#18472,#18473,#18474,#18475,#18476,#18477),.UNSPECIFIED.,.F.,.F.,(4,3,3,
3,3,3,3,4),(-35.2649009415391,-34.7346944074771,-33.7422745672635,-32.7498547270498,
-31.7574348868362,-30.7650150466226,-29.7725952064089,-28.9817156343595),
 .UNSPECIFIED.);
#2296=B_SPLINE_CURVE_WITH_KNOTS('',3,(#18482,#18483,#18484,#18485,#18486,
#18487,#18488,#18489,#18490,#18491,#18492,#18493,#18494,#18495,#18496,#18497,
#18498,#18499,#18500,#18501,#18502,#18503),.UNSPECIFIED.,.F.,.F.,(4,3,3,
3,3,3,3,4),(26.4423043696954,26.795335685768,27.7877555259817,28.7801753661953,
29.7725952064089,30.7650150466226,31.7574348868362,32.725489676875),
 .UNSPECIFIED.);
#2297=B_SPLINE_CURVE_WITH_KNOTS('',3,(#18504,#18505,#18506,#18507,#18508,
#18509,#18510,#18511,#18512,#18513,#18514,#18515,#18516,#18517,#18518,#18519,
#18520,#18521,#18522,#18523,#18524,#18525,#18526,#18527,#18528),
 .UNSPECIFIED.,.F.,.F.,(4,3,3,3,3,3,3,3,4),(-28.9817156343595,-28.7801753661953,
-27.7877555259817,-26.7953356857681,-25.8029158455544,-24.8104960053408,
-23.8180761651272,-22.8256563249135,-22.6985303271799),.UNSPECIFIED.);
#2298=B_SPLINE_CURVE_WITH_KNOTS('',3,(#18533,#18534,#18535,#18536,#18537,
#18538,#18539,#18540,#18541,#18542,#18543,#18544,#18545,#18546,#18547,#18548,
#18549,#18550,#18551,#18552,#18553,#18554),.UNSPECIFIED.,.F.,.F.,(4,3,3,
3,3,3,3,4),(20.1591190625158,20.8408166444862,21.8332364846999,22.8256563249135,
23.8180761651271,24.8104960053408,25.8029158455544,26.4423043696954),
 .UNSPECIFIED.);
#2299=B_SPLINE_CURVE_WITH_KNOTS('',3,(#18555,#18556,#18557,#18558,#18559,
#18560,#18561,#18562,#18563,#18564,#18565,#18566,#18567,#18568,#18569,#18570,
#18571,#18572,#18573,#18574,#18575,#18576),.UNSPECIFIED.,.F.,.F.,(4,3,3,
3,3,3,3,4),(-22.6985303271799,-21.8332364846999,-20.8408166444863,-19.8483968042726,
-18.855976964059,-17.8635571238454,-16.8711372836317,-16.4153450200003),
 .UNSPECIFIED.);
#2300=B_SPLINE_CURVE_WITH_KNOTS('',3,(#18581,#18582,#18583,#18584,#18585,
#18586,#18587,#18588,#18589,#18590,#18591,#18592,#18593,#18594,#18595,#18596,
#18597,#18598,#18599,#18600,#18601,#18602,#18603,#18604,#18605),
 .UNSPECIFIED.,.F.,.F.,(4,3,3,3,3,3,3,3,4),(13.8759337553362,13.8938777629908,
14.8862976032045,15.8787174434181,16.8711372836317,17.8635571238454,18.855976964059,
19.8483968042726,20.1591190625158),.UNSPECIFIED.);
#2301=B_SPLINE_CURVE_WITH_KNOTS('',3,(#18606,#18607,#18608,#18609,#18610,
#18611,#18612,#18613,#18614,#18615,#18616,#18617,#18618,#18619,#18620,#18621,
#18622,#18623,#18624,#18625,#18626,#18627),.UNSPECIFIED.,.F.,.F.,(4,3,3,
3,3,3,3,4),(-16.4153450200003,-15.8787174434181,-14.8862976032045,-13.8938777629908,
-12.9014579227772,-11.9090380825636,-10.9166182423499,-10.1321597128207),
 .UNSPECIFIED.);
#2302=B_SPLINE_CURVE_WITH_KNOTS('',3,(#18633,#18634,#18635,#18636,#18637,
#18638,#18639,#18640,#18641,#18642,#18643,#18644,#18645),.UNSPECIFIED.,
 .F.,.F.,(4,3,3,3,4),(-3.84897440564114,-2.9772595206409,-1.98483968042726,
-0.992419840213632,0.),.UNSPECIFIED.);
#2303=B_SPLINE_CURVE_WITH_KNOTS('',3,(#18648,#18649,#18650,#18651,#18652,
#18653,#18654,#18655,#18656,#18657,#18658,#18659,#18660,#18661,#18662,#18663,
#18664,#18665,#18666),.UNSPECIFIED.,.F.,.F.,(4,3,3,3,3,3,4),(2.01694489302841,
2.97725952064089,3.96967936085453,4.96209920106816,5.95451904128179,6.94693888149542,
7.59274844815661),.UNSPECIFIED.);
#2304=B_SPLINE_CURVE_WITH_KNOTS('',3,(#18672,#18673,#18674,#18675),
 .UNSPECIFIED.,.F.,.F.,(4,4),(95.5573427486709,96.2647245007222),
 .UNSPECIFIED.);
#2305=B_SPLINE_CURVE_WITH_KNOTS('',3,(#18679,#18680,#18681,#18682,#18683,
#18684,#18685,#18686,#18687,#18688,#18689,#18690,#18691,#18692,#18693,#18694,
#18695,#18696,#18697),.UNSPECIFIED.,.F.,.F.,(4,2,2,2,3,2,2,2,4),(1.16162179993387,
1.25828720239456,1.35495260485525,1.45189083571687,1.54882906657849,1.64576729744011,
1.74270552830173,1.83937093076242,1.93603633322311),.UNSPECIFIED.);
#2306=B_SPLINE_CURVE_WITH_KNOTS('',3,(#18700,#18701,#18702,#18703,#18704,
#18705,#18706,#18707,#18708,#18709),.UNSPECIFIED.,.F.,.F.,(4,3,3,4),(-94.2477796076938,
-93.2874649800814,-92.2950451398677,-91.8135687061554),.UNSPECIFIED.);
#2307=B_SPLINE_CURVE_WITH_KNOTS('',3,(#18714,#18715,#18716,#18717,#18718,
#18719,#18720,#18721,#18722,#18723,#18724,#18725,#18726,#18727,#18728,#18729,
#18730,#18731,#18732,#18733,#18734,#18735,#18736,#18737,#18738),
 .UNSPECIFIED.,.F.,.F.,(4,3,3,3,3,3,3,3,4),(89.2741574414913,89.3177856192268,
90.3102054594404,91.3026252996541,92.2950451398677,93.2874649800813,94.279884820295,
95.2723046605086,95.5573427486709),.UNSPECIFIED.);
#2308=B_SPLINE_CURVE_WITH_KNOTS('',3,(#18739,#18740,#18741,#18742,#18743,
#18744,#18745,#18746,#18747,#18748,#18749,#18750,#18751,#18752,#18753,#18754,
#18755,#18756,#18757,#18758,#18759,#18760),.UNSPECIFIED.,.F.,.F.,(4,3,3,
3,3,3,3,4),(-91.8135687061554,-91.3026252996541,-90.3102054594405,-89.3177856192269,
-88.3253657790132,-87.3329459387996,-86.340526098586,-85.5303833989758),
 .UNSPECIFIED.);
#2309=B_SPLINE_CURVE_WITH_KNOTS('',3,(#18765,#18766,#18767,#18768,#18769,
#18770,#18771,#18772,#18773,#18774,#18775,#18776,#18777,#18778,#18779,#18780,
#18781,#18782,#18783,#18784,#18785,#18786),.UNSPECIFIED.,.F.,.F.,(4,3,3,
3,3,3,3,4),(82.9909721343117,83.363266577945,84.3556864181587,85.3481062583723,
86.3405260985859,87.3329459387996,88.3253657790132,89.2741574414913),
 .UNSPECIFIED.);
#2310=B_SPLINE_CURVE_WITH_KNOTS('',3,(#18787,#18788,#18789,#18790,#18791,
#18792,#18793,#18794,#18795,#18796,#18797,#18798,#18799,#18800,#18801,#18802,
#18803,#18804,#18805,#18806,#18807,#18808,#18809,#18810,#18811),
 .UNSPECIFIED.,.F.,.F.,(4,3,3,3,3,3,3,3,4),(-85.5303833989758,-85.3481062583723,
-84.3556864181587,-83.3632665779451,-82.3708467377314,-81.3784268975178,
-80.3860070573042,-79.3935872170905,-79.2471980917962),.UNSPECIFIED.);
#2311=B_SPLINE_CURVE_WITH_KNOTS('',3,(#18816,#18817,#18818,#18819,#18820,
#18821,#18822,#18823,#18824,#18825,#18826,#18827,#18828,#18829,#18830,#18831,
#18832,#18833,#18834,#18835,#18836,#18837),.UNSPECIFIED.,.F.,.F.,(4,3,3,
3,3,3,3,4),(76.7077868271321,77.4087475366632,78.4011673768769,79.3935872170905,
80.3860070573041,81.3784268975178,82.3708467377314,82.9909721343117),
 .UNSPECIFIED.);
#2312=B_SPLINE_CURVE_WITH_KNOTS('',3,(#18838,#18839,#18840,#18841,#18842,
#18843,#18844,#18845,#18846,#18847,#18848,#18849,#18850,#18851,#18852,#18853,
#18854,#18855,#18856,#18857,#18858,#18859),.UNSPECIFIED.,.F.,.F.,(4,3,3,
3,3,3,3,4),(-79.2471980917962,-78.4011673768769,-77.4087475366633,-76.4163276964496,
-75.423907856236,-74.4314880160224,-73.4390681758088,-72.9640127846167),
 .UNSPECIFIED.);
#2313=B_SPLINE_CURVE_WITH_KNOTS('',3,(#18864,#18865,#18866,#18867,#18868,
#18869,#18870,#18871,#18872,#18873,#18874,#18875,#18876,#18877,#18878,#18879,
#18880,#18881,#18882,#18883,#18884,#18885,#18886,#18887,#18888),
 .UNSPECIFIED.,.F.,.F.,(4,3,3,3,3,3,3,3,4),(70.4246015199525,70.4618086551678,
71.4542284953814,72.4466483355951,73.4390681758087,74.4314880160223,75.423907856236,
76.4163276964496,76.7077868271321),.UNSPECIFIED.);
#2314=B_SPLINE_CURVE_WITH_KNOTS('',3,(#18889,#18890,#18891,#18892,#18893,
#18894,#18895,#18896,#18897,#18898,#18899,#18900,#18901,#18902,#18903,#18904,
#18905,#18906,#18907,#18908,#18909,#18910),.UNSPECIFIED.,.F.,.F.,(4,3,3,
3,3,3,3,4),(-72.9640127846167,-72.4466483355951,-71.4542284953815,-70.4618086551678,
-69.4693888149542,-68.4769689747406,-67.4845491345269,-66.680827477437),
 .UNSPECIFIED.);
#2315=B_SPLINE_CURVE_WITH_KNOTS('',3,(#18915,#18916,#18917,#18918,#18919,
#18920,#18921,#18922,#18923,#18924,#18925,#18926,#18927,#18928,#18929,#18930,
#18931,#18932,#18933,#18934,#18935,#18936),.UNSPECIFIED.,.F.,.F.,(4,3,3,
3,3,3,3,4),(64.1414162127729,64.507289613886,65.4997094540997,66.4921292943133,
67.4845491345269,68.4769689747405,69.4693888149542,70.4246015199525),
 .UNSPECIFIED.);
#2316=B_SPLINE_CURVE_WITH_KNOTS('',3,(#18937,#18938,#18939,#18940,#18941,
#18942,#18943,#18944,#18945,#18946,#18947,#18948,#18949,#18950,#18951,#18952,
#18953,#18954,#18955,#18956,#18957,#18958,#18959,#18960,#18961),
 .UNSPECIFIED.,.F.,.F.,(4,3,3,3,3,3,3,3,4),(-66.680827477437,-66.4921292943133,
-65.4997094540997,-64.5072896138861,-63.5148697736724,-62.5224499334588,
-61.5300300932452,-60.5376102530315,-60.3976421702575),.UNSPECIFIED.);
#2317=B_SPLINE_CURVE_WITH_KNOTS('',3,(#18966,#18967,#18968,#18969,#18970,
#18971,#18972,#18973,#18974,#18975,#18976,#18977,#18978,#18979,#18980,#18981,
#18982,#18983,#18984,#18985,#18986,#18987),.UNSPECIFIED.,.F.,.F.,(4,3,3,
3,3,3,3,4),(57.8582309055933,58.5527705726042,59.5451904128179,60.5376102530315,
61.5300300932451,62.5224499334588,63.5148697736724,64.1414162127729),
 .UNSPECIFIED.);
#2318=B_SPLINE_CURVE_WITH_KNOTS('',3,(#18988,#18989,#18990,#18991,#18992,
#18993,#18994,#18995,#18996,#18997,#18998,#18999,#19000,#19001,#19002,#19003,
#19004,#19005,#19006,#19007,#19008,#19009),.UNSPECIFIED.,.F.,.F.,(4,3,3,
3,3,3,3,4),(-60.3976421702575,-59.5451904128179,-58.5527705726043,-57.5603507323906,
-56.567930892177,-55.5755110519634,-54.5830912117497,-54.1144568630778),
 .UNSPECIFIED.);
#2319=B_SPLINE_CURVE_WITH_KNOTS('',3,(#19014,#19015,#19016,#19017,#19018,
#19019,#19020,#19021,#19022,#19023,#19024,#19025,#19026,#19027,#19028,#19029,
#19030,#19031,#19032,#19033,#19034,#19035,#19036,#19037,#19038),
 .UNSPECIFIED.,.F.,.F.,(4,3,3,3,3,3,3,3,4),(51.5750455984138,51.6058316911088,
52.5982515313225,53.5906713715361,54.5830912117497,55.5755110519634,56.567930892177,
57.5603507323906,57.8582309055933),.UNSPECIFIED.);
#2320=B_SPLINE_CURVE_WITH_KNOTS('',3,(#19039,#19040,#19041,#19042,#19043,
#19044,#19045,#19046,#19047,#19048,#19049,#19050,#19051,#19052,#19053,#19054,
#19055,#19056,#19057,#19058,#19059,#19060),.UNSPECIFIED.,.F.,.F.,(4,3,3,
3,3,3,3,4),(-54.1144568630778,-53.5906713715361,-52.5982515313225,-51.6058316911089,
-50.6134118508952,-49.6209920106816,-48.6285721704679,-47.8312715558983),
 .UNSPECIFIED.);
#2321=B_SPLINE_CURVE_WITH_KNOTS('',3,(#19065,#19066,#19067,#19068,#19069,
#19070,#19071,#19072,#19073,#19074,#19075,#19076,#19077,#19078,#19079,#19080,
#19081,#19082,#19083,#19084,#19085,#19086),.UNSPECIFIED.,.F.,.F.,(4,3,3,
3,3,3,3,4),(45.2918602912342,45.651312649827,46.6437324900407,47.6361523302543,
48.6285721704679,49.6209920106816,50.6134118508952,51.5750455984138),
 .UNSPECIFIED.);
#2322=B_SPLINE_CURVE_WITH_KNOTS('',3,(#19087,#19088,#19089,#19090,#19091,
#19092,#19093,#19094,#19095,#19096,#19097,#19098,#19099,#19100,#19101,#19102,
#19103,#19104,#19105,#19106,#19107,#19108,#19109,#19110,#19111),
 .UNSPECIFIED.,.F.,.F.,(4,3,3,3,3,3,3,3,4),(-47.8312715558983,-47.6361523302543,
-46.6437324900407,-45.651312649827,-44.6588928096134,-43.6664729693998,
-42.6740531291861,-41.6816332889725,-41.5480862487187),.UNSPECIFIED.);
#2323=B_SPLINE_CURVE_WITH_KNOTS('',3,(#19116,#19117,#19118,#19119,#19120,
#19121,#19122,#19123,#19124,#19125,#19126,#19127,#19128,#19129,#19130,#19131,
#19132,#19133,#19134,#19135,#19136,#19137),.UNSPECIFIED.,.F.,.F.,(4,3,3,
3,3,3,3,4),(39.0086749840546,39.6967936085453,40.6892134487589,41.6816332889725,
42.6740531291861,43.6664729693998,44.6588928096134,45.2918602912342),
 .UNSPECIFIED.);
#2324=B_SPLINE_CURVE_WITH_KNOTS('',3,(#19138,#19139,#19140,#19141,#19142,
#19143,#19144,#19145,#19146,#19147,#19148,#19149,#19150,#19151,#19152,#19153,
#19154,#19155,#19156,#19157,#19158,#19159),.UNSPECIFIED.,.F.,.F.,(4,3,3,
3,3,3,3,4),(-41.5480862487187,-40.6892134487589,-39.6967936085453,-38.7043737683316,
-37.711953928118,-36.7195340879044,-35.7271142476907,-35.2649009415391),
 .UNSPECIFIED.);
#2325=B_SPLINE_CURVE_WITH_KNOTS('',3,(#19164,#19165,#19166,#19167,#19168,
#19169,#19170,#19171,#19172,#19173,#19174,#19175,#19176,#19177,#19178,#19179,
#19180,#19181,#19182,#19183,#19184,#19185,#19186,#19187,#19188),
 .UNSPECIFIED.,.F.,.F.,(4,3,3,3,3,3,3,3,4),(32.725489676875,32.7498547270498,
33.7422745672635,34.7346944074771,35.7271142476907,36.7195340879043,37.711953928118,
38.7043737683316,39.0086749840546),.UNSPECIFIED.);
#2326=B_SPLINE_CURVE_WITH_KNOTS('',3,(#19189,#19190,#19191,#19192,#19193,
#19194,#19195,#19196,#19197,#19198,#19199,#19200,#19201,#19202,#19203,#19204,
#19205,#19206,#19207,#19208,#19209,#19210),.UNSPECIFIED.,.F.,.F.,(4,3,3,
3,3,3,3,4),(-35.2649009415391,-34.7346944074771,-33.7422745672635,-32.7498547270498,
-31.7574348868362,-30.7650150466226,-29.7725952064089,-28.9817156343595),
 .UNSPECIFIED.);
#2327=B_SPLINE_CURVE_WITH_KNOTS('',3,(#19215,#19216,#19217,#19218,#19219,
#19220,#19221,#19222,#19223,#19224,#19225,#19226,#19227,#19228,#19229,#19230,
#19231,#19232,#19233,#19234,#19235,#19236),.UNSPECIFIED.,.F.,.F.,(4,3,3,
3,3,3,3,4),(26.4423043696954,26.795335685768,27.7877555259817,28.7801753661953,
29.7725952064089,30.7650150466226,31.7574348868362,32.725489676875),
 .UNSPECIFIED.);
#2328=B_SPLINE_CURVE_WITH_KNOTS('',3,(#19237,#19238,#19239,#19240,#19241,
#19242,#19243,#19244,#19245,#19246,#19247,#19248,#19249,#19250,#19251,#19252,
#19253,#19254,#19255,#19256,#19257,#19258,#19259,#19260,#19261),
 .UNSPECIFIED.,.F.,.F.,(4,3,3,3,3,3,3,3,4),(-28.9817156343595,-28.7801753661953,
-27.7877555259817,-26.7953356857681,-25.8029158455544,-24.8104960053408,
-23.8180761651272,-22.8256563249135,-22.6985303271799),.UNSPECIFIED.);
#2329=B_SPLINE_CURVE_WITH_KNOTS('',3,(#19266,#19267,#19268,#19269,#19270,
#19271,#19272,#19273,#19274,#19275,#19276,#19277,#19278,#19279,#19280,#19281,
#19282,#19283,#19284,#19285,#19286,#19287),.UNSPECIFIED.,.F.,.F.,(4,3,3,
3,3,3,3,4),(20.1591190625158,20.8408166444862,21.8332364846999,22.8256563249135,
23.8180761651271,24.8104960053408,25.8029158455544,26.4423043696954),
 .UNSPECIFIED.);
#2330=B_SPLINE_CURVE_WITH_KNOTS('',3,(#19288,#19289,#19290,#19291,#19292,
#19293,#19294,#19295,#19296,#19297,#19298,#19299,#19300,#19301,#19302,#19303,
#19304,#19305,#19306,#19307,#19308,#19309),.UNSPECIFIED.,.F.,.F.,(4,3,3,
3,3,3,3,4),(-22.6985303271799,-21.8332364846999,-20.8408166444863,-19.8483968042726,
-18.855976964059,-17.8635571238454,-16.8711372836317,-16.4153450200003),
 .UNSPECIFIED.);
#2331=B_SPLINE_CURVE_WITH_KNOTS('',3,(#19314,#19315,#19316,#19317,#19318,
#19319,#19320,#19321,#19322,#19323,#19324,#19325,#19326,#19327,#19328,#19329,
#19330,#19331,#19332,#19333,#19334,#19335,#19336,#19337,#19338),
 .UNSPECIFIED.,.F.,.F.,(4,3,3,3,3,3,3,3,4),(13.8759337553362,13.8938777629908,
14.8862976032045,15.8787174434181,16.8711372836317,17.8635571238454,18.855976964059,
19.8483968042726,20.1591190625158),.UNSPECIFIED.);
#2332=B_SPLINE_CURVE_WITH_KNOTS('',3,(#19339,#19340,#19341,#19342,#19343,
#19344,#19345,#19346,#19347,#19348,#19349,#19350,#19351,#19352,#19353,#19354,
#19355,#19356,#19357,#19358,#19359,#19360),.UNSPECIFIED.,.F.,.F.,(4,3,3,
3,3,3,3,4),(-16.4153450200003,-15.8787174434181,-14.8862976032045,-13.8938777629908,
-12.9014579227772,-11.9090380825636,-10.9166182423499,-10.1321597128207),
 .UNSPECIFIED.);
#2333=B_SPLINE_CURVE_WITH_KNOTS('',3,(#19366,#19367,#19368,#19369,#19370,
#19371,#19372,#19373,#19374,#19375,#19376,#19377,#19378),.UNSPECIFIED.,
 .F.,.F.,(4,3,3,3,4),(-3.84897440564114,-2.9772595206409,-1.98483968042726,
-0.992419840213632,0.),.UNSPECIFIED.);
#2334=B_SPLINE_CURVE_WITH_KNOTS('',3,(#19381,#19382,#19383,#19384,#19385,
#19386,#19387,#19388,#19389,#19390,#19391,#19392,#19393,#19394,#19395,#19396,
#19397,#19398,#19399),.UNSPECIFIED.,.F.,.F.,(4,3,3,3,3,3,4),(2.01694489302841,
2.97725952064089,3.96967936085453,4.96209920106816,5.95451904128179,6.94693888149542,
7.59274844815661),.UNSPECIFIED.);
#2335=B_SPLINE_CURVE_WITH_KNOTS('',3,(#19405,#19406,#19407,#19408,#19409,
#19410,#19411,#19412),.UNSPECIFIED.,.F.,.F.,(4,1,1,1,1,4),(103.672557568463,
104.154034002175,105.146453842389,106.138873682603,107.131293522816,108.12371336303),
 .UNSPECIFIED.);
#2336=B_SPLINE_CURVE_WITH_KNOTS('',3,(#19415,#19416,#19417,#19418,#19419,
#19420,#19421,#19422,#19423),.UNSPECIFIED.,.F.,.F.,(4,1,1,1,1,1,4),(103.672557568463,
103.716185746199,104.708605586412,105.701025426626,106.693445266839,107.685865107053,
108.646179734666),.UNSPECIFIED.);
#2337=B_SPLINE_CURVE_WITH_KNOTS('',3,(#19428,#19429,#19430,#19431,#19432,
#19433,#19434,#19435,#19436,#19437),.UNSPECIFIED.,.F.,.F.,(4,1,1,1,1,1,
1,4),(97.3893722612836,98.1995149608937,99.1919348011073,100.184354641321,
101.176774481535,102.169194321748,103.161614161962,103.672557568463),
 .UNSPECIFIED.);
#2338=B_SPLINE_CURVE_WITH_KNOTS('',3,(#19438,#19439,#19440,#19441,#19442,
#19443,#19444,#19445,#19446,#19447),.UNSPECIFIED.,.F.,.F.,(4,1,1,1,1,1,
1,4),(97.3893722612836,97.7616667049168,98.7540865451304,99.7465063853441,
100.738926225558,101.731346065771,102.723765905985,103.672557568463),
 .UNSPECIFIED.);
#2339=B_SPLINE_CURVE_WITH_KNOTS('',3,(#19452,#19453,#19454,#19455,#19456,
#19457,#19458,#19459,#19460,#19461,#19462),.UNSPECIFIED.,.F.,.F.,(4,1,1,
1,1,1,1,1,4),(91.106186954104,91.2525760793983,92.2449959196119,93.2374157598255,
94.2298356000392,95.2222554402528,96.2146752804664,97.2070951206801,97.3893722612836),
 .UNSPECIFIED.);
#2340=B_SPLINE_CURVE_WITH_KNOTS('',3,(#19463,#19464,#19465,#19466,#19467,
#19468,#19469,#19470,#19471,#19472),.UNSPECIFIED.,.F.,.F.,(4,1,1,1,1,1,
1,4),(91.106186954104,91.807147663635,92.7995675038486,93.7919873440623,
94.7844071842759,95.7768270244895,96.7692468647032,97.3893722612836),
 .UNSPECIFIED.);
#2341=B_SPLINE_CURVE_WITH_KNOTS('',3,(#19477,#19478,#19479,#19480,#19481,
#19482,#19483,#19484,#19485,#19486),.UNSPECIFIED.,.F.,.F.,(4,1,1,1,1,1,
1,4),(84.8230016469244,85.2980570381165,86.2904768783301,87.2828967185437,
88.2753165587574,89.267736398971,90.2601562391846,91.106186954104),
 .UNSPECIFIED.);
#2342=B_SPLINE_CURVE_WITH_KNOTS('',3,(#19487,#19488,#19489,#19490,#19491,
#19492,#19493,#19494,#19495,#19496,#19497),.UNSPECIFIED.,.F.,.F.,(4,1,1,
1,1,1,1,1,4),(84.8230016469244,84.8602087821396,85.8526286223532,86.8450484625669,
87.8374683027805,88.8298881429941,89.8223079832078,90.8147278234214,91.106186954104),
 .UNSPECIFIED.);
#2343=B_SPLINE_CURVE_WITH_KNOTS('',3,(#19502,#19503,#19504,#19505,#19506,
#19507,#19508,#19509,#19510,#19511),.UNSPECIFIED.,.F.,.F.,(4,1,1,1,1,1,
1,4),(78.5398163397448,79.3435379968347,80.3359578370483,81.328377677262,
82.3207975174756,83.3132173576892,84.3056371979029,84.8230016469244),
 .UNSPECIFIED.);
#2344=B_SPLINE_CURVE_WITH_KNOTS('',3,(#19512,#19513,#19514,#19515,#19516,
#19517,#19518,#19519,#19520,#19521),.UNSPECIFIED.,.F.,.F.,(4,1,1,1,1,1,
1,4),(78.5398163397448,78.9056897408578,79.8981095810714,80.8905294212851,
81.8829492614987,82.8753691017123,83.867788941926,84.8230016469244),
 .UNSPECIFIED.);
#2345=B_SPLINE_CURVE_WITH_KNOTS('',3,(#19526,#19527,#19528,#19529,#19530,
#19531,#19532,#19533,#19534,#19535,#19536),.UNSPECIFIED.,.F.,.F.,(4,1,1,
1,1,1,1,1,4),(72.2566310325652,72.3965991153393,73.3890189555529,74.3814387957665,
75.3738586359802,76.3662784761938,77.3586983164074,78.3511181566211,78.5398163397448),
 .UNSPECIFIED.);
#2346=B_SPLINE_CURVE_WITH_KNOTS('',3,(#19537,#19538,#19539,#19540,#19541,
#19542,#19543,#19544,#19545,#19546),.UNSPECIFIED.,.F.,.F.,(4,1,1,1,1,1,
1,4),(72.2566310325652,72.951170699576,73.9435905397896,74.9360103800033,
75.9284302202169,76.9208500604305,77.9132699006442,78.5398163397448),
 .UNSPECIFIED.);
#2347=B_SPLINE_CURVE_WITH_KNOTS('',3,(#19551,#19552,#19553,#19554,#19555,
#19556,#19557,#19558,#19559,#19560),.UNSPECIFIED.,.F.,.F.,(4,1,1,1,1,1,
1,4),(65.9734457253856,66.4420800740575,67.4344999142711,68.4269197544847,
69.4193395946984,70.411759434912,71.4041792751256,72.2566310325652),
 .UNSPECIFIED.);
#2348=B_SPLINE_CURVE_WITH_KNOTS('',3,(#19561,#19562,#19563,#19564,#19565,
#19566,#19567,#19568,#19569,#19570,#19571),.UNSPECIFIED.,.F.,.F.,(4,1,1,
1,1,1,1,1,4),(65.9734457253856,66.0042318180806,66.9966516582942,67.9890714985079,
68.9814913387215,69.9739111789351,70.9663310191488,71.9587508593624,72.2566310325652),
 .UNSPECIFIED.);
#2349=B_SPLINE_CURVE_WITH_KNOTS('',3,(#19576,#19577,#19578,#19579,#19580,
#19581,#19582,#19583,#19584,#19585),.UNSPECIFIED.,.F.,.F.,(4,1,1,1,1,1,
1,4),(59.690260418206,60.4875610327757,61.4799808729893,62.4724007132029,
63.4648205534166,64.4572403936302,65.4496602338438,65.9734457253856),
 .UNSPECIFIED.);
#2350=B_SPLINE_CURVE_WITH_KNOTS('',3,(#19586,#19587,#19588,#19589,#19590,
#19591,#19592,#19593,#19594,#19595),.UNSPECIFIED.,.F.,.F.,(4,1,1,1,1,1,
1,4),(59.690260418206,60.0497127767988,61.0421326170124,62.0345524572261,
63.0269722974397,64.0193921376533,65.011811977867,65.9734457253856),
 .UNSPECIFIED.);
#2351=B_SPLINE_CURVE_WITH_KNOTS('',3,(#19600,#19601,#19602,#19603,#19604,
#19605,#19606,#19607,#19608,#19609,#19610),.UNSPECIFIED.,.F.,.F.,(4,1,1,
1,1,1,1,1,4),(53.4070751110264,53.5406221512803,54.5330419914939,55.5254618317075,
56.5178816719212,57.5103015121348,58.5027213523484,59.4951411925621,59.690260418206),
 .UNSPECIFIED.);
#2352=B_SPLINE_CURVE_WITH_KNOTS('',3,(#19611,#19612,#19613,#19614,#19615,
#19616,#19617,#19618,#19619,#19620),.UNSPECIFIED.,.F.,.F.,(4,1,1,1,1,1,
1,4),(53.4070751110264,54.095193735517,55.0876135757306,56.0800334159443,
57.0724532561579,58.0648730963715,59.0572929365852,59.690260418206),
 .UNSPECIFIED.);
#2353=B_SPLINE_CURVE_WITH_KNOTS('',3,(#19625,#19626,#19627,#19628,#19629,
#19630,#19631,#19632,#19633,#19634),.UNSPECIFIED.,.F.,.F.,(4,1,1,1,1,1,
1,4),(47.1238898038468,47.5861031099985,48.5785229502121,49.5709427904257,
50.5633626306394,51.555782470853,52.5482023110666,53.4070751110264),
 .UNSPECIFIED.);
#2354=B_SPLINE_CURVE_WITH_KNOTS('',3,(#19635,#19636,#19637,#19638,#19639,
#19640,#19641,#19642,#19643,#19644,#19645),.UNSPECIFIED.,.F.,.F.,(4,1,1,
1,1,1,1,1,4),(47.1238898038468,47.1482548540216,48.1406746942352,49.1330945344489,
50.1255143746625,51.1179342148761,52.1103540550898,53.1027738953034,53.4070751110264),
 .UNSPECIFIED.);
#2355=B_SPLINE_CURVE_WITH_KNOTS('',3,(#19650,#19651,#19652,#19653,#19654,
#19655,#19656,#19657,#19658,#19659),.UNSPECIFIED.,.F.,.F.,(4,1,1,1,1,1,
1,4),(40.8407044966672,41.6315840687167,42.6240039089303,43.6164237491439,
44.6088435893576,45.6012634295712,46.5936832697848,47.1238898038468),
 .UNSPECIFIED.);
#2356=B_SPLINE_CURVE_WITH_KNOTS('',3,(#19660,#19661,#19662,#19663,#19664,
#19665,#19666,#19667,#19668,#19669),.UNSPECIFIED.,.F.,.F.,(4,1,1,1,1,1,
1,4),(40.8407044966672,41.1937358127398,42.1861556529534,43.1785754931671,
44.1709953333807,45.1634151735943,46.155835013808,47.1238898038468),
 .UNSPECIFIED.);
#2357=B_SPLINE_CURVE_WITH_KNOTS('',3,(#19674,#19675,#19676,#19677,#19678,
#19679,#19680,#19681,#19682,#19683,#19684),.UNSPECIFIED.,.F.,.F.,(4,1,1,
1,1,1,1,1,4),(34.5575191894876,34.6846451872213,35.6770650274349,36.6694848676485,
37.6619047078622,38.6543245480758,39.6467443882894,40.639164228503,40.8407044966672),
 .UNSPECIFIED.);
#2358=B_SPLINE_CURVE_WITH_KNOTS('',3,(#19685,#19686,#19687,#19688,#19689,
#19690,#19691,#19692,#19693,#19694),.UNSPECIFIED.,.F.,.F.,(4,1,1,1,1,1,
1,4),(34.5575191894876,35.239216771458,36.2316366116717,37.2240564518853,
38.2164762920989,39.2088961323126,40.2013159725262,40.8407044966672),
 .UNSPECIFIED.);
#2359=B_SPLINE_CURVE_WITH_KNOTS('',3,(#19699,#19700,#19701,#19702,#19703,
#19704,#19705,#19706,#19707,#19708),.UNSPECIFIED.,.F.,.F.,(4,1,1,1,1,1,
1,4),(28.274333882308,28.7301261459395,29.7225459861531,30.7149658263667,
31.7073856665804,32.699805506794,33.6922253470076,34.5575191894876),
 .UNSPECIFIED.);
#2360=B_SPLINE_CURVE_WITH_KNOTS('',3,(#19709,#19710,#19711,#19712,#19713,
#19714,#19715,#19716,#19717,#19718,#19719),.UNSPECIFIED.,.F.,.F.,(4,1,1,
1,1,1,1,1,4),(28.274333882308,28.2922778899626,29.2846977301762,30.2771175703899,
31.2695374106035,32.2619572508171,33.2543770910308,34.2467969312444,34.5575191894876),
 .UNSPECIFIED.);
#2361=B_SPLINE_CURVE_WITH_KNOTS('',3,(#19724,#19725,#19726,#19727,#19728,
#19729,#19730,#19731,#19732,#19733),.UNSPECIFIED.,.F.,.F.,(4,1,1,1,1,1,
1,4),(21.9911485751285,22.7756071046577,23.7680269448713,24.7604467850849,
25.7528666252986,26.7452864655122,27.7377063057258,28.274333882308),
 .UNSPECIFIED.);
#2362=B_SPLINE_CURVE_WITH_KNOTS('',3,(#19734,#19735,#19736,#19737,#19738,
#19739,#19740,#19741,#19742,#19743),.UNSPECIFIED.,.F.,.F.,(4,1,1,1,1,1,
1,4),(21.9911485751285,22.3377588486808,23.3301786888945,24.3225985291081,
25.3150183693217,26.3074382095353,27.299858049749,28.274333882308),
 .UNSPECIFIED.);
#2363=B_SPLINE_CURVE_WITH_KNOTS('',3,(#19749,#19750,#19751,#19752,#19753),
 .UNSPECIFIED.,.F.,.F.,(4,1,4),(14.3984001269718,15.3908199671854,15.7079632679489),
 .UNSPECIFIED.);
#2364=B_SPLINE_CURVE_WITH_KNOTS('',3,(#19756,#19757,#19758,#19759,#19760),
 .UNSPECIFIED.,.F.,.F.,(4,1,4),(13.8759337553362,14.8362483829486,15.7079632679489),
 .UNSPECIFIED.);
#2365=B_SPLINE_CURVE_WITH_KNOTS('',3,(#19766,#19767,#19768,#19769,#19770,
#19771,#19772,#19773),.UNSPECIFIED.,.F.,.F.,(4,1,1,1,1,4),(103.672557568463,
104.154034002175,105.146453842389,106.138873682603,107.131293522816,108.12371336303),
 .UNSPECIFIED.);
#2366=B_SPLINE_CURVE_WITH_KNOTS('',3,(#19776,#19777,#19778,#19779,#19780,
#19781,#19782,#19783,#19784),.UNSPECIFIED.,.F.,.F.,(4,1,1,1,1,1,4),(103.672557568463,
103.716185746199,104.708605586412,105.701025426626,106.693445266839,107.685865107053,
108.646179734666),.UNSPECIFIED.);
#2367=B_SPLINE_CURVE_WITH_KNOTS('',3,(#19789,#19790,#19791,#19792,#19793,
#19794,#19795,#19796,#19797,#19798),.UNSPECIFIED.,.F.,.F.,(4,1,1,1,1,1,
1,4),(97.3893722612836,98.1995149608937,99.1919348011073,100.184354641321,
101.176774481535,102.169194321748,103.161614161962,103.672557568463),
 .UNSPECIFIED.);
#2368=B_SPLINE_CURVE_WITH_KNOTS('',3,(#19799,#19800,#19801,#19802,#19803,
#19804,#19805,#19806,#19807,#19808),.UNSPECIFIED.,.F.,.F.,(4,1,1,1,1,1,
1,4),(97.3893722612836,97.7616667049168,98.7540865451304,99.7465063853441,
100.738926225558,101.731346065771,102.723765905985,103.672557568463),
 .UNSPECIFIED.);
#2369=B_SPLINE_CURVE_WITH_KNOTS('',3,(#19813,#19814,#19815,#19816,#19817,
#19818,#19819,#19820,#19821,#19822,#19823),.UNSPECIFIED.,.F.,.F.,(4,1,1,
1,1,1,1,1,4),(91.106186954104,91.2525760793983,92.2449959196119,93.2374157598255,
94.2298356000392,95.2222554402528,96.2146752804664,97.2070951206801,97.3893722612836),
 .UNSPECIFIED.);
#2370=B_SPLINE_CURVE_WITH_KNOTS('',3,(#19824,#19825,#19826,#19827,#19828,
#19829,#19830,#19831,#19832,#19833),.UNSPECIFIED.,.F.,.F.,(4,1,1,1,1,1,
1,4),(91.106186954104,91.807147663635,92.7995675038486,93.7919873440623,
94.7844071842759,95.7768270244895,96.7692468647032,97.3893722612836),
 .UNSPECIFIED.);
#2371=B_SPLINE_CURVE_WITH_KNOTS('',3,(#19838,#19839,#19840,#19841,#19842,
#19843,#19844,#19845,#19846,#19847),.UNSPECIFIED.,.F.,.F.,(4,1,1,1,1,1,
1,4),(84.8230016469244,85.2980570381165,86.2904768783301,87.2828967185437,
88.2753165587574,89.267736398971,90.2601562391846,91.106186954104),
 .UNSPECIFIED.);
#2372=B_SPLINE_CURVE_WITH_KNOTS('',3,(#19848,#19849,#19850,#19851,#19852,
#19853,#19854,#19855,#19856,#19857,#19858),.UNSPECIFIED.,.F.,.F.,(4,1,1,
1,1,1,1,1,4),(84.8230016469244,84.8602087821396,85.8526286223532,86.8450484625669,
87.8374683027805,88.8298881429941,89.8223079832078,90.8147278234214,91.106186954104),
 .UNSPECIFIED.);
#2373=B_SPLINE_CURVE_WITH_KNOTS('',3,(#19863,#19864,#19865,#19866,#19867,
#19868,#19869,#19870,#19871,#19872),.UNSPECIFIED.,.F.,.F.,(4,1,1,1,1,1,
1,4),(78.5398163397448,79.3435379968347,80.3359578370483,81.328377677262,
82.3207975174756,83.3132173576892,84.3056371979029,84.8230016469244),
 .UNSPECIFIED.);
#2374=B_SPLINE_CURVE_WITH_KNOTS('',3,(#19873,#19874,#19875,#19876,#19877,
#19878,#19879,#19880,#19881,#19882),.UNSPECIFIED.,.F.,.F.,(4,1,1,1,1,1,
1,4),(78.5398163397448,78.9056897408578,79.8981095810714,80.8905294212851,
81.8829492614987,82.8753691017123,83.867788941926,84.8230016469244),
 .UNSPECIFIED.);
#2375=B_SPLINE_CURVE_WITH_KNOTS('',3,(#19887,#19888,#19889,#19890,#19891,
#19892,#19893,#19894,#19895,#19896,#19897),.UNSPECIFIED.,.F.,.F.,(4,1,1,
1,1,1,1,1,4),(72.2566310325652,72.3965991153393,73.3890189555529,74.3814387957665,
75.3738586359802,76.3662784761938,77.3586983164074,78.3511181566211,78.5398163397448),
 .UNSPECIFIED.);
#2376=B_SPLINE_CURVE_WITH_KNOTS('',3,(#19898,#19899,#19900,#19901,#19902,
#19903,#19904,#19905,#19906,#19907),.UNSPECIFIED.,.F.,.F.,(4,1,1,1,1,1,
1,4),(72.2566310325652,72.951170699576,73.9435905397896,74.9360103800033,
75.9284302202169,76.9208500604305,77.9132699006442,78.5398163397448),
 .UNSPECIFIED.);
#2377=B_SPLINE_CURVE_WITH_KNOTS('',3,(#19912,#19913,#19914,#19915,#19916,
#19917,#19918,#19919,#19920,#19921),.UNSPECIFIED.,.F.,.F.,(4,1,1,1,1,1,
1,4),(65.9734457253856,66.4420800740575,67.4344999142711,68.4269197544847,
69.4193395946984,70.411759434912,71.4041792751256,72.2566310325652),
 .UNSPECIFIED.);
#2378=B_SPLINE_CURVE_WITH_KNOTS('',3,(#19922,#19923,#19924,#19925,#19926,
#19927,#19928,#19929,#19930,#19931,#19932),.UNSPECIFIED.,.F.,.F.,(4,1,1,
1,1,1,1,1,4),(65.9734457253856,66.0042318180806,66.9966516582942,67.9890714985079,
68.9814913387215,69.9739111789351,70.9663310191488,71.9587508593624,72.2566310325652),
 .UNSPECIFIED.);
#2379=B_SPLINE_CURVE_WITH_KNOTS('',3,(#19937,#19938,#19939,#19940,#19941,
#19942,#19943,#19944,#19945,#19946),.UNSPECIFIED.,.F.,.F.,(4,1,1,1,1,1,
1,4),(59.690260418206,60.4875610327757,61.4799808729893,62.4724007132029,
63.4648205534166,64.4572403936302,65.4496602338438,65.9734457253856),
 .UNSPECIFIED.);
#2380=B_SPLINE_CURVE_WITH_KNOTS('',3,(#19947,#19948,#19949,#19950,#19951,
#19952,#19953,#19954,#19955,#19956),.UNSPECIFIED.,.F.,.F.,(4,1,1,1,1,1,
1,4),(59.690260418206,60.0497127767988,61.0421326170124,62.0345524572261,
63.0269722974397,64.0193921376533,65.011811977867,65.9734457253856),
 .UNSPECIFIED.);
#2381=B_SPLINE_CURVE_WITH_KNOTS('',3,(#19961,#19962,#19963,#19964,#19965,
#19966,#19967,#19968,#19969,#19970,#19971),.UNSPECIFIED.,.F.,.F.,(4,1,1,
1,1,1,1,1,4),(53.4070751110264,53.5406221512803,54.5330419914939,55.5254618317075,
56.5178816719212,57.5103015121348,58.5027213523484,59.4951411925621,59.690260418206),
 .UNSPECIFIED.);
#2382=B_SPLINE_CURVE_WITH_KNOTS('',3,(#19972,#19973,#19974,#19975,#19976,
#19977,#19978,#19979,#19980,#19981),.UNSPECIFIED.,.F.,.F.,(4,1,1,1,1,1,
1,4),(53.4070751110264,54.095193735517,55.0876135757306,56.0800334159443,
57.0724532561579,58.0648730963715,59.0572929365852,59.690260418206),
 .UNSPECIFIED.);
#2383=B_SPLINE_CURVE_WITH_KNOTS('',3,(#19986,#19987,#19988,#19989,#19990,
#19991,#19992,#19993,#19994,#19995),.UNSPECIFIED.,.F.,.F.,(4,1,1,1,1,1,
1,4),(47.1238898038468,47.5861031099985,48.5785229502121,49.5709427904257,
50.5633626306394,51.555782470853,52.5482023110666,53.4070751110264),
 .UNSPECIFIED.);
#2384=B_SPLINE_CURVE_WITH_KNOTS('',3,(#19996,#19997,#19998,#19999,#20000,
#20001,#20002,#20003,#20004,#20005,#20006),.UNSPECIFIED.,.F.,.F.,(4,1,1,
1,1,1,1,1,4),(47.1238898038468,47.1482548540216,48.1406746942352,49.1330945344489,
50.1255143746625,51.1179342148761,52.1103540550898,53.1027738953034,53.4070751110264),
 .UNSPECIFIED.);
#2385=B_SPLINE_CURVE_WITH_KNOTS('',3,(#20011,#20012,#20013,#20014,#20015,
#20016,#20017,#20018,#20019,#20020),.UNSPECIFIED.,.F.,.F.,(4,1,1,1,1,1,
1,4),(40.8407044966672,41.6315840687167,42.6240039089303,43.6164237491439,
44.6088435893576,45.6012634295712,46.5936832697848,47.1238898038468),
 .UNSPECIFIED.);
#2386=B_SPLINE_CURVE_WITH_KNOTS('',3,(#20021,#20022,#20023,#20024,#20025,
#20026,#20027,#20028,#20029,#20030),.UNSPECIFIED.,.F.,.F.,(4,1,1,1,1,1,
1,4),(40.8407044966672,41.1937358127398,42.1861556529534,43.1785754931671,
44.1709953333807,45.1634151735943,46.155835013808,47.1238898038468),
 .UNSPECIFIED.);
#2387=B_SPLINE_CURVE_WITH_KNOTS('',3,(#20035,#20036,#20037,#20038,#20039,
#20040,#20041,#20042,#20043,#20044,#20045),.UNSPECIFIED.,.F.,.F.,(4,1,1,
1,1,1,1,1,4),(34.5575191894876,34.6846451872213,35.6770650274349,36.6694848676485,
37.6619047078622,38.6543245480758,39.6467443882894,40.639164228503,40.8407044966672),
 .UNSPECIFIED.);
#2388=B_SPLINE_CURVE_WITH_KNOTS('',3,(#20046,#20047,#20048,#20049,#20050,
#20051,#20052,#20053,#20054,#20055),.UNSPECIFIED.,.F.,.F.,(4,1,1,1,1,1,
1,4),(34.5575191894876,35.239216771458,36.2316366116717,37.2240564518853,
38.2164762920989,39.2088961323126,40.2013159725262,40.8407044966672),
 .UNSPECIFIED.);
#2389=B_SPLINE_CURVE_WITH_KNOTS('',3,(#20060,#20061,#20062,#20063,#20064,
#20065,#20066,#20067,#20068,#20069),.UNSPECIFIED.,.F.,.F.,(4,1,1,1,1,1,
1,4),(28.274333882308,28.7301261459395,29.7225459861531,30.7149658263667,
31.7073856665804,32.699805506794,33.6922253470076,34.5575191894876),
 .UNSPECIFIED.);
#2390=B_SPLINE_CURVE_WITH_KNOTS('',3,(#20070,#20071,#20072,#20073,#20074,
#20075,#20076,#20077,#20078,#20079,#20080),.UNSPECIFIED.,.F.,.F.,(4,1,1,
1,1,1,1,1,4),(28.274333882308,28.2922778899626,29.2846977301762,30.2771175703899,
31.2695374106035,32.2619572508171,33.2543770910308,34.2467969312444,34.5575191894876),
 .UNSPECIFIED.);
#2391=B_SPLINE_CURVE_WITH_KNOTS('',3,(#20085,#20086,#20087,#20088,#20089,
#20090,#20091,#20092,#20093,#20094),.UNSPECIFIED.,.F.,.F.,(4,1,1,1,1,1,
1,4),(21.9911485751285,22.7756071046577,23.7680269448713,24.7604467850849,
25.7528666252986,26.7452864655122,27.7377063057258,28.274333882308),
 .UNSPECIFIED.);
#2392=B_SPLINE_CURVE_WITH_KNOTS('',3,(#20095,#20096,#20097,#20098,#20099,
#20100,#20101,#20102,#20103,#20104),.UNSPECIFIED.,.F.,.F.,(4,1,1,1,1,1,
1,4),(21.9911485751285,22.3377588486808,23.3301786888945,24.3225985291081,
25.3150183693217,26.3074382095353,27.299858049749,28.274333882308),
 .UNSPECIFIED.);
#2393=B_SPLINE_CURVE_WITH_KNOTS('',3,(#20110,#20111,#20112,#20113,#20114),
 .UNSPECIFIED.,.F.,.F.,(4,1,4),(14.3984001269718,15.3908199671854,15.7079632679489),
 .UNSPECIFIED.);
#2394=B_SPLINE_CURVE_WITH_KNOTS('',3,(#20117,#20118,#20119,#20120,#20121),
 .UNSPECIFIED.,.F.,.F.,(4,1,4),(13.8759337553362,14.8362483829486,15.7079632679489),
 .UNSPECIFIED.);
#2395=B_SPLINE_CURVE_WITH_KNOTS('',3,(#20127,#20128,#20129,#20130),
 .UNSPECIFIED.,.F.,.F.,(4,4),(95.5573427486709,96.2647245007222),
 .UNSPECIFIED.);
#2396=B_SPLINE_CURVE_WITH_KNOTS('',3,(#20138,#20139,#20140,#20141,#20142,
#20143,#20144,#20145,#20146,#20147),.UNSPECIFIED.,.F.,.F.,(4,3,3,4),(-94.2477796076938,
-93.2874649800814,-92.2950451398677,-91.8135687061554),.UNSPECIFIED.);
#2397=B_SPLINE_CURVE_WITH_KNOTS('',3,(#20152,#20153,#20154,#20155,#20156,
#20157,#20158,#20159,#20160,#20161,#20162,#20163,#20164,#20165,#20166,#20167,
#20168,#20169,#20170,#20171,#20172,#20173,#20174,#20175,#20176),
 .UNSPECIFIED.,.F.,.F.,(4,3,3,3,3,3,3,3,4),(89.2741574414913,89.3177856192268,
90.3102054594404,91.3026252996541,92.2950451398677,93.2874649800813,94.279884820295,
95.2723046605086,95.5573427486709),.UNSPECIFIED.);
#2398=B_SPLINE_CURVE_WITH_KNOTS('',3,(#20177,#20178,#20179,#20180,#20181,
#20182,#20183,#20184,#20185,#20186,#20187,#20188,#20189,#20190,#20191,#20192,
#20193,#20194,#20195,#20196,#20197,#20198),.UNSPECIFIED.,.F.,.F.,(4,3,3,
3,3,3,3,4),(-91.8135687061554,-91.3026252996541,-90.3102054594405,-89.3177856192269,
-88.3253657790132,-87.3329459387996,-86.340526098586,-85.5303833989758),
 .UNSPECIFIED.);
#2399=B_SPLINE_CURVE_WITH_KNOTS('',3,(#20203,#20204,#20205,#20206,#20207,
#20208,#20209,#20210,#20211,#20212,#20213,#20214,#20215,#20216,#20217,#20218,
#20219,#20220,#20221,#20222,#20223,#20224),.UNSPECIFIED.,.F.,.F.,(4,3,3,
3,3,3,3,4),(82.9909721343117,83.363266577945,84.3556864181587,85.3481062583723,
86.3405260985859,87.3329459387996,88.3253657790132,89.2741574414913),
 .UNSPECIFIED.);
#2400=B_SPLINE_CURVE_WITH_KNOTS('',3,(#20225,#20226,#20227,#20228,#20229,
#20230,#20231,#20232,#20233,#20234,#20235,#20236,#20237,#20238,#20239,#20240,
#20241,#20242,#20243,#20244,#20245,#20246,#20247,#20248,#20249),
 .UNSPECIFIED.,.F.,.F.,(4,3,3,3,3,3,3,3,4),(-85.5303833989758,-85.3481062583723,
-84.3556864181587,-83.3632665779451,-82.3708467377314,-81.3784268975178,
-80.3860070573042,-79.3935872170905,-79.2471980917962),.UNSPECIFIED.);
#2401=B_SPLINE_CURVE_WITH_KNOTS('',3,(#20254,#20255,#20256,#20257,#20258,
#20259,#20260,#20261,#20262,#20263,#20264,#20265,#20266,#20267,#20268,#20269,
#20270,#20271,#20272,#20273,#20274,#20275),.UNSPECIFIED.,.F.,.F.,(4,3,3,
3,3,3,3,4),(76.7077868271321,77.4087475366632,78.4011673768769,79.3935872170905,
80.3860070573041,81.3784268975178,82.3708467377314,82.9909721343117),
 .UNSPECIFIED.);
#2402=B_SPLINE_CURVE_WITH_KNOTS('',3,(#20276,#20277,#20278,#20279,#20280,
#20281,#20282,#20283,#20284,#20285,#20286,#20287,#20288,#20289,#20290,#20291,
#20292,#20293,#20294,#20295,#20296,#20297),.UNSPECIFIED.,.F.,.F.,(4,3,3,
3,3,3,3,4),(-79.2471980917962,-78.4011673768769,-77.4087475366633,-76.4163276964496,
-75.423907856236,-74.4314880160224,-73.4390681758088,-72.9640127846167),
 .UNSPECIFIED.);
#2403=B_SPLINE_CURVE_WITH_KNOTS('',3,(#20302,#20303,#20304,#20305,#20306,
#20307,#20308,#20309,#20310,#20311,#20312,#20313,#20314,#20315,#20316,#20317,
#20318,#20319,#20320,#20321,#20322,#20323,#20324,#20325,#20326),
 .UNSPECIFIED.,.F.,.F.,(4,3,3,3,3,3,3,3,4),(70.4246015199525,70.4618086551678,
71.4542284953814,72.4466483355951,73.4390681758087,74.4314880160223,75.423907856236,
76.4163276964496,76.7077868271321),.UNSPECIFIED.);
#2404=B_SPLINE_CURVE_WITH_KNOTS('',3,(#20327,#20328,#20329,#20330,#20331,
#20332,#20333,#20334,#20335,#20336,#20337,#20338,#20339,#20340,#20341,#20342,
#20343,#20344,#20345,#20346,#20347,#20348),.UNSPECIFIED.,.F.,.F.,(4,3,3,
3,3,3,3,4),(-72.9640127846167,-72.4466483355951,-71.4542284953815,-70.4618086551678,
-69.4693888149542,-68.4769689747406,-67.4845491345269,-66.680827477437),
 .UNSPECIFIED.);
#2405=B_SPLINE_CURVE_WITH_KNOTS('',3,(#20353,#20354,#20355,#20356,#20357,
#20358,#20359,#20360,#20361,#20362,#20363,#20364,#20365,#20366,#20367,#20368,
#20369,#20370,#20371,#20372,#20373,#20374),.UNSPECIFIED.,.F.,.F.,(4,3,3,
3,3,3,3,4),(64.1414162127729,64.507289613886,65.4997094540997,66.4921292943133,
67.4845491345269,68.4769689747405,69.4693888149542,70.4246015199525),
 .UNSPECIFIED.);
#2406=B_SPLINE_CURVE_WITH_KNOTS('',3,(#20375,#20376,#20377,#20378,#20379,
#20380,#20381,#20382,#20383,#20384,#20385,#20386,#20387,#20388,#20389,#20390,
#20391,#20392,#20393,#20394,#20395,#20396,#20397,#20398,#20399),
 .UNSPECIFIED.,.F.,.F.,(4,3,3,3,3,3,3,3,4),(-66.680827477437,-66.4921292943133,
-65.4997094540997,-64.5072896138861,-63.5148697736724,-62.5224499334588,
-61.5300300932452,-60.5376102530315,-60.3976421702575),.UNSPECIFIED.);
#2407=B_SPLINE_CURVE_WITH_KNOTS('',3,(#20404,#20405,#20406,#20407,#20408,
#20409,#20410,#20411,#20412,#20413,#20414,#20415,#20416,#20417,#20418,#20419,
#20420,#20421,#20422,#20423,#20424,#20425),.UNSPECIFIED.,.F.,.F.,(4,3,3,
3,3,3,3,4),(57.8582309055933,58.5527705726042,59.5451904128179,60.5376102530315,
61.5300300932451,62.5224499334588,63.5148697736724,64.1414162127729),
 .UNSPECIFIED.);
#2408=B_SPLINE_CURVE_WITH_KNOTS('',3,(#20426,#20427,#20428,#20429,#20430,
#20431,#20432,#20433,#20434,#20435,#20436,#20437,#20438,#20439,#20440,#20441,
#20442,#20443,#20444,#20445,#20446,#20447),.UNSPECIFIED.,.F.,.F.,(4,3,3,
3,3,3,3,4),(-60.3976421702575,-59.5451904128179,-58.5527705726043,-57.5603507323906,
-56.567930892177,-55.5755110519634,-54.5830912117497,-54.1144568630778),
 .UNSPECIFIED.);
#2409=B_SPLINE_CURVE_WITH_KNOTS('',3,(#20452,#20453,#20454,#20455,#20456,
#20457,#20458,#20459,#20460,#20461,#20462,#20463,#20464,#20465,#20466,#20467,
#20468,#20469,#20470,#20471,#20472,#20473,#20474,#20475,#20476),
 .UNSPECIFIED.,.F.,.F.,(4,3,3,3,3,3,3,3,4),(51.5750455984138,51.6058316911088,
52.5982515313225,53.5906713715361,54.5830912117497,55.5755110519634,56.567930892177,
57.5603507323906,57.8582309055933),.UNSPECIFIED.);
#2410=B_SPLINE_CURVE_WITH_KNOTS('',3,(#20477,#20478,#20479,#20480,#20481,
#20482,#20483,#20484,#20485,#20486,#20487,#20488,#20489,#20490,#20491,#20492,
#20493,#20494,#20495,#20496,#20497,#20498),.UNSPECIFIED.,.F.,.F.,(4,3,3,
3,3,3,3,4),(-54.1144568630778,-53.5906713715361,-52.5982515313225,-51.6058316911089,
-50.6134118508952,-49.6209920106816,-48.628572170468,-47.8312715558983),
 .UNSPECIFIED.);
#2411=B_SPLINE_CURVE_WITH_KNOTS('',3,(#20503,#20504,#20505,#20506,#20507,
#20508,#20509,#20510,#20511,#20512,#20513,#20514,#20515,#20516,#20517,#20518,
#20519,#20520,#20521,#20522,#20523,#20524),.UNSPECIFIED.,.F.,.F.,(4,3,3,
3,3,3,3,4),(45.2918602912342,45.651312649827,46.6437324900407,47.6361523302543,
48.6285721704679,49.6209920106816,50.6134118508952,51.5750455984138),
 .UNSPECIFIED.);
#2412=B_SPLINE_CURVE_WITH_KNOTS('',3,(#20525,#20526,#20527,#20528,#20529,
#20530,#20531,#20532,#20533,#20534,#20535,#20536,#20537,#20538,#20539,#20540,
#20541,#20542,#20543,#20544,#20545,#20546,#20547,#20548,#20549),
 .UNSPECIFIED.,.F.,.F.,(4,3,3,3,3,3,3,3,4),(-47.8312715558983,-47.6361523302543,
-46.6437324900407,-45.6513126498271,-44.6588928096134,-43.6664729693998,
-42.6740531291862,-41.6816332889725,-41.5480862487187),.UNSPECIFIED.);
#2413=B_SPLINE_CURVE_WITH_KNOTS('',3,(#20554,#20555,#20556,#20557,#20558,
#20559,#20560,#20561,#20562,#20563,#20564,#20565,#20566,#20567,#20568,#20569,
#20570,#20571,#20572,#20573,#20574,#20575),.UNSPECIFIED.,.F.,.F.,(4,3,3,
3,3,3,3,4),(39.0086749840546,39.6967936085453,40.6892134487589,41.6816332889725,
42.6740531291861,43.6664729693998,44.6588928096134,45.2918602912342),
 .UNSPECIFIED.);
#2414=B_SPLINE_CURVE_WITH_KNOTS('',3,(#20576,#20577,#20578,#20579,#20580,
#20581,#20582,#20583,#20584,#20585,#20586,#20587,#20588,#20589,#20590,#20591,
#20592,#20593,#20594,#20595,#20596,#20597),.UNSPECIFIED.,.F.,.F.,(4,3,3,
3,3,3,3,4),(-41.5480862487187,-40.6892134487589,-39.6967936085453,-38.7043737683316,
-37.711953928118,-36.7195340879044,-35.7271142476907,-35.2649009415391),
 .UNSPECIFIED.);
#2415=B_SPLINE_CURVE_WITH_KNOTS('',3,(#20602,#20603,#20604,#20605,#20606,
#20607,#20608,#20609,#20610,#20611,#20612,#20613,#20614,#20615,#20616,#20617,
#20618,#20619,#20620,#20621,#20622,#20623,#20624,#20625,#20626),
 .UNSPECIFIED.,.F.,.F.,(4,3,3,3,3,3,3,3,4),(32.725489676875,32.7498547270498,
33.7422745672635,34.7346944074771,35.7271142476907,36.7195340879043,37.711953928118,
38.7043737683316,39.0086749840546),.UNSPECIFIED.);
#2416=B_SPLINE_CURVE_WITH_KNOTS('',3,(#20627,#20628,#20629,#20630,#20631,
#20632,#20633,#20634,#20635,#20636,#20637,#20638,#20639,#20640,#20641,#20642,
#20643,#20644,#20645,#20646,#20647,#20648),.UNSPECIFIED.,.F.,.F.,(4,3,3,
3,3,3,3,4),(-35.2649009415391,-34.7346944074771,-33.7422745672635,-32.7498547270498,
-31.7574348868362,-30.7650150466226,-29.772595206409,-28.9817156343595),
 .UNSPECIFIED.);
#2417=B_SPLINE_CURVE_WITH_KNOTS('',3,(#20653,#20654,#20655,#20656,#20657,
#20658,#20659,#20660,#20661,#20662,#20663,#20664,#20665,#20666,#20667,#20668,
#20669,#20670,#20671,#20672,#20673,#20674),.UNSPECIFIED.,.F.,.F.,(4,3,3,
3,3,3,3,4),(26.4423043696954,26.795335685768,27.7877555259817,28.7801753661953,
29.7725952064089,30.7650150466226,31.7574348868362,32.725489676875),
 .UNSPECIFIED.);
#2418=B_SPLINE_CURVE_WITH_KNOTS('',3,(#20675,#20676,#20677,#20678,#20679,
#20680,#20681,#20682,#20683,#20684,#20685,#20686,#20687,#20688,#20689,#20690,
#20691,#20692,#20693,#20694,#20695,#20696,#20697,#20698,#20699),
 .UNSPECIFIED.,.F.,.F.,(4,3,3,3,3,3,3,3,4),(-28.9817156343595,-28.7801753661953,
-27.7877555259817,-26.7953356857681,-25.8029158455544,-24.8104960053408,
-23.8180761651272,-22.8256563249135,-22.6985303271799),.UNSPECIFIED.);
#2419=B_SPLINE_CURVE_WITH_KNOTS('',3,(#20704,#20705,#20706,#20707,#20708,
#20709,#20710,#20711,#20712,#20713,#20714,#20715,#20716,#20717,#20718,#20719,
#20720,#20721,#20722,#20723,#20724,#20725),.UNSPECIFIED.,.F.,.F.,(4,3,3,
3,3,3,3,4),(20.1591190625158,20.8408166444862,21.8332364846999,22.8256563249135,
23.8180761651271,24.8104960053408,25.8029158455544,26.4423043696954),
 .UNSPECIFIED.);
#2420=B_SPLINE_CURVE_WITH_KNOTS('',3,(#20726,#20727,#20728,#20729,#20730,
#20731,#20732,#20733,#20734,#20735,#20736,#20737,#20738,#20739,#20740,#20741,
#20742,#20743,#20744,#20745,#20746,#20747),.UNSPECIFIED.,.F.,.F.,(4,3,3,
3,3,3,3,4),(-22.6985303271799,-21.8332364846999,-20.8408166444863,-19.8483968042726,
-18.855976964059,-17.8635571238454,-16.8711372836317,-16.4153450200003),
 .UNSPECIFIED.);
#2421=B_SPLINE_CURVE_WITH_KNOTS('',3,(#20752,#20753,#20754,#20755,#20756,
#20757,#20758,#20759,#20760,#20761,#20762,#20763,#20764,#20765,#20766,#20767,
#20768,#20769,#20770,#20771,#20772,#20773,#20774,#20775,#20776),
 .UNSPECIFIED.,.F.,.F.,(4,3,3,3,3,3,3,3,4),(13.8759337553362,13.8938777629908,
14.8862976032045,15.8787174434181,16.8711372836317,17.8635571238454,18.855976964059,
19.8483968042726,20.1591190625158),.UNSPECIFIED.);
#2422=B_SPLINE_CURVE_WITH_KNOTS('',3,(#20777,#20778,#20779,#20780,#20781,
#20782,#20783,#20784,#20785,#20786,#20787,#20788,#20789,#20790,#20791,#20792,
#20793,#20794,#20795,#20796,#20797,#20798),.UNSPECIFIED.,.F.,.F.,(4,3,3,
3,3,3,3,4),(-16.4153450200003,-15.8787174434181,-14.8862976032045,-13.8938777629908,
-12.9014579227772,-11.9090380825636,-10.9166182423499,-10.1321597128207),
 .UNSPECIFIED.);
#2423=B_SPLINE_CURVE_WITH_KNOTS('',3,(#20804,#20805,#20806,#20807,#20808,
#20809,#20810,#20811,#20812,#20813,#20814,#20815,#20816),.UNSPECIFIED.,
 .F.,.F.,(4,3,3,3,4),(-3.84897440564114,-2.9772595206409,-1.98483968042726,
-0.992419840213632,0.),.UNSPECIFIED.);
#2424=B_SPLINE_CURVE_WITH_KNOTS('',3,(#20819,#20820,#20821,#20822,#20823,
#20824,#20825,#20826,#20827,#20828,#20829,#20830,#20831,#20832,#20833,#20834,
#20835,#20836,#20837),.UNSPECIFIED.,.F.,.F.,(4,3,3,3,3,3,4),(2.01694489302841,
2.97725952064089,3.96967936085453,4.96209920106816,5.95451904128179,6.94693888149542,
7.59274844815661),.UNSPECIFIED.);
#2425=B_SPLINE_CURVE_WITH_KNOTS('',3,(#20843,#20844,#20845,#20846,#20847,
#20848,#20849,#20850),.UNSPECIFIED.,.F.,.F.,(4,1,1,1,1,4),(103.672557568463,
104.154034002175,105.146453842389,106.138873682603,107.131293522816,108.12371336303),
 .UNSPECIFIED.);
#2426=B_SPLINE_CURVE_WITH_KNOTS('',3,(#20853,#20854,#20855,#20856,#20857,
#20858,#20859,#20860,#20861),.UNSPECIFIED.,.F.,.F.,(4,1,1,1,1,1,4),(103.672557568463,
103.716185746199,104.708605586412,105.701025426626,106.693445266839,107.685865107053,
108.646179734666),.UNSPECIFIED.);
#2427=B_SPLINE_CURVE_WITH_KNOTS('',3,(#20866,#20867,#20868,#20869,#20870,
#20871,#20872,#20873,#20874,#20875),.UNSPECIFIED.,.F.,.F.,(4,1,1,1,1,1,
1,4),(97.3893722612836,98.1995149608937,99.1919348011073,100.184354641321,
101.176774481535,102.169194321748,103.161614161962,103.672557568463),
 .UNSPECIFIED.);
#2428=B_SPLINE_CURVE_WITH_KNOTS('',3,(#20876,#20877,#20878,#20879,#20880,
#20881,#20882,#20883,#20884,#20885),.UNSPECIFIED.,.F.,.F.,(4,1,1,1,1,1,
1,4),(97.3893722612836,97.7616667049168,98.7540865451304,99.7465063853441,
100.738926225558,101.731346065771,102.723765905985,103.672557568463),
 .UNSPECIFIED.);
#2429=B_SPLINE_CURVE_WITH_KNOTS('',3,(#20890,#20891,#20892,#20893,#20894,
#20895,#20896,#20897,#20898,#20899,#20900),.UNSPECIFIED.,.F.,.F.,(4,1,1,
1,1,1,1,1,4),(91.106186954104,91.2525760793983,92.2449959196119,93.2374157598255,
94.2298356000392,95.2222554402528,96.2146752804664,97.2070951206801,97.3893722612836),
 .UNSPECIFIED.);
#2430=B_SPLINE_CURVE_WITH_KNOTS('',3,(#20901,#20902,#20903,#20904,#20905,
#20906,#20907,#20908,#20909,#20910),.UNSPECIFIED.,.F.,.F.,(4,1,1,1,1,1,
1,4),(91.106186954104,91.807147663635,92.7995675038486,93.7919873440623,
94.7844071842759,95.7768270244895,96.7692468647032,97.3893722612836),
 .UNSPECIFIED.);
#2431=B_SPLINE_CURVE_WITH_KNOTS('',3,(#20915,#20916,#20917,#20918,#20919,
#20920,#20921,#20922,#20923,#20924),.UNSPECIFIED.,.F.,.F.,(4,1,1,1,1,1,
1,4),(84.8230016469244,85.2980570381165,86.2904768783301,87.2828967185437,
88.2753165587574,89.267736398971,90.2601562391846,91.106186954104),
 .UNSPECIFIED.);
#2432=B_SPLINE_CURVE_WITH_KNOTS('',3,(#20925,#20926,#20927,#20928,#20929,
#20930,#20931,#20932,#20933,#20934,#20935),.UNSPECIFIED.,.F.,.F.,(4,1,1,
1,1,1,1,1,4),(84.8230016469244,84.8602087821396,85.8526286223532,86.8450484625669,
87.8374683027805,88.8298881429941,89.8223079832078,90.8147278234214,91.106186954104),
 .UNSPECIFIED.);
#2433=B_SPLINE_CURVE_WITH_KNOTS('',3,(#20940,#20941,#20942,#20943,#20944,
#20945,#20946,#20947,#20948,#20949),.UNSPECIFIED.,.F.,.F.,(4,1,1,1,1,1,
1,4),(78.5398163397448,79.3435379968347,80.3359578370483,81.328377677262,
82.3207975174756,83.3132173576892,84.3056371979029,84.8230016469244),
 .UNSPECIFIED.);
#2434=B_SPLINE_CURVE_WITH_KNOTS('',3,(#20950,#20951,#20952,#20953,#20954,
#20955,#20956,#20957,#20958,#20959),.UNSPECIFIED.,.F.,.F.,(4,1,1,1,1,1,
1,4),(78.5398163397448,78.9056897408578,79.8981095810714,80.8905294212851,
81.8829492614987,82.8753691017123,83.867788941926,84.8230016469244),
 .UNSPECIFIED.);
#2435=B_SPLINE_CURVE_WITH_KNOTS('',3,(#20964,#20965,#20966,#20967,#20968,
#20969,#20970,#20971,#20972,#20973,#20974),.UNSPECIFIED.,.F.,.F.,(4,1,1,
1,1,1,1,1,4),(72.2566310325652,72.3965991153393,73.3890189555529,74.3814387957665,
75.3738586359802,76.3662784761938,77.3586983164074,78.3511181566211,78.5398163397448),
 .UNSPECIFIED.);
#2436=B_SPLINE_CURVE_WITH_KNOTS('',3,(#20975,#20976,#20977,#20978,#20979,
#20980,#20981,#20982,#20983,#20984),.UNSPECIFIED.,.F.,.F.,(4,1,1,1,1,1,
1,4),(72.2566310325652,72.951170699576,73.9435905397896,74.9360103800033,
75.9284302202169,76.9208500604305,77.9132699006442,78.5398163397448),
 .UNSPECIFIED.);
#2437=B_SPLINE_CURVE_WITH_KNOTS('',3,(#20989,#20990,#20991,#20992,#20993,
#20994,#20995,#20996,#20997,#20998),.UNSPECIFIED.,.F.,.F.,(4,1,1,1,1,1,
1,4),(65.9734457253856,66.4420800740575,67.4344999142711,68.4269197544847,
69.4193395946984,70.411759434912,71.4041792751256,72.2566310325652),
 .UNSPECIFIED.);
#2438=B_SPLINE_CURVE_WITH_KNOTS('',3,(#20999,#21000,#21001,#21002,#21003,
#21004,#21005,#21006,#21007,#21008,#21009),.UNSPECIFIED.,.F.,.F.,(4,1,1,
1,1,1,1,1,4),(65.9734457253856,66.0042318180806,66.9966516582942,67.9890714985079,
68.9814913387215,69.9739111789351,70.9663310191488,71.9587508593624,72.2566310325652),
 .UNSPECIFIED.);
#2439=B_SPLINE_CURVE_WITH_KNOTS('',3,(#21014,#21015,#21016,#21017,#21018,
#21019,#21020,#21021,#21022,#21023),.UNSPECIFIED.,.F.,.F.,(4,1,1,1,1,1,
1,4),(59.690260418206,60.4875610327757,61.4799808729893,62.4724007132029,
63.4648205534166,64.4572403936302,65.4496602338438,65.9734457253856),
 .UNSPECIFIED.);
#2440=B_SPLINE_CURVE_WITH_KNOTS('',3,(#21024,#21025,#21026,#21027,#21028,
#21029,#21030,#21031,#21032,#21033),.UNSPECIFIED.,.F.,.F.,(4,1,1,1,1,1,
1,4),(59.690260418206,60.0497127767988,61.0421326170124,62.0345524572261,
63.0269722974397,64.0193921376533,65.011811977867,65.9734457253856),
 .UNSPECIFIED.);
#2441=B_SPLINE_CURVE_WITH_KNOTS('',3,(#21038,#21039,#21040,#21041,#21042,
#21043,#21044,#21045,#21046,#21047,#21048),.UNSPECIFIED.,.F.,.F.,(4,1,1,
1,1,1,1,1,4),(53.4070751110264,53.5406221512803,54.5330419914939,55.5254618317075,
56.5178816719212,57.5103015121348,58.5027213523484,59.4951411925621,59.690260418206),
 .UNSPECIFIED.);
#2442=B_SPLINE_CURVE_WITH_KNOTS('',3,(#21049,#21050,#21051,#21052,#21053,
#21054,#21055,#21056,#21057,#21058),.UNSPECIFIED.,.F.,.F.,(4,1,1,1,1,1,
1,4),(53.4070751110264,54.095193735517,55.0876135757306,56.0800334159443,
57.0724532561579,58.0648730963715,59.0572929365852,59.690260418206),
 .UNSPECIFIED.);
#2443=B_SPLINE_CURVE_WITH_KNOTS('',3,(#21063,#21064,#21065,#21066,#21067,
#21068,#21069,#21070,#21071,#21072),.UNSPECIFIED.,.F.,.F.,(4,1,1,1,1,1,
1,4),(47.1238898038468,47.5861031099985,48.5785229502121,49.5709427904257,
50.5633626306394,51.555782470853,52.5482023110666,53.4070751110264),
 .UNSPECIFIED.);
#2444=B_SPLINE_CURVE_WITH_KNOTS('',3,(#21073,#21074,#21075,#21076,#21077,
#21078,#21079,#21080,#21081,#21082,#21083),.UNSPECIFIED.,.F.,.F.,(4,1,1,
1,1,1,1,1,4),(47.1238898038468,47.1482548540216,48.1406746942352,49.1330945344489,
50.1255143746625,51.1179342148761,52.1103540550898,53.1027738953034,53.4070751110264),
 .UNSPECIFIED.);
#2445=B_SPLINE_CURVE_WITH_KNOTS('',3,(#21088,#21089,#21090,#21091,#21092,
#21093,#21094,#21095,#21096,#21097),.UNSPECIFIED.,.F.,.F.,(4,1,1,1,1,1,
1,4),(40.8407044966672,41.6315840687167,42.6240039089303,43.6164237491439,
44.6088435893576,45.6012634295712,46.5936832697848,47.1238898038468),
 .UNSPECIFIED.);
#2446=B_SPLINE_CURVE_WITH_KNOTS('',3,(#21098,#21099,#21100,#21101,#21102,
#21103,#21104,#21105,#21106,#21107),.UNSPECIFIED.,.F.,.F.,(4,1,1,1,1,1,
1,4),(40.8407044966672,41.1937358127398,42.1861556529534,43.1785754931671,
44.1709953333807,45.1634151735943,46.155835013808,47.1238898038468),
 .UNSPECIFIED.);
#2447=B_SPLINE_CURVE_WITH_KNOTS('',3,(#21112,#21113,#21114,#21115,#21116,
#21117,#21118,#21119,#21120,#21121,#21122),.UNSPECIFIED.,.F.,.F.,(4,1,1,
1,1,1,1,1,4),(34.5575191894876,34.6846451872213,35.6770650274349,36.6694848676485,
37.6619047078622,38.6543245480758,39.6467443882894,40.639164228503,40.8407044966672),
 .UNSPECIFIED.);
#2448=B_SPLINE_CURVE_WITH_KNOTS('',3,(#21123,#21124,#21125,#21126,#21127,
#21128,#21129,#21130,#21131,#21132),.UNSPECIFIED.,.F.,.F.,(4,1,1,1,1,1,
1,4),(34.5575191894876,35.239216771458,36.2316366116717,37.2240564518853,
38.2164762920989,39.2088961323126,40.2013159725262,40.8407044966672),
 .UNSPECIFIED.);
#2449=B_SPLINE_CURVE_WITH_KNOTS('',3,(#21137,#21138,#21139,#21140,#21141,
#21142,#21143,#21144,#21145,#21146),.UNSPECIFIED.,.F.,.F.,(4,1,1,1,1,1,
1,4),(28.274333882308,28.7301261459395,29.7225459861531,30.7149658263667,
31.7073856665804,32.699805506794,33.6922253470076,34.5575191894876),
 .UNSPECIFIED.);
#2450=B_SPLINE_CURVE_WITH_KNOTS('',3,(#21147,#21148,#21149,#21150,#21151,
#21152,#21153,#21154,#21155,#21156,#21157),.UNSPECIFIED.,.F.,.F.,(4,1,1,
1,1,1,1,1,4),(28.274333882308,28.2922778899626,29.2846977301762,30.2771175703899,
31.2695374106035,32.2619572508171,33.2543770910308,34.2467969312444,34.5575191894876),
 .UNSPECIFIED.);
#2451=B_SPLINE_CURVE_WITH_KNOTS('',3,(#21162,#21163,#21164,#21165,#21166,
#21167,#21168,#21169,#21170,#21171),.UNSPECIFIED.,.F.,.F.,(4,1,1,1,1,1,
1,4),(21.9911485751285,22.7756071046577,23.7680269448713,24.7604467850849,
25.7528666252986,26.7452864655122,27.7377063057258,28.274333882308),
 .UNSPECIFIED.);
#2452=B_SPLINE_CURVE_WITH_KNOTS('',3,(#21172,#21173,#21174,#21175,#21176,
#21177,#21178,#21179,#21180,#21181),.UNSPECIFIED.,.F.,.F.,(4,1,1,1,1,1,
1,4),(21.9911485751285,22.3377588486808,23.3301786888945,24.3225985291081,
25.3150183693217,26.3074382095353,27.299858049749,28.274333882308),
 .UNSPECIFIED.);
#2453=B_SPLINE_CURVE_WITH_KNOTS('',3,(#21187,#21188,#21189,#21190,#21191),
 .UNSPECIFIED.,.F.,.F.,(4,1,4),(14.3984001269718,15.3908199671854,15.7079632679489),
 .UNSPECIFIED.);
#2454=B_SPLINE_CURVE_WITH_KNOTS('',3,(#21194,#21195,#21196,#21197,#21198),
 .UNSPECIFIED.,.F.,.F.,(4,1,4),(13.8759337553362,14.8362483829486,15.7079632679489),
 .UNSPECIFIED.);
#2455=B_SPLINE_CURVE_WITH_KNOTS('',3,(#21204,#21205,#21206,#21207),
 .UNSPECIFIED.,.F.,.F.,(4,4),(95.5573427486709,96.2647245007222),
 .UNSPECIFIED.);
#2456=B_SPLINE_CURVE_WITH_KNOTS('',3,(#21215,#21216,#21217,#21218,#21219,
#21220,#21221,#21222,#21223,#21224),.UNSPECIFIED.,.F.,.F.,(4,3,3,4),(-94.2477796076938,
-93.2874649800814,-92.2950451398678,-91.8135687061554),.UNSPECIFIED.);
#2457=B_SPLINE_CURVE_WITH_KNOTS('',3,(#21229,#21230,#21231,#21232,#21233,
#21234,#21235,#21236,#21237,#21238,#21239,#21240,#21241,#21242,#21243,#21244,
#21245,#21246,#21247,#21248,#21249,#21250,#21251,#21252,#21253),
 .UNSPECIFIED.,.F.,.F.,(4,3,3,3,3,3,3,3,4),(89.2741574414913,89.3177856192268,
90.3102054594404,91.3026252996541,92.2950451398677,93.2874649800813,94.279884820295,
95.2723046605086,95.5573427486709),.UNSPECIFIED.);
#2458=B_SPLINE_CURVE_WITH_KNOTS('',3,(#21254,#21255,#21256,#21257,#21258,
#21259,#21260,#21261,#21262,#21263,#21264,#21265,#21266,#21267,#21268,#21269,
#21270,#21271,#21272,#21273,#21274,#21275),.UNSPECIFIED.,.F.,.F.,(4,3,3,
3,3,3,3,4),(-91.8135687061554,-91.3026252996541,-90.3102054594405,-89.3177856192269,
-88.3253657790132,-87.3329459387996,-86.340526098586,-85.5303833989758),
 .UNSPECIFIED.);
#2459=B_SPLINE_CURVE_WITH_KNOTS('',3,(#21280,#21281,#21282,#21283,#21284,
#21285,#21286,#21287,#21288,#21289,#21290,#21291,#21292,#21293,#21294,#21295,
#21296,#21297,#21298,#21299,#21300,#21301),.UNSPECIFIED.,.F.,.F.,(4,3,3,
3,3,3,3,4),(82.9909721343117,83.363266577945,84.3556864181587,85.3481062583723,
86.3405260985859,87.3329459387996,88.3253657790132,89.2741574414913),
 .UNSPECIFIED.);
#2460=B_SPLINE_CURVE_WITH_KNOTS('',3,(#21302,#21303,#21304,#21305,#21306,
#21307,#21308,#21309,#21310,#21311,#21312,#21313,#21314,#21315,#21316,#21317,
#21318,#21319,#21320,#21321,#21322,#21323,#21324,#21325,#21326),
 .UNSPECIFIED.,.F.,.F.,(4,3,3,3,3,3,3,3,4),(-85.5303833989758,-85.3481062583723,
-84.3556864181587,-83.3632665779451,-82.3708467377314,-81.3784268975178,
-80.3860070573042,-79.3935872170905,-79.2471980917962),.UNSPECIFIED.);
#2461=B_SPLINE_CURVE_WITH_KNOTS('',3,(#21331,#21332,#21333,#21334,#21335,
#21336,#21337,#21338,#21339,#21340,#21341,#21342,#21343,#21344,#21345,#21346,
#21347,#21348,#21349,#21350,#21351,#21352),.UNSPECIFIED.,.F.,.F.,(4,3,3,
3,3,3,3,4),(76.7077868271321,77.4087475366632,78.4011673768769,79.3935872170905,
80.3860070573041,81.3784268975178,82.3708467377314,82.9909721343117),
 .UNSPECIFIED.);
#2462=B_SPLINE_CURVE_WITH_KNOTS('',3,(#21353,#21354,#21355,#21356,#21357,
#21358,#21359,#21360,#21361,#21362,#21363,#21364,#21365,#21366,#21367,#21368,
#21369,#21370,#21371,#21372,#21373,#21374),.UNSPECIFIED.,.F.,.F.,(4,3,3,
3,3,3,3,4),(-79.2471980917962,-78.4011673768769,-77.4087475366633,-76.4163276964496,
-75.423907856236,-74.4314880160224,-73.4390681758088,-72.9640127846167),
 .UNSPECIFIED.);
#2463=B_SPLINE_CURVE_WITH_KNOTS('',3,(#21379,#21380,#21381,#21382,#21383,
#21384,#21385,#21386,#21387,#21388,#21389,#21390,#21391,#21392,#21393,#21394,
#21395,#21396,#21397,#21398,#21399,#21400,#21401,#21402,#21403),
 .UNSPECIFIED.,.F.,.F.,(4,3,3,3,3,3,3,3,4),(70.4246015199525,70.4618086551678,
71.4542284953814,72.4466483355951,73.4390681758087,74.4314880160223,75.423907856236,
76.4163276964496,76.7077868271321),.UNSPECIFIED.);
#2464=B_SPLINE_CURVE_WITH_KNOTS('',3,(#21404,#21405,#21406,#21407,#21408,
#21409,#21410,#21411,#21412,#21413,#21414,#21415,#21416,#21417,#21418,#21419,
#21420,#21421,#21422,#21423,#21424,#21425),.UNSPECIFIED.,.F.,.F.,(4,3,3,
3,3,3,3,4),(-72.9640127846167,-72.4466483355951,-71.4542284953815,-70.4618086551678,
-69.4693888149542,-68.4769689747406,-67.4845491345269,-66.680827477437),
 .UNSPECIFIED.);
#2465=B_SPLINE_CURVE_WITH_KNOTS('',3,(#21430,#21431,#21432,#21433,#21434,
#21435,#21436,#21437,#21438,#21439,#21440,#21441,#21442,#21443,#21444,#21445,
#21446,#21447,#21448,#21449,#21450,#21451),.UNSPECIFIED.,.F.,.F.,(4,3,3,
3,3,3,3,4),(64.1414162127729,64.507289613886,65.4997094540997,66.4921292943133,
67.4845491345269,68.4769689747405,69.4693888149542,70.4246015199525),
 .UNSPECIFIED.);
#2466=B_SPLINE_CURVE_WITH_KNOTS('',3,(#21452,#21453,#21454,#21455,#21456,
#21457,#21458,#21459,#21460,#21461,#21462,#21463,#21464,#21465,#21466,#21467,
#21468,#21469,#21470,#21471,#21472,#21473,#21474,#21475,#21476),
 .UNSPECIFIED.,.F.,.F.,(4,3,3,3,3,3,3,3,4),(-66.680827477437,-66.4921292943133,
-65.4997094540997,-64.5072896138861,-63.5148697736724,-62.5224499334588,
-61.5300300932452,-60.5376102530315,-60.3976421702575),.UNSPECIFIED.);
#2467=B_SPLINE_CURVE_WITH_KNOTS('',3,(#21481,#21482,#21483,#21484,#21485,
#21486,#21487,#21488,#21489,#21490,#21491,#21492,#21493,#21494,#21495,#21496,
#21497,#21498,#21499,#21500,#21501,#21502),.UNSPECIFIED.,.F.,.F.,(4,3,3,
3,3,3,3,4),(57.8582309055933,58.5527705726042,59.5451904128179,60.5376102530315,
61.5300300932451,62.5224499334588,63.5148697736724,64.1414162127729),
 .UNSPECIFIED.);
#2468=B_SPLINE_CURVE_WITH_KNOTS('',3,(#21503,#21504,#21505,#21506,#21507,
#21508,#21509,#21510,#21511,#21512,#21513,#21514,#21515,#21516,#21517,#21518,
#21519,#21520,#21521,#21522,#21523,#21524),.UNSPECIFIED.,.F.,.F.,(4,3,3,
3,3,3,3,4),(-60.3976421702575,-59.5451904128179,-58.5527705726043,-57.5603507323906,
-56.567930892177,-55.5755110519634,-54.5830912117497,-54.1144568630779),
 .UNSPECIFIED.);
#2469=B_SPLINE_CURVE_WITH_KNOTS('',3,(#21529,#21530,#21531,#21532,#21533,
#21534,#21535,#21536,#21537,#21538,#21539,#21540,#21541,#21542,#21543,#21544,
#21545,#21546,#21547,#21548,#21549,#21550,#21551,#21552,#21553),
 .UNSPECIFIED.,.F.,.F.,(4,3,3,3,3,3,3,3,4),(51.5750455984138,51.6058316911088,
52.5982515313225,53.5906713715361,54.5830912117497,55.5755110519634,56.567930892177,
57.5603507323906,57.8582309055933),.UNSPECIFIED.);
#2470=B_SPLINE_CURVE_WITH_KNOTS('',3,(#21554,#21555,#21556,#21557,#21558,
#21559,#21560,#21561,#21562,#21563,#21564,#21565,#21566,#21567,#21568,#21569,
#21570,#21571,#21572,#21573,#21574,#21575),.UNSPECIFIED.,.F.,.F.,(4,3,3,
3,3,3,3,4),(-54.1144568630779,-53.5906713715361,-52.5982515313225,-51.6058316911088,
-50.6134118508952,-49.6209920106816,-48.6285721704679,-47.8312715558983),
 .UNSPECIFIED.);
#2471=B_SPLINE_CURVE_WITH_KNOTS('',3,(#21580,#21581,#21582,#21583,#21584,
#21585,#21586,#21587,#21588,#21589,#21590,#21591,#21592,#21593,#21594,#21595,
#21596,#21597,#21598,#21599,#21600,#21601),.UNSPECIFIED.,.F.,.F.,(4,3,3,
3,3,3,3,4),(45.2918602912342,45.651312649827,46.6437324900407,47.6361523302543,
48.6285721704679,49.6209920106816,50.6134118508952,51.5750455984138),
 .UNSPECIFIED.);
#2472=B_SPLINE_CURVE_WITH_KNOTS('',3,(#21602,#21603,#21604,#21605,#21606,
#21607,#21608,#21609,#21610,#21611,#21612,#21613,#21614,#21615,#21616,#21617,
#21618,#21619,#21620,#21621,#21622,#21623,#21624,#21625,#21626),
 .UNSPECIFIED.,.F.,.F.,(4,3,3,3,3,3,3,3,4),(-47.8312715558983,-47.6361523302543,
-46.6437324900407,-45.651312649827,-44.6588928096134,-43.6664729693998,
-42.6740531291862,-41.6816332889725,-41.5480862487187),.UNSPECIFIED.);
#2473=B_SPLINE_CURVE_WITH_KNOTS('',3,(#21631,#21632,#21633,#21634,#21635,
#21636,#21637,#21638,#21639,#21640,#21641,#21642,#21643,#21644,#21645,#21646,
#21647,#21648,#21649,#21650,#21651,#21652),.UNSPECIFIED.,.F.,.F.,(4,3,3,
3,3,3,3,4),(39.0086749840546,39.6967936085453,40.6892134487589,41.6816332889725,
42.6740531291861,43.6664729693998,44.6588928096134,45.2918602912342),
 .UNSPECIFIED.);
#2474=B_SPLINE_CURVE_WITH_KNOTS('',3,(#21653,#21654,#21655,#21656,#21657,
#21658,#21659,#21660,#21661,#21662,#21663,#21664,#21665,#21666,#21667,#21668,
#21669,#21670,#21671,#21672,#21673,#21674),.UNSPECIFIED.,.F.,.F.,(4,3,3,
3,3,3,3,4),(-41.5480862487187,-40.6892134487589,-39.6967936085453,-38.7043737683316,
-37.711953928118,-36.7195340879044,-35.7271142476907,-35.2649009415391),
 .UNSPECIFIED.);
#2475=B_SPLINE_CURVE_WITH_KNOTS('',3,(#21679,#21680,#21681,#21682,#21683,
#21684,#21685,#21686,#21687,#21688,#21689,#21690,#21691,#21692,#21693,#21694,
#21695,#21696,#21697,#21698,#21699,#21700,#21701,#21702,#21703),
 .UNSPECIFIED.,.F.,.F.,(4,3,3,3,3,3,3,3,4),(32.725489676875,32.7498547270498,
33.7422745672635,34.7346944074771,35.7271142476907,36.7195340879043,37.711953928118,
38.7043737683316,39.0086749840546),.UNSPECIFIED.);
#2476=B_SPLINE_CURVE_WITH_KNOTS('',3,(#21704,#21705,#21706,#21707,#21708,
#21709,#21710,#21711,#21712,#21713,#21714,#21715,#21716,#21717,#21718,#21719,
#21720,#21721,#21722,#21723,#21724,#21725),.UNSPECIFIED.,.F.,.F.,(4,3,3,
3,3,3,3,4),(-35.2649009415391,-34.7346944074771,-33.7422745672635,-32.7498547270498,
-31.7574348868362,-30.7650150466226,-29.7725952064089,-28.9817156343595),
 .UNSPECIFIED.);
#2477=B_SPLINE_CURVE_WITH_KNOTS('',3,(#21730,#21731,#21732,#21733,#21734,
#21735,#21736,#21737,#21738,#21739,#21740,#21741,#21742,#21743,#21744,#21745,
#21746,#21747,#21748,#21749,#21750,#21751),.UNSPECIFIED.,.F.,.F.,(4,3,3,
3,3,3,3,4),(26.4423043696954,26.795335685768,27.7877555259817,28.7801753661953,
29.7725952064089,30.7650150466226,31.7574348868362,32.725489676875),
 .UNSPECIFIED.);
#2478=B_SPLINE_CURVE_WITH_KNOTS('',3,(#21752,#21753,#21754,#21755,#21756,
#21757,#21758,#21759,#21760,#21761,#21762,#21763,#21764,#21765,#21766,#21767,
#21768,#21769,#21770,#21771,#21772,#21773,#21774,#21775,#21776),
 .UNSPECIFIED.,.F.,.F.,(4,3,3,3,3,3,3,3,4),(-28.9817156343595,-28.7801753661953,
-27.7877555259817,-26.7953356857681,-25.8029158455544,-24.8104960053408,
-23.8180761651272,-22.8256563249135,-22.6985303271799),.UNSPECIFIED.);
#2479=B_SPLINE_CURVE_WITH_KNOTS('',3,(#21781,#21782,#21783,#21784,#21785,
#21786,#21787,#21788,#21789,#21790,#21791,#21792,#21793,#21794,#21795,#21796,
#21797,#21798,#21799,#21800,#21801,#21802),.UNSPECIFIED.,.F.,.F.,(4,3,3,
3,3,3,3,4),(20.1591190625158,20.8408166444863,21.8332364846999,22.8256563249135,
23.8180761651272,24.8104960053408,25.8029158455544,26.4423043696954),
 .UNSPECIFIED.);
#2480=B_SPLINE_CURVE_WITH_KNOTS('',3,(#21803,#21804,#21805,#21806,#21807,
#21808,#21809,#21810,#21811,#21812,#21813,#21814,#21815,#21816,#21817,#21818,
#21819,#21820,#21821,#21822,#21823,#21824),.UNSPECIFIED.,.F.,.F.,(4,3,3,
3,3,3,3,4),(-22.6985303271799,-21.8332364846999,-20.8408166444863,-19.8483968042726,
-18.855976964059,-17.8635571238454,-16.8711372836317,-16.4153450200003),
 .UNSPECIFIED.);
#2481=B_SPLINE_CURVE_WITH_KNOTS('',3,(#21829,#21830,#21831,#21832,#21833,
#21834,#21835,#21836,#21837,#21838,#21839,#21840,#21841,#21842,#21843,#21844,
#21845,#21846,#21847,#21848,#21849,#21850,#21851,#21852,#21853),
 .UNSPECIFIED.,.F.,.F.,(4,3,3,3,3,3,3,3,4),(13.8759337553362,13.8938777629908,
14.8862976032045,15.8787174434181,16.8711372836317,17.8635571238454,18.855976964059,
19.8483968042726,20.1591190625158),.UNSPECIFIED.);
#2482=B_SPLINE_CURVE_WITH_KNOTS('',3,(#21854,#21855,#21856,#21857,#21858,
#21859,#21860,#21861,#21862,#21863,#21864,#21865,#21866,#21867,#21868,#21869,
#21870,#21871,#21872,#21873,#21874,#21875),.UNSPECIFIED.,.F.,.F.,(4,3,3,
3,3,3,3,4),(-16.4153450200003,-15.8787174434181,-14.8862976032045,-13.8938777629908,
-12.9014579227772,-11.9090380825636,-10.9166182423499,-10.1321597128207),
 .UNSPECIFIED.);
#2483=B_SPLINE_CURVE_WITH_KNOTS('',3,(#21881,#21882,#21883,#21884,#21885,
#21886,#21887,#21888,#21889,#21890,#21891,#21892,#21893),.UNSPECIFIED.,
 .F.,.F.,(4,3,3,3,4),(-3.84897440564114,-2.9772595206409,-1.98483968042726,
-0.992419840213631,0.),.UNSPECIFIED.);
#2484=B_SPLINE_CURVE_WITH_KNOTS('',3,(#21896,#21897,#21898,#21899,#21900,
#21901,#21902,#21903,#21904,#21905,#21906,#21907,#21908,#21909,#21910,#21911,
#21912,#21913,#21914),.UNSPECIFIED.,.F.,.F.,(4,3,3,3,3,3,4),(2.01694489302841,
2.97725952064089,3.96967936085452,4.96209920106815,5.95451904128178,6.94693888149541,
7.59274844815661),.UNSPECIFIED.);
#2485=B_SPLINE_CURVE_WITH_KNOTS('',3,(#21920,#21921,#21922,#21923,#21924,
#21925,#21926,#21927),.UNSPECIFIED.,.F.,.F.,(4,1,1,1,1,4),(103.672557568463,
104.154034002175,105.146453842389,106.138873682603,107.131293522816,108.12371336303),
 .UNSPECIFIED.);
#2486=B_SPLINE_CURVE_WITH_KNOTS('',3,(#21930,#21931,#21932,#21933,#21934,
#21935,#21936,#21937,#21938),.UNSPECIFIED.,.F.,.F.,(4,1,1,1,1,1,4),(103.672557568463,
103.716185746199,104.708605586412,105.701025426626,106.693445266839,107.685865107053,
108.646179734666),.UNSPECIFIED.);
#2487=B_SPLINE_CURVE_WITH_KNOTS('',3,(#21943,#21944,#21945,#21946,#21947,
#21948,#21949,#21950,#21951,#21952),.UNSPECIFIED.,.F.,.F.,(4,1,1,1,1,1,
1,4),(97.3893722612836,98.1995149608937,99.1919348011073,100.184354641321,
101.176774481535,102.169194321748,103.161614161962,103.672557568463),
 .UNSPECIFIED.);
#2488=B_SPLINE_CURVE_WITH_KNOTS('',3,(#21953,#21954,#21955,#21956,#21957,
#21958,#21959,#21960,#21961,#21962),.UNSPECIFIED.,.F.,.F.,(4,1,1,1,1,1,
1,4),(97.3893722612836,97.7616667049168,98.7540865451304,99.7465063853441,
100.738926225558,101.731346065771,102.723765905985,103.672557568463),
 .UNSPECIFIED.);
#2489=B_SPLINE_CURVE_WITH_KNOTS('',3,(#21967,#21968,#21969,#21970,#21971,
#21972,#21973,#21974,#21975,#21976,#21977),.UNSPECIFIED.,.F.,.F.,(4,1,1,
1,1,1,1,1,4),(91.106186954104,91.2525760793983,92.2449959196119,93.2374157598255,
94.2298356000392,95.2222554402528,96.2146752804664,97.2070951206801,97.3893722612836),
 .UNSPECIFIED.);
#2490=B_SPLINE_CURVE_WITH_KNOTS('',3,(#21978,#21979,#21980,#21981,#21982,
#21983,#21984,#21985,#21986,#21987),.UNSPECIFIED.,.F.,.F.,(4,1,1,1,1,1,
1,4),(91.106186954104,91.807147663635,92.7995675038486,93.7919873440623,
94.7844071842759,95.7768270244895,96.7692468647032,97.3893722612836),
 .UNSPECIFIED.);
#2491=B_SPLINE_CURVE_WITH_KNOTS('',3,(#21992,#21993,#21994,#21995,#21996,
#21997,#21998,#21999,#22000,#22001),.UNSPECIFIED.,.F.,.F.,(4,1,1,1,1,1,
1,4),(84.8230016469244,85.2980570381165,86.2904768783301,87.2828967185437,
88.2753165587574,89.267736398971,90.2601562391846,91.106186954104),
 .UNSPECIFIED.);
#2492=B_SPLINE_CURVE_WITH_KNOTS('',3,(#22002,#22003,#22004,#22005,#22006,
#22007,#22008,#22009,#22010,#22011,#22012),.UNSPECIFIED.,.F.,.F.,(4,1,1,
1,1,1,1,1,4),(84.8230016469244,84.8602087821396,85.8526286223532,86.8450484625669,
87.8374683027805,88.8298881429941,89.8223079832078,90.8147278234214,91.106186954104),
 .UNSPECIFIED.);
#2493=B_SPLINE_CURVE_WITH_KNOTS('',3,(#22017,#22018,#22019,#22020,#22021,
#22022,#22023,#22024,#22025,#22026),.UNSPECIFIED.,.F.,.F.,(4,1,1,1,1,1,
1,4),(78.5398163397448,79.3435379968347,80.3359578370483,81.328377677262,
82.3207975174756,83.3132173576892,84.3056371979029,84.8230016469244),
 .UNSPECIFIED.);
#2494=B_SPLINE_CURVE_WITH_KNOTS('',3,(#22027,#22028,#22029,#22030,#22031,
#22032,#22033,#22034,#22035,#22036),.UNSPECIFIED.,.F.,.F.,(4,1,1,1,1,1,
1,4),(78.5398163397448,78.9056897408578,79.8981095810714,80.8905294212851,
81.8829492614987,82.8753691017123,83.867788941926,84.8230016469244),
 .UNSPECIFIED.);
#2495=B_SPLINE_CURVE_WITH_KNOTS('',3,(#22041,#22042,#22043,#22044,#22045,
#22046,#22047,#22048,#22049,#22050,#22051),.UNSPECIFIED.,.F.,.F.,(4,1,1,
1,1,1,1,1,4),(72.2566310325652,72.3965991153393,73.3890189555529,74.3814387957665,
75.3738586359802,76.3662784761938,77.3586983164074,78.3511181566211,78.5398163397448),
 .UNSPECIFIED.);
#2496=B_SPLINE_CURVE_WITH_KNOTS('',3,(#22052,#22053,#22054,#22055,#22056,
#22057,#22058,#22059,#22060,#22061),.UNSPECIFIED.,.F.,.F.,(4,1,1,1,1,1,
1,4),(72.2566310325652,72.951170699576,73.9435905397896,74.9360103800033,
75.9284302202169,76.9208500604305,77.9132699006442,78.5398163397448),
 .UNSPECIFIED.);
#2497=B_SPLINE_CURVE_WITH_KNOTS('',3,(#22066,#22067,#22068,#22069,#22070,
#22071,#22072,#22073,#22074,#22075),.UNSPECIFIED.,.F.,.F.,(4,1,1,1,1,1,
1,4),(65.9734457253856,66.4420800740575,67.4344999142711,68.4269197544847,
69.4193395946984,70.411759434912,71.4041792751256,72.2566310325652),
 .UNSPECIFIED.);
#2498=B_SPLINE_CURVE_WITH_KNOTS('',3,(#22076,#22077,#22078,#22079,#22080,
#22081,#22082,#22083,#22084,#22085,#22086),.UNSPECIFIED.,.F.,.F.,(4,1,1,
1,1,1,1,1,4),(65.9734457253856,66.0042318180806,66.9966516582942,67.9890714985079,
68.9814913387215,69.9739111789351,70.9663310191488,71.9587508593624,72.2566310325652),
 .UNSPECIFIED.);
#2499=B_SPLINE_CURVE_WITH_KNOTS('',3,(#22091,#22092,#22093,#22094,#22095,
#22096,#22097,#22098,#22099,#22100),.UNSPECIFIED.,.F.,.F.,(4,1,1,1,1,1,
1,4),(59.690260418206,60.4875610327757,61.4799808729893,62.4724007132029,
63.4648205534166,64.4572403936302,65.4496602338438,65.9734457253856),
 .UNSPECIFIED.);
#2500=B_SPLINE_CURVE_WITH_KNOTS('',3,(#22101,#22102,#22103,#22104,#22105,
#22106,#22107,#22108,#22109,#22110),.UNSPECIFIED.,.F.,.F.,(4,1,1,1,1,1,
1,4),(59.690260418206,60.0497127767988,61.0421326170124,62.0345524572261,
63.0269722974397,64.0193921376533,65.011811977867,65.9734457253856),
 .UNSPECIFIED.);
#2501=B_SPLINE_CURVE_WITH_KNOTS('',3,(#22115,#22116,#22117,#22118,#22119,
#22120,#22121,#22122,#22123,#22124,#22125),.UNSPECIFIED.,.F.,.F.,(4,1,1,
1,1,1,1,1,4),(53.4070751110264,53.5406221512803,54.5330419914939,55.5254618317075,
56.5178816719212,57.5103015121348,58.5027213523484,59.4951411925621,59.690260418206),
 .UNSPECIFIED.);
#2502=B_SPLINE_CURVE_WITH_KNOTS('',3,(#22126,#22127,#22128,#22129,#22130,
#22131,#22132,#22133,#22134,#22135),.UNSPECIFIED.,.F.,.F.,(4,1,1,1,1,1,
1,4),(53.4070751110264,54.095193735517,55.0876135757306,56.0800334159443,
57.0724532561579,58.0648730963715,59.0572929365852,59.690260418206),
 .UNSPECIFIED.);
#2503=B_SPLINE_CURVE_WITH_KNOTS('',3,(#22140,#22141,#22142,#22143,#22144,
#22145,#22146,#22147,#22148,#22149),.UNSPECIFIED.,.F.,.F.,(4,1,1,1,1,1,
1,4),(47.1238898038468,47.5861031099985,48.5785229502121,49.5709427904257,
50.5633626306394,51.555782470853,52.5482023110666,53.4070751110264),
 .UNSPECIFIED.);
#2504=B_SPLINE_CURVE_WITH_KNOTS('',3,(#22150,#22151,#22152,#22153,#22154,
#22155,#22156,#22157,#22158,#22159,#22160),.UNSPECIFIED.,.F.,.F.,(4,1,1,
1,1,1,1,1,4),(47.1238898038468,47.1482548540216,48.1406746942352,49.1330945344489,
50.1255143746625,51.1179342148761,52.1103540550898,53.1027738953034,53.4070751110264),
 .UNSPECIFIED.);
#2505=B_SPLINE_CURVE_WITH_KNOTS('',3,(#22165,#22166,#22167,#22168,#22169,
#22170,#22171,#22172,#22173,#22174),.UNSPECIFIED.,.F.,.F.,(4,1,1,1,1,1,
1,4),(40.8407044966672,41.6315840687167,42.6240039089303,43.6164237491439,
44.6088435893576,45.6012634295712,46.5936832697848,47.1238898038468),
 .UNSPECIFIED.);
#2506=B_SPLINE_CURVE_WITH_KNOTS('',3,(#22175,#22176,#22177,#22178,#22179,
#22180,#22181,#22182,#22183,#22184),.UNSPECIFIED.,.F.,.F.,(4,1,1,1,1,1,
1,4),(40.8407044966673,41.1937358127398,42.1861556529534,43.1785754931671,
44.1709953333807,45.1634151735943,46.155835013808,47.1238898038468),
 .UNSPECIFIED.);
#2507=B_SPLINE_CURVE_WITH_KNOTS('',3,(#22189,#22190,#22191,#22192,#22193,
#22194,#22195,#22196,#22197,#22198,#22199),.UNSPECIFIED.,.F.,.F.,(4,1,1,
1,1,1,1,1,4),(34.5575191894876,34.6846451872213,35.6770650274349,36.6694848676485,
37.6619047078622,38.6543245480758,39.6467443882894,40.639164228503,40.8407044966672),
 .UNSPECIFIED.);
#2508=B_SPLINE_CURVE_WITH_KNOTS('',3,(#22200,#22201,#22202,#22203,#22204,
#22205,#22206,#22207,#22208,#22209),.UNSPECIFIED.,.F.,.F.,(4,1,1,1,1,1,
1,4),(34.5575191894877,35.239216771458,36.2316366116717,37.2240564518853,
38.2164762920989,39.2088961323126,40.2013159725262,40.8407044966673),
 .UNSPECIFIED.);
#2509=B_SPLINE_CURVE_WITH_KNOTS('',3,(#22214,#22215,#22216,#22217,#22218,
#22219,#22220,#22221,#22222,#22223),.UNSPECIFIED.,.F.,.F.,(4,1,1,1,1,1,
1,4),(28.274333882308,28.7301261459395,29.7225459861531,30.7149658263667,
31.7073856665804,32.699805506794,33.6922253470076,34.5575191894876),
 .UNSPECIFIED.);
#2510=B_SPLINE_CURVE_WITH_KNOTS('',3,(#22224,#22225,#22226,#22227,#22228,
#22229,#22230,#22231,#22232,#22233,#22234),.UNSPECIFIED.,.F.,.F.,(4,1,1,
1,1,1,1,1,4),(28.2743338823081,28.2922778899626,29.2846977301762,30.2771175703899,
31.2695374106035,32.2619572508171,33.2543770910308,34.2467969312444,34.5575191894877),
 .UNSPECIFIED.);
#2511=B_SPLINE_CURVE_WITH_KNOTS('',3,(#22239,#22240,#22241,#22242,#22243,
#22244,#22245,#22246,#22247,#22248),.UNSPECIFIED.,.F.,.F.,(4,1,1,1,1,1,
1,4),(21.9911485751285,22.7756071046577,23.7680269448713,24.7604467850849,
25.7528666252986,26.7452864655122,27.7377063057258,28.274333882308),
 .UNSPECIFIED.);
#2512=B_SPLINE_CURVE_WITH_KNOTS('',3,(#22249,#22250,#22251,#22252,#22253,
#22254,#22255,#22256,#22257,#22258),.UNSPECIFIED.,.F.,.F.,(4,1,1,1,1,1,
1,4),(21.9911485751285,22.3377588486808,23.3301786888945,24.3225985291081,
25.3150183693217,26.3074382095353,27.299858049749,28.2743338823081),
 .UNSPECIFIED.);
#2513=B_SPLINE_CURVE_WITH_KNOTS('',3,(#22264,#22265,#22266,#22267,#22268),
 .UNSPECIFIED.,.F.,.F.,(4,1,4),(14.3984001269718,15.3908199671854,15.7079632679489),
 .UNSPECIFIED.);
#2514=B_SPLINE_CURVE_WITH_KNOTS('',3,(#22271,#22272,#22273,#22274,#22275),
 .UNSPECIFIED.,.F.,.F.,(4,1,4),(13.8759337553362,14.8362483829486,15.7079632679489),
 .UNSPECIFIED.);
#2515=B_SPLINE_CURVE_WITH_KNOTS('',3,(#22281,#22282,#22283,#22284,#22285,
#22286,#22287,#22288,#22289,#22290,#22291,#22292,#22293,#22294,#22295,#22296,
#22297,#22298,#22299,#22300,#22301,#22302,#22303,#22304,#22305),
 .UNSPECIFIED.,.F.,.F.,(4,3,3,3,3,3,3,3,4),(-3.86106640140271,-3.4533318021373,
-2.95999868754626,-2.46666557295522,-1.97333245836417,-1.47999934377313,
-0.986666229182085,-0.493333114591042,0.),.UNSPECIFIED.);
#2516=B_SPLINE_CURVE_WITH_KNOTS('',3,(#22308,#22309,#22310,#22311,#22312,
#22313,#22314,#22315,#22316,#22317,#22318,#22319,#22320,#22321,#22322,#22323,
#22324,#22325,#22326,#22327,#22328,#22329,#22330,#22331,#22332,#22333,#22334,
#22335,#22336,#22337,#22338,#22339,#22340,#22341,#22342,#22343,#22344),
 .UNSPECIFIED.,.F.,.F.,(4,3,3,3,3,3,3,3,3,3,3,3,4),(2.02782768921384,2.46666557295522,
2.95999868754626,3.45333180213731,3.94666491672835,4.43999803131939,4.93333114591043,
5.42666426050148,5.91999737509252,6.41333048968356,6.90666360427461,7.39999671886565,
7.59153924858053),.UNSPECIFIED.);
#2517=B_SPLINE_CURVE_WITH_KNOTS('',3,(#22349,#22350,#22351,#22352,#22353,
#22354,#22355,#22356,#22357,#22358,#22359,#22360,#22361,#22362,#22363,#22364,
#22365,#22366,#22367,#22368,#22369,#22370,#22371,#22372,#22373,#22374,#22375,
#22376,#22377,#22378,#22379,#22380,#22381,#22382,#22383,#22384,#22385,#22386,
#22387,#22388,#22389,#22390,#22391),.UNSPECIFIED.,.F.,.F.,(4,3,3,3,3,3,
3,3,3,3,3,3,3,3,4),(-10.1442517085823,-9.86666229182086,-9.37332917722982,
-8.87999606263878,-8.38666294804773,-7.89332983345669,-7.39999671886565,
-6.9066636042746,-6.41333048968356,-5.91999737509252,-5.42666426050147,
-4.93333114591043,-4.43999803131939,-3.94666491672835,-3.86106640140271),
 .UNSPECIFIED.);
#2518=B_SPLINE_CURVE_WITH_KNOTS('',3,(#22392,#22393,#22394,#22395,#22396,
#22397,#22398,#22399,#22400,#22401,#22402,#22403,#22404,#22405,#22406,#22407,
#22408,#22409,#22410,#22411,#22412,#22413,#22414,#22415,#22416,#22417,#22418,
#22419,#22420,#22421,#22422,#22423,#22424,#22425,#22426,#22427,#22428,#22429,
#22430,#22431,#22432,#22433,#22434),.UNSPECIFIED.,.F.,.F.,(4,3,3,3,3,3,
3,3,3,3,3,3,3,3,4),(7.59153924858053,7.89332983345669,8.38666294804774,
8.87999606263878,9.37332917722982,9.86666229182087,10.3599954064119,10.853328521003,
11.346661635594,11.839994750185,12.3333278647761,12.8266609793671,13.3199940939582,
13.8133272085492,13.8747245557601),.UNSPECIFIED.);
#2519=B_SPLINE_CURVE_WITH_KNOTS('',3,(#22439,#22440,#22441,#22442,#22443,
#22444,#22445,#22446,#22447,#22448,#22449,#22450,#22451,#22452,#22453,#22454,
#22455,#22456,#22457,#22458,#22459,#22460,#22461,#22462,#22463,#22464,#22465,
#22466,#22467,#22468,#22469,#22470,#22471,#22472,#22473,#22474,#22475,#22476,
#22477,#22478,#22479,#22480,#22481),.UNSPECIFIED.,.F.,.F.,(4,3,3,3,3,3,
3,3,3,3,3,3,3,3,4),(-16.4274370157619,-16.2799927815044,-15.7866596669134,
-15.2933265523223,-14.7999934377313,-14.3066603231402,-13.8133272085492,
-13.3199940939582,-12.8266609793671,-12.3333278647761,-11.839994750185,
-11.346661635594,-10.8533285210029,-10.3599954064119,-10.1442517085823),
 .UNSPECIFIED.);
#2520=B_SPLINE_CURVE_WITH_KNOTS('',3,(#22482,#22483,#22484,#22485,#22486,
#22487,#22488,#22489,#22490,#22491,#22492,#22493,#22494,#22495,#22496,#22497,
#22498,#22499,#22500,#22501,#22502,#22503,#22504,#22505,#22506,#22507,#22508,
#22509,#22510,#22511,#22512,#22513,#22514,#22515,#22516,#22517,#22518,#22519,
#22520,#22521),.UNSPECIFIED.,.F.,.F.,(4,3,3,3,3,3,3,3,3,3,3,3,3,4),(13.8747245557601,
14.3066603231403,14.7999934377313,15.2933265523223,15.7866596669134,16.2799927815044,
16.7733258960955,17.2666590106865,17.7599921252775,18.2533252398686,18.7466583544596,
19.2399914690507,19.7333245836417,20.1579098629397),.UNSPECIFIED.);
#2521=B_SPLINE_CURVE_WITH_KNOTS('',3,(#22526,#22527,#22528,#22529,#22530,
#22531,#22532,#22533,#22534,#22535,#22536,#22537,#22538,#22539,#22540,#22541,
#22542,#22543,#22544,#22545,#22546,#22547,#22548,#22549,#22550,#22551,#22552,
#22553,#22554,#22555,#22556,#22557,#22558,#22559,#22560,#22561,#22562,#22563,
#22564,#22565,#22566,#22567,#22568),.UNSPECIFIED.,.F.,.F.,(4,3,3,3,3,3,
3,3,3,3,3,3,3,3,4),(-22.7106223229415,-22.693323271188,-22.1999901565969,
-21.7066570420059,-21.2133239274149,-20.7199908128238,-20.2266576982328,
-19.7333245836417,-19.2399914690507,-18.7466583544596,-18.2533252398686,
-17.7599921252776,-17.2666590106865,-16.7733258960955,-16.4274370157619),
 .UNSPECIFIED.);
#2522=B_SPLINE_CURVE_WITH_KNOTS('',3,(#22569,#22570,#22571,#22572,#22573,
#22574,#22575,#22576,#22577,#22578,#22579,#22580,#22581,#22582,#22583,#22584,
#22585,#22586,#22587,#22588,#22589,#22590,#22591,#22592,#22593,#22594,#22595,
#22596,#22597,#22598,#22599,#22600,#22601,#22602,#22603,#22604,#22605,#22606,
#22607,#22608,#22609,#22610,#22611),.UNSPECIFIED.,.F.,.F.,(4,3,3,3,3,3,
3,3,3,3,3,3,3,3,4),(20.1579098629397,20.2266576982328,20.7199908128238,
21.2133239274148,21.7066570420059,22.1999901565969,22.693323271188,23.186656385779,
23.6799895003701,24.1733226149611,24.6666557295522,25.1599888441432,25.6533219587342,
26.1466550733253,26.4410951701193),.UNSPECIFIED.);
#2523=B_SPLINE_CURVE_WITH_KNOTS('',3,(#22616,#22617,#22618,#22619,#22620,
#22621,#22622,#22623,#22624,#22625,#22626,#22627,#22628,#22629,#22630,#22631,
#22632,#22633,#22634,#22635,#22636,#22637,#22638,#22639,#22640,#22641,#22642,
#22643,#22644,#22645,#22646,#22647,#22648,#22649,#22650,#22651,#22652,#22653,
#22654,#22655),.UNSPECIFIED.,.F.,.F.,(4,3,3,3,3,3,3,3,3,3,3,3,3,4),(-28.9938076301211,
-28.6133206462805,-28.1199875316895,-27.6266544170984,-27.1333213025074,
-26.6399881879163,-26.1466550733253,-25.6533219587342,-25.1599888441432,
-24.6666557295522,-24.1733226149611,-23.6799895003701,-23.186656385779,
-22.7106223229415),.UNSPECIFIED.);
#2524=B_SPLINE_CURVE_WITH_KNOTS('',3,(#22656,#22657,#22658,#22659,#22660,
#22661,#22662,#22663,#22664,#22665,#22666,#22667,#22668,#22669,#22670,#22671,
#22672,#22673,#22674,#22675,#22676,#22677,#22678,#22679,#22680,#22681,#22682,
#22683,#22684,#22685,#22686,#22687,#22688,#22689,#22690,#22691,#22692,#22693,
#22694,#22695,#22696,#22697,#22698),.UNSPECIFIED.,.F.,.F.,(4,3,3,3,3,3,
3,3,3,3,3,3,3,3,4),(26.4410951701193,26.6399881879163,27.1333213025074,
27.6266544170984,28.1199875316895,28.6133206462805,29.1066537608716,29.5999868754626,
30.0933199900536,30.5866531046447,31.0799862192357,31.5733193338268,32.0666524484178,
32.5599855630089,32.7242804772989),.UNSPECIFIED.);
#2525=B_SPLINE_CURVE_WITH_KNOTS('',3,(#22703,#22704,#22705,#22706,#22707,
#22708,#22709,#22710,#22711,#22712,#22713,#22714,#22715,#22716,#22717,#22718,
#22719,#22720,#22721,#22722,#22723,#22724,#22725,#22726,#22727,#22728,#22729,
#22730,#22731,#22732,#22733,#22734,#22735,#22736,#22737,#22738,#22739,#22740,
#22741,#22742,#22743,#22744,#22745),.UNSPECIFIED.,.F.,.F.,(4,3,3,3,3,3,
3,3,3,3,3,3,3,3,4),(-35.2769929373007,-35.0266511359641,-34.533318021373,
-34.039984906782,-33.5466517921909,-33.0533186775999,-32.5599855630088,
-32.0666524484178,-31.5733193338268,-31.0799862192357,-30.5866531046447,
-30.0933199900536,-29.5999868754626,-29.1066537608715,-28.9938076301211),
 .UNSPECIFIED.);
#2526=B_SPLINE_CURVE_WITH_KNOTS('',3,(#22746,#22747,#22748,#22749,#22750,
#22751,#22752,#22753,#22754,#22755,#22756,#22757,#22758,#22759,#22760,#22761,
#22762,#22763,#22764,#22765,#22766,#22767,#22768,#22769,#22770,#22771,#22772,
#22773,#22774,#22775,#22776,#22777,#22778,#22779,#22780,#22781,#22782,#22783,
#22784,#22785,#22786,#22787,#22788),.UNSPECIFIED.,.F.,.F.,(4,3,3,3,3,3,
3,3,3,3,3,3,3,3,4),(32.7242804772989,33.0533186775999,33.5466517921909,
34.039984906782,34.533318021373,35.0266511359641,35.5199842505551,36.0133173651462,
36.5066504797372,36.9999835943282,37.4933167089193,37.9866498235103,38.4799829381014,
38.9733160526924,39.0074657844785),.UNSPECIFIED.);
#2527=B_SPLINE_CURVE_WITH_KNOTS('',3,(#22793,#22794,#22795,#22796,#22797,
#22798,#22799,#22800,#22801,#22802,#22803,#22804,#22805,#22806,#22807,#22808,
#22809,#22810,#22811,#22812,#22813,#22814,#22815,#22816,#22817,#22818,#22819,
#22820,#22821,#22822,#22823,#22824,#22825,#22826,#22827,#22828,#22829,#22830,
#22831,#22832,#22833,#22834,#22835),.UNSPECIFIED.,.F.,.F.,(4,3,3,3,3,3,
3,3,3,3,3,3,3,3,4),(-41.5601782444803,-41.4399816256476,-40.9466485110566,
-40.4533153964655,-39.9599822818745,-39.4666491672834,-38.9733160526924,
-38.4799829381014,-37.9866498235103,-37.4933167089193,-36.9999835943282,
-36.5066504797372,-36.0133173651462,-35.5199842505551,-35.2769929373007),
 .UNSPECIFIED.);
#2528=B_SPLINE_CURVE_WITH_KNOTS('',3,(#22836,#22837,#22838,#22839,#22840,
#22841,#22842,#22843,#22844,#22845,#22846,#22847,#22848,#22849,#22850,#22851,
#22852,#22853,#22854,#22855,#22856,#22857,#22858,#22859,#22860,#22861,#22862,
#22863,#22864,#22865,#22866,#22867,#22868,#22869,#22870,#22871,#22872,#22873,
#22874,#22875),.UNSPECIFIED.,.F.,.F.,(4,3,3,3,3,3,3,3,3,3,3,3,3,4),(39.0074657844785,
39.4666491672835,39.9599822818745,40.4533153964655,40.9466485110566,41.4399816256476,
41.9333147402387,42.4266478548297,42.9199809694208,43.4133140840118,43.9066471986028,
44.3999803131939,44.8933134277849,45.2906510916581),.UNSPECIFIED.);
#2529=B_SPLINE_CURVE_WITH_KNOTS('',3,(#22881,#22882,#22883,#22884,#22885,
#22886,#22887),.UNSPECIFIED.,.F.,.F.,(4,3,4),(51.5738363988376,51.7999770320595,
52.2933101466506),.UNSPECIFIED.);
#2530=B_SPLINE_CURVE_WITH_KNOTS('',3,(#22890,#22891,#22892,#22893,#22894,
#22895,#22896,#22897,#22898,#22899,#22900,#22901,#22902,#22903,#22904,#22905,
#22906,#22907,#22908),.UNSPECIFIED.,.F.,.F.,(4,3,3,3,3,3,4),(-50.2654824574367,
-49.8266445736954,-49.3333114591043,-48.8399783445133,-48.3466452299222,
-47.8533121153312,-47.8433635516598),.UNSPECIFIED.);
#2531=B_SPLINE_CURVE_WITH_KNOTS('',3,(#22914,#22915,#22916,#22917,#22918,
#22919,#22920,#22921,#22922,#22923,#22924,#22925,#22926),.UNSPECIFIED.,
 .F.,.F.,(4,1,1,1,1,1,1,1,1,1,4),(59.6902604182061,59.7002089818774,60.1935420964684,
60.6868752110595,61.1802083256505,61.6735414402416,62.1668745548326,62.6602076694237,
63.1535407840147,63.6468738986057,64.1402070131968),.UNSPECIFIED.);
#2532=B_SPLINE_CURVE_WITH_KNOTS('',3,(#22929,#22930,#22931,#22932,#22933,
#22934,#22935,#22936,#22937,#22938,#22939,#22940,#22941,#22942),
 .UNSPECIFIED.,.F.,.F.,(4,1,1,1,1,1,1,1,1,1,1,4),(59.6902604182061,59.786255868924,
60.279588983515,60.7729220981061,61.2662552126971,61.7595883272881,62.2529214418792,
62.7462545564702,63.2395876710613,63.7329207856523,64.2262539002434,64.6650917839847),
 .UNSPECIFIED.);
#2533=B_SPLINE_CURVE_WITH_KNOTS('',3,(#22947,#22948,#22949,#22950,#22951,
#22952,#22953,#22954,#22955,#22956,#22957,#22958,#22959,#22960,#22961,#22962),
 .UNSPECIFIED.,.F.,.F.,(4,1,1,1,1,1,1,1,1,1,1,1,1,4),(53.4070751110265,
53.7802116067849,54.2735447213759,54.766877835967,55.260210950558,55.7535440651491,
56.2468771797401,56.7402102943311,57.2335434089222,57.7268765235132,58.2202096381043,
58.7135427526953,59.2068758672864,59.6902604182061),.UNSPECIFIED.);
#2534=B_SPLINE_CURVE_WITH_KNOTS('',3,(#22963,#22964,#22965,#22966,#22967,
#22968,#22969,#22970,#22971,#22972,#22973,#22974,#22975,#22976,#22977,#22978),
 .UNSPECIFIED.,.F.,.F.,(4,1,1,1,1,1,1,1,1,1,1,1,1,4),(53.4070751110265,
53.8662584938314,54.3595916084225,54.8529247230135,55.3462578376046,55.8395909521956,
56.3329240667867,56.8262571813777,57.3195902959688,57.8129234105598,58.3062565251508,
58.7995896397419,59.2929227543329,59.6902604182061),.UNSPECIFIED.);
#2535=B_SPLINE_CURVE_WITH_KNOTS('',3,(#22983,#22984,#22985,#22986,#22987,
#22988,#22989,#22990,#22991,#22992,#22993,#22994,#22995,#22996,#22997,#22998,
#22999),.UNSPECIFIED.,.F.,.F.,(4,1,1,1,1,1,1,1,1,1,1,1,1,1,4),(47.1238898038469,
47.3668811171013,47.8602142316924,48.3535473462834,48.8468804608745,49.3402135754655,
49.8335466900565,50.3268798046476,50.8202129192386,51.3135460338297,51.8068791484207,
52.3002122630117,52.7935453776028,53.2868784921938,53.4070751110265),
 .UNSPECIFIED.);
#2536=B_SPLINE_CURVE_WITH_KNOTS('',3,(#23000,#23001,#23002,#23003,#23004,
#23005,#23006,#23007,#23008,#23009,#23010,#23011,#23012,#23013,#23014,#23015,
#23016),.UNSPECIFIED.,.F.,.F.,(4,1,1,1,1,1,1,1,1,1,1,1,1,1,4),(47.1238898038469,
47.4529280041479,47.9462611187389,48.43959423333,48.932927347921,49.4262604625121,
49.9195935771031,50.4129266916941,50.9062598062852,51.3995929208762,51.8929260354673,
52.3862591500583,52.8795922646494,53.3729253792404,53.4070751110265),
 .UNSPECIFIED.);
#2537=B_SPLINE_CURVE_WITH_KNOTS('',3,(#23021,#23022,#23023,#23024,#23025,
#23026,#23027,#23028,#23029,#23030,#23031,#23032,#23033,#23034,#23035,#23036,
#23037),.UNSPECIFIED.,.F.,.F.,(4,1,1,1,1,1,1,1,1,1,1,1,1,1,4),(40.8407044966673,
40.9535506274178,41.4468837420088,41.9402168565998,42.4335499711909,42.9268830857819,
43.420216200373,43.913549314964,44.4068824295551,44.9002155441461,45.3935486587371,
45.8868817733282,46.3802148879192,46.8735480025103,47.1238898038469),
 .UNSPECIFIED.);
#2538=B_SPLINE_CURVE_WITH_KNOTS('',3,(#23038,#23039,#23040,#23041,#23042,
#23043,#23044,#23045,#23046,#23047,#23048,#23049,#23050,#23051,#23052,#23053,
#23054),.UNSPECIFIED.,.F.,.F.,(4,1,1,1,1,1,1,1,1,1,1,1,1,1,4),(40.8407044966673,
41.0395975144643,41.5329306290554,42.0262637436464,42.5195968582374,43.0129299728285,
43.5062630874195,43.9995962020106,44.4929293166016,44.9862624311927,45.4795955457837,
45.9729286603748,46.4662617749658,46.9595948895568,47.1238898038469),
 .UNSPECIFIED.);
#2539=B_SPLINE_CURVE_WITH_KNOTS('',3,(#23059,#23060,#23061,#23062,#23063,
#23064,#23065,#23066,#23067,#23068,#23069,#23070,#23071,#23072,#23073,#23074),
 .UNSPECIFIED.,.F.,.F.,(4,1,1,1,1,1,1,1,1,1,1,1,1,4),(34.5575191894877,
35.0335532523252,35.5268863669163,36.0202194815073,36.5135525960984,37.0068857106894,
37.5002188252805,37.9935519398715,38.4868850544625,38.9802181690536,39.4735512836446,
39.9668843982357,40.4602175128267,40.8407044966673),.UNSPECIFIED.);
#2540=B_SPLINE_CURVE_WITH_KNOTS('',3,(#23075,#23076,#23077,#23078,#23079,
#23080,#23081,#23082,#23083,#23084,#23085,#23086,#23087,#23088,#23089,#23090,
#23091),.UNSPECIFIED.,.F.,.F.,(4,1,1,1,1,1,1,1,1,1,1,1,1,1,4),(34.5575191894877,
34.6262670247808,35.1196001393718,35.6129332539629,36.1062663685539,36.5995994831449,
37.092932597736,37.586265712327,38.0795988269181,38.5729319415091,39.0662650561001,
39.5595981706912,40.0529312852822,40.5462643998733,40.8407044966673),
 .UNSPECIFIED.);
#2541=B_SPLINE_CURVE_WITH_KNOTS('',3,(#23096,#23097,#23098,#23099,#23100,
#23101,#23102,#23103,#23104,#23105,#23106,#23107,#23108,#23109,#23110,#23111,
#23112),.UNSPECIFIED.,.F.,.F.,(4,1,1,1,1,1,1,1,1,1,1,1,1,1,4),(28.2743338823081,
28.6202227626417,29.1135558772327,29.6068889918238,30.1002221064148,30.5935552210059,
31.0868883355969,31.5802214501879,32.073554564779,32.56688767937,33.0602207939611,
33.5535539085521,34.0468870231432,34.5402201377342,34.5575191894877),
 .UNSPECIFIED.);
#2542=B_SPLINE_CURVE_WITH_KNOTS('',3,(#23113,#23114,#23115,#23116,#23117,
#23118,#23119,#23120,#23121,#23122,#23123,#23124,#23125,#23126,#23127,#23128),
 .UNSPECIFIED.,.F.,.F.,(4,1,1,1,1,1,1,1,1,1,1,1,1,4),(28.2743338823081,
28.7062696496882,29.1996027642793,29.6929358788703,30.1862689934614,30.6796021080524,
31.1729352226435,31.6662683372345,32.1596014518255,32.6529345664166,33.1462676810076,
33.6396007955987,34.1329339101897,34.5575191894877),.UNSPECIFIED.);
#2543=B_SPLINE_CURVE_WITH_KNOTS('',3,(#23133,#23134,#23135,#23136,#23137,
#23138,#23139,#23140,#23141,#23142,#23143,#23144,#23145,#23146,#23147,#23148,
#23149),.UNSPECIFIED.,.F.,.F.,(4,1,1,1,1,1,1,1,1,1,1,1,1,1,4),(21.9911485751285,
22.2068922729581,22.7002253875492,23.1935585021402,23.6868916167312,24.1802247313223,
24.6735578459133,25.1668909605044,25.6602240750954,26.1535571896865,26.6468903042775,
27.1402234188686,27.6335565334596,28.1268896480506,28.2743338823081),
 .UNSPECIFIED.);
#2544=B_SPLINE_CURVE_WITH_KNOTS('',3,(#23150,#23151,#23152,#23153,#23154,
#23155,#23156,#23157,#23158,#23159,#23160,#23161,#23162,#23163,#23164,#23165,
#23166),.UNSPECIFIED.,.F.,.F.,(4,1,1,1,1,1,1,1,1,1,1,1,1,1,4),(21.9911485751285,
22.2929391600047,22.7862722745957,23.2796053891868,23.7729385037778,24.2662716183689,
24.7596047329599,25.2529378475509,25.746270962142,26.239604076733,26.7329371913241,
27.2262703059151,27.7196034205062,28.2129365350972,28.2743338823081),
 .UNSPECIFIED.);
#2545=B_SPLINE_CURVE_WITH_KNOTS('',3,(#23172,#23173,#23174,#23175,#23176,
#23177),.UNSPECIFIED.,.F.,.F.,(4,1,1,4),(14.399609326548,14.892942441139,
15.3862755557301,15.7079632679489),.UNSPECIFIED.);
#2546=B_SPLINE_CURVE_WITH_KNOTS('',3,(#23180,#23181,#23182,#23183,#23184,
#23185,#23186),.UNSPECIFIED.,.F.,.F.,(4,1,1,1,4),(13.8747245557601,14.3135624395014,
14.8068955540925,15.3002286686835,15.7079632679489),.UNSPECIFIED.);
#2547=B_SPLINE_CURVE_WITH_KNOTS('',3,(#23188,#23189,#23190,#23191,#23192,
#23193,#23194,#23195,#23196,#23197,#23198,#23199,#23200,#23201,#23202,#23203,
#23204),.UNSPECIFIED.,.F.,.F.,(4,1,1,1,1,1,1,1,1,1,1,1,1,1,4),(15.7079632679489,
15.7935617832746,16.2868948978656,16.7802280124566,17.2735611270477,17.7668942416387,
18.2602273562298,18.7535604708208,19.2468935854119,19.7402267000029,20.2335598145939,
20.726892929185,21.220226043776,21.7135591583671,21.9911485751285),
 .UNSPECIFIED.);
#2548=B_SPLINE_CURVE_WITH_KNOTS('',3,(#23205,#23206,#23207,#23208,#23209,
#23210,#23211,#23212,#23213,#23214,#23215,#23216,#23217,#23218,#23219,#23220,
#23221),.UNSPECIFIED.,.F.,.F.,(4,1,1,1,1,1,1,1,1,1,1,1,1,1,4),(15.7079632679489,
15.8796086703211,16.3729417849122,16.8662748995032,17.3596080140942,17.8529411286853,
18.3462742432763,18.8396073578674,19.3329404724584,19.8262735870495,20.3196067016405,
20.8129398162316,21.3062729308226,21.7996060454136,21.9911485751285),
 .UNSPECIFIED.);
#2549=B_SPLINE_CURVE_WITH_KNOTS('',3,(#23658,#23659,#23660,#23661,#23662,
#23663,#23664,#23665,#23666,#23667,#23668,#23669,#23670,#23671,#23672,#23673,
#23674,#23675,#23676,#23677,#23678,#23679,#23680,#23681,#23682,#23683,#23684,
#23685,#23686,#23687,#23688,#23689,#23690,#23691,#23692,#23693,#23694,#23695,
#23696,#23697,#23698,#23699,#23700,#23701,#23702,#23703,#23704,#23705,#23706,
#23707,#23708,#23709,#23710,#23711,#23712,#23713,#23714,#23715,#23716,#23717,
#23718,#23719,#23720,#23721,#23722,#23723,#23724,#23725,#23726,#23727,#23728,
#23729,#23730,#23731,#23732,#23733,#23734,#23735,#23736,#23737,#23738,#23739,
#23740,#23741,#23742,#23743,#23744,#23745,#23746,#23747,#23748,#23749,#23750,
#23751,#23752,#23753,#23754,#23755,#23756,#23757,#23758,#23759,#23760,#23761,
#23762,#23763,#23764,#23765,#23766,#23767,#23768,#23769,#23770,#23771,#23772,
#23773,#23774,#23775),.UNSPECIFIED.,.F.,.F.,(4,3,3,3,3,3,3,3,3,3,3,3,3,
3,3,3,3,3,3,3,3,3,3,3,3,3,3,3,3,3,3,3,3,3,3,3,3,3,3,4),(0.,0.0627492990436898,
0.126104878557015,0.189559165750867,0.252240710610912,0.288293603463481,
0.305992302061488,0.313657647656099,0.376040517871268,0.396452282021189,
0.458859852998567,0.521377063013053,0.583471845815152,0.608441703375899,
0.617034910983491,0.624625669288178,0.686130542524575,0.747366752808485,
0.783230706301131,0.844791963679094,0.884204320253698,0.904295818732976,
0.915687585522282,0.925544690548276,0.986118296783461,1.04668162399669,
1.10647431181231,1.16009081627592,1.20586175519752,1.21479111361079,1.22268680003196,
1.28246147175047,1.34341068572502,1.36939753329053,1.38708197012437,1.39811570618177,
1.45723390803205,1.51569706964298,1.52625832764867,1.5660690749997),
 .UNSPECIFIED.);
#2550=B_SPLINE_CURVE_WITH_KNOTS('',3,(#23776,#23777,#23778,#23779,#23780,
#23781,#23782,#23783,#23784,#23785,#23786,#23787,#23788,#23789,#23790,#23791,
#23792,#23793,#23794,#23795,#23796,#23797,#23798,#23799,#23800,#23801,#23802,
#23803,#23804,#23805,#23806,#23807,#23808,#23809,#23810,#23811,#23812,#23813,
#23814,#23815,#23816,#23817,#23818,#23819,#23820,#23821,#23822,#23823,#23824,
#23825,#23826,#23827,#23828,#23829,#23830,#23831,#23832,#23833,#23834,#23835,
#23836,#23837,#23838,#23839,#23840,#23841,#23842,#23843,#23844,#23845,#23846,
#23847,#23848,#23849,#23850,#23851,#23852,#23853,#23854,#23855,#23856,#23857,
#23858,#23859,#23860,#23861,#23862,#23863,#23864,#23865,#23866,#23867,#23868,
#23869,#23870,#23871,#23872,#23873,#23874,#23875,#23876,#23877,#23878,#23879,
#23880,#23881,#23882,#23883,#23884,#23885,#23886,#23887,#23888,#23889,#23890),
 .UNSPECIFIED.,.F.,.F.,(4,3,3,3,3,3,3,3,3,3,3,3,3,3,3,3,3,3,3,3,3,3,3,3,
3,3,3,3,3,3,3,3,3,3,3,3,3,3,4),(0.,0.0577406588992485,0.116385458548516,
0.178509073187712,0.237685128911259,0.26948382595977,0.284721470013156,
0.290885054843453,0.350989811053008,0.364879917105302,0.424389656797942,
0.484492894172679,0.544731621925967,0.569116073872798,0.578654385819093,
0.585597036801517,0.646393915917858,0.707630011320198,0.73980723750061,
0.800806777752653,0.841276065989419,0.862788429498789,0.876711500915515,
0.884407389586128,0.946057888963432,1.00815397980749,1.07016859908497,1.12456108364678,
1.17378987619966,1.18207737487297,1.1898217223955,1.2520187672784,1.3147895064124,
1.36568998582675,1.37764504908115,1.44103981650812,1.50440163169237,1.5183914240698,
1.56247950813563),.UNSPECIFIED.);
#2551=B_SPLINE_CURVE_WITH_KNOTS('',3,(#23891,#23892,#23893,#23894,#23895,
#23896,#23897,#23898,#23899,#23900,#23901,#23902,#23903,#23904,#23905,#23906,
#23907,#23908,#23909,#23910,#23911,#23912,#23913,#23914,#23915,#23916,#23917,
#23918,#23919,#23920,#23921,#23922,#23923,#23924,#23925,#23926,#23927,#23928,
#23929,#23930),.UNSPECIFIED.,.F.,.F.,(4,3,3,3,3,3,3,3,3,3,3,3,3,4),(-47.8433635516598,
-47.3599790007401,-46.8666458861491,-46.3733127715581,-45.879979656967,
-45.386646542376,-44.8933134277849,-44.3999803131939,-43.9066471986028,
-43.4133140840118,-42.9199809694207,-42.4266478548297,-41.9333147402387,
-41.5601782444803),.UNSPECIFIED.);
#2552=B_SPLINE_CURVE_WITH_KNOTS('',3,(#24367,#24368,#24369,#24370,#24371,
#24372,#24373,#24374,#24375,#24376,#24377,#24378,#24379,#24380,#24381,#24382,
#24383,#24384,#24385,#24386,#24387,#24388,#24389,#24390,#24391,#24392,#24393,
#24394,#24395,#24396,#24397,#24398,#24399,#24400,#24401,#24402,#24403,#24404,
#24405,#24406,#24407,#24408,#24409,#24410,#24411,#24412,#24413,#24414,#24415,
#24416,#24417,#24418,#24419,#24420,#24421,#24422,#24423,#24424,#24425,#24426,
#24427,#24428,#24429,#24430,#24431,#24432,#24433,#24434,#24435,#24436,#24437,
#24438,#24439,#24440,#24441,#24442,#24443,#24444,#24445,#24446,#24447,#24448,
#24449,#24450,#24451,#24452,#24453,#24454,#24455,#24456,#24457,#24458,#24459,
#24460,#24461,#24462,#24463,#24464,#24465,#24466,#24467,#24468,#24469,#24470,
#24471,#24472,#24473,#24474,#24475,#24476,#24477,#24478,#24479,#24480,#24481),
 .UNSPECIFIED.,.F.,.F.,(4,3,3,3,3,3,3,3,3,3,3,3,3,3,3,3,3,3,3,3,3,3,3,3,
3,3,3,3,3,3,3,3,3,3,3,3,3,3,4),(0.,0.0577407111586883,0.116385549588121,
0.178509141467415,0.237685182802617,0.269483866378287,0.284721532925159,
0.290885122681355,0.350989895531535,0.364879917105296,0.424389621803389,
0.484492840377873,0.544731565736105,0.56911602470667,0.578654437928008,
0.58559704689236,0.646393901436191,0.707629993882402,0.739807237500627,
0.800806786500127,0.841276073643457,0.862788446713888,0.876711473705084,
0.884407384588612,0.946057896589746,1.00815399351749,1.07016861248816,1.12456108364677,
1.17378987619965,1.18207737505914,1.18982172246769,1.25201876607222,1.31478950544163,
1.36568998509867,1.3776450487033,1.44103981654898,1.50440163107218,1.51839142406977,
1.56247950813554),.UNSPECIFIED.);
#2553=B_SPLINE_CURVE_WITH_KNOTS('',3,(#24482,#24483,#24484,#24485,#24486,
#24487,#24488,#24489,#24490,#24491,#24492,#24493,#24494,#24495,#24496,#24497,
#24498,#24499,#24500,#24501,#24502,#24503,#24504,#24505,#24506,#24507,#24508,
#24509,#24510,#24511,#24512,#24513,#24514,#24515,#24516,#24517,#24518,#24519,
#24520,#24521,#24522,#24523,#24524),.UNSPECIFIED.,.F.,.F.,(4,3,3,3,3,3,
3,3,3,3,3,3,3,3,4),(45.2906510916581,45.386646542376,45.879979656967,46.3733127715581,
46.8666458861491,47.3599790007402,47.8533121153312,48.3466452299222,48.8399783445133,
49.3333114591043,49.8266445736954,50.3199776882864,50.8133108028775,51.3066439174685,
51.5738363988376),.UNSPECIFIED.);
#2554=B_SPLINE_CURVE_WITH_KNOTS('',3,(#24525,#24526,#24527,#24528,#24529,
#24530,#24531,#24532,#24533,#24534,#24535,#24536,#24537,#24538,#24539,#24540,
#24541,#24542,#24543,#24544,#24545,#24546,#24547,#24548,#24549,#24550,#24551,
#24552,#24553,#24554,#24555,#24556,#24557,#24558,#24559,#24560,#24561,#24562,
#24563,#24564,#24565,#24566,#24567,#24568,#24569,#24570,#24571,#24572,#24573,
#24574,#24575,#24576,#24577,#24578,#24579,#24580,#24581,#24582,#24583,#24584,
#24585,#24586,#24587,#24588,#24589,#24590,#24591,#24592,#24593,#24594,#24595,
#24596,#24597,#24598,#24599,#24600,#24601,#24602,#24603,#24604,#24605,#24606,
#24607,#24608,#24609,#24610,#24611,#24612,#24613,#24614,#24615,#24616,#24617,
#24618,#24619,#24620,#24621,#24622,#24623,#24624,#24625,#24626,#24627,#24628,
#24629,#24630,#24631,#24632,#24633,#24634,#24635,#24636,#24637,#24638,#24639,
#24640,#24641,#24642),.UNSPECIFIED.,.F.,.F.,(4,3,3,3,3,3,3,3,3,3,3,3,3,
3,3,3,3,3,3,3,3,3,3,3,3,3,3,3,3,3,3,3,3,3,3,3,3,3,3,4),(0.,0.0627493370856802,
0.126104932649105,0.189559213327594,0.252240727815851,0.288293616367183,
0.305992302583669,0.313657647775325,0.376040508715825,0.396452282021179,
0.458859839175422,0.521377049363119,0.583471840572106,0.608441698788235,
0.617034861909103,0.624625665831328,0.686130535161024,0.747366753389966,
0.783230706301136,0.844791964570227,0.884204321033441,0.904295823092356,
0.915687649661771,0.925544683877737,0.98611829233901,1.04668162002177,1.1064743111715,
1.16009081627594,1.20586175519753,1.21479111379007,1.22268680009421,1.28246147324105,
1.34341068684296,1.36939753500024,1.3870819748845,1.39811570742417,1.45723390831247,
1.51569706474686,1.52625832764868,1.56606907499972),.UNSPECIFIED.);
#2555=B_SPLINE_CURVE_WITH_KNOTS('',3,(#24660,#24661,#24662,#24663,#24664,
#24665,#24666,#24667,#24668,#24669,#24670,#24671,#24672,#24673,#24674,#24675,
#24676,#24677,#24678,#24679,#24680,#24681,#24682,#24683,#24684,#24685,#24686,
#24687,#24688,#24689,#24690,#24691,#24692,#24693,#24694,#24695,#24696,#24697,
#24698,#24699,#24700,#24701,#24702,#24703,#24704,#24705,#24706,#24707,#24708,
#24709,#24710,#24711,#24712,#24713,#24714,#24715,#24716,#24717,#24718,#24719,
#24720,#24721,#24722,#24723,#24724,#24725,#24726,#24727,#24728,#24729,#24730,
#24731,#24732,#24733,#24734,#24735,#24736,#24737,#24738,#24739,#24740,#24741,
#24742,#24743,#24744,#24745,#24746,#24747,#24748,#24749,#24750),
 .UNSPECIFIED.,.F.,.F.,(4,3,3,3,3,3,3,3,3,3,3,3,3,3,3,3,3,3,3,3,3,3,3,3,
3,3,3,3,3,3,4),(0.,0.0297288188736182,0.0601143137532858,0.0893457032423633,
0.114923169045306,0.120627215633482,0.150386402906777,0.17998053365335,
0.208476757656489,0.220427983970411,0.228734462393759,0.234133594656578,
0.264049512161242,0.291954347405626,0.293965429665906,0.322911719928455,
0.339205408301995,0.343413416245237,0.371505798227718,0.399644786528458,
0.427380412744627,0.437702076823844,0.444667737156878,0.449308449996483,
0.477249012718954,0.498204434760807,0.506474258991161,0.511856137621095,
0.53779059950688,0.561070700886365,0.569248610399433),.UNSPECIFIED.);
#2556=B_SPLINE_CURVE_WITH_KNOTS('',3,(#24751,#24752,#24753,#24754,#24755,
#24756,#24757,#24758,#24759,#24760,#24761,#24762,#24763,#24764,#24765,#24766,
#24767,#24768,#24769,#24770,#24771,#24772,#24773,#24774,#24775,#24776,#24777,
#24778,#24779,#24780,#24781,#24782,#24783,#24784,#24785,#24786,#24787,#24788,
#24789,#24790,#24791,#24792,#24793,#24794,#24795,#24796,#24797,#24798,#24799,
#24800,#24801,#24802,#24803,#24804,#24805,#24806,#24807,#24808,#24809,#24810,
#24811,#24812,#24813,#24814,#24815,#24816,#24817,#24818,#24819,#24820,#24821,
#24822,#24823,#24824,#24825,#24826,#24827,#24828,#24829,#24830,#24831,#24832,
#24833,#24834,#24835,#24836,#24837,#24838,#24839,#24840,#24841,#24842,#24843,
#24844),.UNSPECIFIED.,.F.,.F.,(4,3,3,3,3,3,3,3,3,3,3,3,3,3,3,3,3,3,3,3,
3,3,3,3,3,3,3,3,3,3,3,4),(0.,0.0253686794174057,0.0514083856253428,0.0781556456631177,
0.0899216241726569,0.0966318743809286,0.10267802399304,0.12998244418627,
0.157736117425355,0.184648704550902,0.195933028986547,0.203013212233092,
0.207157428316433,0.236271947121987,0.265386465927542,0.293276540785509,
0.302549255500035,0.31126847526333,0.31569998302984,0.343808925905663,0.372948812494613,
0.402401913058982,0.413322292212205,0.422821815526522,0.427499464953869,
0.457558884663827,0.48241578665523,0.491036990018943,0.49835751386338,0.528866710916645,
0.556986492629438,0.566847306048074),.UNSPECIFIED.);
#2557=B_SPLINE_CURVE_WITH_KNOTS('',3,(#24845,#24846,#24847,#24848,#24849,
#24850,#24851,#24852,#24853,#24854,#24855,#24856,#24857,#24858,#24859,#24860,
#24861,#24862,#24863,#24864,#24865,#24866,#24867,#24868,#24869,#24870,#24871,
#24872,#24873,#24874,#24875,#24876,#24877,#24878,#24879,#24880,#24881,#24882,
#24883,#24884,#24885,#24886,#24887,#24888,#24889,#24890,#24891,#24892,#24893,
#24894,#24895,#24896,#24897,#24898,#24899,#24900,#24901,#24902,#24903,#24904,
#24905,#24906,#24907,#24908,#24909,#24910,#24911,#24912,#24913,#24914,#24915,
#24916,#24917,#24918,#24919,#24920,#24921,#24922,#24923,#24924,#24925,#24926,
#24927,#24928,#24929,#24930,#24931,#24932,#24933,#24934,#24935),
 .UNSPECIFIED.,.F.,.F.,(4,3,3,3,3,3,3,3,3,3,3,3,3,3,3,3,3,3,3,3,3,3,3,3,
3,3,3,3,3,3,4),(0.,0.0297288300137718,0.0601143303526995,0.0893457177668503,
0.114923181754232,0.120627216473642,0.150386403780864,0.179980531396028,
0.208476755963498,0.220427980048027,0.228734451696019,0.2341335924423,0.264049511054103,
0.291954343374694,0.293965429665906,0.322911720395065,0.339205406534996,
0.343413414673066,0.371505796934876,0.399644785176017,0.42738040871261,
0.437702067530731,0.444667652090904,0.449308353053096,0.477248940011413,
0.498204380230151,0.50647415245726,0.51185608788507,0.537790544146639,0.561070700886365,
0.569248610399433),.UNSPECIFIED.);
#2558=B_SPLINE_CURVE_WITH_KNOTS('',3,(#24936,#24937,#24938,#24939,#24940,
#24941,#24942,#24943,#24944,#24945,#24946,#24947,#24948,#24949,#24950,#24951,
#24952,#24953,#24954,#24955,#24956,#24957,#24958,#24959,#24960,#24961,#24962,
#24963,#24964,#24965,#24966,#24967,#24968,#24969,#24970,#24971,#24972,#24973,
#24974,#24975,#24976,#24977,#24978,#24979,#24980,#24981,#24982,#24983,#24984,
#24985,#24986,#24987,#24988,#24989,#24990,#24991,#24992,#24993,#24994,#24995,
#24996,#24997,#24998,#24999,#25000,#25001,#25002,#25003,#25004,#25005,#25006,
#25007,#25008,#25009,#25010,#25011,#25012,#25013,#25014,#25015,#25016,#25017,
#25018,#25019,#25020,#25021,#25022,#25023,#25024,#25025,#25026,#25027,#25028,
#25029),.UNSPECIFIED.,.F.,.F.,(4,3,3,3,3,3,3,3,3,3,3,3,3,3,3,3,3,3,3,3,
3,3,3,3,3,3,3,3,3,3,3,4),(0.,0.025368693811206,0.05140841299331,0.0781556696100889,
0.0899216297021826,0.0966318750772424,0.102678024005019,0.129982454186119,
0.157736132240341,0.184648715662141,0.19593303134926,0.203013213057673,
0.207157430078829,0.236271948003186,0.265386465927542,0.293276533635152,
0.302549240751372,0.311268412157304,0.315699971306864,0.343808903791577,
0.372948785654744,0.40240188507586,0.41332223980539,0.422821617175178,0.427499196231939,
0.457558610846334,0.48241558129211,0.491036574482664,0.498357488494488,
0.528866685800111,0.556986492629438,0.566847306048074),.UNSPECIFIED.);
#2559=B_SPLINE_CURVE_WITH_KNOTS('',3,(#25030,#25031,#25032,#25033,#25034,
#25035,#25036,#25037,#25038,#25039,#25040,#25041,#25042,#25043,#25044,#25045,
#25046,#25047,#25048,#25049,#25050,#25051,#25052,#25053,#25054,#25055,#25056,
#25057,#25058,#25059,#25060,#25061,#25062,#25063,#25064,#25065,#25066,#25067,
#25068,#25069,#25070,#25071,#25072,#25073,#25074,#25075,#25076,#25077,#25078,
#25079,#25080,#25081,#25082,#25083,#25084,#25085,#25086,#25087,#25088,#25089,
#25090,#25091,#25092,#25093,#25094,#25095,#25096,#25097,#25098,#25099,#25100,
#25101,#25102,#25103,#25104,#25105,#25106,#25107,#25108,#25109,#25110,#25111,
#25112,#25113,#25114,#25115,#25116,#25117,#25118,#25119,#25120),
 .UNSPECIFIED.,.F.,.F.,(4,3,3,3,3,3,3,3,3,3,3,3,3,3,3,3,3,3,3,3,3,3,3,3,
3,3,3,3,3,3,4),(0.,0.0297288424070436,0.0601143488180543,0.0893457339240374,
0.114923195891773,0.120627217421351,0.150386404765411,0.179980528895957,
0.208476754088448,0.220427975697114,0.228734439831626,0.234133589983501,
0.26404950982471,0.291954338892652,0.293965429665919,0.322911720916077,
0.339205404572844,0.343413412951878,0.371505795524539,0.399644783698224,
0.427380404250721,0.437702057239815,0.4446675578577,0.449308245657091,0.477248859464417,
0.498204319819911,0.506474034422274,0.511856032820092,0.537790482818068,
0.561070700886393,0.569248610399461),.UNSPECIFIED.);
#2560=B_SPLINE_CURVE_WITH_KNOTS('',3,(#25121,#25122,#25123,#25124,#25125,
#25126,#25127,#25128,#25129,#25130,#25131,#25132,#25133,#25134,#25135,#25136,
#25137,#25138,#25139,#25140,#25141,#25142,#25143,#25144,#25145,#25146,#25147,
#25148,#25149,#25150,#25151,#25152,#25153,#25154,#25155,#25156,#25157,#25158,
#25159,#25160,#25161,#25162,#25163,#25164,#25165,#25166,#25167,#25168,#25169,
#25170,#25171,#25172,#25173,#25174,#25175,#25176,#25177,#25178,#25179,#25180,
#25181,#25182,#25183,#25184,#25185,#25186,#25187,#25188,#25189,#25190,#25191,
#25192,#25193,#25194,#25195,#25196,#25197,#25198,#25199,#25200,#25201,#25202,
#25203,#25204,#25205,#25206,#25207,#25208,#25209,#25210,#25211,#25212,#25213,
#25214),.UNSPECIFIED.,.F.,.F.,(4,3,3,3,3,3,3,3,3,3,3,3,3,3,3,3,3,3,3,3,
3,3,3,3,3,3,3,3,3,3,3,4),(0.,0.0253686551369141,0.0514083394586729,0.0781556052672844,
0.0899216148451408,0.0966318732064026,0.102678023982166,0.1299824273254,
0.157736092440688,0.184648685812407,0.19593302500215,0.203013210837855,
0.20715742531342,0.236271945620492,0.265386465927564,0.293276552845118,
0.302549280374791,0.311268581698407,0.315700002803736,0.343808963203445,
0.372948857762899,0.402401960255444,0.413322380602343,0.42282215008815,
0.427499918423473,0.45755934672975,0.482416133204678,0.491037691280722,
0.498357556788384,0.528866753414147,0.556986492629462,0.566847306048097),
 .UNSPECIFIED.);
#2561=B_SPLINE_CURVE_WITH_KNOTS('',3,(#25215,#25216,#25217,#25218,#25219,
#25220,#25221,#25222,#25223,#25224,#25225,#25226,#25227,#25228,#25229,#25230,
#25231,#25232,#25233,#25234,#25235,#25236,#25237,#25238,#25239,#25240,#25241,
#25242,#25243,#25244,#25245,#25246,#25247,#25248,#25249,#25250,#25251,#25252,
#25253,#25254,#25255,#25256,#25257,#25258,#25259,#25260,#25261,#25262,#25263,
#25264,#25265,#25266,#25267,#25268,#25269,#25270,#25271,#25272,#25273,#25274,
#25275,#25276,#25277,#25278,#25279,#25280,#25281,#25282,#25283,#25284,#25285,
#25286,#25287,#25288,#25289,#25290,#25291,#25292,#25293,#25294,#25295,#25296,
#25297,#25298,#25299,#25300,#25301,#25302,#25303,#25304,#25305),
 .UNSPECIFIED.,.F.,.F.,(4,3,3,3,3,3,3,3,3,3,3,3,3,3,3,3,3,3,3,3,3,3,3,3,
3,3,3,3,3,3,4),(0.,0.0297288560421965,0.060114369134978,0.0893457517013431,
0.114923211446913,0.120627218448761,0.150386405832768,0.179980526129192,
0.208476752013369,0.220427970890768,0.228734426721466,0.234133587258058,
0.264049508461979,0.291954333951181,0.293965429665899,0.322911721485533,
0.339205402404708,0.343413411034994,0.371505793949006,0.399644782047769,
0.427380399316125,0.437702045866938,0.444667453732877,0.449308126997909,
0.47724877047002,0.498204253074103,0.506473904026581,0.511855971995141,
0.537790415102179,0.561070700886353,0.56924861039942),.UNSPECIFIED.);
#2562=B_SPLINE_CURVE_WITH_KNOTS('',3,(#25306,#25307,#25308,#25309,#25310,
#25311,#25312,#25313,#25314,#25315,#25316,#25317,#25318,#25319,#25320,#25321,
#25322,#25323,#25324,#25325,#25326,#25327,#25328,#25329,#25330,#25331,#25332,
#25333,#25334,#25335,#25336,#25337,#25338,#25339,#25340,#25341,#25342,#25343,
#25344,#25345,#25346,#25347,#25348,#25349,#25350,#25351,#25352,#25353,#25354,
#25355,#25356,#25357,#25358,#25359,#25360,#25361,#25362,#25363,#25364,#25365,
#25366,#25367,#25368,#25369,#25370,#25371,#25372,#25373,#25374,#25375,#25376,
#25377,#25378,#25379,#25380,#25381,#25382,#25383,#25384,#25385,#25386,#25387,
#25388,#25389,#25390,#25391,#25392,#25393,#25394,#25395,#25396,#25397,#25398,
#25399),.UNSPECIFIED.,.F.,.F.,(4,3,3,3,3,3,3,3,3,3,3,3,3,3,3,3,3,3,3,3,
3,3,3,3,3,3,3,3,3,3,3,4),(0.,0.0253686665250508,0.0514083611125175,0.0781556242143958,
0.0899216192202383,0.0966318737573469,0.102678023990962,0.129982435238011,
0.157736104164076,0.184648694604943,0.195933026871913,0.203013211491678,
0.207157426736985,0.236271946332265,0.265386465927544,0.29327654718868,
0.302549268707551,0.311268531776406,0.315699993528777,0.34380894570794,
0.372948836529036,0.402401938117202,0.413322339141515,0.422821993154248,
0.427499705665215,0.457559129940086,0.482415970612417,0.4910373622589,0.498357536637505,
0.528866733464123,0.556986492629412,0.566847306048045),.UNSPECIFIED.);
#2563=B_SPLINE_CURVE_WITH_KNOTS('',3,(#25401,#25402,#25403,#25404,#25405,
#25406,#25407,#25408,#25409,#25410,#25411,#25412,#25413,#25414,#25415,#25416,
#25417,#25418,#25419,#25420,#25421,#25422,#25423,#25424,#25425,#25426,#25427,
#25428,#25429,#25430,#25431,#25432,#25433,#25434,#25435,#25436,#25437,#25438,
#25439,#25440,#25441,#25442,#25443,#25444,#25445,#25446,#25447,#25448,#25449,
#25450,#25451,#25452,#25453,#25454,#25455,#25456,#25457,#25458,#25459,#25460,
#25461,#25462,#25463,#25464,#25465,#25466,#25467,#25468,#25469,#25470,#25471,
#25472,#25473,#25474,#25475,#25476,#25477,#25478,#25479,#25480,#25481,#25482,
#25483,#25484,#25485,#25486,#25487,#25488,#25489,#25490,#25491,#25492,#25493,
#25494),.UNSPECIFIED.,.F.,.F.,(4,3,3,3,3,3,3,3,3,3,3,3,3,3,3,3,3,3,3,3,
3,3,3,3,3,3,3,3,3,3,3,4),(-0.569248610399439,-0.543569219999376,-0.51726245007343,
-0.510383830357802,-0.504799176206508,-0.477734550505478,-0.455898128177116,
-0.447143555146704,-0.442467632926928,-0.414733780296404,-0.386572344665108,
-0.358632098172949,-0.344734866599356,-0.340184942209154,-0.311254405969609,
-0.30304317187858,-0.275230199031541,-0.246787090793276,-0.236990270246434,
-0.232158279697281,-0.227903807505874,-0.198913875468756,-0.169351066942439,
-0.13955255925445,-0.12334611597552,-0.118091324130729,-0.113402165305129,
-0.0828552636377898,-0.0522813313134371,-0.022324559840541,-0.0099010130230106,
0.),.UNSPECIFIED.);
#2564=B_SPLINE_CURVE_WITH_KNOTS('',3,(#25495,#25496,#25497,#25498,#25499,
#25500,#25501,#25502,#25503,#25504,#25505,#25506,#25507,#25508,#25509,#25510,
#25511,#25512,#25513,#25514,#25515,#25516,#25517,#25518,#25519,#25520,#25521,
#25522,#25523,#25524,#25525,#25526,#25527,#25528,#25529,#25530,#25531,#25532,
#25533,#25534,#25535,#25536,#25537,#25538,#25539,#25540,#25541,#25542,#25543,
#25544,#25545,#25546,#25547,#25548,#25549,#25550,#25551,#25552,#25553,#25554,
#25555,#25556,#25557,#25558,#25559,#25560,#25561,#25562,#25563,#25564,#25565,
#25566,#25567,#25568,#25569,#25570,#25571,#25572,#25573,#25574,#25575,#25576,
#25577,#25578,#25579,#25580,#25581,#25582,#25583,#25584,#25585,#25586,#25587,
#25588),.UNSPECIFIED.,.F.,.F.,(4,3,3,3,3,3,3,3,3,3,3,3,3,3,3,3,3,3,3,3,
3,3,3,3,3,3,3,3,3,3,3,4),(-0.566847306048102,-0.536662350861785,-0.506055522441016,
-0.497410970877117,-0.490478592762268,-0.460331914265818,-0.437093650808009,
-0.424723077676165,-0.420481376095385,-0.391056955765019,-0.361899168474601,
-0.333575784057379,-0.318788289693871,-0.313125278571146,-0.308695666218845,
-0.280706728188629,-0.274425806603346,-0.24594922105141,-0.216224375904036,
-0.204597160989918,-0.200878778856265,-0.173045052463213,-0.145277293489921,
-0.117981907776077,-0.104252976788119,-0.100010196974054,-0.095829444774943,
-0.0691576524997616,-0.0429343526171,-0.0175124074222168,-0.00815045987241754,
0.),.UNSPECIFIED.);
#2565=B_SPLINE_CURVE_WITH_KNOTS('',3,(#25590,#25591,#25592,#25593,#25594,
#25595,#25596,#25597,#25598,#25599,#25600),.UNSPECIFIED.,.F.,.F.,(4,1,1,
1,1,1,1,1,4),(15.7079632679489,15.8286682231623,16.8210880633759,17.8135079035895,
18.8059277438032,19.7983475840168,20.7907674242304,21.7831872644441,21.9911485751285),
 .UNSPECIFIED.);
#2566=B_SPLINE_CURVE_WITH_KNOTS('',3,(#25601,#25602,#25603,#25604,#25605,
#25606,#25607,#25608,#25609,#25610),.UNSPECIFIED.,.F.,.F.,(4,1,1,1,1,1,
1,4),(15.7079632679489,16.383239807399,17.3756596476127,18.3680794878263,
19.3604993280399,20.3529191682536,21.3453390084672,21.9911485751285),
 .UNSPECIFIED.);
#2567=B_SPLINE_CURVE_WITH_KNOTS('',3,(#26011,#26012,#26013,#26014,#26015,
#26016,#26017,#26018,#26019,#26020,#26021,#26022,#26023,#26024,#26025,#26026,
#26027,#26028,#26029,#26030,#26031,#26032,#26033,#26034,#26035),
 .UNSPECIFIED.,.F.,.F.,(4,3,3,3,3,3,3,3,4),(-10.1321597128207,-9.92419840213631,
-8.93177856192268,-7.93935872170905,-6.94693888149542,-5.95451904128179,
-4.96209920106816,-3.96967936085453,-3.84897440564114),.UNSPECIFIED.);
#2568=B_SPLINE_CURVE_WITH_KNOTS('',3,(#26436,#26437,#26438,#26439,#26440,
#26441,#26442,#26443,#26444,#26445,#26446,#26447,#26448,#26449,#26450,#26451,
#26452,#26453,#26454,#26455,#26456,#26457),.UNSPECIFIED.,.F.,.F.,(4,3,3,
3,3,3,3,4),(7.59274844815661,7.93935872170905,8.93177856192268,9.92419840213631,
10.9166182423499,11.9090380825636,12.9014579227772,13.8759337553362),
 .UNSPECIFIED.);
#2569=B_SPLINE_CURVE_WITH_KNOTS('',3,(#26460,#26461,#26462,#26463,#26464,
#26465,#26466,#26467,#26468,#26469,#26470,#26471,#26472,#26473,#26474,#26475,
#26476,#26477,#26478,#26479,#26480,#26481,#26482,#26483,#26484,#26485,#26486,
#26487,#26488,#26489,#26490,#26491,#26492,#26493,#26494,#26495,#26496,#26497,
#26498,#26499,#26500,#26501,#26502,#26503,#26504,#26505,#26506,#26507,#26508,
#26509,#26510,#26511,#26512,#26513,#26514,#26515,#26516,#26517,#26518,#26519,
#26520,#26521,#26522,#26523,#26524,#26525,#26526,#26527,#26528,#26529,#26530,
#26531,#26532,#26533,#26534,#26535,#26536,#26537,#26538,#26539,#26540,#26541,
#26542,#26543,#26544,#26545,#26546,#26547,#26548,#26549,#26550,#26551,#26552,
#26553),.UNSPECIFIED.,.F.,.F.,(4,3,3,3,3,3,3,3,3,3,3,3,3,3,3,3,3,3,3,3,
3,3,3,3,3,3,3,3,3,3,3,4),(-0.569248610399384,-0.543569235590288,-0.517262478651252,
-0.510383901889905,-0.5047991812893,-0.477734566431476,-0.45589814211236,
-0.447143686501957,-0.442467743120936,-0.414733902739171,-0.386572466363187,
-0.358632212682089,-0.344734952481205,-0.340185022063421,-0.311254485448412,
-0.303043171878551,-0.275230188458927,-0.24678707363057,-0.236990217909345,
-0.232158195033693,-0.227903714787798,-0.198913772270501,-0.169350958285975,
-0.139552450005073,-0.123346020382315,-0.118091100987548,-0.11340214359472,
-0.0828552403272742,-0.052281308311463,-0.0223245354250729,-0.00990101302301064,
0.),.UNSPECIFIED.);
#2570=B_SPLINE_CURVE_WITH_KNOTS('',3,(#26554,#26555,#26556,#26557,#26558,
#26559,#26560,#26561,#26562,#26563,#26564,#26565,#26566,#26567,#26568,#26569,
#26570,#26571,#26572,#26573,#26574,#26575,#26576,#26577,#26578,#26579,#26580,
#26581,#26582,#26583,#26584,#26585,#26586,#26587,#26588,#26589,#26590,#26591,
#26592,#26593,#26594,#26595,#26596,#26597,#26598,#26599,#26600,#26601,#26602,
#26603,#26604,#26605,#26606,#26607,#26608,#26609,#26610,#26611,#26612,#26613,
#26614,#26615,#26616,#26617,#26618,#26619,#26620,#26621,#26622,#26623,#26624,
#26625,#26626,#26627,#26628,#26629,#26630,#26631,#26632,#26633,#26634,#26635,
#26636,#26637,#26638,#26639,#26640,#26641,#26642,#26643,#26644,#26645,#26646,
#26647),.UNSPECIFIED.,.F.,.F.,(4,3,3,3,3,3,3,3,3,3,3,3,3,3,3,3,3,3,3,3,
3,3,3,3,3,3,3,3,3,3,3,4),(-0.566847306048057,-0.536662357910539,-0.506055531265482,
-0.49741098170805,-0.490478594836811,-0.460331915979511,-0.437093652307487,
-0.424723081249797,-0.420481379994704,-0.391056958700494,-0.361899170676201,
-0.333575783700219,-0.318788289425995,-0.31312527916877,-0.308695666742216,
-0.28070672569703,-0.274425806603323,-0.245949220781907,-0.21622437566822,
-0.204597161217252,-0.200878778552373,-0.173045052561144,-0.145277293074677,
-0.117981904358029,-0.104252973797327,-0.100010187224494,-0.0958294424246432,
-0.0691576481481108,-0.0429343440651014,-0.0175123918711586,-0.00815045987241372,
0.),.UNSPECIFIED.);
#2571=B_SPLINE_CURVE_WITH_KNOTS('',3,(#26649,#26650,#26651,#26652,#26653,
#26654,#26655,#26656,#26657,#26658,#26659),.UNSPECIFIED.,.F.,.F.,(4,1,1,
1,1,1,1,1,4),(15.7079632679489,15.8286682231623,16.8210880633759,17.8135079035895,
18.8059277438032,19.7983475840168,20.7907674242304,21.7831872644441,21.9911485751285),
 .UNSPECIFIED.);
#2572=B_SPLINE_CURVE_WITH_KNOTS('',3,(#26660,#26661,#26662,#26663,#26664,
#26665,#26666,#26667,#26668,#26669),.UNSPECIFIED.,.F.,.F.,(4,1,1,1,1,1,
1,4),(15.7079632679489,16.383239807399,17.3756596476127,18.3680794878263,
19.3604993280399,20.3529191682536,21.3453390084672,21.9911485751285),
 .UNSPECIFIED.);
#2573=B_SPLINE_CURVE_WITH_KNOTS('',3,(#27070,#27071,#27072,#27073,#27074,
#27075,#27076,#27077,#27078,#27079,#27080,#27081,#27082,#27083,#27084,#27085,
#27086,#27087,#27088,#27089,#27090,#27091,#27092,#27093,#27094),
 .UNSPECIFIED.,.F.,.F.,(4,3,3,3,3,3,3,3,4),(-10.1321597128207,-9.92419840213631,
-8.93177856192268,-7.93935872170905,-6.94693888149542,-5.95451904128179,
-4.96209920106816,-3.96967936085453,-3.84897440564114),.UNSPECIFIED.);
#2574=B_SPLINE_CURVE_WITH_KNOTS('',3,(#27495,#27496,#27497,#27498,#27499,
#27500,#27501,#27502,#27503,#27504,#27505,#27506,#27507,#27508,#27509,#27510,
#27511,#27512,#27513,#27514,#27515,#27516),.UNSPECIFIED.,.F.,.F.,(4,3,3,
3,3,3,3,4),(7.59274844815661,7.93935872170905,8.93177856192269,9.92419840213631,
10.9166182423499,11.9090380825636,12.9014579227772,13.8759337553362),
 .UNSPECIFIED.);
#2575=B_SPLINE_CURVE_WITH_KNOTS('',3,(#27521,#27522,#27523,#27524,#27525,
#27526,#27527,#27528,#27529,#27530,#27531,#27532,#27533,#27534,#27535,#27536,
#27537,#27538,#27539,#27540,#27541,#27542,#27543,#27544,#27545,#27546,#27547,
#27548,#27549,#27550,#27551),.UNSPECIFIED.,.F.,.F.,(4,3,3,3,3,3,3,3,3,3,
4),(-0.186478347341216,-0.158619634599147,-0.131056531933734,-0.104105248740391,
-0.100056848097327,-0.0957909510082901,-0.0691196899172101,-0.0428971352288845,
-0.0174757607808009,-0.00815045987241733,0.),.UNSPECIFIED.);
#2576=B_SPLINE_CURVE_WITH_KNOTS('',3,(#27555,#27556,#27557,#27558,#27559,
#27560,#27561,#27562,#27563,#27564,#27565,#27566,#27567,#27568,#27569,#27570,
#27571,#27572,#27573,#27574,#27575,#27576,#27577,#27578,#27579,#27580,#27581,
#27582,#27583,#27584,#27585,#27586,#27587,#27588,#27589,#27590,#27591,#27592,
#27593,#27594,#27595,#27596,#27597,#27598,#27599,#27600,#27601,#27602,#27603,
#27604,#27605,#27606,#27607,#27608,#27609,#27610,#27611,#27612,#27613,#27614,
#27615,#27616,#27617,#27618),.UNSPECIFIED.,.F.,.F.,(4,3,3,3,3,3,3,3,3,3,
3,3,3,3,3,3,3,3,3,3,3,4),(-0.382265902471371,-0.354388912953647,-0.344229210342304,
-0.337959875745192,-0.309029041715164,-0.303043171878561,-0.275230178847725,
-0.246787058020227,-0.236990170309578,-0.232158118032837,-0.227903630488106,
-0.198913678448654,-0.169350859502243,-0.139552350678771,-0.123345933471801,
-0.118090898210581,-0.113402123852804,-0.0828552191246252,-0.0522812873900625,
-0.0223245132224302,-0.00990101302301068,0.),.UNSPECIFIED.);
#2577=B_SPLINE_CURVE_WITH_KNOTS('',3,(#27619,#27620,#27621,#27622,#27623,
#27624,#27625,#27626,#27627,#27628,#27629,#27630,#27631,#27632,#27633,#27634,
#27635,#27636,#27637,#27638,#27639,#27640,#27641,#27642,#27643,#27644,#27645,
#27646,#27647,#27648,#27649,#27650,#27651,#27652,#27653,#27654,#27655,#27656,
#27657,#27658,#27659,#27660,#27661,#27662,#27663,#27664,#27665,#27666,#27667,
#27668,#27669,#27670,#27671,#27672,#27673,#27674,#27675,#27676,#27677,#27678,
#27679,#27680,#27681,#27682),.UNSPECIFIED.,.F.,.F.,(4,3,3,3,3,3,3,3,3,3,
3,3,3,3,3,3,3,3,3,3,3,4),(-0.566847306048054,-0.536662333984777,-0.506055501317574,
-0.49741094495226,-0.490478587792416,-0.46033191015455,-0.437093647210649,
-0.424723069108858,-0.42048136705109,-0.391056949034952,-0.361899163427049,
-0.333575785136632,-0.318788290503309,-0.313125277598956,-0.308695665438203,
-0.280706734635303,-0.274425806603339,-0.24586775158787,-0.216173049464543,
-0.206760965590708,-0.202702619221145,-0.186478347341216),.UNSPECIFIED.);
#2578=B_SPLINE_CURVE_WITH_KNOTS('',3,(#27687,#27688,#27689,#27690,#27691,
#27692,#27693,#27694,#27695,#27696,#27697,#27698,#27699,#27700,#27701,#27702,
#27703,#27704,#27705,#27706,#27707,#27708,#27709,#27710,#27711,#27712,#27713,
#27714,#27715,#27716,#27717,#27718,#27719,#27720),.UNSPECIFIED.,.F.,.F.,
(4,3,3,3,3,3,3,3,3,3,3,4),(-0.569248610399408,-0.543383188674187,-0.523243527898835,
-0.5111120528569,-0.504565698233315,-0.477731171126537,-0.453864853962746,
-0.447746320338163,-0.443048137353461,-0.415379481235353,-0.38724361464334,
-0.382265902471371),.UNSPECIFIED.);
#2579=B_SPLINE_CURVE_WITH_KNOTS('',3,(#27722,#27723,#27724,#27725,#27726,
#27727,#27728,#27729,#27730,#27731,#27732),.UNSPECIFIED.,.F.,.F.,(4,1,1,
1,1,1,1,1,4),(15.7079632679489,15.8286682231623,16.8210880633759,17.8135079035895,
18.8059277438032,19.7983475840168,20.7907674242304,21.7831872644441,21.9911485751285),
 .UNSPECIFIED.);
#2580=B_SPLINE_CURVE_WITH_KNOTS('',3,(#27733,#27734,#27735,#27736,#27737,
#27738,#27739,#27740,#27741,#27742),.UNSPECIFIED.,.F.,.F.,(4,1,1,1,1,1,
1,4),(15.7079632679489,16.383239807399,17.3756596476127,18.3680794878263,
19.3604993280399,20.3529191682536,21.3453390084672,21.9911485751285),
 .UNSPECIFIED.);
#2581=B_SPLINE_CURVE_WITH_KNOTS('',3,(#28143,#28144,#28145,#28146,#28147,
#28148,#28149,#28150,#28151,#28152,#28153,#28154,#28155,#28156,#28157,#28158,
#28159,#28160,#28161,#28162,#28163,#28164,#28165,#28166,#28167),
 .UNSPECIFIED.,.F.,.F.,(4,3,3,3,3,3,3,3,4),(-10.1321597128207,-9.92419840213631,
-8.93177856192268,-7.93935872170905,-6.94693888149542,-5.95451904128179,
-4.96209920106816,-3.96967936085453,-3.84897440564114),.UNSPECIFIED.);
#2582=B_SPLINE_CURVE_WITH_KNOTS('',3,(#28568,#28569,#28570,#28571,#28572,
#28573,#28574,#28575,#28576,#28577,#28578,#28579,#28580,#28581,#28582,#28583,
#28584,#28585,#28586,#28587,#28588,#28589),.UNSPECIFIED.,.F.,.F.,(4,3,3,
3,3,3,3,4),(7.59274844815661,7.93935872170905,8.93177856192269,9.92419840213631,
10.9166182423499,11.9090380825636,12.9014579227772,13.8759337553362),
 .UNSPECIFIED.);
#2583=B_SPLINE_CURVE_WITH_KNOTS('',3,(#28592,#28593,#28594,#28595,#28596,
#28597,#28598,#28599,#28600,#28601),.UNSPECIFIED.,.F.,.F.,(4,2,2,2,4),(1.93603633322311,
2.0327017356838,2.12936713814449,2.22630536900611,2.32324359986774),
 .UNSPECIFIED.);
#2584=B_SPLINE_CURVE_WITH_KNOTS('',3,(#28602,#28603,#28604,#28605,#28606,
#28607,#28608,#28609,#28610,#28611),.UNSPECIFIED.,.F.,.F.,(4,2,2,2,4),(0.774414533289245,
0.871352764150867,0.968290995012489,1.06495639747318,1.16162179993387),
 .UNSPECIFIED.);
#2585=B_SPLINE_CURVE_WITH_KNOTS('',3,(#28615,#28616,#28617,#28618,#28619,
#28620,#28621,#28622,#28623,#28624,#28625,#28626,#28627,#28628,#28629,#28630,
#28631,#28632,#28633,#28634,#28635,#28636,#28637,#28638,#28639,#28640,#28641,
#28642,#28643,#28644,#28645),.UNSPECIFIED.,.F.,.F.,(4,3,3,3,3,3,3,3,3,3,
4),(-0.186478347341219,-0.158619634855163,-0.131056530031512,-0.104105241249995,
-0.100056821695491,-0.0957909465603036,-0.0691196829588407,-0.0428971229819699,
-0.0174757397045835,-0.00815045987241733,0.),.UNSPECIFIED.);
#2586=B_SPLINE_CURVE_WITH_KNOTS('',3,(#28649,#28650,#28651,#28652,#28653,
#28654,#28655,#28656,#28657,#28658,#28659,#28660,#28661,#28662,#28663,#28664,
#28665,#28666,#28667,#28668,#28669,#28670,#28671,#28672,#28673,#28674,#28675,
#28676,#28677,#28678,#28679,#28680,#28681,#28682,#28683,#28684,#28685,#28686,
#28687,#28688,#28689,#28690,#28691,#28692,#28693,#28694,#28695,#28696,#28697,
#28698,#28699,#28700,#28701,#28702,#28703,#28704,#28705,#28706,#28707,#28708,
#28709,#28710,#28711,#28712),.UNSPECIFIED.,.F.,.F.,(4,3,3,3,3,3,3,3,3,3,
3,3,3,3,3,3,3,3,3,3,3,4),(-0.382265902471371,-0.354388907971518,-0.344229193097268,
-0.337959880834284,-0.309029046216205,-0.303043171878561,-0.275230170211377,
-0.246787044002095,-0.236990127562464,-0.232158048919115,-0.227903554968478,
-0.198913594373769,-0.169350770972404,-0.139552261670151,-0.123345855589258,
-0.11809071636682,-0.11340210613496,-0.0828552000931288,-0.0522812686134481,
-0.0223244932935985,-0.00990101302301068,0.),.UNSPECIFIED.);
#2587=B_SPLINE_CURVE_WITH_KNOTS('',3,(#28713,#28714,#28715,#28716,#28717,
#28718,#28719,#28720,#28721,#28722,#28723,#28724,#28725,#28726,#28727,#28728,
#28729,#28730,#28731,#28732,#28733,#28734,#28735,#28736,#28737,#28738,#28739,
#28740,#28741,#28742,#28743,#28744,#28745,#28746,#28747,#28748,#28749,#28750,
#28751,#28752,#28753,#28754,#28755,#28756,#28757,#28758,#28759,#28760,#28761,
#28762,#28763,#28764,#28765,#28766,#28767,#28768,#28769,#28770,#28771,#28772,
#28773,#28774,#28775,#28776),.UNSPECIFIED.,.F.,.F.,(4,3,3,3,3,3,3,3,3,3,
3,3,3,3,3,3,3,3,3,3,3,4),(-0.566847306048054,-0.53666234288915,-0.506055512459245,
-0.497410958629855,-0.490478590394541,-0.460331912302746,-0.43709364909032,
-0.424723073596147,-0.420481371815357,-0.391056952578469,-0.361899166084687,
-0.333575784563524,-0.318788290073478,-0.313125278104711,-0.308695665838356,
-0.280706731221203,-0.274425806603339,-0.24586775166354,-0.21617304950238,
-0.206760964784706,-0.20270261672099,-0.186478347341219),.UNSPECIFIED.);
#2588=B_SPLINE_CURVE_WITH_KNOTS('',3,(#28781,#28782,#28783,#28784,#28785,
#28786,#28787,#28788,#28789,#28790,#28791,#28792,#28793,#28794,#28795,#28796,
#28797,#28798,#28799,#28800,#28801,#28802,#28803,#28804,#28805,#28806,#28807,
#28808,#28809,#28810,#28811,#28812,#28813,#28814),.UNSPECIFIED.,.F.,.F.,
(4,3,3,3,3,3,3,3,3,3,3,4),(-0.569248610399408,-0.543383200898257,-0.523243538594896,
-0.511112056843439,-0.504565699175182,-0.477731182424187,-0.453864862435983,
-0.447746321418146,-0.443048138290636,-0.415379490937535,-0.387243626784474,
-0.382265902471371),.UNSPECIFIED.);
#2589=B_SPLINE_CURVE_WITH_KNOTS('',3,(#28816,#28817,#28818,#28819,#28820,
#28821,#28822,#28823,#28824,#28825,#28826),.UNSPECIFIED.,.F.,.F.,(4,1,1,
1,1,1,1,1,4),(15.7079632679489,15.8286682231623,16.8210880633759,17.8135079035895,
18.8059277438032,19.7983475840168,20.7907674242304,21.7831872644441,21.9911485751285),
 .UNSPECIFIED.);
#2590=B_SPLINE_CURVE_WITH_KNOTS('',3,(#28827,#28828,#28829,#28830,#28831,
#28832,#28833,#28834,#28835,#28836),.UNSPECIFIED.,.F.,.F.,(4,1,1,1,1,1,
1,4),(15.7079632679489,16.383239807399,17.3756596476127,18.3680794878263,
19.3604993280399,20.3529191682536,21.3453390084672,21.9911485751285),
 .UNSPECIFIED.);
#2591=B_SPLINE_CURVE_WITH_KNOTS('',3,(#29237,#29238,#29239,#29240,#29241,
#29242,#29243,#29244,#29245,#29246,#29247,#29248,#29249,#29250,#29251,#29252,
#29253,#29254,#29255,#29256,#29257,#29258,#29259,#29260,#29261),
 .UNSPECIFIED.,.F.,.F.,(4,3,3,3,3,3,3,3,4),(-10.1321597128207,-9.92419840213631,
-8.93177856192268,-7.93935872170905,-6.94693888149542,-5.95451904128179,
-4.96209920106816,-3.96967936085453,-3.84897440564114),.UNSPECIFIED.);
#2592=B_SPLINE_CURVE_WITH_KNOTS('',3,(#29662,#29663,#29664,#29665,#29666,
#29667,#29668,#29669,#29670,#29671,#29672,#29673,#29674,#29675,#29676,#29677,
#29678,#29679,#29680,#29681,#29682,#29683),.UNSPECIFIED.,.F.,.F.,(4,3,3,
3,3,3,3,4),(7.59274844815661,7.93935872170905,8.93177856192269,9.92419840213631,
10.9166182423499,11.9090380825636,12.9014579227772,13.8759337553362),
 .UNSPECIFIED.);
#2593=B_SPLINE_CURVE_WITH_KNOTS('',3,(#29686,#29687,#29688,#29689,#29690,
#29691,#29692,#29693,#29694,#29695),.UNSPECIFIED.,.F.,.F.,(4,2,2,2,4),(1.93603633322311,
2.0327017356838,2.12936713814449,2.22630536900611,2.32324359986774),
 .UNSPECIFIED.);
#2594=B_SPLINE_CURVE_WITH_KNOTS('',3,(#29696,#29697,#29698,#29699,#29700,
#29701,#29702,#29703,#29704,#29705),.UNSPECIFIED.,.F.,.F.,(4,2,2,2,4),(0.774414533289245,
0.871352764150867,0.968290995012489,1.06495639747318,1.16162179993387),
 .UNSPECIFIED.);
#2595=B_SPLINE_CURVE_WITH_KNOTS('',3,(#29711,#29712,#29713,#29714,#29715,
#29716,#29717,#29718,#29719,#29720,#29721,#29722,#29723,#29724,#29725,#29726,
#29727,#29728,#29729,#29730,#29731,#29732,#29733,#29734,#29735,#29736,#29737,
#29738,#29739,#29740,#29741,#29742,#29743,#29744,#29745,#29746,#29747,#29748,
#29749,#29750,#29751,#29752,#29753,#29754,#29755,#29756,#29757,#29758,#29759,
#29760,#29761,#29762,#29763,#29764,#29765,#29766,#29767,#29768,#29769,#29770,
#29771,#29772,#29773,#29774,#29775,#29776,#29777,#29778,#29779,#29780,#29781,
#29782,#29783,#29784,#29785,#29786,#29787,#29788,#29789,#29790,#29791,#29792,
#29793,#29794,#29795,#29796,#29797,#29798),.UNSPECIFIED.,.F.,.F.,(4,3,3,
3,3,3,3,3,3,3,3,3,3,3,3,3,3,3,3,3,3,3,3,3,3,3,3,3,3,4),(-0.378621596831415,
-0.359797488651071,-0.347859564017193,-0.339721384340795,-0.335383707835788,
-0.315512004032695,-0.301177697597527,-0.297260794867737,-0.293227238012395,
-0.27282498756368,-0.252127330348507,-0.239304885899219,-0.228805595020818,
-0.224505148589752,-0.203200592223416,-0.200837552551353,-0.18035024909426,
-0.158310752857967,-0.154330298823938,-0.150809435172749,-0.129426160732041,
-0.10759198857076,-0.085625366894301,-0.0802031148086871,-0.0759441736813679,
-0.0533965995856124,-0.030824430585221,-0.00876579303116958,-0.0040342792039134,
0.),.UNSPECIFIED.);
#2596=B_SPLINE_CURVE_WITH_KNOTS('',3,(#29799,#29800,#29801,#29802,#29803,
#29804,#29805,#29806,#29807,#29808,#29809,#29810,#29811,#29812,#29813,#29814,
#29815,#29816,#29817,#29818,#29819,#29820,#29821,#29822,#29823,#29824,#29825,
#29826,#29827,#29828,#29829,#29830,#29831,#29832,#29833,#29834,#29835,#29836,
#29837,#29838,#29839,#29840,#29841,#29842,#29843,#29844,#29845,#29846,#29847,
#29848,#29849,#29850,#29851,#29852,#29853,#29854,#29855,#29856,#29857,#29858,
#29859,#29860,#29861,#29862,#29863,#29864,#29865,#29866,#29867,#29868,#29869,
#29870,#29871,#29872,#29873,#29874,#29875,#29876,#29877,#29878,#29879,#29880,
#29881,#29882,#29883),.UNSPECIFIED.,.F.,.F.,(4,3,3,3,3,3,3,3,3,3,3,3,3,
3,3,3,3,3,3,3,3,3,3,3,3,3,3,3,4),(-0.376940817211644,-0.354634297224817,
-0.332912868281746,-0.328064575910149,-0.305815976299773,-0.290196837472332,
-0.284261042344383,-0.278600436982198,-0.256917266795448,-0.235699705654349,
-0.214947482958391,-0.208197203240807,-0.204402057618207,-0.183825925259162,
-0.180862865680244,-0.159880209119453,-0.140305785753204,-0.136021308905087,
-0.132587897579495,-0.112128579246988,-0.0917639886504933,-0.0718357414527914,
-0.0676216417654861,-0.0636601334983857,-0.0441022477646612,-0.0249163166467412,
-0.00635335474236993,-0.00328482218946179,0.),.UNSPECIFIED.);
#2597=B_SPLINE_CURVE_WITH_KNOTS('',3,(#29885,#29886,#29887,#29888,#29889,
#29890,#29891,#29892,#29893,#29894,#29895),.UNSPECIFIED.,.F.,.F.,(4,1,1,
1,1,1,1,1,4),(15.7079632679489,15.851694142003,16.8492226764396,17.8467512108762,
18.8442797453128,19.8418082797494,20.839336814186,21.8368653486226,21.9911485751285),
 .UNSPECIFIED.);
#2598=B_SPLINE_CURVE_WITH_KNOTS('',3,(#29896,#29897,#29898,#29899,#29900,
#29901,#29902,#29903,#29904,#29905),.UNSPECIFIED.,.F.,.F.,(4,1,1,1,1,1,
1,4),(15.7079632679489,16.39319808165,17.3907266160866,18.3882551505232,
19.3857836849598,20.3833122193964,21.380840753833,21.9911485751284),
 .UNSPECIFIED.);
#2599=B_SPLINE_CURVE_WITH_KNOTS('',3,(#30322,#30323,#30324,#30325,#30326,
#30327,#30328,#30329,#30330,#30331,#30332,#30333,#30334,#30335,#30336,#30337,
#30338,#30339,#30340,#30341,#30342,#30343,#30344,#30345,#30346,#30347,#30348,
#30349,#30350,#30351,#30352,#30353,#30354,#30355,#30356,#30357,#30358,#30359,
#30360,#30361,#30362,#30363,#30364,#30365,#30366,#30367,#30368,#30369,#30370,
#30371,#30372,#30373,#30374,#30375,#30376,#30377,#30378,#30379,#30380,#30381,
#30382,#30383,#30384,#30385,#30386,#30387,#30388,#30389,#30390,#30391,#30392,
#30393,#30394,#30395,#30396,#30397,#30398,#30399,#30400,#30401,#30402,#30403),
 .UNSPECIFIED.,.F.,.F.,(4,3,3,3,3,3,3,3,3,3,3,3,3,3,3,3,3,3,3,3,3,3,3,3,
3,3,3,4),(0.,0.0185974702011865,0.0384224406125438,0.0557692897224814,0.0644714144177272,
0.0684505998290036,0.0885047671947535,0.108914689664935,0.125985325621712,
0.133848200607443,0.137284581833955,0.158359464766614,0.177197233492045,
0.197725006274794,0.20564964402825,0.20912533594064,0.230131014427894,0.251623268601124,
0.268075190636431,0.278317576716938,0.284044648983082,0.306313636977894,
0.322966020148207,0.328172647466716,0.333184029352957,0.355705443842072,
0.372923169659143,0.376940817211587),.UNSPECIFIED.);
#2600=B_SPLINE_CURVE_WITH_KNOTS('',3,(#30404,#30405,#30406,#30407,#30408,
#30409,#30410,#30411,#30412,#30413,#30414,#30415,#30416,#30417,#30418,#30419,
#30420,#30421,#30422,#30423,#30424,#30425,#30426,#30427,#30428),
 .UNSPECIFIED.,.F.,.F.,(4,3,3,3,3,3,3,3,4),(-10.1295685708719,-9.975285344366,
-8.9777568099294,-7.9802282754928,-6.9826997410562,-5.9851712066196,-4.987642672183,
-3.9901141377464,-3.84638326369234),.UNSPECIFIED.);
#2601=B_SPLINE_CURVE_WITH_KNOTS('',3,(#30845,#30846,#30847,#30848,#30849,
#30850,#30851,#30852,#30853,#30854,#30855,#30856,#30857,#30858,#30859,#30860,
#30861,#30862,#30863,#30864,#30865,#30866),.UNSPECIFIED.,.F.,.F.,(4,3,3,
3,3,3,3,4),(7.59300756235157,7.9802282754928,8.9777568099294,9.975285344366,
10.9728138788026,11.9703424132392,12.9678709476758,13.8761928695312),
 .UNSPECIFIED.);
#2602=B_SPLINE_CURVE_WITH_KNOTS('',3,(#30867,#30868,#30869,#30870,#30871,
#30872,#30873,#30874,#30875,#30876,#30877,#30878,#30879,#30880,#30881,#30882,
#30883,#30884,#30885,#30886,#30887,#30888,#30889,#30890,#30891,#30892,#30893,
#30894,#30895,#30896,#30897,#30898,#30899,#30900,#30901,#30902,#30903,#30904,
#30905,#30906,#30907,#30908,#30909,#30910,#30911,#30912,#30913,#30914,#30915,
#30916,#30917,#30918,#30919,#30920,#30921,#30922,#30923,#30924,#30925,#30926,
#30927,#30928,#30929,#30930,#30931,#30932,#30933,#30934,#30935,#30936,#30937,
#30938,#30939,#30940,#30941,#30942,#30943,#30944,#30945,#30946,#30947,#30948,
#30949,#30950,#30951),.UNSPECIFIED.,.F.,.F.,(4,3,3,3,3,3,3,3,3,3,3,3,3,
3,3,3,3,3,3,3,3,3,3,3,3,3,3,3,4),(0.,0.0219661302700472,0.0445436036366041,
0.06362009313796,0.0720969467217393,0.0767544176956762,0.0810485403387707,
0.102995140835155,0.124771437273058,0.142867457866657,0.150422750087673,
0.153917807515336,0.157566643421491,0.178337400691585,0.197155519647451,
0.219426672701591,0.224328239844768,0.22940123318273,0.25006631851888,0.27072713343305,
0.285676237002597,0.296892227344257,0.30062314254954,0.320395494413919,
0.334302188530373,0.338768597396786,0.357793672729449,0.375324744080571,
0.378621596831418),.UNSPECIFIED.);
#2603=B_SPLINE_CURVE_WITH_KNOTS('',3,(#30954,#30955,#30956,#30957,#30958,
#30959,#30960,#30961,#30962,#30963,#30964,#30965,#30966,#30967,#30968,#30969,
#30970,#30971,#30972,#30973,#30974,#30975,#30976,#30977,#30978,#30979,#30980,
#30981,#30982,#30983,#30984,#30985,#30986,#30987,#30988,#30989,#30990,#30991,
#30992,#30993,#30994,#30995,#30996,#30997,#30998,#30999,#31000,#31001,#31002,
#31003,#31004,#31005,#31006,#31007,#31008,#31009,#31010,#31011,#31012,#31013,
#31014,#31015,#31016,#31017,#31018,#31019,#31020,#31021,#31022,#31023,#31024,
#31025,#31026,#31027,#31028,#31029,#31030,#31031,#31032,#31033,#31034,#31035,
#31036,#31037,#31038,#31039,#31040,#31041),.UNSPECIFIED.,.F.,.F.,(4,3,3,
3,3,3,3,3,3,3,3,3,3,3,3,3,3,3,3,3,3,3,3,3,3,3,3,3,3,4),(-0.378621596831449,
-0.359797495255613,-0.347859580799326,-0.339721534947358,-0.335383781754089,
-0.31551208410872,-0.301177767664049,-0.297260953938726,-0.293227258605859,
-0.272825012825785,-0.252127354965836,-0.239304904362215,-0.228805622237141,
-0.224505157276384,-0.203200600638345,-0.200837552551351,-0.180350244595754,
-0.158310748921773,-0.154330272617166,-0.150809430446371,-0.129426152351927,
-0.107591978572832,-0.0856253568644043,-0.0802030973073672,-0.0759441676007146,
-0.0533965927429803,-0.0308244238812939,-0.00876578556903723,-0.00403427920390745,
0.),.UNSPECIFIED.);
#2604=B_SPLINE_CURVE_WITH_KNOTS('',3,(#31042,#31043,#31044,#31045,#31046,
#31047,#31048,#31049,#31050,#31051,#31052,#31053,#31054,#31055,#31056,#31057,
#31058,#31059,#31060,#31061,#31062,#31063,#31064,#31065,#31066,#31067,#31068,
#31069,#31070,#31071,#31072,#31073,#31074,#31075,#31076,#31077,#31078,#31079,
#31080,#31081,#31082,#31083,#31084,#31085,#31086,#31087,#31088,#31089,#31090,
#31091,#31092,#31093,#31094,#31095,#31096,#31097,#31098,#31099,#31100,#31101,
#31102,#31103,#31104,#31105,#31106,#31107,#31108,#31109,#31110,#31111,#31112,
#31113,#31114,#31115,#31116,#31117,#31118,#31119,#31120,#31121,#31122,#31123,
#31124,#31125,#31126),.UNSPECIFIED.,.F.,.F.,(4,3,3,3,3,3,3,3,3,3,3,3,3,
3,3,3,3,3,3,3,3,3,3,3,3,3,3,3,4),(-0.376940817211602,-0.354634286106805,
-0.332912858553484,-0.328064564631197,-0.305815965171254,-0.290196827734877,
-0.284261020742464,-0.278600438394339,-0.25691727004817,-0.235699713647721,
-0.214947494052335,-0.208197196081605,-0.204402058518297,-0.183825930761354,
-0.180862865680241,-0.159880209155866,-0.140305785785065,-0.136021316510379,
-0.132587903785407,-0.112128584732708,-0.0917639954653299,-0.0718357542938654,
-0.067621677650879,-0.0636601454777048,-0.0441022630341506,-0.0249163391034165,
-0.00635338900437089,-0.00328482218946166,0.),.UNSPECIFIED.);
#2605=B_SPLINE_CURVE_WITH_KNOTS('',3,(#31128,#31129,#31130,#31131,#31132,
#31133,#31134,#31135,#31136,#31137,#31138),.UNSPECIFIED.,.F.,.F.,(4,1,1,
1,1,1,1,1,4),(15.7079632679489,15.851694142003,16.8492226764396,17.8467512108762,
18.8442797453128,19.8418082797494,20.839336814186,21.8368653486226,21.9911485751285),
 .UNSPECIFIED.);
#2606=B_SPLINE_CURVE_WITH_KNOTS('',3,(#31139,#31140,#31141,#31142,#31143,
#31144,#31145,#31146,#31147,#31148),.UNSPECIFIED.,.F.,.F.,(4,1,1,1,1,1,
1,4),(15.7079632679489,16.3931980816501,17.3907266160867,18.3882551505233,
19.3857836849599,20.3833122193965,21.3808407538331,21.9911485751285),
 .UNSPECIFIED.);
#2607=B_SPLINE_CURVE_WITH_KNOTS('',3,(#31565,#31566,#31567,#31568,#31569,
#31570,#31571,#31572,#31573,#31574,#31575,#31576,#31577,#31578,#31579,#31580,
#31581,#31582,#31583,#31584,#31585,#31586,#31587,#31588,#31589,#31590,#31591,
#31592,#31593,#31594,#31595,#31596,#31597,#31598,#31599,#31600,#31601,#31602,
#31603,#31604,#31605,#31606,#31607,#31608,#31609,#31610,#31611,#31612,#31613,
#31614,#31615,#31616,#31617,#31618,#31619,#31620,#31621,#31622,#31623,#31624,
#31625,#31626,#31627,#31628,#31629,#31630,#31631,#31632,#31633,#31634,#31635,
#31636,#31637,#31638,#31639,#31640,#31641,#31642,#31643,#31644,#31645,#31646),
 .UNSPECIFIED.,.F.,.F.,(4,3,3,3,3,3,3,3,3,3,3,3,3,3,3,3,3,3,3,3,3,3,3,3,
3,3,3,4),(0.,0.0185974884483997,0.038422456578859,0.0557693036930108,0.0644714385966712,
0.0684506061088201,0.0885047864975771,0.108914714586146,0.125985344312628,
0.133848230034327,0.137284597158202,0.15835947839364,0.177197233492074,
0.197724997131683,0.205649639196346,0.209125332530892,0.230131000272577,
0.25162324878857,0.268075195219975,0.278317587273375,0.284044646363506,
0.30631363368784,0.32296601768069,0.328172641994334,0.33318402658793,0.355705441161373,
0.37292316965924,0.376940817211689),.UNSPECIFIED.);
#2608=B_SPLINE_CURVE_WITH_KNOTS('',3,(#31647,#31648,#31649,#31650,#31651,
#31652,#31653,#31654,#31655,#31656,#31657,#31658,#31659,#31660,#31661,#31662,
#31663,#31664,#31665,#31666,#31667,#31668,#31669,#31670,#31671),
 .UNSPECIFIED.,.F.,.F.,(4,3,3,3,3,3,3,3,4),(-10.1295685708719,-9.975285344366,
-8.9777568099294,-7.9802282754928,-6.9826997410562,-5.98517120661959,-4.98764267218299,
-3.9901141377464,-3.8463832636923),.UNSPECIFIED.);
#2609=B_SPLINE_CURVE_WITH_KNOTS('',3,(#32088,#32089,#32090,#32091,#32092,
#32093,#32094,#32095,#32096,#32097,#32098,#32099,#32100,#32101,#32102,#32103,
#32104,#32105,#32106,#32107,#32108,#32109),.UNSPECIFIED.,.F.,.F.,(4,3,3,
3,3,3,3,4),(7.59300756235153,7.98022827549279,8.97775680992939,9.97528534436599,
10.9728138788026,11.9703424132392,12.9678709476758,13.8761928695311),
 .UNSPECIFIED.);
#2610=B_SPLINE_CURVE_WITH_KNOTS('',3,(#32110,#32111,#32112,#32113,#32114,
#32115,#32116,#32117,#32118,#32119,#32120,#32121,#32122,#32123,#32124,#32125,
#32126,#32127,#32128,#32129,#32130,#32131,#32132,#32133,#32134,#32135,#32136,
#32137,#32138,#32139,#32140,#32141,#32142,#32143,#32144,#32145,#32146,#32147,
#32148,#32149,#32150,#32151,#32152,#32153,#32154,#32155,#32156,#32157,#32158,
#32159,#32160,#32161,#32162,#32163,#32164,#32165,#32166,#32167,#32168,#32169,
#32170,#32171,#32172,#32173,#32174,#32175,#32176,#32177,#32178,#32179,#32180,
#32181,#32182,#32183,#32184,#32185,#32186,#32187,#32188,#32189,#32190,#32191,
#32192,#32193,#32194),.UNSPECIFIED.,.F.,.F.,(4,3,3,3,3,3,3,3,3,3,3,3,3,
3,3,3,3,3,3,3,3,3,3,3,3,3,3,3,4),(0.,0.0219661245323709,0.0445435973437788,
0.0636200876317427,0.0720969450783383,0.0767544142172396,0.0810485394126128,
0.102995140020355,0.124771438188379,0.142867458553157,0.150422749787228,
0.153917805670854,0.15756664284234,0.178337401835923,0.197155519647491,
0.219426672701635,0.224328240299076,0.229401233191324,0.250066318299861,
0.27072713341503,0.285676242163978,0.296892236301983,0.30062314509683,0.320395498999285,
0.33430219613105,0.338768604407738,0.35779368297658,0.375324744080643,0.37862159683149),
 .UNSPECIFIED.);
#2611=B_SPLINE_CURVE_WITH_KNOTS('',3,(#32197,#32198,#32199,#32200,#32201,
#32202,#32203,#32204,#32205,#32206,#32207,#32208,#32209,#32210,#32211,#32212,
#32213,#32214,#32215,#32216,#32217,#32218,#32219,#32220,#32221,#32222,#32223,
#32224,#32225,#32226,#32227,#32228,#32229,#32230,#32231,#32232,#32233,#32234,
#32235,#32236,#32237,#32238,#32239,#32240,#32241,#32242,#32243,#32244,#32245,
#32246,#32247,#32248,#32249,#32250,#32251,#32252,#32253,#32254,#32255,#32256,
#32257,#32258,#32259,#32260,#32261,#32262,#32263,#32264,#32265,#32266,#32267,
#32268,#32269,#32270,#32271,#32272,#32273,#32274,#32275,#32276,#32277,#32278,
#32279,#32280,#32281,#32282,#32283,#32284),.UNSPECIFIED.,.F.,.F.,(4,3,3,
3,3,3,3,3,3,3,3,3,3,3,3,3,3,3,3,3,3,3,3,3,3,3,3,3,3,4),(-0.378621596831488,
-0.359797481501605,-0.347859545826129,-0.339721221124185,-0.335383627670914,
-0.315511917204206,-0.3011776216226,-0.297260622327209,-0.293227215665992,
-0.27282496017426,-0.252127303658145,-0.239304865881448,-0.228805565513104,
-0.224505139143286,-0.203200583084544,-0.200837552551356,-0.180350253956889,
-0.158310757112766,-0.154330327284575,-0.150809440304414,-0.129426169815667,
-0.10759199940592,-0.0856253777649029,-0.0802031337731618,-0.0759441802619393,
-0.0533966069861228,-0.030824437843487,-0.0087658011087857,-0.00403427920390734,
0.),.UNSPECIFIED.);
#2612=B_SPLINE_CURVE_WITH_KNOTS('',3,(#32285,#32286,#32287,#32288,#32289,
#32290,#32291,#32292,#32293,#32294,#32295,#32296,#32297,#32298,#32299,#32300,
#32301,#32302,#32303,#32304,#32305,#32306,#32307,#32308,#32309,#32310,#32311,
#32312,#32313,#32314,#32315,#32316,#32317,#32318,#32319,#32320,#32321,#32322,
#32323,#32324,#32325,#32326,#32327,#32328,#32329,#32330,#32331,#32332,#32333,
#32334,#32335,#32336,#32337,#32338,#32339,#32340,#32341,#32342,#32343,#32344,
#32345,#32346,#32347,#32348,#32349,#32350,#32351,#32352,#32353,#32354,#32355,
#32356,#32357,#32358,#32359,#32360,#32361,#32362,#32363,#32364,#32365,#32366,
#32367,#32368,#32369),.UNSPECIFIED.,.F.,.F.,(4,3,3,3,3,3,3,3,3,3,3,3,3,
3,3,3,3,3,3,3,3,3,3,3,3,3,3,3,4),(-0.376940817211602,-0.354634293861075,
-0.33291286533847,-0.328064572493281,-0.305815972928742,-0.290196834522679,
-0.284261035801492,-0.278600437373896,-0.256917267743233,-0.23569970803568,
-0.214947486273917,-0.208197201094579,-0.204402057890941,-0.18382592692174,
-0.180862865680237,-0.159880209131733,-0.140305785763948,-0.136021311207514,
-0.132587899444004,-0.112128580894037,-0.0917639906987552,-0.0718357453221696,
-0.067621652583724,-0.0636601371117171,-0.0441022523717969,-0.0249163234274699,
-0.00635336509323165,-0.00328482218945463,0.),.UNSPECIFIED.);
#2613=B_SPLINE_CURVE_WITH_KNOTS('',3,(#32371,#32372,#32373,#32374,#32375,
#32376,#32377,#32378,#32379,#32380,#32381),.UNSPECIFIED.,.F.,.F.,(4,1,1,
1,1,1,1,1,4),(15.7079632679489,15.851694142003,16.8492226764396,17.8467512108762,
18.8442797453128,19.8418082797494,20.839336814186,21.8368653486226,21.9911485751284),
 .UNSPECIFIED.);
#2614=B_SPLINE_CURVE_WITH_KNOTS('',3,(#32382,#32383,#32384,#32385,#32386,
#32387,#32388,#32389,#32390,#32391),.UNSPECIFIED.,.F.,.F.,(4,1,1,1,1,1,
1,4),(15.7079632679489,16.3931980816501,17.3907266160867,18.3882551505233,
19.3857836849599,20.3833122193965,21.3808407538331,21.9911485751284),
 .UNSPECIFIED.);
#2615=B_SPLINE_CURVE_WITH_KNOTS('',3,(#32808,#32809,#32810,#32811,#32812,
#32813,#32814,#32815,#32816,#32817,#32818,#32819,#32820,#32821,#32822,#32823,
#32824,#32825,#32826,#32827,#32828,#32829,#32830,#32831,#32832,#32833,#32834,
#32835,#32836,#32837,#32838,#32839,#32840,#32841,#32842,#32843,#32844,#32845,
#32846,#32847,#32848,#32849,#32850,#32851,#32852,#32853,#32854,#32855,#32856,
#32857,#32858,#32859,#32860,#32861,#32862,#32863,#32864,#32865,#32866,#32867,
#32868,#32869,#32870,#32871,#32872,#32873,#32874,#32875,#32876,#32877,#32878,
#32879,#32880,#32881,#32882,#32883,#32884,#32885,#32886,#32887,#32888,#32889),
 .UNSPECIFIED.,.F.,.F.,(4,3,3,3,3,3,3,3,3,3,3,3,3,3,3,3,3,3,3,3,3,3,3,3,
3,3,3,4),(0.,0.018597475715232,0.0384224454373358,0.0557692939441765,0.0644714217242545,
0.0684506017224621,0.0885047730237999,0.108914697191781,0.125985331266851,
0.133848209495266,0.137284586474664,0.158359468894701,0.177197233492062,
0.197725003512179,0.205649642568506,0.209125334915843,0.230131010156213,
0.251623262619965,0.268075192018812,0.278317579898386,0.28404464818755,
0.306313635980069,0.322966019399851,0.328172645794683,0.333184028513746,
0.355705443028296,0.372923169659198,0.376940817211644),.UNSPECIFIED.);
#2616=B_SPLINE_CURVE_WITH_KNOTS('',3,(#32890,#32891,#32892,#32893,#32894,
#32895,#32896,#32897,#32898,#32899,#32900,#32901,#32902,#32903,#32904,#32905,
#32906,#32907,#32908,#32909,#32910,#32911,#32912,#32913,#32914),
 .UNSPECIFIED.,.F.,.F.,(4,3,3,3,3,3,3,3,4),(-10.1295685708719,-9.975285344366,
-8.9777568099294,-7.9802282754928,-6.9826997410562,-5.9851712066196,-4.987642672183,
-3.9901141377464,-3.84638326369226),.UNSPECIFIED.);
#2617=B_SPLINE_CURVE_WITH_KNOTS('',3,(#33331,#33332,#33333,#33334,#33335,
#33336,#33337,#33338,#33339,#33340,#33341,#33342,#33343,#33344,#33345,#33346,
#33347,#33348,#33349,#33350,#33351,#33352),.UNSPECIFIED.,.F.,.F.,(4,3,3,
3,3,3,3,4),(7.59300756235149,7.9802282754928,8.97775680992939,9.975285344366,
10.9728138788026,11.9703424132392,12.9678709476758,13.8761928695311),
 .UNSPECIFIED.);
#2618=B_SPLINE_CURVE_WITH_KNOTS('',3,(#33353,#33354,#33355,#33356,#33357,
#33358,#33359,#33360,#33361,#33362,#33363,#33364,#33365,#33366,#33367,#33368,
#33369,#33370,#33371,#33372,#33373,#33374,#33375,#33376,#33377,#33378,#33379,
#33380,#33381,#33382,#33383,#33384,#33385,#33386,#33387,#33388,#33389,#33390,
#33391,#33392,#33393,#33394,#33395,#33396,#33397,#33398,#33399,#33400,#33401,
#33402,#33403,#33404,#33405,#33406,#33407,#33408,#33409,#33410,#33411,#33412,
#33413,#33414,#33415,#33416,#33417,#33418,#33419,#33420,#33421,#33422,#33423,
#33424,#33425,#33426,#33427,#33428,#33429,#33430,#33431,#33432,#33433,#33434,
#33435,#33436,#33437),.UNSPECIFIED.,.F.,.F.,(4,3,3,3,3,3,3,3,3,3,3,3,3,
3,3,3,3,3,3,3,3,3,3,3,3,3,3,3,4),(0.,0.021966136475729,0.0445436104424182,
0.0636200990930523,0.0720969484993908,0.076754421458333,0.0810485413537662,
0.102995141729322,0.124771436295877,0.142867457133781,0.150422750419918,
0.153917809521016,0.157566644049533,0.178337399455209,0.197155519647491,
0.219426672701638,0.224328239353299,0.229401233155315,0.250066318737277,
0.270727133433929,0.285676231370121,0.296892217575307,0.300623139776961,
0.320395489436602,0.334302180285225,0.338768589797073,0.357793661628995,
0.375324744080664,0.378621596831513),.UNSPECIFIED.);
#2619=B_SPLINE_CURVE_WITH_KNOTS('',3,(#33440,#33441,#33442,#33443,#33444,
#33445,#33446,#33447,#33448,#33449,#33450,#33451,#33452,#33453,#33454,#33455,
#33456,#33457,#33458,#33459,#33460,#33461,#33462,#33463,#33464,#33465,#33466,
#33467,#33468,#33469,#33470,#33471,#33472,#33473,#33474,#33475,#33476,#33477,
#33478,#33479,#33480,#33481,#33482,#33483,#33484,#33485,#33486,#33487,#33488,
#33489,#33490,#33491,#33492,#33493,#33494,#33495,#33496,#33497,#33498,#33499,
#33500,#33501,#33502,#33503,#33504,#33505,#33506,#33507,#33508,#33509,#33510,
#33511,#33512,#33513,#33514,#33515,#33516,#33517,#33518,#33519,#33520,#33521,
#33522,#33523,#33524,#33525,#33526,#33527),.UNSPECIFIED.,.F.,.F.,(4,3,3,
3,3,3,3,3,3,3,3,3,3,3,3,3,3,3,3,3,3,3,3,3,3,3,3,3,3,4),(-0.37862159683143,
-0.359797501318257,-0.347859596220205,-0.339721673305066,-0.335383849687154,
-0.315512157696412,-0.301177832053279,-0.297261100044044,-0.29322727751319,
-0.272825036004271,-0.252127377552038,-0.239304921301865,-0.228805647209281,
-0.224505165286516,-0.203200608394255,-0.200837552551346,-0.180350240469658,
-0.158310745311439,-0.154330248529997,-0.150809426102653,-0.129426144653503,
-0.107591969385708,-0.0856253476495468,-0.0802030812324167,-0.0759441620234358,
-0.0533965864690057,-0.0308244177267148,-0.00876577872099265,-0.00403427920390747,
0.),.UNSPECIFIED.);
#2620=B_SPLINE_CURVE_WITH_KNOTS('',3,(#33528,#33529,#33530,#33531,#33532,
#33533,#33534,#33535,#33536,#33537,#33538,#33539,#33540,#33541,#33542,#33543,
#33544,#33545,#33546,#33547,#33548,#33549,#33550,#33551,#33552,#33553,#33554,
#33555,#33556,#33557,#33558,#33559,#33560,#33561,#33562,#33563,#33564,#33565,
#33566,#33567,#33568,#33569,#33570,#33571,#33572,#33573,#33574,#33575,#33576,
#33577,#33578,#33579,#33580,#33581,#33582,#33583,#33584,#33585,#33586,#33587,
#33588,#33589,#33590,#33591,#33592,#33593,#33594,#33595,#33596,#33597,#33598,
#33599,#33600,#33601,#33602,#33603,#33604,#33605,#33606,#33607,#33608,#33609,
#33610,#33611,#33612),.UNSPECIFIED.,.F.,.F.,(4,3,3,3,3,3,3,3,3,3,3,3,3,
3,3,3,3,3,3,3,3,3,3,3,3,3,3,3,4),(-0.376940817211612,-0.354634290157469,
-0.332912862097815,-0.328064568788163,-0.305815969273377,-0.290196831324235,
-0.284261028697448,-0.278600437869163,-0.256917268853247,-0.235699710725379,
-0.214947489998165,-0.208197198698434,-0.204402058220254,-0.183825928780986,
-0.180862865680237,-0.159880209146386,-0.140305785776771,-0.136021313755173,
-0.132587901565395,-0.112128582775151,-0.0917639930231176,-0.0718357496511476,
-0.0676216646608822,-0.0636601411314518,-0.0441022574876565,-0.0249163309364235,
-0.00635337653324212,-0.00328482218946178,0.),.UNSPECIFIED.);
#2621=B_SPLINE_CURVE_WITH_KNOTS('',3,(#33614,#33615,#33616,#33617,#33618,
#33619,#33620,#33621,#33622,#33623,#33624),.UNSPECIFIED.,.F.,.F.,(4,1,1,
1,1,1,1,1,4),(15.7079632679489,15.851694142003,16.8492226764396,17.8467512108762,
18.8442797453128,19.8418082797494,20.839336814186,21.8368653486226,21.9911485751285),
 .UNSPECIFIED.);
#2622=B_SPLINE_CURVE_WITH_KNOTS('',3,(#33625,#33626,#33627,#33628,#33629,
#33630,#33631,#33632,#33633,#33634),.UNSPECIFIED.,.F.,.F.,(4,1,1,1,1,1,
1,4),(15.7079632679489,16.3931980816501,17.3907266160867,18.3882551505233,
19.3857836849599,20.3833122193965,21.3808407538331,21.9911485751285),
 .UNSPECIFIED.);
#2623=B_SPLINE_CURVE_WITH_KNOTS('',3,(#34051,#34052,#34053,#34054,#34055,
#34056,#34057,#34058,#34059,#34060,#34061,#34062,#34063,#34064,#34065,#34066,
#34067,#34068,#34069,#34070,#34071,#34072,#34073,#34074,#34075,#34076,#34077,
#34078,#34079,#34080,#34081,#34082,#34083,#34084,#34085,#34086,#34087,#34088,
#34089,#34090,#34091,#34092,#34093,#34094,#34095,#34096,#34097,#34098,#34099,
#34100,#34101,#34102,#34103,#34104,#34105,#34106,#34107,#34108,#34109,#34110,
#34111,#34112,#34113,#34114,#34115,#34116,#34117,#34118,#34119,#34120,#34121,
#34122,#34123,#34124,#34125,#34126,#34127,#34128,#34129,#34130,#34131,#34132),
 .UNSPECIFIED.,.F.,.F.,(4,3,3,3,3,3,3,3,3,3,3,3,3,3,3,3,3,3,3,3,3,3,3,3,
3,3,3,4),(0.,0.0185974817976789,0.038422450759474,0.0557692986010447,0.0644714297839629,
0.06845060381893,0.0885047794607919,0.108914705501413,0.12598533749907,
0.133848219307247,0.137284591577423,0.158359473431624,0.17719723349204,
0.197725000464005,0.205649640957615,0.209125333762854,0.230131005420896,
0.251623255998715,0.26807519355603,0.278317583444313,0.284044647320971,
0.306313634890073,0.322966018582345,0.328172643984831,0.333184027594933,
0.355705442137259,0.37292316965916,0.376940817211606),.UNSPECIFIED.);
#2624=B_SPLINE_CURVE_WITH_KNOTS('',3,(#34133,#34134,#34135,#34136,#34137,
#34138,#34139,#34140,#34141,#34142,#34143,#34144,#34145,#34146,#34147,#34148,
#34149,#34150,#34151,#34152,#34153,#34154,#34155,#34156,#34157),
 .UNSPECIFIED.,.F.,.F.,(4,3,3,3,3,3,3,3,4),(-10.1295685708719,-9.975285344366,
-8.9777568099294,-7.9802282754928,-6.9826997410562,-5.9851712066196,-4.98764267218299,
-3.9901141377464,-3.8463832636923),.UNSPECIFIED.);
#2625=B_SPLINE_CURVE_WITH_KNOTS('',3,(#34574,#34575,#34576,#34577,#34578,
#34579,#34580,#34581,#34582,#34583,#34584,#34585,#34586,#34587,#34588,#34589,
#34590,#34591,#34592,#34593,#34594,#34595),.UNSPECIFIED.,.F.,.F.,(4,3,3,
3,3,3,3,4),(7.59300756235153,7.98022827549279,8.97775680992939,9.97528534436599,
10.9728138788026,11.9703424132392,12.9678709476758,13.8761928695311),
 .UNSPECIFIED.);
#2626=B_SPLINE_CURVE_WITH_KNOTS('',3,(#34596,#34597,#34598,#34599,#34600,
#34601,#34602,#34603,#34604,#34605,#34606,#34607,#34608,#34609,#34610,#34611,
#34612,#34613,#34614,#34615,#34616,#34617,#34618,#34619,#34620,#34621,#34622,
#34623,#34624,#34625,#34626,#34627,#34628,#34629,#34630,#34631,#34632,#34633,
#34634,#34635,#34636,#34637,#34638,#34639,#34640,#34641,#34642,#34643,#34644,
#34645,#34646,#34647,#34648,#34649,#34650,#34651,#34652,#34653,#34654,#34655,
#34656,#34657,#34658,#34659,#34660,#34661,#34662,#34663,#34664,#34665,#34666,
#34667,#34668,#34669,#34670,#34671,#34672,#34673,#34674,#34675,#34676,#34677,
#34678,#34679,#34680),.UNSPECIFIED.,.F.,.F.,(4,3,3,3,3,3,3,3,3,3,3,3,3,
3,3,3,3,3,3,3,3,3,3,3,3,3,3,3,4),(0.,0.0219661192670637,0.0445435915688456,
0.063620082578671,0.0720969435699582,0.0767544110241794,0.0810485385530744,
0.102995139263397,0.124771439019085,0.142867459176176,0.150422749506048,
0.153917803983106,0.157566642311518,0.178337402886831,0.197155519647449,
0.219426672701589,0.224328240715824,0.229401233202951,0.250066318102677,
0.270727133401917,0.28567624690996,0.296892244536993,0.300623147437404,
0.32039550320955,0.33430220310881,0.33876861083147,0.357793692369518,0.375324744080569,
0.378621596831417),.UNSPECIFIED.);
#2799=LINE('',#13453,#3337);
#2800=LINE('',#13482,#3338);
#2801=LINE('',#13509,#3339);
#2802=LINE('',#13560,#3340);
#2803=LINE('',#13608,#3341);
#2804=LINE('',#13659,#3342);
#2805=LINE('',#13710,#3343);
#2806=LINE('',#13758,#3344);
#2807=LINE('',#13806,#3345);
#2808=LINE('',#13857,#3346);
#2809=LINE('',#13905,#3347);
#2810=LINE('',#13953,#3348);
#2811=LINE('',#14004,#3349);
#2812=LINE('',#14055,#3350);
#2813=LINE('',#14103,#3351);
#2814=LINE('',#14154,#3352);
#2815=LINE('',#14193,#3353);
#2816=LINE('',#14213,#3354);
#2817=LINE('',#14237,#3355);
#2818=LINE('',#14262,#3356);
#2819=LINE('',#14287,#3357);
#2820=LINE('',#14311,#3358);
#2821=LINE('',#14336,#3359);
#2822=LINE('',#14360,#3360);
#2823=LINE('',#14385,#3361);
#2824=LINE('',#14410,#3362);
#2825=LINE('',#14434,#3363);
#2826=LINE('',#14459,#3364);
#2827=LINE('',#14483,#3365);
#2828=LINE('',#14508,#3366);
#2829=LINE('',#14533,#3367);
#2830=LINE('',#14557,#3368);
#2831=LINE('',#14574,#3369);
#2832=LINE('',#14603,#3370);
#2833=LINE('',#14630,#3371);
#2834=LINE('',#14681,#3372);
#2835=LINE('',#14729,#3373);
#2836=LINE('',#14780,#3374);
#2837=LINE('',#14831,#3375);
#2838=LINE('',#14879,#3376);
#2839=LINE('',#14927,#3377);
#2840=LINE('',#14978,#3378);
#2841=LINE('',#15026,#3379);
#2842=LINE('',#15074,#3380);
#2843=LINE('',#15125,#3381);
#2844=LINE('',#15176,#3382);
#2845=LINE('',#15224,#3383);
#2846=LINE('',#15275,#3384);
#2847=LINE('',#15314,#3385);
#2848=LINE('',#15334,#3386);
#2849=LINE('',#15358,#3387);
#2850=LINE('',#15383,#3388);
#2851=LINE('',#15408,#3389);
#2852=LINE('',#15432,#3390);
#2853=LINE('',#15457,#3391);
#2854=LINE('',#15481,#3392);
#2855=LINE('',#15506,#3393);
#2856=LINE('',#15531,#3394);
#2857=LINE('',#15555,#3395);
#2858=LINE('',#15580,#3396);
#2859=LINE('',#15604,#3397);
#2860=LINE('',#15629,#3398);
#2861=LINE('',#15654,#3399);
#2862=LINE('',#15678,#3400);
#2863=LINE('',#15695,#3401);
#2864=LINE('',#15724,#3402);
#2865=LINE('',#15751,#3403);
#2866=LINE('',#15802,#3404);
#2867=LINE('',#15850,#3405);
#2868=LINE('',#15901,#3406);
#2869=LINE('',#15952,#3407);
#2870=LINE('',#16000,#3408);
#2871=LINE('',#16048,#3409);
#2872=LINE('',#16099,#3410);
#2873=LINE('',#16147,#3411);
#2874=LINE('',#16195,#3412);
#2875=LINE('',#16246,#3413);
#2876=LINE('',#16297,#3414);
#2877=LINE('',#16345,#3415);
#2878=LINE('',#16396,#3416);
#2879=LINE('',#16435,#3417);
#2880=LINE('',#16455,#3418);
#2881=LINE('',#16479,#3419);
#2882=LINE('',#16504,#3420);
#2883=LINE('',#16529,#3421);
#2884=LINE('',#16553,#3422);
#2885=LINE('',#16578,#3423);
#2886=LINE('',#16602,#3424);
#2887=LINE('',#16627,#3425);
#2888=LINE('',#16652,#3426);
#2889=LINE('',#16676,#3427);
#2890=LINE('',#16701,#3428);
#2891=LINE('',#16725,#3429);
#2892=LINE('',#16750,#3430);
#2893=LINE('',#16775,#3431);
#2894=LINE('',#16799,#3432);
#2895=LINE('',#16816,#3433);
#2896=LINE('',#16845,#3434);
#2897=LINE('',#16872,#3435);
#2898=LINE('',#16923,#3436);
#2899=LINE('',#16971,#3437);
#2900=LINE('',#17022,#3438);
#2901=LINE('',#17073,#3439);
#2902=LINE('',#17121,#3440);
#2903=LINE('',#17169,#3441);
#2904=LINE('',#17220,#3442);
#2905=LINE('',#17268,#3443);
#2906=LINE('',#17316,#3444);
#2907=LINE('',#17367,#3445);
#2908=LINE('',#17418,#3446);
#2909=LINE('',#17466,#3447);
#2910=LINE('',#17517,#3448);
#2911=LINE('',#17556,#3449);
#2912=LINE('',#17576,#3450);
#2913=LINE('',#17600,#3451);
#2914=LINE('',#17625,#3452);
#2915=LINE('',#17650,#3453);
#2916=LINE('',#17674,#3454);
#2917=LINE('',#17699,#3455);
#2918=LINE('',#17723,#3456);
#2919=LINE('',#17748,#3457);
#2920=LINE('',#17773,#3458);
#2921=LINE('',#17797,#3459);
#2922=LINE('',#17822,#3460);
#2923=LINE('',#17846,#3461);
#2924=LINE('',#17871,#3462);
#2925=LINE('',#17896,#3463);
#2926=LINE('',#17920,#3464);
#2927=LINE('',#17937,#3465);
#2928=LINE('',#17980,#3466);
#2929=LINE('',#18031,#3467);
#2930=LINE('',#18082,#3468);
#2931=LINE('',#18130,#3469);
#2932=LINE('',#18181,#3470);
#2933=LINE('',#18232,#3471);
#2934=LINE('',#18280,#3472);
#2935=LINE('',#18331,#3473);
#2936=LINE('',#18382,#3474);
#2937=LINE('',#18430,#3475);
#2938=LINE('',#18481,#3476);
#2939=LINE('',#18532,#3477);
#2940=LINE('',#18580,#3478);
#2941=LINE('',#18631,#3479);
#2942=LINE('',#18670,#3480);
#2943=LINE('',#18713,#3481);
#2944=LINE('',#18764,#3482);
#2945=LINE('',#18815,#3483);
#2946=LINE('',#18863,#3484);
#2947=LINE('',#18914,#3485);
#2948=LINE('',#18965,#3486);
#2949=LINE('',#19013,#3487);
#2950=LINE('',#19064,#3488);
#2951=LINE('',#19115,#3489);
#2952=LINE('',#19163,#3490);
#2953=LINE('',#19214,#3491);
#2954=LINE('',#19265,#3492);
#2955=LINE('',#19313,#3493);
#2956=LINE('',#19364,#3494);
#2957=LINE('',#19403,#3495);
#2958=LINE('',#19427,#3496);
#2959=LINE('',#19451,#3497);
#2960=LINE('',#19476,#3498);
#2961=LINE('',#19501,#3499);
#2962=LINE('',#19525,#3500);
#2963=LINE('',#19550,#3501);
#2964=LINE('',#19575,#3502);
#2965=LINE('',#19599,#3503);
#2966=LINE('',#19624,#3504);
#2967=LINE('',#19649,#3505);
#2968=LINE('',#19673,#3506);
#2969=LINE('',#19698,#3507);
#2970=LINE('',#19723,#3508);
#2971=LINE('',#19747,#3509);
#2972=LINE('',#19764,#3510);
#2973=LINE('',#19788,#3511);
#2974=LINE('',#19812,#3512);
#2975=LINE('',#19837,#3513);
#2976=LINE('',#19862,#3514);
#2977=LINE('',#19886,#3515);
#2978=LINE('',#19911,#3516);
#2979=LINE('',#19936,#3517);
#2980=LINE('',#19960,#3518);
#2981=LINE('',#19985,#3519);
#2982=LINE('',#20010,#3520);
#2983=LINE('',#20034,#3521);
#2984=LINE('',#20059,#3522);
#2985=LINE('',#20084,#3523);
#2986=LINE('',#20108,#3524);
#2987=LINE('',#20125,#3525);
#2988=LINE('',#20134,#3526);
#2989=LINE('',#20151,#3527);
#2990=LINE('',#20202,#3528);
#2991=LINE('',#20253,#3529);
#2992=LINE('',#20301,#3530);
#2993=LINE('',#20352,#3531);
#2994=LINE('',#20403,#3532);
#2995=LINE('',#20451,#3533);
#2996=LINE('',#20502,#3534);
#2997=LINE('',#20553,#3535);
#2998=LINE('',#20601,#3536);
#2999=LINE('',#20652,#3537);
#3000=LINE('',#20703,#3538);
#3001=LINE('',#20751,#3539);
#3002=LINE('',#20802,#3540);
#3003=LINE('',#20841,#3541);
#3004=LINE('',#20865,#3542);
#3005=LINE('',#20889,#3543);
#3006=LINE('',#20914,#3544);
#3007=LINE('',#20939,#3545);
#3008=LINE('',#20963,#3546);
#3009=LINE('',#20988,#3547);
#3010=LINE('',#21013,#3548);
#3011=LINE('',#21037,#3549);
#3012=LINE('',#21062,#3550);
#3013=LINE('',#21087,#3551);
#3014=LINE('',#21111,#3552);
#3015=LINE('',#21136,#3553);
#3016=LINE('',#21161,#3554);
#3017=LINE('',#21185,#3555);
#3018=LINE('',#21202,#3556);
#3019=LINE('',#21211,#3557);
#3020=LINE('',#21228,#3558);
#3021=LINE('',#21279,#3559);
#3022=LINE('',#21330,#3560);
#3023=LINE('',#21378,#3561);
#3024=LINE('',#21429,#3562);
#3025=LINE('',#21480,#3563);
#3026=LINE('',#21528,#3564);
#3027=LINE('',#21579,#3565);
#3028=LINE('',#21630,#3566);
#3029=LINE('',#21678,#3567);
#3030=LINE('',#21729,#3568);
#3031=LINE('',#21780,#3569);
#3032=LINE('',#21828,#3570);
#3033=LINE('',#21879,#3571);
#3034=LINE('',#21918,#3572);
#3035=LINE('',#21942,#3573);
#3036=LINE('',#21966,#3574);
#3037=LINE('',#21991,#3575);
#3038=LINE('',#22016,#3576);
#3039=LINE('',#22040,#3577);
#3040=LINE('',#22065,#3578);
#3041=LINE('',#22090,#3579);
#3042=LINE('',#22114,#3580);
#3043=LINE('',#22139,#3581);
#3044=LINE('',#22164,#3582);
#3045=LINE('',#22188,#3583);
#3046=LINE('',#22213,#3584);
#3047=LINE('',#22238,#3585);
#3048=LINE('',#22262,#3586);
#3049=LINE('',#22279,#3587);
#3050=LINE('',#22348,#3588);
#3051=LINE('',#22438,#3589);
#3052=LINE('',#22525,#3590);
#3053=LINE('',#22615,#3591);
#3054=LINE('',#22702,#3592);
#3055=LINE('',#22792,#3593);
#3056=LINE('',#22879,#3594);
#3057=LINE('',#22912,#3595);
#3058=LINE('',#22946,#3596);
#3059=LINE('',#22982,#3597);
#3060=LINE('',#23020,#3598);
#3061=LINE('',#23058,#3599);
#3062=LINE('',#23095,#3600);
#3063=LINE('',#23132,#3601);
#3064=LINE('',#23170,#3602);
#3065=LINE('',#24650,#3603);
#3066=LINE('',#24654,#3604);
#3067=LINE('',#24656,#3605);
#3068=LINE('',#24658,#3606);
#3069=LINE('',#24659,#3607);
#3070=LINE('',#27520,#3608);
#3071=LINE('',#27554,#3609);
#3072=LINE('',#27683,#3610);
#3073=LINE('',#27686,#3611);
#3074=LINE('',#28614,#3612);
#3075=LINE('',#28648,#3613);
#3076=LINE('',#28777,#3614);
#3077=LINE('',#28780,#3615);
#3078=LINE('',#34690,#3616);
#3079=LINE('',#34696,#3617);
#3080=LINE('',#34702,#3618);
#3081=LINE('',#34708,#3619);
#3082=LINE('',#34714,#3620);
#3083=LINE('',#34720,#3621);
#3084=LINE('',#34726,#3622);
#3085=LINE('',#34732,#3623);
#3086=LINE('',#34737,#3624);
#3087=LINE('',#34739,#3625);
#3088=LINE('',#34745,#3626);
#3089=LINE('',#34751,#3627);
#3090=LINE('',#34757,#3628);
#3091=LINE('',#34763,#3629);
#3092=LINE('',#34769,#3630);
#3093=LINE('',#34775,#3631);
#3094=LINE('',#34781,#3632);
#3095=LINE('',#34786,#3633);
#3096=LINE('',#34788,#3634);
#3097=LINE('',#34794,#3635);
#3098=LINE('',#34799,#3636);
#3099=LINE('',#34801,#3637);
#3100=LINE('',#34803,#3638);
#3101=LINE('',#34804,#3639);
#3102=LINE('',#34807,#3640);
#3103=LINE('',#34809,#3641);
#3104=LINE('',#34810,#3642);
#3105=LINE('',#34813,#3643);
#3106=LINE('',#34815,#3644);
#3107=LINE('',#34816,#3645);
#3108=LINE('',#34818,#3646);
#3109=LINE('',#34819,#3647);
#3110=LINE('',#34823,#3648);
#3111=LINE('',#34825,#3649);
#3112=LINE('',#34826,#3650);
#3113=LINE('',#34829,#3651);
#3114=LINE('',#34830,#3652);
#3115=LINE('',#34833,#3653);
#3116=LINE('',#34834,#3654);
#3117=LINE('',#34836,#3655);
#3337=VECTOR('',#11312,2.);
#3338=VECTOR('',#11315,2.);
#3339=VECTOR('',#11320,2.);
#3340=VECTOR('',#11323,2.);
#3341=VECTOR('',#11326,2.);
#3342=VECTOR('',#11329,2.);
#3343=VECTOR('',#11332,2.);
#3344=VECTOR('',#11335,2.);
#3345=VECTOR('',#11338,2.);
#3346=VECTOR('',#11341,2.);
#3347=VECTOR('',#11344,2.);
#3348=VECTOR('',#11347,2.);
#3349=VECTOR('',#11350,2.);
#3350=VECTOR('',#11353,2.);
#3351=VECTOR('',#11356,2.);
#3352=VECTOR('',#11359,2.);
#3353=VECTOR('',#11364,2.05475000000001);
#3354=VECTOR('',#11369,2.05475000000001);
#3355=VECTOR('',#11372,2.05475000000001);
#3356=VECTOR('',#11375,2.05475000000001);
#3357=VECTOR('',#11378,2.05475000000001);
#3358=VECTOR('',#11381,2.05475000000001);
#3359=VECTOR('',#11384,2.05475000000001);
#3360=VECTOR('',#11387,2.05475000000001);
#3361=VECTOR('',#11390,2.05475000000001);
#3362=VECTOR('',#11393,2.05475000000001);
#3363=VECTOR('',#11396,2.05475000000001);
#3364=VECTOR('',#11399,2.05475000000001);
#3365=VECTOR('',#11402,2.05475000000001);
#3366=VECTOR('',#11405,2.05475000000001);
#3367=VECTOR('',#11408,2.05475000000001);
#3368=VECTOR('',#11411,2.05475000000001);
#3369=VECTOR('',#11416,2.);
#3370=VECTOR('',#11419,2.);
#3371=VECTOR('',#11424,2.);
#3372=VECTOR('',#11427,2.);
#3373=VECTOR('',#11430,2.);
#3374=VECTOR('',#11433,2.);
#3375=VECTOR('',#11436,2.);
#3376=VECTOR('',#11439,2.);
#3377=VECTOR('',#11442,2.);
#3378=VECTOR('',#11445,2.);
#3379=VECTOR('',#11448,2.);
#3380=VECTOR('',#11451,2.);
#3381=VECTOR('',#11454,2.);
#3382=VECTOR('',#11457,2.);
#3383=VECTOR('',#11460,2.);
#3384=VECTOR('',#11463,2.);
#3385=VECTOR('',#11468,2.05475);
#3386=VECTOR('',#11473,2.05475);
#3387=VECTOR('',#11476,2.05475);
#3388=VECTOR('',#11479,2.05475);
#3389=VECTOR('',#11482,2.05475);
#3390=VECTOR('',#11485,2.05475);
#3391=VECTOR('',#11488,2.05475);
#3392=VECTOR('',#11491,2.05475);
#3393=VECTOR('',#11494,2.05475);
#3394=VECTOR('',#11497,2.05475);
#3395=VECTOR('',#11500,2.05475);
#3396=VECTOR('',#11503,2.05475);
#3397=VECTOR('',#11506,2.05475);
#3398=VECTOR('',#11509,2.05475);
#3399=VECTOR('',#11512,2.05475);
#3400=VECTOR('',#11515,2.05475);
#3401=VECTOR('',#11520,2.);
#3402=VECTOR('',#11523,2.);
#3403=VECTOR('',#11528,2.);
#3404=VECTOR('',#11531,2.);
#3405=VECTOR('',#11534,2.);
#3406=VECTOR('',#11537,2.);
#3407=VECTOR('',#11540,2.);
#3408=VECTOR('',#11543,2.);
#3409=VECTOR('',#11546,2.);
#3410=VECTOR('',#11549,2.);
#3411=VECTOR('',#11552,2.);
#3412=VECTOR('',#11555,2.);
#3413=VECTOR('',#11558,2.);
#3414=VECTOR('',#11561,2.);
#3415=VECTOR('',#11564,2.);
#3416=VECTOR('',#11567,2.);
#3417=VECTOR('',#11572,2.05475000000001);
#3418=VECTOR('',#11577,2.05475000000001);
#3419=VECTOR('',#11580,2.05475000000001);
#3420=VECTOR('',#11583,2.05475000000001);
#3421=VECTOR('',#11586,2.05475000000001);
#3422=VECTOR('',#11589,2.05475000000001);
#3423=VECTOR('',#11592,2.05475000000001);
#3424=VECTOR('',#11595,2.05475000000001);
#3425=VECTOR('',#11598,2.05475000000001);
#3426=VECTOR('',#11601,2.05475000000001);
#3427=VECTOR('',#11604,2.05475000000001);
#3428=VECTOR('',#11607,2.05475000000001);
#3429=VECTOR('',#11610,2.05475000000001);
#3430=VECTOR('',#11613,2.05475000000001);
#3431=VECTOR('',#11616,2.05475000000001);
#3432=VECTOR('',#11619,2.05475000000001);
#3433=VECTOR('',#11624,2.);
#3434=VECTOR('',#11627,2.);
#3435=VECTOR('',#11632,2.);
#3436=VECTOR('',#11635,2.);
#3437=VECTOR('',#11638,2.);
#3438=VECTOR('',#11641,2.);
#3439=VECTOR('',#11644,2.);
#3440=VECTOR('',#11647,2.);
#3441=VECTOR('',#11650,2.);
#3442=VECTOR('',#11653,2.);
#3443=VECTOR('',#11656,2.);
#3444=VECTOR('',#11659,2.);
#3445=VECTOR('',#11662,2.);
#3446=VECTOR('',#11665,2.);
#3447=VECTOR('',#11668,2.);
#3448=VECTOR('',#11671,2.);
#3449=VECTOR('',#11676,2.05475);
#3450=VECTOR('',#11681,2.05475);
#3451=VECTOR('',#11684,2.05475);
#3452=VECTOR('',#11687,2.05475);
#3453=VECTOR('',#11690,2.05475);
#3454=VECTOR('',#11693,2.05475);
#3455=VECTOR('',#11696,2.05475);
#3456=VECTOR('',#11699,2.05475);
#3457=VECTOR('',#11702,2.05475);
#3458=VECTOR('',#11705,2.05475);
#3459=VECTOR('',#11708,2.05475);
#3460=VECTOR('',#11711,2.05475);
#3461=VECTOR('',#11714,2.05475);
#3462=VECTOR('',#11717,2.05475);
#3463=VECTOR('',#11720,2.05475);
#3464=VECTOR('',#11723,2.05475);
#3465=VECTOR('',#11728,3.);
#3466=VECTOR('',#11735,3.);
#3467=VECTOR('',#11738,3.);
#3468=VECTOR('',#11741,3.);
#3469=VECTOR('',#11744,3.);
#3470=VECTOR('',#11747,3.);
#3471=VECTOR('',#11750,3.);
#3472=VECTOR('',#11753,3.);
#3473=VECTOR('',#11756,3.);
#3474=VECTOR('',#11759,3.);
#3475=VECTOR('',#11762,3.);
#3476=VECTOR('',#11765,3.);
#3477=VECTOR('',#11768,3.);
#3478=VECTOR('',#11771,3.);
#3479=VECTOR('',#11774,3.);
#3480=VECTOR('',#11779,3.);
#3481=VECTOR('',#11786,3.);
#3482=VECTOR('',#11789,3.);
#3483=VECTOR('',#11792,3.);
#3484=VECTOR('',#11795,3.);
#3485=VECTOR('',#11798,3.);
#3486=VECTOR('',#11801,3.);
#3487=VECTOR('',#11804,3.);
#3488=VECTOR('',#11807,3.);
#3489=VECTOR('',#11810,3.);
#3490=VECTOR('',#11813,3.);
#3491=VECTOR('',#11816,3.);
#3492=VECTOR('',#11819,3.);
#3493=VECTOR('',#11822,3.);
#3494=VECTOR('',#11825,3.);
#3495=VECTOR('',#11830,3.0735);
#3496=VECTOR('',#11835,3.0735);
#3497=VECTOR('',#11838,3.0735);
#3498=VECTOR('',#11841,3.0735);
#3499=VECTOR('',#11844,3.0735);
#3500=VECTOR('',#11847,3.0735);
#3501=VECTOR('',#11850,3.0735);
#3502=VECTOR('',#11853,3.0735);
#3503=VECTOR('',#11856,3.0735);
#3504=VECTOR('',#11859,3.0735);
#3505=VECTOR('',#11862,3.0735);
#3506=VECTOR('',#11865,3.0735);
#3507=VECTOR('',#11868,3.0735);
#3508=VECTOR('',#11871,3.0735);
#3509=VECTOR('',#11874,3.0735);
#3510=VECTOR('',#11879,3.0735);
#3511=VECTOR('',#11884,3.0735);
#3512=VECTOR('',#11887,3.0735);
#3513=VECTOR('',#11890,3.0735);
#3514=VECTOR('',#11893,3.0735);
#3515=VECTOR('',#11896,3.0735);
#3516=VECTOR('',#11899,3.0735);
#3517=VECTOR('',#11902,3.0735);
#3518=VECTOR('',#11905,3.0735);
#3519=VECTOR('',#11908,3.0735);
#3520=VECTOR('',#11911,3.0735);
#3521=VECTOR('',#11914,3.0735);
#3522=VECTOR('',#11917,3.0735);
#3523=VECTOR('',#11920,3.0735);
#3524=VECTOR('',#11923,3.0735);
#3525=VECTOR('',#11928,3.);
#3526=VECTOR('',#11931,3.);
#3527=VECTOR('',#11938,3.);
#3528=VECTOR('',#11941,3.);
#3529=VECTOR('',#11944,3.);
#3530=VECTOR('',#11947,3.);
#3531=VECTOR('',#11950,3.);
#3532=VECTOR('',#11953,3.);
#3533=VECTOR('',#11956,3.);
#3534=VECTOR('',#11959,3.);
#3535=VECTOR('',#11962,3.);
#3536=VECTOR('',#11965,3.);
#3537=VECTOR('',#11968,3.);
#3538=VECTOR('',#11971,3.);
#3539=VECTOR('',#11974,3.);
#3540=VECTOR('',#11977,3.);
#3541=VECTOR('',#11982,3.0735);
#3542=VECTOR('',#11987,3.0735);
#3543=VECTOR('',#11990,3.0735);
#3544=VECTOR('',#11993,3.0735);
#3545=VECTOR('',#11996,3.0735);
#3546=VECTOR('',#11999,3.0735);
#3547=VECTOR('',#12002,3.0735);
#3548=VECTOR('',#12005,3.0735);
#3549=VECTOR('',#12008,3.0735);
#3550=VECTOR('',#12011,3.0735);
#3551=VECTOR('',#12014,3.0735);
#3552=VECTOR('',#12017,3.0735);
#3553=VECTOR('',#12020,3.0735);
#3554=VECTOR('',#12023,3.0735);
#3555=VECTOR('',#12026,3.0735);
#3556=VECTOR('',#12031,3.);
#3557=VECTOR('',#12034,3.);
#3558=VECTOR('',#12041,3.);
#3559=VECTOR('',#12044,3.);
#3560=VECTOR('',#12047,3.);
#3561=VECTOR('',#12050,3.);
#3562=VECTOR('',#12053,3.);
#3563=VECTOR('',#12056,3.);
#3564=VECTOR('',#12059,3.);
#3565=VECTOR('',#12062,3.);
#3566=VECTOR('',#12065,3.);
#3567=VECTOR('',#12068,3.);
#3568=VECTOR('',#12071,3.);
#3569=VECTOR('',#12074,3.);
#3570=VECTOR('',#12077,3.);
#3571=VECTOR('',#12080,3.);
#3572=VECTOR('',#12085,3.0735);
#3573=VECTOR('',#12090,3.0735);
#3574=VECTOR('',#12093,3.0735);
#3575=VECTOR('',#12096,3.0735);
#3576=VECTOR('',#12099,3.0735);
#3577=VECTOR('',#12102,3.0735);
#3578=VECTOR('',#12105,3.0735);
#3579=VECTOR('',#12108,3.0735);
#3580=VECTOR('',#12111,3.0735);
#3581=VECTOR('',#12114,3.0735);
#3582=VECTOR('',#12117,3.0735);
#3583=VECTOR('',#12120,3.0735);
#3584=VECTOR('',#12123,3.0735);
#3585=VECTOR('',#12126,3.0735);
#3586=VECTOR('',#12129,3.0735);
#3587=VECTOR('',#12134,8.);
#3588=VECTOR('',#12139,8.);
#3589=VECTOR('',#12142,8.);
#3590=VECTOR('',#12145,8.);
#3591=VECTOR('',#12148,8.);
#3592=VECTOR('',#12151,8.);
#3593=VECTOR('',#12154,8.);
#3594=VECTOR('',#12157,8.);
#3595=VECTOR('',#12162,8.1015);
#3596=VECTOR('',#12167,8.1015);
#3597=VECTOR('',#12170,8.1015);
#3598=VECTOR('',#12173,8.1015);
#3599=VECTOR('',#12176,8.1015);
#3600=VECTOR('',#12179,8.1015);
#3601=VECTOR('',#12182,8.1015);
#3602=VECTOR('',#12185,8.1015);
#3603=VECTOR('',#12200,12.);
#3604=VECTOR('',#12203,10.);
#3605=VECTOR('',#12204,10.);
#3606=VECTOR('',#12205,10.);
#3607=VECTOR('',#12206,10.);
#3608=VECTOR('',#12221,10.);
#3609=VECTOR('',#12224,10.);
#3610=VECTOR('',#12225,10.);
#3611=VECTOR('',#12230,10.);
#3612=VECTOR('',#12237,10.);
#3613=VECTOR('',#12240,10.);
#3614=VECTOR('',#12241,10.);
#3615=VECTOR('',#12246,10.);
#3616=VECTOR('',#12295,5.);
#3617=VECTOR('',#12302,5.);
#3618=VECTOR('',#12309,5.);
#3619=VECTOR('',#12316,5.);
#3620=VECTOR('',#12323,5.);
#3621=VECTOR('',#12330,5.);
#3622=VECTOR('',#12337,5.);
#3623=VECTOR('',#12344,5.);
#3624=VECTOR('',#12351,5.);
#3625=VECTOR('',#12352,5.);
#3626=VECTOR('',#12359,5.);
#3627=VECTOR('',#12366,5.);
#3628=VECTOR('',#12373,5.);
#3629=VECTOR('',#12380,5.);
#3630=VECTOR('',#12387,5.);
#3631=VECTOR('',#12394,5.);
#3632=VECTOR('',#12401,5.);
#3633=VECTOR('',#12408,5.);
#3634=VECTOR('',#12409,5.);
#3635=VECTOR('',#12416,5.);
#3636=VECTOR('',#12421,10.);
#3637=VECTOR('',#12422,10.);
#3638=VECTOR('',#12423,10.);
#3639=VECTOR('',#12424,10.);
#3640=VECTOR('',#12427,10.);
#3641=VECTOR('',#12428,10.);
#3642=VECTOR('',#12429,10.);
#3643=VECTOR('',#12432,10.);
#3644=VECTOR('',#12433,10.);
#3645=VECTOR('',#12434,10.);
#3646=VECTOR('',#12437,10.);
#3647=VECTOR('',#12438,10.);
#3648=VECTOR('',#12443,10.);
#3649=VECTOR('',#12444,10.);
#3650=VECTOR('',#12445,10.);
#3651=VECTOR('',#12448,10.);
#3652=VECTOR('',#12449,10.);
#3653=VECTOR('',#12452,10.);
#3654=VECTOR('',#12453,10.);
#3655=VECTOR('',#12456,10.);
#3875=VERTEX_POINT('',#13451);
#3876=VERTEX_POINT('',#13452);
#3877=VERTEX_POINT('',#13454);
#3878=VERTEX_POINT('',#13474);
#3879=VERTEX_POINT('',#13476);
#3880=VERTEX_POINT('',#13481);
#3881=VERTEX_POINT('',#13507);
#3882=VERTEX_POINT('',#13508);
#3883=VERTEX_POINT('',#13558);
#3884=VERTEX_POINT('',#13559);
#3885=VERTEX_POINT('',#13606);
#3886=VERTEX_POINT('',#13607);
#3887=VERTEX_POINT('',#13657);
#3888=VERTEX_POINT('',#13658);
#3889=VERTEX_POINT('',#13708);
#3890=VERTEX_POINT('',#13709);
#3891=VERTEX_POINT('',#13756);
#3892=VERTEX_POINT('',#13757);
#3893=VERTEX_POINT('',#13804);
#3894=VERTEX_POINT('',#13805);
#3895=VERTEX_POINT('',#13855);
#3896=VERTEX_POINT('',#13856);
#3897=VERTEX_POINT('',#13903);
#3898=VERTEX_POINT('',#13904);
#3899=VERTEX_POINT('',#13951);
#3900=VERTEX_POINT('',#13952);
#3901=VERTEX_POINT('',#14002);
#3902=VERTEX_POINT('',#14003);
#3903=VERTEX_POINT('',#14053);
#3904=VERTEX_POINT('',#14054);
#3905=VERTEX_POINT('',#14101);
#3906=VERTEX_POINT('',#14102);
#3907=VERTEX_POINT('',#14152);
#3908=VERTEX_POINT('',#14153);
#3909=VERTEX_POINT('',#14155);
#3910=VERTEX_POINT('',#14169);
#3911=VERTEX_POINT('',#14191);
#3912=VERTEX_POINT('',#14192);
#3913=VERTEX_POINT('',#14194);
#3914=VERTEX_POINT('',#14201);
#3915=VERTEX_POINT('',#14211);
#3916=VERTEX_POINT('',#14212);
#3917=VERTEX_POINT('',#14235);
#3918=VERTEX_POINT('',#14236);
#3919=VERTEX_POINT('',#14260);
#3920=VERTEX_POINT('',#14261);
#3921=VERTEX_POINT('',#14285);
#3922=VERTEX_POINT('',#14286);
#3923=VERTEX_POINT('',#14309);
#3924=VERTEX_POINT('',#14310);
#3925=VERTEX_POINT('',#14334);
#3926=VERTEX_POINT('',#14335);
#3927=VERTEX_POINT('',#14358);
#3928=VERTEX_POINT('',#14359);
#3929=VERTEX_POINT('',#14383);
#3930=VERTEX_POINT('',#14384);
#3931=VERTEX_POINT('',#14408);
#3932=VERTEX_POINT('',#14409);
#3933=VERTEX_POINT('',#14432);
#3934=VERTEX_POINT('',#14433);
#3935=VERTEX_POINT('',#14457);
#3936=VERTEX_POINT('',#14458);
#3937=VERTEX_POINT('',#14481);
#3938=VERTEX_POINT('',#14482);
#3939=VERTEX_POINT('',#14506);
#3940=VERTEX_POINT('',#14507);
#3941=VERTEX_POINT('',#14531);
#3942=VERTEX_POINT('',#14532);
#3943=VERTEX_POINT('',#14555);
#3944=VERTEX_POINT('',#14556);
#3945=VERTEX_POINT('',#14558);
#3946=VERTEX_POINT('',#14564);
#3947=VERTEX_POINT('',#14572);
#3948=VERTEX_POINT('',#14573);
#3949=VERTEX_POINT('',#14575);
#3950=VERTEX_POINT('',#14595);
#3951=VERTEX_POINT('',#14597);
#3952=VERTEX_POINT('',#14602);
#3953=VERTEX_POINT('',#14628);
#3954=VERTEX_POINT('',#14629);
#3955=VERTEX_POINT('',#14679);
#3956=VERTEX_POINT('',#14680);
#3957=VERTEX_POINT('',#14727);
#3958=VERTEX_POINT('',#14728);
#3959=VERTEX_POINT('',#14778);
#3960=VERTEX_POINT('',#14779);
#3961=VERTEX_POINT('',#14829);
#3962=VERTEX_POINT('',#14830);
#3963=VERTEX_POINT('',#14877);
#3964=VERTEX_POINT('',#14878);
#3965=VERTEX_POINT('',#14925);
#3966=VERTEX_POINT('',#14926);
#3967=VERTEX_POINT('',#14976);
#3968=VERTEX_POINT('',#14977);
#3969=VERTEX_POINT('',#15024);
#3970=VERTEX_POINT('',#15025);
#3971=VERTEX_POINT('',#15072);
#3972=VERTEX_POINT('',#15073);
#3973=VERTEX_POINT('',#15123);
#3974=VERTEX_POINT('',#15124);
#3975=VERTEX_POINT('',#15174);
#3976=VERTEX_POINT('',#15175);
#3977=VERTEX_POINT('',#15222);
#3978=VERTEX_POINT('',#15223);
#3979=VERTEX_POINT('',#15273);
#3980=VERTEX_POINT('',#15274);
#3981=VERTEX_POINT('',#15276);
#3982=VERTEX_POINT('',#15290);
#3983=VERTEX_POINT('',#15312);
#3984=VERTEX_POINT('',#15313);
#3985=VERTEX_POINT('',#15315);
#3986=VERTEX_POINT('',#15322);
#3987=VERTEX_POINT('',#15332);
#3988=VERTEX_POINT('',#15333);
#3989=VERTEX_POINT('',#15356);
#3990=VERTEX_POINT('',#15357);
#3991=VERTEX_POINT('',#15381);
#3992=VERTEX_POINT('',#15382);
#3993=VERTEX_POINT('',#15406);
#3994=VERTEX_POINT('',#15407);
#3995=VERTEX_POINT('',#15430);
#3996=VERTEX_POINT('',#15431);
#3997=VERTEX_POINT('',#15455);
#3998=VERTEX_POINT('',#15456);
#3999=VERTEX_POINT('',#15479);
#4000=VERTEX_POINT('',#15480);
#4001=VERTEX_POINT('',#15504);
#4002=VERTEX_POINT('',#15505);
#4003=VERTEX_POINT('',#15529);
#4004=VERTEX_POINT('',#15530);
#4005=VERTEX_POINT('',#15553);
#4006=VERTEX_POINT('',#15554);
#4007=VERTEX_POINT('',#15578);
#4008=VERTEX_POINT('',#15579);
#4009=VERTEX_POINT('',#15602);
#4010=VERTEX_POINT('',#15603);
#4011=VERTEX_POINT('',#15627);
#4012=VERTEX_POINT('',#15628);
#4013=VERTEX_POINT('',#15652);
#4014=VERTEX_POINT('',#15653);
#4015=VERTEX_POINT('',#15676);
#4016=VERTEX_POINT('',#15677);
#4017=VERTEX_POINT('',#15679);
#4018=VERTEX_POINT('',#15685);
#4019=VERTEX_POINT('',#15693);
#4020=VERTEX_POINT('',#15694);
#4021=VERTEX_POINT('',#15696);
#4022=VERTEX_POINT('',#15716);
#4023=VERTEX_POINT('',#15718);
#4024=VERTEX_POINT('',#15723);
#4025=VERTEX_POINT('',#15749);
#4026=VERTEX_POINT('',#15750);
#4027=VERTEX_POINT('',#15800);
#4028=VERTEX_POINT('',#15801);
#4029=VERTEX_POINT('',#15848);
#4030=VERTEX_POINT('',#15849);
#4031=VERTEX_POINT('',#15899);
#4032=VERTEX_POINT('',#15900);
#4033=VERTEX_POINT('',#15950);
#4034=VERTEX_POINT('',#15951);
#4035=VERTEX_POINT('',#15998);
#4036=VERTEX_POINT('',#15999);
#4037=VERTEX_POINT('',#16046);
#4038=VERTEX_POINT('',#16047);
#4039=VERTEX_POINT('',#16097);
#4040=VERTEX_POINT('',#16098);
#4041=VERTEX_POINT('',#16145);
#4042=VERTEX_POINT('',#16146);
#4043=VERTEX_POINT('',#16193);
#4044=VERTEX_POINT('',#16194);
#4045=VERTEX_POINT('',#16244);
#4046=VERTEX_POINT('',#16245);
#4047=VERTEX_POINT('',#16295);
#4048=VERTEX_POINT('',#16296);
#4049=VERTEX_POINT('',#16343);
#4050=VERTEX_POINT('',#16344);
#4051=VERTEX_POINT('',#16394);
#4052=VERTEX_POINT('',#16395);
#4053=VERTEX_POINT('',#16397);
#4054=VERTEX_POINT('',#16411);
#4055=VERTEX_POINT('',#16433);
#4056=VERTEX_POINT('',#16434);
#4057=VERTEX_POINT('',#16436);
#4058=VERTEX_POINT('',#16443);
#4059=VERTEX_POINT('',#16453);
#4060=VERTEX_POINT('',#16454);
#4061=VERTEX_POINT('',#16477);
#4062=VERTEX_POINT('',#16478);
#4063=VERTEX_POINT('',#16502);
#4064=VERTEX_POINT('',#16503);
#4065=VERTEX_POINT('',#16527);
#4066=VERTEX_POINT('',#16528);
#4067=VERTEX_POINT('',#16551);
#4068=VERTEX_POINT('',#16552);
#4069=VERTEX_POINT('',#16576);
#4070=VERTEX_POINT('',#16577);
#4071=VERTEX_POINT('',#16600);
#4072=VERTEX_POINT('',#16601);
#4073=VERTEX_POINT('',#16625);
#4074=VERTEX_POINT('',#16626);
#4075=VERTEX_POINT('',#16650);
#4076=VERTEX_POINT('',#16651);
#4077=VERTEX_POINT('',#16674);
#4078=VERTEX_POINT('',#16675);
#4079=VERTEX_POINT('',#16699);
#4080=VERTEX_POINT('',#16700);
#4081=VERTEX_POINT('',#16723);
#4082=VERTEX_POINT('',#16724);
#4083=VERTEX_POINT('',#16748);
#4084=VERTEX_POINT('',#16749);
#4085=VERTEX_POINT('',#16773);
#4086=VERTEX_POINT('',#16774);
#4087=VERTEX_POINT('',#16797);
#4088=VERTEX_POINT('',#16798);
#4089=VERTEX_POINT('',#16800);
#4090=VERTEX_POINT('',#16806);
#4091=VERTEX_POINT('',#16814);
#4092=VERTEX_POINT('',#16815);
#4093=VERTEX_POINT('',#16817);
#4094=VERTEX_POINT('',#16837);
#4095=VERTEX_POINT('',#16839);
#4096=VERTEX_POINT('',#16844);
#4097=VERTEX_POINT('',#16870);
#4098=VERTEX_POINT('',#16871);
#4099=VERTEX_POINT('',#16921);
#4100=VERTEX_POINT('',#16922);
#4101=VERTEX_POINT('',#16969);
#4102=VERTEX_POINT('',#16970);
#4103=VERTEX_POINT('',#17020);
#4104=VERTEX_POINT('',#17021);
#4105=VERTEX_POINT('',#17071);
#4106=VERTEX_POINT('',#17072);
#4107=VERTEX_POINT('',#17119);
#4108=VERTEX_POINT('',#17120);
#4109=VERTEX_POINT('',#17167);
#4110=VERTEX_POINT('',#17168);
#4111=VERTEX_POINT('',#17218);
#4112=VERTEX_POINT('',#17219);
#4113=VERTEX_POINT('',#17266);
#4114=VERTEX_POINT('',#17267);
#4115=VERTEX_POINT('',#17314);
#4116=VERTEX_POINT('',#17315);
#4117=VERTEX_POINT('',#17365);
#4118=VERTEX_POINT('',#17366);
#4119=VERTEX_POINT('',#17416);
#4120=VERTEX_POINT('',#17417);
#4121=VERTEX_POINT('',#17464);
#4122=VERTEX_POINT('',#17465);
#4123=VERTEX_POINT('',#17515);
#4124=VERTEX_POINT('',#17516);
#4125=VERTEX_POINT('',#17518);
#4126=VERTEX_POINT('',#17532);
#4127=VERTEX_POINT('',#17554);
#4128=VERTEX_POINT('',#17555);
#4129=VERTEX_POINT('',#17557);
#4130=VERTEX_POINT('',#17564);
#4131=VERTEX_POINT('',#17574);
#4132=VERTEX_POINT('',#17575);
#4133=VERTEX_POINT('',#17598);
#4134=VERTEX_POINT('',#17599);
#4135=VERTEX_POINT('',#17623);
#4136=VERTEX_POINT('',#17624);
#4137=VERTEX_POINT('',#17648);
#4138=VERTEX_POINT('',#17649);
#4139=VERTEX_POINT('',#17672);
#4140=VERTEX_POINT('',#17673);
#4141=VERTEX_POINT('',#17697);
#4142=VERTEX_POINT('',#17698);
#4143=VERTEX_POINT('',#17721);
#4144=VERTEX_POINT('',#17722);
#4145=VERTEX_POINT('',#17746);
#4146=VERTEX_POINT('',#17747);
#4147=VERTEX_POINT('',#17771);
#4148=VERTEX_POINT('',#17772);
#4149=VERTEX_POINT('',#17795);
#4150=VERTEX_POINT('',#17796);
#4151=VERTEX_POINT('',#17820);
#4152=VERTEX_POINT('',#17821);
#4153=VERTEX_POINT('',#17844);
#4154=VERTEX_POINT('',#17845);
#4155=VERTEX_POINT('',#17869);
#4156=VERTEX_POINT('',#17870);
#4157=VERTEX_POINT('',#17894);
#4158=VERTEX_POINT('',#17895);
#4159=VERTEX_POINT('',#17918);
#4160=VERTEX_POINT('',#17919);
#4161=VERTEX_POINT('',#17921);
#4162=VERTEX_POINT('',#17927);
#4163=VERTEX_POINT('',#17935);
#4164=VERTEX_POINT('',#17936);
#4165=VERTEX_POINT('',#17938);
#4166=VERTEX_POINT('',#17943);
#4167=VERTEX_POINT('',#17945);
#4168=VERTEX_POINT('',#17965);
#4169=VERTEX_POINT('',#17978);
#4170=VERTEX_POINT('',#17979);
#4171=VERTEX_POINT('',#18029);
#4172=VERTEX_POINT('',#18030);
#4173=VERTEX_POINT('',#18080);
#4174=VERTEX_POINT('',#18081);
#4175=VERTEX_POINT('',#18128);
#4176=VERTEX_POINT('',#18129);
#4177=VERTEX_POINT('',#18179);
#4178=VERTEX_POINT('',#18180);
#4179=VERTEX_POINT('',#18230);
#4180=VERTEX_POINT('',#18231);
#4181=VERTEX_POINT('',#18278);
#4182=VERTEX_POINT('',#18279);
#4183=VERTEX_POINT('',#18329);
#4184=VERTEX_POINT('',#18330);
#4185=VERTEX_POINT('',#18380);
#4186=VERTEX_POINT('',#18381);
#4187=VERTEX_POINT('',#18428);
#4188=VERTEX_POINT('',#18429);
#4189=VERTEX_POINT('',#18479);
#4190=VERTEX_POINT('',#18480);
#4191=VERTEX_POINT('',#18530);
#4192=VERTEX_POINT('',#18531);
#4193=VERTEX_POINT('',#18578);
#4194=VERTEX_POINT('',#18579);
#4195=VERTEX_POINT('',#18629);
#4196=VERTEX_POINT('',#18630);
#4197=VERTEX_POINT('',#18632);
#4198=VERTEX_POINT('',#18646);
#4199=VERTEX_POINT('',#18668);
#4200=VERTEX_POINT('',#18669);
#4201=VERTEX_POINT('',#18671);
#4202=VERTEX_POINT('',#18676);
#4203=VERTEX_POINT('',#18678);
#4204=VERTEX_POINT('',#18698);
#4205=VERTEX_POINT('',#18711);
#4206=VERTEX_POINT('',#18712);
#4207=VERTEX_POINT('',#18762);
#4208=VERTEX_POINT('',#18763);
#4209=VERTEX_POINT('',#18813);
#4210=VERTEX_POINT('',#18814);
#4211=VERTEX_POINT('',#18861);
#4212=VERTEX_POINT('',#18862);
#4213=VERTEX_POINT('',#18912);
#4214=VERTEX_POINT('',#18913);
#4215=VERTEX_POINT('',#18963);
#4216=VERTEX_POINT('',#18964);
#4217=VERTEX_POINT('',#19011);
#4218=VERTEX_POINT('',#19012);
#4219=VERTEX_POINT('',#19062);
#4220=VERTEX_POINT('',#19063);
#4221=VERTEX_POINT('',#19113);
#4222=VERTEX_POINT('',#19114);
#4223=VERTEX_POINT('',#19161);
#4224=VERTEX_POINT('',#19162);
#4225=VERTEX_POINT('',#19212);
#4226=VERTEX_POINT('',#19213);
#4227=VERTEX_POINT('',#19263);
#4228=VERTEX_POINT('',#19264);
#4229=VERTEX_POINT('',#19311);
#4230=VERTEX_POINT('',#19312);
#4231=VERTEX_POINT('',#19362);
#4232=VERTEX_POINT('',#19363);
#4233=VERTEX_POINT('',#19365);
#4234=VERTEX_POINT('',#19379);
#4235=VERTEX_POINT('',#19401);
#4236=VERTEX_POINT('',#19402);
#4237=VERTEX_POINT('',#19404);
#4238=VERTEX_POINT('',#19413);
#4239=VERTEX_POINT('',#19425);
#4240=VERTEX_POINT('',#19426);
#4241=VERTEX_POINT('',#19449);
#4242=VERTEX_POINT('',#19450);
#4243=VERTEX_POINT('',#19474);
#4244=VERTEX_POINT('',#19475);
#4245=VERTEX_POINT('',#19499);
#4246=VERTEX_POINT('',#19500);
#4247=VERTEX_POINT('',#19523);
#4248=VERTEX_POINT('',#19524);
#4249=VERTEX_POINT('',#19548);
#4250=VERTEX_POINT('',#19549);
#4251=VERTEX_POINT('',#19573);
#4252=VERTEX_POINT('',#19574);
#4253=VERTEX_POINT('',#19597);
#4254=VERTEX_POINT('',#19598);
#4255=VERTEX_POINT('',#19622);
#4256=VERTEX_POINT('',#19623);
#4257=VERTEX_POINT('',#19647);
#4258=VERTEX_POINT('',#19648);
#4259=VERTEX_POINT('',#19671);
#4260=VERTEX_POINT('',#19672);
#4261=VERTEX_POINT('',#19696);
#4262=VERTEX_POINT('',#19697);
#4263=VERTEX_POINT('',#19721);
#4264=VERTEX_POINT('',#19722);
#4265=VERTEX_POINT('',#19745);
#4266=VERTEX_POINT('',#19746);
#4267=VERTEX_POINT('',#19748);
#4268=VERTEX_POINT('',#19754);
#4269=VERTEX_POINT('',#19762);
#4270=VERTEX_POINT('',#19763);
#4271=VERTEX_POINT('',#19765);
#4272=VERTEX_POINT('',#19774);
#4273=VERTEX_POINT('',#19786);
#4274=VERTEX_POINT('',#19787);
#4275=VERTEX_POINT('',#19810);
#4276=VERTEX_POINT('',#19811);
#4277=VERTEX_POINT('',#19835);
#4278=VERTEX_POINT('',#19836);
#4279=VERTEX_POINT('',#19860);
#4280=VERTEX_POINT('',#19861);
#4281=VERTEX_POINT('',#19884);
#4282=VERTEX_POINT('',#19885);
#4283=VERTEX_POINT('',#19909);
#4284=VERTEX_POINT('',#19910);
#4285=VERTEX_POINT('',#19934);
#4286=VERTEX_POINT('',#19935);
#4287=VERTEX_POINT('',#19958);
#4288=VERTEX_POINT('',#19959);
#4289=VERTEX_POINT('',#19983);
#4290=VERTEX_POINT('',#19984);
#4291=VERTEX_POINT('',#20008);
#4292=VERTEX_POINT('',#20009);
#4293=VERTEX_POINT('',#20032);
#4294=VERTEX_POINT('',#20033);
#4295=VERTEX_POINT('',#20057);
#4296=VERTEX_POINT('',#20058);
#4297=VERTEX_POINT('',#20082);
#4298=VERTEX_POINT('',#20083);
#4299=VERTEX_POINT('',#20106);
#4300=VERTEX_POINT('',#20107);
#4301=VERTEX_POINT('',#20109);
#4302=VERTEX_POINT('',#20115);
#4303=VERTEX_POINT('',#20123);
#4304=VERTEX_POINT('',#20124);
#4305=VERTEX_POINT('',#20126);
#4306=VERTEX_POINT('',#20131);
#4307=VERTEX_POINT('',#20133);
#4308=VERTEX_POINT('',#20136);
#4309=VERTEX_POINT('',#20149);
#4310=VERTEX_POINT('',#20150);
#4311=VERTEX_POINT('',#20200);
#4312=VERTEX_POINT('',#20201);
#4313=VERTEX_POINT('',#20251);
#4314=VERTEX_POINT('',#20252);
#4315=VERTEX_POINT('',#20299);
#4316=VERTEX_POINT('',#20300);
#4317=VERTEX_POINT('',#20350);
#4318=VERTEX_POINT('',#20351);
#4319=VERTEX_POINT('',#20401);
#4320=VERTEX_POINT('',#20402);
#4321=VERTEX_POINT('',#20449);
#4322=VERTEX_POINT('',#20450);
#4323=VERTEX_POINT('',#20500);
#4324=VERTEX_POINT('',#20501);
#4325=VERTEX_POINT('',#20551);
#4326=VERTEX_POINT('',#20552);
#4327=VERTEX_POINT('',#20599);
#4328=VERTEX_POINT('',#20600);
#4329=VERTEX_POINT('',#20650);
#4330=VERTEX_POINT('',#20651);
#4331=VERTEX_POINT('',#20701);
#4332=VERTEX_POINT('',#20702);
#4333=VERTEX_POINT('',#20749);
#4334=VERTEX_POINT('',#20750);
#4335=VERTEX_POINT('',#20800);
#4336=VERTEX_POINT('',#20801);
#4337=VERTEX_POINT('',#20803);
#4338=VERTEX_POINT('',#20817);
#4339=VERTEX_POINT('',#20839);
#4340=VERTEX_POINT('',#20840);
#4341=VERTEX_POINT('',#20842);
#4342=VERTEX_POINT('',#20851);
#4343=VERTEX_POINT('',#20863);
#4344=VERTEX_POINT('',#20864);
#4345=VERTEX_POINT('',#20887);
#4346=VERTEX_POINT('',#20888);
#4347=VERTEX_POINT('',#20912);
#4348=VERTEX_POINT('',#20913);
#4349=VERTEX_POINT('',#20937);
#4350=VERTEX_POINT('',#20938);
#4351=VERTEX_POINT('',#20961);
#4352=VERTEX_POINT('',#20962);
#4353=VERTEX_POINT('',#20986);
#4354=VERTEX_POINT('',#20987);
#4355=VERTEX_POINT('',#21011);
#4356=VERTEX_POINT('',#21012);
#4357=VERTEX_POINT('',#21035);
#4358=VERTEX_POINT('',#21036);
#4359=VERTEX_POINT('',#21060);
#4360=VERTEX_POINT('',#21061);
#4361=VERTEX_POINT('',#21085);
#4362=VERTEX_POINT('',#21086);
#4363=VERTEX_POINT('',#21109);
#4364=VERTEX_POINT('',#21110);
#4365=VERTEX_POINT('',#21134);
#4366=VERTEX_POINT('',#21135);
#4367=VERTEX_POINT('',#21159);
#4368=VERTEX_POINT('',#21160);
#4369=VERTEX_POINT('',#21183);
#4370=VERTEX_POINT('',#21184);
#4371=VERTEX_POINT('',#21186);
#4372=VERTEX_POINT('',#21192);
#4373=VERTEX_POINT('',#21200);
#4374=VERTEX_POINT('',#21201);
#4375=VERTEX_POINT('',#21203);
#4376=VERTEX_POINT('',#21208);
#4377=VERTEX_POINT('',#21210);
#4378=VERTEX_POINT('',#21213);
#4379=VERTEX_POINT('',#21226);
#4380=VERTEX_POINT('',#21227);
#4381=VERTEX_POINT('',#21277);
#4382=VERTEX_POINT('',#21278);
#4383=VERTEX_POINT('',#21328);
#4384=VERTEX_POINT('',#21329);
#4385=VERTEX_POINT('',#21376);
#4386=VERTEX_POINT('',#21377);
#4387=VERTEX_POINT('',#21427);
#4388=VERTEX_POINT('',#21428);
#4389=VERTEX_POINT('',#21478);
#4390=VERTEX_POINT('',#21479);
#4391=VERTEX_POINT('',#21526);
#4392=VERTEX_POINT('',#21527);
#4393=VERTEX_POINT('',#21577);
#4394=VERTEX_POINT('',#21578);
#4395=VERTEX_POINT('',#21628);
#4396=VERTEX_POINT('',#21629);
#4397=VERTEX_POINT('',#21676);
#4398=VERTEX_POINT('',#21677);
#4399=VERTEX_POINT('',#21727);
#4400=VERTEX_POINT('',#21728);
#4401=VERTEX_POINT('',#21778);
#4402=VERTEX_POINT('',#21779);
#4403=VERTEX_POINT('',#21826);
#4404=VERTEX_POINT('',#21827);
#4405=VERTEX_POINT('',#21877);
#4406=VERTEX_POINT('',#21878);
#4407=VERTEX_POINT('',#21880);
#4408=VERTEX_POINT('',#21894);
#4409=VERTEX_POINT('',#21916);
#4410=VERTEX_POINT('',#21917);
#4411=VERTEX_POINT('',#21919);
#4412=VERTEX_POINT('',#21928);
#4413=VERTEX_POINT('',#21940);
#4414=VERTEX_POINT('',#21941);
#4415=VERTEX_POINT('',#21964);
#4416=VERTEX_POINT('',#21965);
#4417=VERTEX_POINT('',#21989);
#4418=VERTEX_POINT('',#21990);
#4419=VERTEX_POINT('',#22014);
#4420=VERTEX_POINT('',#22015);
#4421=VERTEX_POINT('',#22038);
#4422=VERTEX_POINT('',#22039);
#4423=VERTEX_POINT('',#22063);
#4424=VERTEX_POINT('',#22064);
#4425=VERTEX_POINT('',#22088);
#4426=VERTEX_POINT('',#22089);
#4427=VERTEX_POINT('',#22112);
#4428=VERTEX_POINT('',#22113);
#4429=VERTEX_POINT('',#22137);
#4430=VERTEX_POINT('',#22138);
#4431=VERTEX_POINT('',#22162);
#4432=VERTEX_POINT('',#22163);
#4433=VERTEX_POINT('',#22186);
#4434=VERTEX_POINT('',#22187);
#4435=VERTEX_POINT('',#22211);
#4436=VERTEX_POINT('',#22212);
#4437=VERTEX_POINT('',#22236);
#4438=VERTEX_POINT('',#22237);
#4439=VERTEX_POINT('',#22260);
#4440=VERTEX_POINT('',#22261);
#4441=VERTEX_POINT('',#22263);
#4442=VERTEX_POINT('',#22269);
#4443=VERTEX_POINT('',#22277);
#4444=VERTEX_POINT('',#22278);
#4445=VERTEX_POINT('',#22280);
#4446=VERTEX_POINT('',#22306);
#4447=VERTEX_POINT('',#22346);
#4448=VERTEX_POINT('',#22347);
#4449=VERTEX_POINT('',#22436);
#4450=VERTEX_POINT('',#22437);
#4451=VERTEX_POINT('',#22523);
#4452=VERTEX_POINT('',#22524);
#4453=VERTEX_POINT('',#22613);
#4454=VERTEX_POINT('',#22614);
#4455=VERTEX_POINT('',#22700);
#4456=VERTEX_POINT('',#22701);
#4457=VERTEX_POINT('',#22790);
#4458=VERTEX_POINT('',#22791);
#4459=VERTEX_POINT('',#22877);
#4460=VERTEX_POINT('',#22878);
#4461=VERTEX_POINT('',#22880);
#4462=VERTEX_POINT('',#22888);
#4463=VERTEX_POINT('',#22910);
#4464=VERTEX_POINT('',#22911);
#4465=VERTEX_POINT('',#22913);
#4466=VERTEX_POINT('',#22927);
#4467=VERTEX_POINT('',#22944);
#4468=VERTEX_POINT('',#22945);
#4469=VERTEX_POINT('',#22980);
#4470=VERTEX_POINT('',#22981);
#4471=VERTEX_POINT('',#23018);
#4472=VERTEX_POINT('',#23019);
#4473=VERTEX_POINT('',#23056);
#4474=VERTEX_POINT('',#23057);
#4475=VERTEX_POINT('',#23093);
#4476=VERTEX_POINT('',#23094);
#4477=VERTEX_POINT('',#23130);
#4478=VERTEX_POINT('',#23131);
#4479=VERTEX_POINT('',#23168);
#4480=VERTEX_POINT('',#23169);
#4481=VERTEX_POINT('',#23171);
#4482=VERTEX_POINT('',#23178);
#4483=VERTEX_POINT('',#24644);
#4484=VERTEX_POINT('',#24648);
#4485=VERTEX_POINT('',#24652);
#4486=VERTEX_POINT('',#24653);
#4487=VERTEX_POINT('',#24655);
#4488=VERTEX_POINT('',#24657);
#4489=VERTEX_POINT('',#27519);
#4490=VERTEX_POINT('',#27553);
#4491=VERTEX_POINT('',#28591);
#4492=VERTEX_POINT('',#28613);
#4493=VERTEX_POINT('',#28647);
#4494=VERTEX_POINT('',#29685);
#4495=VERTEX_POINT('',#34687);
#4496=VERTEX_POINT('',#34689);
#4497=VERTEX_POINT('',#34693);
#4498=VERTEX_POINT('',#34695);
#4499=VERTEX_POINT('',#34699);
#4500=VERTEX_POINT('',#34701);
#4501=VERTEX_POINT('',#34705);
#4502=VERTEX_POINT('',#34707);
#4503=VERTEX_POINT('',#34711);
#4504=VERTEX_POINT('',#34713);
#4505=VERTEX_POINT('',#34717);
#4506=VERTEX_POINT('',#34719);
#4507=VERTEX_POINT('',#34723);
#4508=VERTEX_POINT('',#34725);
#4509=VERTEX_POINT('',#34729);
#4510=VERTEX_POINT('',#34731);
#4511=VERTEX_POINT('',#34735);
#4512=VERTEX_POINT('',#34738);
#4513=VERTEX_POINT('',#34742);
#4514=VERTEX_POINT('',#34744);
#4515=VERTEX_POINT('',#34748);
#4516=VERTEX_POINT('',#34750);
#4517=VERTEX_POINT('',#34754);
#4518=VERTEX_POINT('',#34756);
#4519=VERTEX_POINT('',#34760);
#4520=VERTEX_POINT('',#34762);
#4521=VERTEX_POINT('',#34766);
#4522=VERTEX_POINT('',#34768);
#4523=VERTEX_POINT('',#34772);
#4524=VERTEX_POINT('',#34774);
#4525=VERTEX_POINT('',#34778);
#4526=VERTEX_POINT('',#34780);
#4527=VERTEX_POINT('',#34784);
#4528=VERTEX_POINT('',#34787);
#4529=VERTEX_POINT('',#34791);
#4530=VERTEX_POINT('',#34793);
#4531=VERTEX_POINT('',#34797);
#4532=VERTEX_POINT('',#34798);
#4533=VERTEX_POINT('',#34800);
#4534=VERTEX_POINT('',#34802);
#4535=VERTEX_POINT('',#34806);
#4536=VERTEX_POINT('',#34808);
#4537=VERTEX_POINT('',#34812);
#4538=VERTEX_POINT('',#34814);
#4539=VERTEX_POINT('',#34822);
#4540=VERTEX_POINT('',#34824);
#4541=VERTEX_POINT('',#34828);
#4542=VERTEX_POINT('',#34832);
#4877=EDGE_CURVE('',#3875,#3876,#2799,.T.);
#4878=EDGE_CURVE('',#3876,#3877,#2021,.T.);
#4879=EDGE_CURVE('',#3877,#3878,#1825,.T.);
#4880=EDGE_CURVE('',#3878,#3879,#2022,.T.);
#4881=EDGE_CURVE('',#3879,#3880,#2800,.T.);
#4882=EDGE_CURVE('',#3880,#3880,#1826,.F.);
#4883=EDGE_CURVE('',#3879,#3875,#2023,.T.);
#4884=EDGE_CURVE('',#3881,#3882,#2801,.T.);
#4885=EDGE_CURVE('',#3882,#3876,#2024,.T.);
#4886=EDGE_CURVE('',#3875,#3881,#2025,.T.);
#4887=EDGE_CURVE('',#3883,#3884,#2802,.T.);
#4888=EDGE_CURVE('',#3884,#3882,#2026,.T.);
#4889=EDGE_CURVE('',#3881,#3883,#2027,.T.);
#4890=EDGE_CURVE('',#3885,#3886,#2803,.T.);
#4891=EDGE_CURVE('',#3886,#3884,#2028,.T.);
#4892=EDGE_CURVE('',#3883,#3885,#2029,.T.);
#4893=EDGE_CURVE('',#3887,#3888,#2804,.T.);
#4894=EDGE_CURVE('',#3888,#3886,#2030,.T.);
#4895=EDGE_CURVE('',#3885,#3887,#2031,.T.);
#4896=EDGE_CURVE('',#3889,#3890,#2805,.T.);
#4897=EDGE_CURVE('',#3890,#3888,#2032,.T.);
#4898=EDGE_CURVE('',#3887,#3889,#2033,.T.);
#4899=EDGE_CURVE('',#3891,#3892,#2806,.T.);
#4900=EDGE_CURVE('',#3892,#3890,#2034,.T.);
#4901=EDGE_CURVE('',#3889,#3891,#2035,.T.);
#4902=EDGE_CURVE('',#3893,#3894,#2807,.T.);
#4903=EDGE_CURVE('',#3894,#3892,#2036,.T.);
#4904=EDGE_CURVE('',#3891,#3893,#2037,.T.);
#4905=EDGE_CURVE('',#3895,#3896,#2808,.T.);
#4906=EDGE_CURVE('',#3896,#3894,#2038,.T.);
#4907=EDGE_CURVE('',#3893,#3895,#2039,.T.);
#4908=EDGE_CURVE('',#3897,#3898,#2809,.T.);
#4909=EDGE_CURVE('',#3898,#3896,#2040,.T.);
#4910=EDGE_CURVE('',#3895,#3897,#2041,.T.);
#4911=EDGE_CURVE('',#3899,#3900,#2810,.T.);
#4912=EDGE_CURVE('',#3900,#3898,#2042,.T.);
#4913=EDGE_CURVE('',#3897,#3899,#2043,.T.);
#4914=EDGE_CURVE('',#3901,#3902,#2811,.T.);
#4915=EDGE_CURVE('',#3902,#3900,#2044,.T.);
#4916=EDGE_CURVE('',#3899,#3901,#2045,.T.);
#4917=EDGE_CURVE('',#3903,#3904,#2812,.T.);
#4918=EDGE_CURVE('',#3904,#3902,#2046,.T.);
#4919=EDGE_CURVE('',#3901,#3903,#2047,.T.);
#4920=EDGE_CURVE('',#3905,#3906,#2813,.T.);
#4921=EDGE_CURVE('',#3906,#3904,#2048,.T.);
#4922=EDGE_CURVE('',#3903,#3905,#2049,.T.);
#4923=EDGE_CURVE('',#3907,#3908,#2814,.T.);
#4924=EDGE_CURVE('',#3907,#3909,#2050,.T.);
#4925=EDGE_CURVE('',#3910,#3909,#1827,.T.);
#4926=EDGE_CURVE('',#3910,#3908,#2051,.T.);
#4927=EDGE_CURVE('',#3911,#3912,#2815,.T.);
#4928=EDGE_CURVE('',#3912,#3913,#2052,.T.);
#4929=EDGE_CURVE('',#3914,#3913,#1828,.T.);
#4930=EDGE_CURVE('',#3911,#3914,#2053,.T.);
#4931=EDGE_CURVE('',#3915,#3916,#2816,.T.);
#4932=EDGE_CURVE('',#3916,#3912,#2054,.T.);
#4933=EDGE_CURVE('',#3915,#3911,#2055,.T.);
#4934=EDGE_CURVE('',#3917,#3918,#2817,.T.);
#4935=EDGE_CURVE('',#3918,#3916,#2056,.T.);
#4936=EDGE_CURVE('',#3917,#3915,#2057,.T.);
#4937=EDGE_CURVE('',#3919,#3920,#2818,.T.);
#4938=EDGE_CURVE('',#3920,#3918,#2058,.T.);
#4939=EDGE_CURVE('',#3919,#3917,#2059,.T.);
#4940=EDGE_CURVE('',#3921,#3922,#2819,.T.);
#4941=EDGE_CURVE('',#3922,#3920,#2060,.T.);
#4942=EDGE_CURVE('',#3921,#3919,#2061,.T.);
#4943=EDGE_CURVE('',#3923,#3924,#2820,.T.);
#4944=EDGE_CURVE('',#3924,#3922,#2062,.T.);
#4945=EDGE_CURVE('',#3923,#3921,#2063,.T.);
#4946=EDGE_CURVE('',#3925,#3926,#2821,.T.);
#4947=EDGE_CURVE('',#3926,#3924,#2064,.T.);
#4948=EDGE_CURVE('',#3925,#3923,#2065,.T.);
#4949=EDGE_CURVE('',#3927,#3928,#2822,.T.);
#4950=EDGE_CURVE('',#3928,#3926,#2066,.T.);
#4951=EDGE_CURVE('',#3927,#3925,#2067,.T.);
#4952=EDGE_CURVE('',#3929,#3930,#2823,.T.);
#4953=EDGE_CURVE('',#3930,#3928,#2068,.T.);
#4954=EDGE_CURVE('',#3929,#3927,#2069,.T.);
#4955=EDGE_CURVE('',#3931,#3932,#2824,.T.);
#4956=EDGE_CURVE('',#3932,#3930,#2070,.T.);
#4957=EDGE_CURVE('',#3931,#3929,#2071,.T.);
#4958=EDGE_CURVE('',#3933,#3934,#2825,.T.);
#4959=EDGE_CURVE('',#3934,#3932,#2072,.T.);
#4960=EDGE_CURVE('',#3933,#3931,#2073,.T.);
#4961=EDGE_CURVE('',#3935,#3936,#2826,.T.);
#4962=EDGE_CURVE('',#3936,#3934,#2074,.T.);
#4963=EDGE_CURVE('',#3935,#3933,#2075,.T.);
#4964=EDGE_CURVE('',#3937,#3938,#2827,.T.);
#4965=EDGE_CURVE('',#3938,#3936,#2076,.T.);
#4966=EDGE_CURVE('',#3937,#3935,#2077,.T.);
#4967=EDGE_CURVE('',#3939,#3940,#2828,.T.);
#4968=EDGE_CURVE('',#3940,#3938,#2078,.T.);
#4969=EDGE_CURVE('',#3939,#3937,#2079,.T.);
#4970=EDGE_CURVE('',#3941,#3942,#2829,.T.);
#4971=EDGE_CURVE('',#3942,#3940,#2080,.T.);
#4972=EDGE_CURVE('',#3941,#3939,#2081,.T.);
#4973=EDGE_CURVE('',#3943,#3944,#2830,.T.);
#4974=EDGE_CURVE('',#3945,#3943,#2082,.T.);
#4975=EDGE_CURVE('',#3946,#3945,#1829,.T.);
#4976=EDGE_CURVE('',#3946,#3944,#2083,.T.);
#4977=EDGE_CURVE('',#3947,#3948,#2831,.T.);
#4978=EDGE_CURVE('',#3948,#3949,#2084,.T.);
#4979=EDGE_CURVE('',#3949,#3950,#1830,.T.);
#4980=EDGE_CURVE('',#3950,#3951,#2085,.T.);
#4981=EDGE_CURVE('',#3951,#3952,#2832,.T.);
#4982=EDGE_CURVE('',#3952,#3952,#1831,.F.);
#4983=EDGE_CURVE('',#3951,#3947,#2086,.T.);
#4984=EDGE_CURVE('',#3953,#3954,#2833,.T.);
#4985=EDGE_CURVE('',#3954,#3948,#2087,.T.);
#4986=EDGE_CURVE('',#3947,#3953,#2088,.T.);
#4987=EDGE_CURVE('',#3955,#3956,#2834,.T.);
#4988=EDGE_CURVE('',#3956,#3954,#2089,.T.);
#4989=EDGE_CURVE('',#3953,#3955,#2090,.T.);
#4990=EDGE_CURVE('',#3957,#3958,#2835,.T.);
#4991=EDGE_CURVE('',#3958,#3956,#2091,.T.);
#4992=EDGE_CURVE('',#3955,#3957,#2092,.T.);
#4993=EDGE_CURVE('',#3959,#3960,#2836,.T.);
#4994=EDGE_CURVE('',#3960,#3958,#2093,.T.);
#4995=EDGE_CURVE('',#3957,#3959,#2094,.T.);
#4996=EDGE_CURVE('',#3961,#3962,#2837,.T.);
#4997=EDGE_CURVE('',#3962,#3960,#2095,.T.);
#4998=EDGE_CURVE('',#3959,#3961,#2096,.T.);
#4999=EDGE_CURVE('',#3963,#3964,#2838,.T.);
#5000=EDGE_CURVE('',#3964,#3962,#2097,.T.);
#5001=EDGE_CURVE('',#3961,#3963,#2098,.T.);
#5002=EDGE_CURVE('',#3965,#3966,#2839,.T.);
#5003=EDGE_CURVE('',#3966,#3964,#2099,.T.);
#5004=EDGE_CURVE('',#3963,#3965,#2100,.T.);
#5005=EDGE_CURVE('',#3967,#3968,#2840,.T.);
#5006=EDGE_CURVE('',#3968,#3966,#2101,.T.);
#5007=EDGE_CURVE('',#3965,#3967,#2102,.T.);
#5008=EDGE_CURVE('',#3969,#3970,#2841,.T.);
#5009=EDGE_CURVE('',#3970,#3968,#2103,.T.);
#5010=EDGE_CURVE('',#3967,#3969,#2104,.T.);
#5011=EDGE_CURVE('',#3971,#3972,#2842,.T.);
#5012=EDGE_CURVE('',#3972,#3970,#2105,.T.);
#5013=EDGE_CURVE('',#3969,#3971,#2106,.T.);
#5014=EDGE_CURVE('',#3973,#3974,#2843,.T.);
#5015=EDGE_CURVE('',#3974,#3972,#2107,.T.);
#5016=EDGE_CURVE('',#3971,#3973,#2108,.T.);
#5017=EDGE_CURVE('',#3975,#3976,#2844,.T.);
#5018=EDGE_CURVE('',#3976,#3974,#2109,.T.);
#5019=EDGE_CURVE('',#3973,#3975,#2110,.T.);
#5020=EDGE_CURVE('',#3977,#3978,#2845,.T.);
#5021=EDGE_CURVE('',#3978,#3976,#2111,.T.);
#5022=EDGE_CURVE('',#3975,#3977,#2112,.T.);
#5023=EDGE_CURVE('',#3979,#3980,#2846,.T.);
#5024=EDGE_CURVE('',#3979,#3981,#2113,.T.);
#5025=EDGE_CURVE('',#3982,#3981,#1832,.T.);
#5026=EDGE_CURVE('',#3982,#3980,#2114,.T.);
#5027=EDGE_CURVE('',#3983,#3984,#2847,.T.);
#5028=EDGE_CURVE('',#3984,#3985,#2115,.T.);
#5029=EDGE_CURVE('',#3986,#3985,#1833,.T.);
#5030=EDGE_CURVE('',#3983,#3986,#2116,.T.);
#5031=EDGE_CURVE('',#3987,#3988,#2848,.T.);
#5032=EDGE_CURVE('',#3988,#3984,#2117,.T.);
#5033=EDGE_CURVE('',#3987,#3983,#2118,.T.);
#5034=EDGE_CURVE('',#3989,#3990,#2849,.T.);
#5035=EDGE_CURVE('',#3990,#3988,#2119,.T.);
#5036=EDGE_CURVE('',#3989,#3987,#2120,.T.);
#5037=EDGE_CURVE('',#3991,#3992,#2850,.T.);
#5038=EDGE_CURVE('',#3992,#3990,#2121,.T.);
#5039=EDGE_CURVE('',#3991,#3989,#2122,.T.);
#5040=EDGE_CURVE('',#3993,#3994,#2851,.T.);
#5041=EDGE_CURVE('',#3994,#3992,#2123,.T.);
#5042=EDGE_CURVE('',#3993,#3991,#2124,.T.);
#5043=EDGE_CURVE('',#3995,#3996,#2852,.T.);
#5044=EDGE_CURVE('',#3996,#3994,#2125,.T.);
#5045=EDGE_CURVE('',#3995,#3993,#2126,.T.);
#5046=EDGE_CURVE('',#3997,#3998,#2853,.T.);
#5047=EDGE_CURVE('',#3998,#3996,#2127,.T.);
#5048=EDGE_CURVE('',#3997,#3995,#2128,.T.);
#5049=EDGE_CURVE('',#3999,#4000,#2854,.T.);
#5050=EDGE_CURVE('',#4000,#3998,#2129,.T.);
#5051=EDGE_CURVE('',#3999,#3997,#2130,.T.);
#5052=EDGE_CURVE('',#4001,#4002,#2855,.T.);
#5053=EDGE_CURVE('',#4002,#4000,#2131,.T.);
#5054=EDGE_CURVE('',#4001,#3999,#2132,.T.);
#5055=EDGE_CURVE('',#4003,#4004,#2856,.T.);
#5056=EDGE_CURVE('',#4004,#4002,#2133,.T.);
#5057=EDGE_CURVE('',#4003,#4001,#2134,.T.);
#5058=EDGE_CURVE('',#4005,#4006,#2857,.T.);
#5059=EDGE_CURVE('',#4006,#4004,#2135,.T.);
#5060=EDGE_CURVE('',#4005,#4003,#2136,.T.);
#5061=EDGE_CURVE('',#4007,#4008,#2858,.T.);
#5062=EDGE_CURVE('',#4008,#4006,#2137,.T.);
#5063=EDGE_CURVE('',#4007,#4005,#2138,.T.);
#5064=EDGE_CURVE('',#4009,#4010,#2859,.T.);
#5065=EDGE_CURVE('',#4010,#4008,#2139,.T.);
#5066=EDGE_CURVE('',#4009,#4007,#2140,.T.);
#5067=EDGE_CURVE('',#4011,#4012,#2860,.T.);
#5068=EDGE_CURVE('',#4012,#4010,#2141,.T.);
#5069=EDGE_CURVE('',#4011,#4009,#2142,.T.);
#5070=EDGE_CURVE('',#4013,#4014,#2861,.T.);
#5071=EDGE_CURVE('',#4014,#4012,#2143,.T.);
#5072=EDGE_CURVE('',#4013,#4011,#2144,.T.);
#5073=EDGE_CURVE('',#4015,#4016,#2862,.T.);
#5074=EDGE_CURVE('',#4017,#4015,#2145,.T.);
#5075=EDGE_CURVE('',#4018,#4017,#1834,.T.);
#5076=EDGE_CURVE('',#4018,#4016,#2146,.T.);
#5077=EDGE_CURVE('',#4019,#4020,#2863,.T.);
#5078=EDGE_CURVE('',#4020,#4021,#2147,.T.);
#5079=EDGE_CURVE('',#4021,#4022,#1835,.T.);
#5080=EDGE_CURVE('',#4022,#4023,#2148,.T.);
#5081=EDGE_CURVE('',#4023,#4024,#2864,.T.);
#5082=EDGE_CURVE('',#4024,#4024,#1836,.F.);
#5083=EDGE_CURVE('',#4023,#4019,#2149,.T.);
#5084=EDGE_CURVE('',#4025,#4026,#2865,.T.);
#5085=EDGE_CURVE('',#4026,#4020,#2150,.T.);
#5086=EDGE_CURVE('',#4019,#4025,#2151,.T.);
#5087=EDGE_CURVE('',#4027,#4028,#2866,.T.);
#5088=EDGE_CURVE('',#4028,#4026,#2152,.T.);
#5089=EDGE_CURVE('',#4025,#4027,#2153,.T.);
#5090=EDGE_CURVE('',#4029,#4030,#2867,.T.);
#5091=EDGE_CURVE('',#4030,#4028,#2154,.T.);
#5092=EDGE_CURVE('',#4027,#4029,#2155,.T.);
#5093=EDGE_CURVE('',#4031,#4032,#2868,.T.);
#5094=EDGE_CURVE('',#4032,#4030,#2156,.T.);
#5095=EDGE_CURVE('',#4029,#4031,#2157,.T.);
#5096=EDGE_CURVE('',#4033,#4034,#2869,.T.);
#5097=EDGE_CURVE('',#4034,#4032,#2158,.T.);
#5098=EDGE_CURVE('',#4031,#4033,#2159,.T.);
#5099=EDGE_CURVE('',#4035,#4036,#2870,.T.);
#5100=EDGE_CURVE('',#4036,#4034,#2160,.T.);
#5101=EDGE_CURVE('',#4033,#4035,#2161,.T.);
#5102=EDGE_CURVE('',#4037,#4038,#2871,.T.);
#5103=EDGE_CURVE('',#4038,#4036,#2162,.T.);
#5104=EDGE_CURVE('',#4035,#4037,#2163,.T.);
#5105=EDGE_CURVE('',#4039,#4040,#2872,.T.);
#5106=EDGE_CURVE('',#4040,#4038,#2164,.T.);
#5107=EDGE_CURVE('',#4037,#4039,#2165,.T.);
#5108=EDGE_CURVE('',#4041,#4042,#2873,.T.);
#5109=EDGE_CURVE('',#4042,#4040,#2166,.T.);
#5110=EDGE_CURVE('',#4039,#4041,#2167,.T.);
#5111=EDGE_CURVE('',#4043,#4044,#2874,.T.);
#5112=EDGE_CURVE('',#4044,#4042,#2168,.T.);
#5113=EDGE_CURVE('',#4041,#4043,#2169,.T.);
#5114=EDGE_CURVE('',#4045,#4046,#2875,.T.);
#5115=EDGE_CURVE('',#4046,#4044,#2170,.T.);
#5116=EDGE_CURVE('',#4043,#4045,#2171,.T.);
#5117=EDGE_CURVE('',#4047,#4048,#2876,.T.);
#5118=EDGE_CURVE('',#4048,#4046,#2172,.T.);
#5119=EDGE_CURVE('',#4045,#4047,#2173,.T.);
#5120=EDGE_CURVE('',#4049,#4050,#2877,.T.);
#5121=EDGE_CURVE('',#4050,#4048,#2174,.T.);
#5122=EDGE_CURVE('',#4047,#4049,#2175,.T.);
#5123=EDGE_CURVE('',#4051,#4052,#2878,.T.);
#5124=EDGE_CURVE('',#4051,#4053,#2176,.T.);
#5125=EDGE_CURVE('',#4054,#4053,#1837,.T.);
#5126=EDGE_CURVE('',#4054,#4052,#2177,.T.);
#5127=EDGE_CURVE('',#4055,#4056,#2879,.T.);
#5128=EDGE_CURVE('',#4056,#4057,#2178,.T.);
#5129=EDGE_CURVE('',#4058,#4057,#1838,.T.);
#5130=EDGE_CURVE('',#4055,#4058,#2179,.T.);
#5131=EDGE_CURVE('',#4059,#4060,#2880,.T.);
#5132=EDGE_CURVE('',#4060,#4056,#2180,.T.);
#5133=EDGE_CURVE('',#4059,#4055,#2181,.T.);
#5134=EDGE_CURVE('',#4061,#4062,#2881,.T.);
#5135=EDGE_CURVE('',#4062,#4060,#2182,.T.);
#5136=EDGE_CURVE('',#4061,#4059,#2183,.T.);
#5137=EDGE_CURVE('',#4063,#4064,#2882,.T.);
#5138=EDGE_CURVE('',#4064,#4062,#2184,.T.);
#5139=EDGE_CURVE('',#4063,#4061,#2185,.T.);
#5140=EDGE_CURVE('',#4065,#4066,#2883,.T.);
#5141=EDGE_CURVE('',#4066,#4064,#2186,.T.);
#5142=EDGE_CURVE('',#4065,#4063,#2187,.T.);
#5143=EDGE_CURVE('',#4067,#4068,#2884,.T.);
#5144=EDGE_CURVE('',#4068,#4066,#2188,.T.);
#5145=EDGE_CURVE('',#4067,#4065,#2189,.T.);
#5146=EDGE_CURVE('',#4069,#4070,#2885,.T.);
#5147=EDGE_CURVE('',#4070,#4068,#2190,.T.);
#5148=EDGE_CURVE('',#4069,#4067,#2191,.T.);
#5149=EDGE_CURVE('',#4071,#4072,#2886,.T.);
#5150=EDGE_CURVE('',#4072,#4070,#2192,.T.);
#5151=EDGE_CURVE('',#4071,#4069,#2193,.T.);
#5152=EDGE_CURVE('',#4073,#4074,#2887,.T.);
#5153=EDGE_CURVE('',#4074,#4072,#2194,.T.);
#5154=EDGE_CURVE('',#4073,#4071,#2195,.T.);
#5155=EDGE_CURVE('',#4075,#4076,#2888,.T.);
#5156=EDGE_CURVE('',#4076,#4074,#2196,.T.);
#5157=EDGE_CURVE('',#4075,#4073,#2197,.T.);
#5158=EDGE_CURVE('',#4077,#4078,#2889,.T.);
#5159=EDGE_CURVE('',#4078,#4076,#2198,.T.);
#5160=EDGE_CURVE('',#4077,#4075,#2199,.T.);
#5161=EDGE_CURVE('',#4079,#4080,#2890,.T.);
#5162=EDGE_CURVE('',#4080,#4078,#2200,.T.);
#5163=EDGE_CURVE('',#4079,#4077,#2201,.T.);
#5164=EDGE_CURVE('',#4081,#4082,#2891,.T.);
#5165=EDGE_CURVE('',#4082,#4080,#2202,.T.);
#5166=EDGE_CURVE('',#4081,#4079,#2203,.T.);
#5167=EDGE_CURVE('',#4083,#4084,#2892,.T.);
#5168=EDGE_CURVE('',#4084,#4082,#2204,.T.);
#5169=EDGE_CURVE('',#4083,#4081,#2205,.T.);
#5170=EDGE_CURVE('',#4085,#4086,#2893,.T.);
#5171=EDGE_CURVE('',#4086,#4084,#2206,.T.);
#5172=EDGE_CURVE('',#4085,#4083,#2207,.T.);
#5173=EDGE_CURVE('',#4087,#4088,#2894,.T.);
#5174=EDGE_CURVE('',#4089,#4087,#2208,.T.);
#5175=EDGE_CURVE('',#4090,#4089,#1839,.T.);
#5176=EDGE_CURVE('',#4090,#4088,#2209,.T.);
#5177=EDGE_CURVE('',#4091,#4092,#2895,.T.);
#5178=EDGE_CURVE('',#4092,#4093,#2210,.T.);
#5179=EDGE_CURVE('',#4093,#4094,#1840,.T.);
#5180=EDGE_CURVE('',#4094,#4095,#2211,.T.);
#5181=EDGE_CURVE('',#4095,#4096,#2896,.T.);
#5182=EDGE_CURVE('',#4096,#4096,#1841,.F.);
#5183=EDGE_CURVE('',#4095,#4091,#2212,.T.);
#5184=EDGE_CURVE('',#4097,#4098,#2897,.T.);
#5185=EDGE_CURVE('',#4098,#4092,#2213,.T.);
#5186=EDGE_CURVE('',#4091,#4097,#2214,.T.);
#5187=EDGE_CURVE('',#4099,#4100,#2898,.T.);
#5188=EDGE_CURVE('',#4100,#4098,#2215,.T.);
#5189=EDGE_CURVE('',#4097,#4099,#2216,.T.);
#5190=EDGE_CURVE('',#4101,#4102,#2899,.T.);
#5191=EDGE_CURVE('',#4102,#4100,#2217,.T.);
#5192=EDGE_CURVE('',#4099,#4101,#2218,.T.);
#5193=EDGE_CURVE('',#4103,#4104,#2900,.T.);
#5194=EDGE_CURVE('',#4104,#4102,#2219,.T.);
#5195=EDGE_CURVE('',#4101,#4103,#2220,.T.);
#5196=EDGE_CURVE('',#4105,#4106,#2901,.T.);
#5197=EDGE_CURVE('',#4106,#4104,#2221,.T.);
#5198=EDGE_CURVE('',#4103,#4105,#2222,.T.);
#5199=EDGE_CURVE('',#4107,#4108,#2902,.T.);
#5200=EDGE_CURVE('',#4108,#4106,#2223,.T.);
#5201=EDGE_CURVE('',#4105,#4107,#2224,.T.);
#5202=EDGE_CURVE('',#4109,#4110,#2903,.T.);
#5203=EDGE_CURVE('',#4110,#4108,#2225,.T.);
#5204=EDGE_CURVE('',#4107,#4109,#2226,.T.);
#5205=EDGE_CURVE('',#4111,#4112,#2904,.T.);
#5206=EDGE_CURVE('',#4112,#4110,#2227,.T.);
#5207=EDGE_CURVE('',#4109,#4111,#2228,.T.);
#5208=EDGE_CURVE('',#4113,#4114,#2905,.T.);
#5209=EDGE_CURVE('',#4114,#4112,#2229,.T.);
#5210=EDGE_CURVE('',#4111,#4113,#2230,.T.);
#5211=EDGE_CURVE('',#4115,#4116,#2906,.T.);
#5212=EDGE_CURVE('',#4116,#4114,#2231,.T.);
#5213=EDGE_CURVE('',#4113,#4115,#2232,.T.);
#5214=EDGE_CURVE('',#4117,#4118,#2907,.T.);
#5215=EDGE_CURVE('',#4118,#4116,#2233,.T.);
#5216=EDGE_CURVE('',#4115,#4117,#2234,.T.);
#5217=EDGE_CURVE('',#4119,#4120,#2908,.T.);
#5218=EDGE_CURVE('',#4120,#4118,#2235,.T.);
#5219=EDGE_CURVE('',#4117,#4119,#2236,.T.);
#5220=EDGE_CURVE('',#4121,#4122,#2909,.T.);
#5221=EDGE_CURVE('',#4122,#4120,#2237,.T.);
#5222=EDGE_CURVE('',#4119,#4121,#2238,.T.);
#5223=EDGE_CURVE('',#4123,#4124,#2910,.T.);
#5224=EDGE_CURVE('',#4123,#4125,#2239,.T.);
#5225=EDGE_CURVE('',#4126,#4125,#1842,.T.);
#5226=EDGE_CURVE('',#4126,#4124,#2240,.T.);
#5227=EDGE_CURVE('',#4127,#4128,#2911,.T.);
#5228=EDGE_CURVE('',#4128,#4129,#2241,.T.);
#5229=EDGE_CURVE('',#4130,#4129,#1843,.T.);
#5230=EDGE_CURVE('',#4127,#4130,#2242,.T.);
#5231=EDGE_CURVE('',#4131,#4132,#2912,.T.);
#5232=EDGE_CURVE('',#4132,#4128,#2243,.T.);
#5233=EDGE_CURVE('',#4131,#4127,#2244,.T.);
#5234=EDGE_CURVE('',#4133,#4134,#2913,.T.);
#5235=EDGE_CURVE('',#4134,#4132,#2245,.T.);
#5236=EDGE_CURVE('',#4133,#4131,#2246,.T.);
#5237=EDGE_CURVE('',#4135,#4136,#2914,.T.);
#5238=EDGE_CURVE('',#4136,#4134,#2247,.T.);
#5239=EDGE_CURVE('',#4135,#4133,#2248,.T.);
#5240=EDGE_CURVE('',#4137,#4138,#2915,.T.);
#5241=EDGE_CURVE('',#4138,#4136,#2249,.T.);
#5242=EDGE_CURVE('',#4137,#4135,#2250,.T.);
#5243=EDGE_CURVE('',#4139,#4140,#2916,.T.);
#5244=EDGE_CURVE('',#4140,#4138,#2251,.T.);
#5245=EDGE_CURVE('',#4139,#4137,#2252,.T.);
#5246=EDGE_CURVE('',#4141,#4142,#2917,.T.);
#5247=EDGE_CURVE('',#4142,#4140,#2253,.T.);
#5248=EDGE_CURVE('',#4141,#4139,#2254,.T.);
#5249=EDGE_CURVE('',#4143,#4144,#2918,.T.);
#5250=EDGE_CURVE('',#4144,#4142,#2255,.T.);
#5251=EDGE_CURVE('',#4143,#4141,#2256,.T.);
#5252=EDGE_CURVE('',#4145,#4146,#2919,.T.);
#5253=EDGE_CURVE('',#4146,#4144,#2257,.T.);
#5254=EDGE_CURVE('',#4145,#4143,#2258,.T.);
#5255=EDGE_CURVE('',#4147,#4148,#2920,.T.);
#5256=EDGE_CURVE('',#4148,#4146,#2259,.T.);
#5257=EDGE_CURVE('',#4147,#4145,#2260,.T.);
#5258=EDGE_CURVE('',#4149,#4150,#2921,.T.);
#5259=EDGE_CURVE('',#4150,#4148,#2261,.T.);
#5260=EDGE_CURVE('',#4149,#4147,#2262,.T.);
#5261=EDGE_CURVE('',#4151,#4152,#2922,.T.);
#5262=EDGE_CURVE('',#4152,#4150,#2263,.T.);
#5263=EDGE_CURVE('',#4151,#4149,#2264,.T.);
#5264=EDGE_CURVE('',#4153,#4154,#2923,.T.);
#5265=EDGE_CURVE('',#4154,#4152,#2265,.T.);
#5266=EDGE_CURVE('',#4153,#4151,#2266,.T.);
#5267=EDGE_CURVE('',#4155,#4156,#2924,.T.);
#5268=EDGE_CURVE('',#4156,#4154,#2267,.T.);
#5269=EDGE_CURVE('',#4155,#4153,#2268,.T.);
#5270=EDGE_CURVE('',#4157,#4158,#2925,.T.);
#5271=EDGE_CURVE('',#4158,#4156,#2269,.T.);
#5272=EDGE_CURVE('',#4157,#4155,#2270,.T.);
#5273=EDGE_CURVE('',#4159,#4160,#2926,.T.);
#5274=EDGE_CURVE('',#4161,#4159,#2271,.T.);
#5275=EDGE_CURVE('',#4162,#4161,#1844,.T.);
#5276=EDGE_CURVE('',#4162,#4160,#2272,.T.);
#5277=EDGE_CURVE('',#4163,#4164,#2927,.T.);
#5278=EDGE_CURVE('',#4164,#4165,#2273,.T.);
#5279=EDGE_CURVE('',#4165,#4166,#1845,.T.);
#5280=EDGE_CURVE('',#4167,#4166,#2274,.F.);
#5281=EDGE_CURVE('',#4167,#4168,#1846,.T.);
#5282=EDGE_CURVE('',#4168,#4163,#2275,.T.);
#5283=EDGE_CURVE('',#4169,#4170,#2928,.T.);
#5284=EDGE_CURVE('',#4170,#4164,#2276,.T.);
#5285=EDGE_CURVE('',#4163,#4169,#2277,.T.);
#5286=EDGE_CURVE('',#4171,#4172,#2929,.T.);
#5287=EDGE_CURVE('',#4172,#4170,#2278,.T.);
#5288=EDGE_CURVE('',#4169,#4171,#2279,.T.);
#5289=EDGE_CURVE('',#4173,#4174,#2930,.T.);
#5290=EDGE_CURVE('',#4174,#4172,#2280,.T.);
#5291=EDGE_CURVE('',#4171,#4173,#2281,.T.);
#5292=EDGE_CURVE('',#4175,#4176,#2931,.T.);
#5293=EDGE_CURVE('',#4176,#4174,#2282,.T.);
#5294=EDGE_CURVE('',#4173,#4175,#2283,.T.);
#5295=EDGE_CURVE('',#4177,#4178,#2932,.T.);
#5296=EDGE_CURVE('',#4178,#4176,#2284,.T.);
#5297=EDGE_CURVE('',#4175,#4177,#2285,.T.);
#5298=EDGE_CURVE('',#4179,#4180,#2933,.T.);
#5299=EDGE_CURVE('',#4180,#4178,#2286,.T.);
#5300=EDGE_CURVE('',#4177,#4179,#2287,.T.);
#5301=EDGE_CURVE('',#4181,#4182,#2934,.T.);
#5302=EDGE_CURVE('',#4182,#4180,#2288,.T.);
#5303=EDGE_CURVE('',#4179,#4181,#2289,.T.);
#5304=EDGE_CURVE('',#4183,#4184,#2935,.T.);
#5305=EDGE_CURVE('',#4184,#4182,#2290,.T.);
#5306=EDGE_CURVE('',#4181,#4183,#2291,.T.);
#5307=EDGE_CURVE('',#4185,#4186,#2936,.T.);
#5308=EDGE_CURVE('',#4186,#4184,#2292,.T.);
#5309=EDGE_CURVE('',#4183,#4185,#2293,.T.);
#5310=EDGE_CURVE('',#4187,#4188,#2937,.T.);
#5311=EDGE_CURVE('',#4188,#4186,#2294,.T.);
#5312=EDGE_CURVE('',#4185,#4187,#2295,.T.);
#5313=EDGE_CURVE('',#4189,#4190,#2938,.T.);
#5314=EDGE_CURVE('',#4190,#4188,#2296,.T.);
#5315=EDGE_CURVE('',#4187,#4189,#2297,.T.);
#5316=EDGE_CURVE('',#4191,#4192,#2939,.T.);
#5317=EDGE_CURVE('',#4192,#4190,#2298,.T.);
#5318=EDGE_CURVE('',#4189,#4191,#2299,.T.);
#5319=EDGE_CURVE('',#4193,#4194,#2940,.T.);
#5320=EDGE_CURVE('',#4194,#4192,#2300,.T.);
#5321=EDGE_CURVE('',#4191,#4193,#2301,.T.);
#5322=EDGE_CURVE('',#4195,#4196,#2941,.T.);
#5323=EDGE_CURVE('',#4195,#4197,#2302,.T.);
#5324=EDGE_CURVE('',#4198,#4197,#1847,.F.);
#5325=EDGE_CURVE('',#4198,#4196,#2303,.T.);
#5326=EDGE_CURVE('',#4199,#4200,#2942,.T.);
#5327=EDGE_CURVE('',#4200,#4201,#2304,.T.);
#5328=EDGE_CURVE('',#4201,#4202,#1848,.T.);
#5329=EDGE_CURVE('',#4203,#4202,#2305,.F.);
#5330=EDGE_CURVE('',#4203,#4204,#1849,.T.);
#5331=EDGE_CURVE('',#4204,#4199,#2306,.T.);
#5332=EDGE_CURVE('',#4205,#4206,#2943,.T.);
#5333=EDGE_CURVE('',#4206,#4200,#2307,.T.);
#5334=EDGE_CURVE('',#4199,#4205,#2308,.T.);
#5335=EDGE_CURVE('',#4207,#4208,#2944,.T.);
#5336=EDGE_CURVE('',#4208,#4206,#2309,.T.);
#5337=EDGE_CURVE('',#4205,#4207,#2310,.T.);
#5338=EDGE_CURVE('',#4209,#4210,#2945,.T.);
#5339=EDGE_CURVE('',#4210,#4208,#2311,.T.);
#5340=EDGE_CURVE('',#4207,#4209,#2312,.T.);
#5341=EDGE_CURVE('',#4211,#4212,#2946,.T.);
#5342=EDGE_CURVE('',#4212,#4210,#2313,.T.);
#5343=EDGE_CURVE('',#4209,#4211,#2314,.T.);
#5344=EDGE_CURVE('',#4213,#4214,#2947,.T.);
#5345=EDGE_CURVE('',#4214,#4212,#2315,.T.);
#5346=EDGE_CURVE('',#4211,#4213,#2316,.T.);
#5347=EDGE_CURVE('',#4215,#4216,#2948,.T.);
#5348=EDGE_CURVE('',#4216,#4214,#2317,.T.);
#5349=EDGE_CURVE('',#4213,#4215,#2318,.T.);
#5350=EDGE_CURVE('',#4217,#4218,#2949,.T.);
#5351=EDGE_CURVE('',#4218,#4216,#2319,.T.);
#5352=EDGE_CURVE('',#4215,#4217,#2320,.T.);
#5353=EDGE_CURVE('',#4219,#4220,#2950,.T.);
#5354=EDGE_CURVE('',#4220,#4218,#2321,.T.);
#5355=EDGE_CURVE('',#4217,#4219,#2322,.T.);
#5356=EDGE_CURVE('',#4221,#4222,#2951,.T.);
#5357=EDGE_CURVE('',#4222,#4220,#2323,.T.);
#5358=EDGE_CURVE('',#4219,#4221,#2324,.T.);
#5359=EDGE_CURVE('',#4223,#4224,#2952,.T.);
#5360=EDGE_CURVE('',#4224,#4222,#2325,.T.);
#5361=EDGE_CURVE('',#4221,#4223,#2326,.T.);
#5362=EDGE_CURVE('',#4225,#4226,#2953,.T.);
#5363=EDGE_CURVE('',#4226,#4224,#2327,.T.);
#5364=EDGE_CURVE('',#4223,#4225,#2328,.T.);
#5365=EDGE_CURVE('',#4227,#4228,#2954,.T.);
#5366=EDGE_CURVE('',#4228,#4226,#2329,.T.);
#5367=EDGE_CURVE('',#4225,#4227,#2330,.T.);
#5368=EDGE_CURVE('',#4229,#4230,#2955,.T.);
#5369=EDGE_CURVE('',#4230,#4228,#2331,.T.);
#5370=EDGE_CURVE('',#4227,#4229,#2332,.T.);
#5371=EDGE_CURVE('',#4231,#4232,#2956,.T.);
#5372=EDGE_CURVE('',#4231,#4233,#2333,.T.);
#5373=EDGE_CURVE('',#4234,#4233,#1850,.F.);
#5374=EDGE_CURVE('',#4234,#4232,#2334,.T.);
#5375=EDGE_CURVE('',#4235,#4236,#2957,.T.);
#5376=EDGE_CURVE('',#4236,#4237,#2335,.T.);
#5377=EDGE_CURVE('',#4238,#4237,#1851,.T.);
#5378=EDGE_CURVE('',#4235,#4238,#2336,.T.);
#5379=EDGE_CURVE('',#4239,#4240,#2958,.T.);
#5380=EDGE_CURVE('',#4240,#4236,#2337,.T.);
#5381=EDGE_CURVE('',#4239,#4235,#2338,.T.);
#5382=EDGE_CURVE('',#4241,#4242,#2959,.T.);
#5383=EDGE_CURVE('',#4242,#4240,#2339,.T.);
#5384=EDGE_CURVE('',#4241,#4239,#2340,.T.);
#5385=EDGE_CURVE('',#4243,#4244,#2960,.T.);
#5386=EDGE_CURVE('',#4244,#4242,#2341,.T.);
#5387=EDGE_CURVE('',#4243,#4241,#2342,.T.);
#5388=EDGE_CURVE('',#4245,#4246,#2961,.T.);
#5389=EDGE_CURVE('',#4246,#4244,#2343,.T.);
#5390=EDGE_CURVE('',#4245,#4243,#2344,.T.);
#5391=EDGE_CURVE('',#4247,#4248,#2962,.T.);
#5392=EDGE_CURVE('',#4248,#4246,#2345,.T.);
#5393=EDGE_CURVE('',#4247,#4245,#2346,.T.);
#5394=EDGE_CURVE('',#4249,#4250,#2963,.T.);
#5395=EDGE_CURVE('',#4250,#4248,#2347,.T.);
#5396=EDGE_CURVE('',#4249,#4247,#2348,.T.);
#5397=EDGE_CURVE('',#4251,#4252,#2964,.T.);
#5398=EDGE_CURVE('',#4252,#4250,#2349,.T.);
#5399=EDGE_CURVE('',#4251,#4249,#2350,.T.);
#5400=EDGE_CURVE('',#4253,#4254,#2965,.T.);
#5401=EDGE_CURVE('',#4254,#4252,#2351,.T.);
#5402=EDGE_CURVE('',#4253,#4251,#2352,.T.);
#5403=EDGE_CURVE('',#4255,#4256,#2966,.T.);
#5404=EDGE_CURVE('',#4256,#4254,#2353,.T.);
#5405=EDGE_CURVE('',#4255,#4253,#2354,.T.);
#5406=EDGE_CURVE('',#4257,#4258,#2967,.T.);
#5407=EDGE_CURVE('',#4258,#4256,#2355,.T.);
#5408=EDGE_CURVE('',#4257,#4255,#2356,.T.);
#5409=EDGE_CURVE('',#4259,#4260,#2968,.T.);
#5410=EDGE_CURVE('',#4260,#4258,#2357,.T.);
#5411=EDGE_CURVE('',#4259,#4257,#2358,.T.);
#5412=EDGE_CURVE('',#4261,#4262,#2969,.T.);
#5413=EDGE_CURVE('',#4262,#4260,#2359,.T.);
#5414=EDGE_CURVE('',#4261,#4259,#2360,.T.);
#5415=EDGE_CURVE('',#4263,#4264,#2970,.T.);
#5416=EDGE_CURVE('',#4264,#4262,#2361,.T.);
#5417=EDGE_CURVE('',#4263,#4261,#2362,.T.);
#5418=EDGE_CURVE('',#4265,#4266,#2971,.T.);
#5419=EDGE_CURVE('',#4267,#4265,#2363,.T.);
#5420=EDGE_CURVE('',#4268,#4267,#1852,.T.);
#5421=EDGE_CURVE('',#4268,#4266,#2364,.T.);
#5422=EDGE_CURVE('',#4269,#4270,#2972,.T.);
#5423=EDGE_CURVE('',#4270,#4271,#2365,.T.);
#5424=EDGE_CURVE('',#4272,#4271,#1853,.T.);
#5425=EDGE_CURVE('',#4269,#4272,#2366,.T.);
#5426=EDGE_CURVE('',#4273,#4274,#2973,.T.);
#5427=EDGE_CURVE('',#4274,#4270,#2367,.T.);
#5428=EDGE_CURVE('',#4273,#4269,#2368,.T.);
#5429=EDGE_CURVE('',#4275,#4276,#2974,.T.);
#5430=EDGE_CURVE('',#4276,#4274,#2369,.T.);
#5431=EDGE_CURVE('',#4275,#4273,#2370,.T.);
#5432=EDGE_CURVE('',#4277,#4278,#2975,.T.);
#5433=EDGE_CURVE('',#4278,#4276,#2371,.T.);
#5434=EDGE_CURVE('',#4277,#4275,#2372,.T.);
#5435=EDGE_CURVE('',#4279,#4280,#2976,.T.);
#5436=EDGE_CURVE('',#4280,#4278,#2373,.T.);
#5437=EDGE_CURVE('',#4279,#4277,#2374,.T.);
#5438=EDGE_CURVE('',#4281,#4282,#2977,.T.);
#5439=EDGE_CURVE('',#4282,#4280,#2375,.T.);
#5440=EDGE_CURVE('',#4281,#4279,#2376,.T.);
#5441=EDGE_CURVE('',#4283,#4284,#2978,.T.);
#5442=EDGE_CURVE('',#4284,#4282,#2377,.T.);
#5443=EDGE_CURVE('',#4283,#4281,#2378,.T.);
#5444=EDGE_CURVE('',#4285,#4286,#2979,.T.);
#5445=EDGE_CURVE('',#4286,#4284,#2379,.T.);
#5446=EDGE_CURVE('',#4285,#4283,#2380,.T.);
#5447=EDGE_CURVE('',#4287,#4288,#2980,.T.);
#5448=EDGE_CURVE('',#4288,#4286,#2381,.T.);
#5449=EDGE_CURVE('',#4287,#4285,#2382,.T.);
#5450=EDGE_CURVE('',#4289,#4290,#2981,.T.);
#5451=EDGE_CURVE('',#4290,#4288,#2383,.T.);
#5452=EDGE_CURVE('',#4289,#4287,#2384,.T.);
#5453=EDGE_CURVE('',#4291,#4292,#2982,.T.);
#5454=EDGE_CURVE('',#4292,#4290,#2385,.T.);
#5455=EDGE_CURVE('',#4291,#4289,#2386,.T.);
#5456=EDGE_CURVE('',#4293,#4294,#2983,.T.);
#5457=EDGE_CURVE('',#4294,#4292,#2387,.T.);
#5458=EDGE_CURVE('',#4293,#4291,#2388,.T.);
#5459=EDGE_CURVE('',#4295,#4296,#2984,.T.);
#5460=EDGE_CURVE('',#4296,#4294,#2389,.T.);
#5461=EDGE_CURVE('',#4295,#4293,#2390,.T.);
#5462=EDGE_CURVE('',#4297,#4298,#2985,.T.);
#5463=EDGE_CURVE('',#4298,#4296,#2391,.T.);
#5464=EDGE_CURVE('',#4297,#4295,#2392,.T.);
#5465=EDGE_CURVE('',#4299,#4300,#2986,.T.);
#5466=EDGE_CURVE('',#4301,#4299,#2393,.T.);
#5467=EDGE_CURVE('',#4302,#4301,#1854,.T.);
#5468=EDGE_CURVE('',#4302,#4300,#2394,.T.);
#5469=EDGE_CURVE('',#4303,#4304,#2987,.T.);
#5470=EDGE_CURVE('',#4304,#4305,#2395,.T.);
#5471=EDGE_CURVE('',#4305,#4306,#1855,.T.);
#5472=EDGE_CURVE('',#4306,#4307,#2988,.T.);
#5473=EDGE_CURVE('',#4307,#4307,#1856,.F.);
#5474=EDGE_CURVE('',#4306,#4308,#1857,.T.);
#5475=EDGE_CURVE('',#4308,#4303,#2396,.T.);
#5476=EDGE_CURVE('',#4309,#4310,#2989,.T.);
#5477=EDGE_CURVE('',#4310,#4304,#2397,.T.);
#5478=EDGE_CURVE('',#4303,#4309,#2398,.T.);
#5479=EDGE_CURVE('',#4311,#4312,#2990,.T.);
#5480=EDGE_CURVE('',#4312,#4310,#2399,.T.);
#5481=EDGE_CURVE('',#4309,#4311,#2400,.T.);
#5482=EDGE_CURVE('',#4313,#4314,#2991,.T.);
#5483=EDGE_CURVE('',#4314,#4312,#2401,.T.);
#5484=EDGE_CURVE('',#4311,#4313,#2402,.T.);
#5485=EDGE_CURVE('',#4315,#4316,#2992,.T.);
#5486=EDGE_CURVE('',#4316,#4314,#2403,.T.);
#5487=EDGE_CURVE('',#4313,#4315,#2404,.T.);
#5488=EDGE_CURVE('',#4317,#4318,#2993,.T.);
#5489=EDGE_CURVE('',#4318,#4316,#2405,.T.);
#5490=EDGE_CURVE('',#4315,#4317,#2406,.T.);
#5491=EDGE_CURVE('',#4319,#4320,#2994,.T.);
#5492=EDGE_CURVE('',#4320,#4318,#2407,.T.);
#5493=EDGE_CURVE('',#4317,#4319,#2408,.T.);
#5494=EDGE_CURVE('',#4321,#4322,#2995,.T.);
#5495=EDGE_CURVE('',#4322,#4320,#2409,.T.);
#5496=EDGE_CURVE('',#4319,#4321,#2410,.T.);
#5497=EDGE_CURVE('',#4323,#4324,#2996,.T.);
#5498=EDGE_CURVE('',#4324,#4322,#2411,.T.);
#5499=EDGE_CURVE('',#4321,#4323,#2412,.T.);
#5500=EDGE_CURVE('',#4325,#4326,#2997,.T.);
#5501=EDGE_CURVE('',#4326,#4324,#2413,.T.);
#5502=EDGE_CURVE('',#4323,#4325,#2414,.T.);
#5503=EDGE_CURVE('',#4327,#4328,#2998,.T.);
#5504=EDGE_CURVE('',#4328,#4326,#2415,.T.);
#5505=EDGE_CURVE('',#4325,#4327,#2416,.T.);
#5506=EDGE_CURVE('',#4329,#4330,#2999,.T.);
#5507=EDGE_CURVE('',#4330,#4328,#2417,.T.);
#5508=EDGE_CURVE('',#4327,#4329,#2418,.T.);
#5509=EDGE_CURVE('',#4331,#4332,#3000,.T.);
#5510=EDGE_CURVE('',#4332,#4330,#2419,.T.);
#5511=EDGE_CURVE('',#4329,#4331,#2420,.T.);
#5512=EDGE_CURVE('',#4333,#4334,#3001,.T.);
#5513=EDGE_CURVE('',#4334,#4332,#2421,.T.);
#5514=EDGE_CURVE('',#4331,#4333,#2422,.T.);
#5515=EDGE_CURVE('',#4335,#4336,#3002,.T.);
#5516=EDGE_CURVE('',#4335,#4337,#2423,.T.);
#5517=EDGE_CURVE('',#4338,#4337,#1858,.F.);
#5518=EDGE_CURVE('',#4338,#4336,#2424,.T.);
#5519=EDGE_CURVE('',#4339,#4340,#3003,.T.);
#5520=EDGE_CURVE('',#4340,#4341,#2425,.T.);
#5521=EDGE_CURVE('',#4342,#4341,#1859,.T.);
#5522=EDGE_CURVE('',#4339,#4342,#2426,.T.);
#5523=EDGE_CURVE('',#4343,#4344,#3004,.T.);
#5524=EDGE_CURVE('',#4344,#4340,#2427,.T.);
#5525=EDGE_CURVE('',#4343,#4339,#2428,.T.);
#5526=EDGE_CURVE('',#4345,#4346,#3005,.T.);
#5527=EDGE_CURVE('',#4346,#4344,#2429,.T.);
#5528=EDGE_CURVE('',#4345,#4343,#2430,.T.);
#5529=EDGE_CURVE('',#4347,#4348,#3006,.T.);
#5530=EDGE_CURVE('',#4348,#4346,#2431,.T.);
#5531=EDGE_CURVE('',#4347,#4345,#2432,.T.);
#5532=EDGE_CURVE('',#4349,#4350,#3007,.T.);
#5533=EDGE_CURVE('',#4350,#4348,#2433,.T.);
#5534=EDGE_CURVE('',#4349,#4347,#2434,.T.);
#5535=EDGE_CURVE('',#4351,#4352,#3008,.T.);
#5536=EDGE_CURVE('',#4352,#4350,#2435,.T.);
#5537=EDGE_CURVE('',#4351,#4349,#2436,.T.);
#5538=EDGE_CURVE('',#4353,#4354,#3009,.T.);
#5539=EDGE_CURVE('',#4354,#4352,#2437,.T.);
#5540=EDGE_CURVE('',#4353,#4351,#2438,.T.);
#5541=EDGE_CURVE('',#4355,#4356,#3010,.T.);
#5542=EDGE_CURVE('',#4356,#4354,#2439,.T.);
#5543=EDGE_CURVE('',#4355,#4353,#2440,.T.);
#5544=EDGE_CURVE('',#4357,#4358,#3011,.T.);
#5545=EDGE_CURVE('',#4358,#4356,#2441,.T.);
#5546=EDGE_CURVE('',#4357,#4355,#2442,.T.);
#5547=EDGE_CURVE('',#4359,#4360,#3012,.T.);
#5548=EDGE_CURVE('',#4360,#4358,#2443,.T.);
#5549=EDGE_CURVE('',#4359,#4357,#2444,.T.);
#5550=EDGE_CURVE('',#4361,#4362,#3013,.T.);
#5551=EDGE_CURVE('',#4362,#4360,#2445,.T.);
#5552=EDGE_CURVE('',#4361,#4359,#2446,.T.);
#5553=EDGE_CURVE('',#4363,#4364,#3014,.T.);
#5554=EDGE_CURVE('',#4364,#4362,#2447,.T.);
#5555=EDGE_CURVE('',#4363,#4361,#2448,.T.);
#5556=EDGE_CURVE('',#4365,#4366,#3015,.T.);
#5557=EDGE_CURVE('',#4366,#4364,#2449,.T.);
#5558=EDGE_CURVE('',#4365,#4363,#2450,.T.);
#5559=EDGE_CURVE('',#4367,#4368,#3016,.T.);
#5560=EDGE_CURVE('',#4368,#4366,#2451,.T.);
#5561=EDGE_CURVE('',#4367,#4365,#2452,.T.);
#5562=EDGE_CURVE('',#4369,#4370,#3017,.T.);
#5563=EDGE_CURVE('',#4371,#4369,#2453,.T.);
#5564=EDGE_CURVE('',#4372,#4371,#1860,.T.);
#5565=EDGE_CURVE('',#4372,#4370,#2454,.T.);
#5566=EDGE_CURVE('',#4373,#4374,#3018,.T.);
#5567=EDGE_CURVE('',#4374,#4375,#2455,.T.);
#5568=EDGE_CURVE('',#4375,#4376,#1861,.T.);
#5569=EDGE_CURVE('',#4376,#4377,#3019,.T.);
#5570=EDGE_CURVE('',#4377,#4377,#1862,.F.);
#5571=EDGE_CURVE('',#4376,#4378,#1863,.T.);
#5572=EDGE_CURVE('',#4378,#4373,#2456,.T.);
#5573=EDGE_CURVE('',#4379,#4380,#3020,.T.);
#5574=EDGE_CURVE('',#4380,#4374,#2457,.T.);
#5575=EDGE_CURVE('',#4373,#4379,#2458,.T.);
#5576=EDGE_CURVE('',#4381,#4382,#3021,.T.);
#5577=EDGE_CURVE('',#4382,#4380,#2459,.T.);
#5578=EDGE_CURVE('',#4379,#4381,#2460,.T.);
#5579=EDGE_CURVE('',#4383,#4384,#3022,.T.);
#5580=EDGE_CURVE('',#4384,#4382,#2461,.T.);
#5581=EDGE_CURVE('',#4381,#4383,#2462,.T.);
#5582=EDGE_CURVE('',#4385,#4386,#3023,.T.);
#5583=EDGE_CURVE('',#4386,#4384,#2463,.T.);
#5584=EDGE_CURVE('',#4383,#4385,#2464,.T.);
#5585=EDGE_CURVE('',#4387,#4388,#3024,.T.);
#5586=EDGE_CURVE('',#4388,#4386,#2465,.T.);
#5587=EDGE_CURVE('',#4385,#4387,#2466,.T.);
#5588=EDGE_CURVE('',#4389,#4390,#3025,.T.);
#5589=EDGE_CURVE('',#4390,#4388,#2467,.T.);
#5590=EDGE_CURVE('',#4387,#4389,#2468,.T.);
#5591=EDGE_CURVE('',#4391,#4392,#3026,.T.);
#5592=EDGE_CURVE('',#4392,#4390,#2469,.T.);
#5593=EDGE_CURVE('',#4389,#4391,#2470,.T.);
#5594=EDGE_CURVE('',#4393,#4394,#3027,.T.);
#5595=EDGE_CURVE('',#4394,#4392,#2471,.T.);
#5596=EDGE_CURVE('',#4391,#4393,#2472,.T.);
#5597=EDGE_CURVE('',#4395,#4396,#3028,.T.);
#5598=EDGE_CURVE('',#4396,#4394,#2473,.T.);
#5599=EDGE_CURVE('',#4393,#4395,#2474,.T.);
#5600=EDGE_CURVE('',#4397,#4398,#3029,.T.);
#5601=EDGE_CURVE('',#4398,#4396,#2475,.T.);
#5602=EDGE_CURVE('',#4395,#4397,#2476,.T.);
#5603=EDGE_CURVE('',#4399,#4400,#3030,.T.);
#5604=EDGE_CURVE('',#4400,#4398,#2477,.T.);
#5605=EDGE_CURVE('',#4397,#4399,#2478,.T.);
#5606=EDGE_CURVE('',#4401,#4402,#3031,.T.);
#5607=EDGE_CURVE('',#4402,#4400,#2479,.T.);
#5608=EDGE_CURVE('',#4399,#4401,#2480,.T.);
#5609=EDGE_CURVE('',#4403,#4404,#3032,.T.);
#5610=EDGE_CURVE('',#4404,#4402,#2481,.T.);
#5611=EDGE_CURVE('',#4401,#4403,#2482,.T.);
#5612=EDGE_CURVE('',#4405,#4406,#3033,.T.);
#5613=EDGE_CURVE('',#4405,#4407,#2483,.T.);
#5614=EDGE_CURVE('',#4408,#4407,#1864,.F.);
#5615=EDGE_CURVE('',#4408,#4406,#2484,.T.);
#5616=EDGE_CURVE('',#4409,#4410,#3034,.T.);
#5617=EDGE_CURVE('',#4410,#4411,#2485,.T.);
#5618=EDGE_CURVE('',#4412,#4411,#1865,.T.);
#5619=EDGE_CURVE('',#4409,#4412,#2486,.T.);
#5620=EDGE_CURVE('',#4413,#4414,#3035,.T.);
#5621=EDGE_CURVE('',#4414,#4410,#2487,.T.);
#5622=EDGE_CURVE('',#4413,#4409,#2488,.T.);
#5623=EDGE_CURVE('',#4415,#4416,#3036,.T.);
#5624=EDGE_CURVE('',#4416,#4414,#2489,.T.);
#5625=EDGE_CURVE('',#4415,#4413,#2490,.T.);
#5626=EDGE_CURVE('',#4417,#4418,#3037,.T.);
#5627=EDGE_CURVE('',#4418,#4416,#2491,.T.);
#5628=EDGE_CURVE('',#4417,#4415,#2492,.T.);
#5629=EDGE_CURVE('',#4419,#4420,#3038,.T.);
#5630=EDGE_CURVE('',#4420,#4418,#2493,.T.);
#5631=EDGE_CURVE('',#4419,#4417,#2494,.T.);
#5632=EDGE_CURVE('',#4421,#4422,#3039,.T.);
#5633=EDGE_CURVE('',#4422,#4420,#2495,.T.);
#5634=EDGE_CURVE('',#4421,#4419,#2496,.T.);
#5635=EDGE_CURVE('',#4423,#4424,#3040,.T.);
#5636=EDGE_CURVE('',#4424,#4422,#2497,.T.);
#5637=EDGE_CURVE('',#4423,#4421,#2498,.T.);
#5638=EDGE_CURVE('',#4425,#4426,#3041,.T.);
#5639=EDGE_CURVE('',#4426,#4424,#2499,.T.);
#5640=EDGE_CURVE('',#4425,#4423,#2500,.T.);
#5641=EDGE_CURVE('',#4427,#4428,#3042,.T.);
#5642=EDGE_CURVE('',#4428,#4426,#2501,.T.);
#5643=EDGE_CURVE('',#4427,#4425,#2502,.T.);
#5644=EDGE_CURVE('',#4429,#4430,#3043,.T.);
#5645=EDGE_CURVE('',#4430,#4428,#2503,.T.);
#5646=EDGE_CURVE('',#4429,#4427,#2504,.T.);
#5647=EDGE_CURVE('',#4431,#4432,#3044,.T.);
#5648=EDGE_CURVE('',#4432,#4430,#2505,.T.);
#5649=EDGE_CURVE('',#4431,#4429,#2506,.T.);
#5650=EDGE_CURVE('',#4433,#4434,#3045,.T.);
#5651=EDGE_CURVE('',#4434,#4432,#2507,.T.);
#5652=EDGE_CURVE('',#4433,#4431,#2508,.T.);
#5653=EDGE_CURVE('',#4435,#4436,#3046,.T.);
#5654=EDGE_CURVE('',#4436,#4434,#2509,.T.);
#5655=EDGE_CURVE('',#4435,#4433,#2510,.T.);
#5656=EDGE_CURVE('',#4437,#4438,#3047,.T.);
#5657=EDGE_CURVE('',#4438,#4436,#2511,.T.);
#5658=EDGE_CURVE('',#4437,#4435,#2512,.T.);
#5659=EDGE_CURVE('',#4439,#4440,#3048,.T.);
#5660=EDGE_CURVE('',#4441,#4439,#2513,.T.);
#5661=EDGE_CURVE('',#4442,#4441,#1866,.T.);
#5662=EDGE_CURVE('',#4442,#4440,#2514,.T.);
#5663=EDGE_CURVE('',#4443,#4444,#3049,.T.);
#5664=EDGE_CURVE('',#4444,#4445,#2515,.T.);
#5665=EDGE_CURVE('',#4445,#4446,#1867,.F.);
#5666=EDGE_CURVE('',#4446,#4443,#2516,.T.);
#5667=EDGE_CURVE('',#4447,#4448,#3050,.T.);
#5668=EDGE_CURVE('',#4448,#4444,#2517,.T.);
#5669=EDGE_CURVE('',#4443,#4447,#2518,.T.);
#5670=EDGE_CURVE('',#4449,#4450,#3051,.T.);
#5671=EDGE_CURVE('',#4450,#4448,#2519,.T.);
#5672=EDGE_CURVE('',#4447,#4449,#2520,.T.);
#5673=EDGE_CURVE('',#4451,#4452,#3052,.T.);
#5674=EDGE_CURVE('',#4452,#4450,#2521,.T.);
#5675=EDGE_CURVE('',#4449,#4451,#2522,.T.);
#5676=EDGE_CURVE('',#4453,#4454,#3053,.T.);
#5677=EDGE_CURVE('',#4454,#4452,#2523,.T.);
#5678=EDGE_CURVE('',#4451,#4453,#2524,.T.);
#5679=EDGE_CURVE('',#4455,#4456,#3054,.T.);
#5680=EDGE_CURVE('',#4456,#4454,#2525,.T.);
#5681=EDGE_CURVE('',#4453,#4455,#2526,.T.);
#5682=EDGE_CURVE('',#4457,#4458,#3055,.T.);
#5683=EDGE_CURVE('',#4458,#4456,#2527,.T.);
#5684=EDGE_CURVE('',#4455,#4457,#2528,.T.);
#5685=EDGE_CURVE('',#4459,#4460,#3056,.T.);
#5686=EDGE_CURVE('',#4459,#4461,#2529,.T.);
#5687=EDGE_CURVE('',#4462,#4461,#1868,.T.);
#5688=EDGE_CURVE('',#4462,#4460,#2530,.T.);
#5689=EDGE_CURVE('',#4463,#4464,#3057,.T.);
#5690=EDGE_CURVE('',#4464,#4465,#2531,.T.);
#5691=EDGE_CURVE('',#4466,#4465,#1869,.T.);
#5692=EDGE_CURVE('',#4463,#4466,#2532,.T.);
#5693=EDGE_CURVE('',#4467,#4468,#3058,.T.);
#5694=EDGE_CURVE('',#4468,#4464,#2533,.T.);
#5695=EDGE_CURVE('',#4467,#4463,#2534,.T.);
#5696=EDGE_CURVE('',#4469,#4470,#3059,.T.);
#5697=EDGE_CURVE('',#4470,#4468,#2535,.T.);
#5698=EDGE_CURVE('',#4469,#4467,#2536,.T.);
#5699=EDGE_CURVE('',#4471,#4472,#3060,.T.);
#5700=EDGE_CURVE('',#4472,#4470,#2537,.T.);
#5701=EDGE_CURVE('',#4471,#4469,#2538,.T.);
#5702=EDGE_CURVE('',#4473,#4474,#3061,.T.);
#5703=EDGE_CURVE('',#4474,#4472,#2539,.T.);
#5704=EDGE_CURVE('',#4473,#4471,#2540,.T.);
#5705=EDGE_CURVE('',#4475,#4476,#3062,.T.);
#5706=EDGE_CURVE('',#4476,#4474,#2541,.T.);
#5707=EDGE_CURVE('',#4475,#4473,#2542,.T.);
#5708=EDGE_CURVE('',#4477,#4478,#3063,.T.);
#5709=EDGE_CURVE('',#4478,#4476,#2543,.T.);
#5710=EDGE_CURVE('',#4477,#4475,#2544,.T.);
#5711=EDGE_CURVE('',#4479,#4480,#3064,.T.);
#5712=EDGE_CURVE('',#4481,#4479,#2545,.T.);
#5713=EDGE_CURVE('',#4482,#4481,#1870,.T.);
#5714=EDGE_CURVE('',#4482,#4480,#2546,.T.);
#5715=EDGE_CURVE('',#4480,#4478,#2547,.T.);
#5716=EDGE_CURVE('',#4479,#4477,#2548,.T.);
#5717=EDGE_CURVE('',#4465,#4462,#2549,.T.);
#5718=EDGE_CURVE('',#4445,#4482,#2550,.T.);
#5719=EDGE_CURVE('',#4460,#4458,#2551,.T.);
#5720=EDGE_CURVE('',#4461,#4466,#2552,.T.);
#5721=EDGE_CURVE('',#4457,#4459,#2553,.T.);
#5722=EDGE_CURVE('',#4481,#4446,#2554,.T.);
#5723=EDGE_CURVE('',#4483,#4483,#1871,.T.);
#5724=EDGE_CURVE('',#4484,#4484,#1872,.T.);
#5725=EDGE_CURVE('',#4484,#4483,#3065,.T.);
#5726=EDGE_CURVE('',#4485,#4486,#3066,.F.);
#5727=EDGE_CURVE('',#4487,#4485,#3067,.F.);
#5728=EDGE_CURVE('',#4488,#4487,#3068,.T.);
#5729=EDGE_CURVE('',#4486,#4488,#3069,.F.);
#5730=EDGE_CURVE('',#4267,#4234,#2555,.T.);
#5731=EDGE_CURVE('',#4233,#4268,#2556,.T.);
#5732=EDGE_CURVE('',#4301,#4198,#2557,.T.);
#5733=EDGE_CURVE('',#4197,#4302,#2558,.T.);
#5734=EDGE_CURVE('',#4371,#4338,#2559,.T.);
#5735=EDGE_CURVE('',#4337,#4372,#2560,.T.);
#5736=EDGE_CURVE('',#4441,#4408,#2561,.T.);
#5737=EDGE_CURVE('',#4407,#4442,#2562,.T.);
#5738=EDGE_CURVE('',#4375,#4412,#2563,.T.);
#5739=EDGE_CURVE('',#4411,#4378,#2564,.T.);
#5740=EDGE_CURVE('',#4440,#4438,#2565,.T.);
#5741=EDGE_CURVE('',#4439,#4437,#2566,.T.);
#5742=EDGE_CURVE('',#4403,#4405,#2567,.T.);
#5743=EDGE_CURVE('',#4406,#4404,#2568,.T.);
#5744=EDGE_CURVE('',#4305,#4342,#2569,.T.);
#5745=EDGE_CURVE('',#4341,#4308,#2570,.T.);
#5746=EDGE_CURVE('',#4370,#4368,#2571,.T.);
#5747=EDGE_CURVE('',#4369,#4367,#2572,.T.);
#5748=EDGE_CURVE('',#4333,#4335,#2573,.T.);
#5749=EDGE_CURVE('',#4336,#4334,#2574,.T.);
#5750=EDGE_CURVE('',#4489,#4167,#3070,.T.);
#5751=EDGE_CURVE('',#4489,#4168,#2575,.T.);
#5752=EDGE_CURVE('',#4166,#4490,#3071,.T.);
#5753=EDGE_CURVE('',#4490,#4272,#2576,.T.);
#5754=EDGE_CURVE('',#4271,#4489,#2577,.T.);
#5755=EDGE_CURVE('',#4489,#4167,#3072,.T.);
#5756=EDGE_CURVE('',#4166,#4167,#1873,.T.);
#5757=EDGE_CURVE('',#4166,#4490,#3073,.T.);
#5758=EDGE_CURVE('',#4165,#4490,#2578,.T.);
#5759=EDGE_CURVE('',#4300,#4298,#2579,.T.);
#5760=EDGE_CURVE('',#4299,#4297,#2580,.T.);
#5761=EDGE_CURVE('',#4193,#4195,#2581,.T.);
#5762=EDGE_CURVE('',#4196,#4194,#2582,.T.);
#5763=EDGE_CURVE('',#4491,#4167,#2583,.F.);
#5764=EDGE_CURVE('',#4166,#4491,#2584,.F.);
#5765=EDGE_CURVE('',#4492,#4203,#3074,.T.);
#5766=EDGE_CURVE('',#4492,#4204,#2585,.T.);
#5767=EDGE_CURVE('',#4202,#4493,#3075,.T.);
#5768=EDGE_CURVE('',#4493,#4238,#2586,.T.);
#5769=EDGE_CURVE('',#4237,#4492,#2587,.T.);
#5770=EDGE_CURVE('',#4492,#4203,#3076,.T.);
#5771=EDGE_CURVE('',#4202,#4203,#1874,.T.);
#5772=EDGE_CURVE('',#4202,#4493,#3077,.T.);
#5773=EDGE_CURVE('',#4201,#4493,#2588,.T.);
#5774=EDGE_CURVE('',#4266,#4264,#2589,.T.);
#5775=EDGE_CURVE('',#4265,#4263,#2590,.T.);
#5776=EDGE_CURVE('',#4229,#4231,#2591,.T.);
#5777=EDGE_CURVE('',#4232,#4230,#2592,.T.);
#5778=EDGE_CURVE('',#4494,#4203,#2593,.F.);
#5779=EDGE_CURVE('',#4202,#4494,#2594,.F.);
#5780=EDGE_CURVE('',#4093,#4130,#2595,.T.);
#5781=EDGE_CURVE('',#4129,#4094,#2596,.T.);
#5782=EDGE_CURVE('',#4160,#4158,#2597,.T.);
#5783=EDGE_CURVE('',#4159,#4157,#2598,.T.);
#5784=EDGE_CURVE('',#4125,#4162,#2599,.T.);
#5785=EDGE_CURVE('',#4121,#4123,#2600,.T.);
#5786=EDGE_CURVE('',#4124,#4122,#2601,.T.);
#5787=EDGE_CURVE('',#4161,#4126,#2602,.T.);
#5788=EDGE_CURVE('',#4021,#4058,#2603,.T.);
#5789=EDGE_CURVE('',#4057,#4022,#2604,.T.);
#5790=EDGE_CURVE('',#4088,#4086,#2605,.T.);
#5791=EDGE_CURVE('',#4087,#4085,#2606,.T.);
#5792=EDGE_CURVE('',#4053,#4090,#2607,.T.);
#5793=EDGE_CURVE('',#4049,#4051,#2608,.T.);
#5794=EDGE_CURVE('',#4052,#4050,#2609,.T.);
#5795=EDGE_CURVE('',#4089,#4054,#2610,.T.);
#5796=EDGE_CURVE('',#3949,#3986,#2611,.T.);
#5797=EDGE_CURVE('',#3985,#3950,#2612,.T.);
#5798=EDGE_CURVE('',#4016,#4014,#2613,.T.);
#5799=EDGE_CURVE('',#4015,#4013,#2614,.T.);
#5800=EDGE_CURVE('',#3981,#4018,#2615,.T.);
#5801=EDGE_CURVE('',#3977,#3979,#2616,.T.);
#5802=EDGE_CURVE('',#3980,#3978,#2617,.T.);
#5803=EDGE_CURVE('',#4017,#3982,#2618,.T.);
#5804=EDGE_CURVE('',#3877,#3914,#2619,.T.);
#5805=EDGE_CURVE('',#3913,#3878,#2620,.T.);
#5806=EDGE_CURVE('',#3944,#3942,#2621,.T.);
#5807=EDGE_CURVE('',#3943,#3941,#2622,.T.);
#5808=EDGE_CURVE('',#3909,#3946,#2623,.T.);
#5809=EDGE_CURVE('',#3905,#3907,#2624,.T.);
#5810=EDGE_CURVE('',#3908,#3906,#2625,.T.);
#5811=EDGE_CURVE('',#3945,#3910,#2626,.T.);
#5812=EDGE_CURVE('',#4495,#4495,#1875,.T.);
#5813=EDGE_CURVE('',#4495,#4496,#3078,.T.);
#5814=EDGE_CURVE('',#4496,#4496,#1876,.T.);
#5815=EDGE_CURVE('',#4497,#4497,#1877,.T.);
#5816=EDGE_CURVE('',#4497,#4498,#3079,.T.);
#5817=EDGE_CURVE('',#4498,#4498,#1878,.T.);
#5818=EDGE_CURVE('',#4499,#4499,#1879,.T.);
#5819=EDGE_CURVE('',#4499,#4500,#3080,.T.);
#5820=EDGE_CURVE('',#4500,#4500,#1880,.T.);
#5821=EDGE_CURVE('',#4501,#4501,#1881,.T.);
#5822=EDGE_CURVE('',#4501,#4502,#3081,.T.);
#5823=EDGE_CURVE('',#4502,#4502,#1882,.T.);
#5824=EDGE_CURVE('',#4503,#4503,#1883,.T.);
#5825=EDGE_CURVE('',#4503,#4504,#3082,.T.);
#5826=EDGE_CURVE('',#4504,#4504,#1884,.T.);
#5827=EDGE_CURVE('',#4505,#4505,#1885,.T.);
#5828=EDGE_CURVE('',#4505,#4506,#3083,.T.);
#5829=EDGE_CURVE('',#4506,#4506,#1886,.T.);
#5830=EDGE_CURVE('',#4507,#4507,#1887,.T.);
#5831=EDGE_CURVE('',#4507,#4508,#3084,.T.);
#5832=EDGE_CURVE('',#4508,#4508,#1888,.T.);
#5833=EDGE_CURVE('',#4509,#4509,#1889,.T.);
#5834=EDGE_CURVE('',#4509,#4510,#3085,.T.);
#5835=EDGE_CURVE('',#4510,#4510,#1890,.T.);
#5836=EDGE_CURVE('',#4511,#4511,#1891,.T.);
#5837=EDGE_CURVE('',#4511,#4493,#3086,.T.);
#5838=EDGE_CURVE('',#4492,#4512,#3087,.T.);
#5839=EDGE_CURVE('',#4512,#4512,#1892,.T.);
#5840=EDGE_CURVE('',#4513,#4513,#1893,.T.);
#5841=EDGE_CURVE('',#4513,#4514,#3088,.T.);
#5842=EDGE_CURVE('',#4514,#4514,#1894,.T.);
#5843=EDGE_CURVE('',#4515,#4515,#1895,.T.);
#5844=EDGE_CURVE('',#4515,#4516,#3089,.T.);
#5845=EDGE_CURVE('',#4516,#4516,#1896,.T.);
#5846=EDGE_CURVE('',#4517,#4517,#1897,.T.);
#5847=EDGE_CURVE('',#4517,#4518,#3090,.T.);
#5848=EDGE_CURVE('',#4518,#4518,#1898,.T.);
#5849=EDGE_CURVE('',#4519,#4519,#1899,.T.);
#5850=EDGE_CURVE('',#4519,#4520,#3091,.T.);
#5851=EDGE_CURVE('',#4520,#4520,#1900,.T.);
#5852=EDGE_CURVE('',#4521,#4521,#1901,.T.);
#5853=EDGE_CURVE('',#4521,#4522,#3092,.T.);
#5854=EDGE_CURVE('',#4522,#4522,#1902,.T.);
#5855=EDGE_CURVE('',#4523,#4523,#1903,.T.);
#5856=EDGE_CURVE('',#4523,#4524,#3093,.T.);
#5857=EDGE_CURVE('',#4524,#4524,#1904,.T.);
#5858=EDGE_CURVE('',#4525,#4525,#1905,.T.);
#5859=EDGE_CURVE('',#4525,#4526,#3094,.T.);
#5860=EDGE_CURVE('',#4526,#4526,#1906,.T.);
#5861=EDGE_CURVE('',#4527,#4527,#1907,.T.);
#5862=EDGE_CURVE('',#4527,#4490,#3095,.T.);
#5863=EDGE_CURVE('',#4489,#4528,#3096,.T.);
#5864=EDGE_CURVE('',#4528,#4528,#1908,.T.);
#5865=EDGE_CURVE('',#4529,#4529,#1909,.T.);
#5866=EDGE_CURVE('',#4529,#4530,#3097,.T.);
#5867=EDGE_CURVE('',#4530,#4530,#1910,.T.);
#5868=EDGE_CURVE('',#4531,#4532,#3098,.T.);
#5869=EDGE_CURVE('',#4531,#4533,#3099,.T.);
#5870=EDGE_CURVE('',#4533,#4534,#3100,.T.);
#5871=EDGE_CURVE('',#4532,#4534,#3101,.T.);
#5872=EDGE_CURVE('',#4535,#4531,#3102,.T.);
#5873=EDGE_CURVE('',#4535,#4536,#3103,.T.);
#5874=EDGE_CURVE('',#4536,#4533,#3104,.T.);
#5875=EDGE_CURVE('',#4537,#4535,#3105,.T.);
#5876=EDGE_CURVE('',#4537,#4538,#3106,.T.);
#5877=EDGE_CURVE('',#4538,#4536,#3107,.T.);
#5878=EDGE_CURVE('',#4532,#4537,#3108,.T.);
#5879=EDGE_CURVE('',#4534,#4538,#3109,.T.);
#5880=EDGE_CURVE('',#4485,#4539,#3110,.T.);
#5881=EDGE_CURVE('',#4540,#4539,#3111,.F.);
#5882=EDGE_CURVE('',#4487,#4540,#3112,.F.);
#5883=EDGE_CURVE('',#4541,#4540,#3113,.T.);
#5884=EDGE_CURVE('',#4488,#4541,#3114,.T.);
#5885=EDGE_CURVE('',#4542,#4541,#3115,.F.);
#5886=EDGE_CURVE('',#4486,#4542,#3116,.F.);
#5887=EDGE_CURVE('',#4539,#4542,#3117,.F.);
#6389=ORIENTED_EDGE('',*,*,#4877,.T.);
#6390=ORIENTED_EDGE('',*,*,#4878,.T.);
#6391=ORIENTED_EDGE('',*,*,#4879,.T.);
#6392=ORIENTED_EDGE('',*,*,#4880,.T.);
#6393=ORIENTED_EDGE('',*,*,#4881,.T.);
#6394=ORIENTED_EDGE('',*,*,#4882,.T.);
#6395=ORIENTED_EDGE('',*,*,#4881,.F.);
#6396=ORIENTED_EDGE('',*,*,#4883,.T.);
#6397=ORIENTED_EDGE('',*,*,#4884,.T.);
#6398=ORIENTED_EDGE('',*,*,#4885,.T.);
#6399=ORIENTED_EDGE('',*,*,#4877,.F.);
#6400=ORIENTED_EDGE('',*,*,#4886,.T.);
#6401=ORIENTED_EDGE('',*,*,#4887,.T.);
#6402=ORIENTED_EDGE('',*,*,#4888,.T.);
#6403=ORIENTED_EDGE('',*,*,#4884,.F.);
#6404=ORIENTED_EDGE('',*,*,#4889,.T.);
#6405=ORIENTED_EDGE('',*,*,#4890,.T.);
#6406=ORIENTED_EDGE('',*,*,#4891,.T.);
#6407=ORIENTED_EDGE('',*,*,#4887,.F.);
#6408=ORIENTED_EDGE('',*,*,#4892,.T.);
#6409=ORIENTED_EDGE('',*,*,#4893,.T.);
#6410=ORIENTED_EDGE('',*,*,#4894,.T.);
#6411=ORIENTED_EDGE('',*,*,#4890,.F.);
#6412=ORIENTED_EDGE('',*,*,#4895,.T.);
#6413=ORIENTED_EDGE('',*,*,#4896,.T.);
#6414=ORIENTED_EDGE('',*,*,#4897,.T.);
#6415=ORIENTED_EDGE('',*,*,#4893,.F.);
#6416=ORIENTED_EDGE('',*,*,#4898,.T.);
#6417=ORIENTED_EDGE('',*,*,#4899,.T.);
#6418=ORIENTED_EDGE('',*,*,#4900,.T.);
#6419=ORIENTED_EDGE('',*,*,#4896,.F.);
#6420=ORIENTED_EDGE('',*,*,#4901,.T.);
#6421=ORIENTED_EDGE('',*,*,#4902,.T.);
#6422=ORIENTED_EDGE('',*,*,#4903,.T.);
#6423=ORIENTED_EDGE('',*,*,#4899,.F.);
#6424=ORIENTED_EDGE('',*,*,#4904,.T.);
#6425=ORIENTED_EDGE('',*,*,#4905,.T.);
#6426=ORIENTED_EDGE('',*,*,#4906,.T.);
#6427=ORIENTED_EDGE('',*,*,#4902,.F.);
#6428=ORIENTED_EDGE('',*,*,#4907,.T.);
#6429=ORIENTED_EDGE('',*,*,#4908,.T.);
#6430=ORIENTED_EDGE('',*,*,#4909,.T.);
#6431=ORIENTED_EDGE('',*,*,#4905,.F.);
#6432=ORIENTED_EDGE('',*,*,#4910,.T.);
#6433=ORIENTED_EDGE('',*,*,#4911,.T.);
#6434=ORIENTED_EDGE('',*,*,#4912,.T.);
#6435=ORIENTED_EDGE('',*,*,#4908,.F.);
#6436=ORIENTED_EDGE('',*,*,#4913,.T.);
#6437=ORIENTED_EDGE('',*,*,#4914,.T.);
#6438=ORIENTED_EDGE('',*,*,#4915,.T.);
#6439=ORIENTED_EDGE('',*,*,#4911,.F.);
#6440=ORIENTED_EDGE('',*,*,#4916,.T.);
#6441=ORIENTED_EDGE('',*,*,#4917,.T.);
#6442=ORIENTED_EDGE('',*,*,#4918,.T.);
#6443=ORIENTED_EDGE('',*,*,#4914,.F.);
#6444=ORIENTED_EDGE('',*,*,#4919,.T.);
#6445=ORIENTED_EDGE('',*,*,#4920,.T.);
#6446=ORIENTED_EDGE('',*,*,#4921,.T.);
#6447=ORIENTED_EDGE('',*,*,#4917,.F.);
#6448=ORIENTED_EDGE('',*,*,#4922,.T.);
#6449=ORIENTED_EDGE('',*,*,#4923,.F.);
#6450=ORIENTED_EDGE('',*,*,#4924,.T.);
#6451=ORIENTED_EDGE('',*,*,#4925,.F.);
#6452=ORIENTED_EDGE('',*,*,#4926,.T.);
#6453=ORIENTED_EDGE('',*,*,#4927,.T.);
#6454=ORIENTED_EDGE('',*,*,#4928,.T.);
#6455=ORIENTED_EDGE('',*,*,#4929,.F.);
#6456=ORIENTED_EDGE('',*,*,#4930,.F.);
#6457=ORIENTED_EDGE('',*,*,#4931,.T.);
#6458=ORIENTED_EDGE('',*,*,#4932,.T.);
#6459=ORIENTED_EDGE('',*,*,#4927,.F.);
#6460=ORIENTED_EDGE('',*,*,#4933,.F.);
#6461=ORIENTED_EDGE('',*,*,#4934,.T.);
#6462=ORIENTED_EDGE('',*,*,#4935,.T.);
#6463=ORIENTED_EDGE('',*,*,#4931,.F.);
#6464=ORIENTED_EDGE('',*,*,#4936,.F.);
#6465=ORIENTED_EDGE('',*,*,#4937,.T.);
#6466=ORIENTED_EDGE('',*,*,#4938,.T.);
#6467=ORIENTED_EDGE('',*,*,#4934,.F.);
#6468=ORIENTED_EDGE('',*,*,#4939,.F.);
#6469=ORIENTED_EDGE('',*,*,#4940,.T.);
#6470=ORIENTED_EDGE('',*,*,#4941,.T.);
#6471=ORIENTED_EDGE('',*,*,#4937,.F.);
#6472=ORIENTED_EDGE('',*,*,#4942,.F.);
#6473=ORIENTED_EDGE('',*,*,#4943,.T.);
#6474=ORIENTED_EDGE('',*,*,#4944,.T.);
#6475=ORIENTED_EDGE('',*,*,#4940,.F.);
#6476=ORIENTED_EDGE('',*,*,#4945,.F.);
#6477=ORIENTED_EDGE('',*,*,#4946,.T.);
#6478=ORIENTED_EDGE('',*,*,#4947,.T.);
#6479=ORIENTED_EDGE('',*,*,#4943,.F.);
#6480=ORIENTED_EDGE('',*,*,#4948,.F.);
#6481=ORIENTED_EDGE('',*,*,#4949,.T.);
#6482=ORIENTED_EDGE('',*,*,#4950,.T.);
#6483=ORIENTED_EDGE('',*,*,#4946,.F.);
#6484=ORIENTED_EDGE('',*,*,#4951,.F.);
#6485=ORIENTED_EDGE('',*,*,#4952,.T.);
#6486=ORIENTED_EDGE('',*,*,#4953,.T.);
#6487=ORIENTED_EDGE('',*,*,#4949,.F.);
#6488=ORIENTED_EDGE('',*,*,#4954,.F.);
#6489=ORIENTED_EDGE('',*,*,#4955,.T.);
#6490=ORIENTED_EDGE('',*,*,#4956,.T.);
#6491=ORIENTED_EDGE('',*,*,#4952,.F.);
#6492=ORIENTED_EDGE('',*,*,#4957,.F.);
#6493=ORIENTED_EDGE('',*,*,#4958,.T.);
#6494=ORIENTED_EDGE('',*,*,#4959,.T.);
#6495=ORIENTED_EDGE('',*,*,#4955,.F.);
#6496=ORIENTED_EDGE('',*,*,#4960,.F.);
#6497=ORIENTED_EDGE('',*,*,#4961,.T.);
#6498=ORIENTED_EDGE('',*,*,#4962,.T.);
#6499=ORIENTED_EDGE('',*,*,#4958,.F.);
#6500=ORIENTED_EDGE('',*,*,#4963,.F.);
#6501=ORIENTED_EDGE('',*,*,#4964,.T.);
#6502=ORIENTED_EDGE('',*,*,#4965,.T.);
#6503=ORIENTED_EDGE('',*,*,#4961,.F.);
#6504=ORIENTED_EDGE('',*,*,#4966,.F.);
#6505=ORIENTED_EDGE('',*,*,#4967,.T.);
#6506=ORIENTED_EDGE('',*,*,#4968,.T.);
#6507=ORIENTED_EDGE('',*,*,#4964,.F.);
#6508=ORIENTED_EDGE('',*,*,#4969,.F.);
#6509=ORIENTED_EDGE('',*,*,#4970,.T.);
#6510=ORIENTED_EDGE('',*,*,#4971,.T.);
#6511=ORIENTED_EDGE('',*,*,#4967,.F.);
#6512=ORIENTED_EDGE('',*,*,#4972,.F.);
#6513=ORIENTED_EDGE('',*,*,#4973,.F.);
#6514=ORIENTED_EDGE('',*,*,#4974,.F.);
#6515=ORIENTED_EDGE('',*,*,#4975,.F.);
#6516=ORIENTED_EDGE('',*,*,#4976,.T.);
#6517=ORIENTED_EDGE('',*,*,#4977,.T.);
#6518=ORIENTED_EDGE('',*,*,#4978,.T.);
#6519=ORIENTED_EDGE('',*,*,#4979,.T.);
#6520=ORIENTED_EDGE('',*,*,#4980,.T.);
#6521=ORIENTED_EDGE('',*,*,#4981,.T.);
#6522=ORIENTED_EDGE('',*,*,#4982,.T.);
#6523=ORIENTED_EDGE('',*,*,#4981,.F.);
#6524=ORIENTED_EDGE('',*,*,#4983,.T.);
#6525=ORIENTED_EDGE('',*,*,#4984,.T.);
#6526=ORIENTED_EDGE('',*,*,#4985,.T.);
#6527=ORIENTED_EDGE('',*,*,#4977,.F.);
#6528=ORIENTED_EDGE('',*,*,#4986,.T.);
#6529=ORIENTED_EDGE('',*,*,#4987,.T.);
#6530=ORIENTED_EDGE('',*,*,#4988,.T.);
#6531=ORIENTED_EDGE('',*,*,#4984,.F.);
#6532=ORIENTED_EDGE('',*,*,#4989,.T.);
#6533=ORIENTED_EDGE('',*,*,#4990,.T.);
#6534=ORIENTED_EDGE('',*,*,#4991,.T.);
#6535=ORIENTED_EDGE('',*,*,#4987,.F.);
#6536=ORIENTED_EDGE('',*,*,#4992,.T.);
#6537=ORIENTED_EDGE('',*,*,#4993,.T.);
#6538=ORIENTED_EDGE('',*,*,#4994,.T.);
#6539=ORIENTED_EDGE('',*,*,#4990,.F.);
#6540=ORIENTED_EDGE('',*,*,#4995,.T.);
#6541=ORIENTED_EDGE('',*,*,#4996,.T.);
#6542=ORIENTED_EDGE('',*,*,#4997,.T.);
#6543=ORIENTED_EDGE('',*,*,#4993,.F.);
#6544=ORIENTED_EDGE('',*,*,#4998,.T.);
#6545=ORIENTED_EDGE('',*,*,#4999,.T.);
#6546=ORIENTED_EDGE('',*,*,#5000,.T.);
#6547=ORIENTED_EDGE('',*,*,#4996,.F.);
#6548=ORIENTED_EDGE('',*,*,#5001,.T.);
#6549=ORIENTED_EDGE('',*,*,#5002,.T.);
#6550=ORIENTED_EDGE('',*,*,#5003,.T.);
#6551=ORIENTED_EDGE('',*,*,#4999,.F.);
#6552=ORIENTED_EDGE('',*,*,#5004,.T.);
#6553=ORIENTED_EDGE('',*,*,#5005,.T.);
#6554=ORIENTED_EDGE('',*,*,#5006,.T.);
#6555=ORIENTED_EDGE('',*,*,#5002,.F.);
#6556=ORIENTED_EDGE('',*,*,#5007,.T.);
#6557=ORIENTED_EDGE('',*,*,#5008,.T.);
#6558=ORIENTED_EDGE('',*,*,#5009,.T.);
#6559=ORIENTED_EDGE('',*,*,#5005,.F.);
#6560=ORIENTED_EDGE('',*,*,#5010,.T.);
#6561=ORIENTED_EDGE('',*,*,#5011,.T.);
#6562=ORIENTED_EDGE('',*,*,#5012,.T.);
#6563=ORIENTED_EDGE('',*,*,#5008,.F.);
#6564=ORIENTED_EDGE('',*,*,#5013,.T.);
#6565=ORIENTED_EDGE('',*,*,#5014,.T.);
#6566=ORIENTED_EDGE('',*,*,#5015,.T.);
#6567=ORIENTED_EDGE('',*,*,#5011,.F.);
#6568=ORIENTED_EDGE('',*,*,#5016,.T.);
#6569=ORIENTED_EDGE('',*,*,#5017,.T.);
#6570=ORIENTED_EDGE('',*,*,#5018,.T.);
#6571=ORIENTED_EDGE('',*,*,#5014,.F.);
#6572=ORIENTED_EDGE('',*,*,#5019,.T.);
#6573=ORIENTED_EDGE('',*,*,#5020,.T.);
#6574=ORIENTED_EDGE('',*,*,#5021,.T.);
#6575=ORIENTED_EDGE('',*,*,#5017,.F.);
#6576=ORIENTED_EDGE('',*,*,#5022,.T.);
#6577=ORIENTED_EDGE('',*,*,#5023,.F.);
#6578=ORIENTED_EDGE('',*,*,#5024,.T.);
#6579=ORIENTED_EDGE('',*,*,#5025,.F.);
#6580=ORIENTED_EDGE('',*,*,#5026,.T.);
#6581=ORIENTED_EDGE('',*,*,#5027,.T.);
#6582=ORIENTED_EDGE('',*,*,#5028,.T.);
#6583=ORIENTED_EDGE('',*,*,#5029,.F.);
#6584=ORIENTED_EDGE('',*,*,#5030,.F.);
#6585=ORIENTED_EDGE('',*,*,#5031,.T.);
#6586=ORIENTED_EDGE('',*,*,#5032,.T.);
#6587=ORIENTED_EDGE('',*,*,#5027,.F.);
#6588=ORIENTED_EDGE('',*,*,#5033,.F.);
#6589=ORIENTED_EDGE('',*,*,#5034,.T.);
#6590=ORIENTED_EDGE('',*,*,#5035,.T.);
#6591=ORIENTED_EDGE('',*,*,#5031,.F.);
#6592=ORIENTED_EDGE('',*,*,#5036,.F.);
#6593=ORIENTED_EDGE('',*,*,#5037,.T.);
#6594=ORIENTED_EDGE('',*,*,#5038,.T.);
#6595=ORIENTED_EDGE('',*,*,#5034,.F.);
#6596=ORIENTED_EDGE('',*,*,#5039,.F.);
#6597=ORIENTED_EDGE('',*,*,#5040,.T.);
#6598=ORIENTED_EDGE('',*,*,#5041,.T.);
#6599=ORIENTED_EDGE('',*,*,#5037,.F.);
#6600=ORIENTED_EDGE('',*,*,#5042,.F.);
#6601=ORIENTED_EDGE('',*,*,#5043,.T.);
#6602=ORIENTED_EDGE('',*,*,#5044,.T.);
#6603=ORIENTED_EDGE('',*,*,#5040,.F.);
#6604=ORIENTED_EDGE('',*,*,#5045,.F.);
#6605=ORIENTED_EDGE('',*,*,#5046,.T.);
#6606=ORIENTED_EDGE('',*,*,#5047,.T.);
#6607=ORIENTED_EDGE('',*,*,#5043,.F.);
#6608=ORIENTED_EDGE('',*,*,#5048,.F.);
#6609=ORIENTED_EDGE('',*,*,#5049,.T.);
#6610=ORIENTED_EDGE('',*,*,#5050,.T.);
#6611=ORIENTED_EDGE('',*,*,#5046,.F.);
#6612=ORIENTED_EDGE('',*,*,#5051,.F.);
#6613=ORIENTED_EDGE('',*,*,#5052,.T.);
#6614=ORIENTED_EDGE('',*,*,#5053,.T.);
#6615=ORIENTED_EDGE('',*,*,#5049,.F.);
#6616=ORIENTED_EDGE('',*,*,#5054,.F.);
#6617=ORIENTED_EDGE('',*,*,#5055,.T.);
#6618=ORIENTED_EDGE('',*,*,#5056,.T.);
#6619=ORIENTED_EDGE('',*,*,#5052,.F.);
#6620=ORIENTED_EDGE('',*,*,#5057,.F.);
#6621=ORIENTED_EDGE('',*,*,#5058,.T.);
#6622=ORIENTED_EDGE('',*,*,#5059,.T.);
#6623=ORIENTED_EDGE('',*,*,#5055,.F.);
#6624=ORIENTED_EDGE('',*,*,#5060,.F.);
#6625=ORIENTED_EDGE('',*,*,#5061,.T.);
#6626=ORIENTED_EDGE('',*,*,#5062,.T.);
#6627=ORIENTED_EDGE('',*,*,#5058,.F.);
#6628=ORIENTED_EDGE('',*,*,#5063,.F.);
#6629=ORIENTED_EDGE('',*,*,#5064,.T.);
#6630=ORIENTED_EDGE('',*,*,#5065,.T.);
#6631=ORIENTED_EDGE('',*,*,#5061,.F.);
#6632=ORIENTED_EDGE('',*,*,#5066,.F.);
#6633=ORIENTED_EDGE('',*,*,#5067,.T.);
#6634=ORIENTED_EDGE('',*,*,#5068,.T.);
#6635=ORIENTED_EDGE('',*,*,#5064,.F.);
#6636=ORIENTED_EDGE('',*,*,#5069,.F.);
#6637=ORIENTED_EDGE('',*,*,#5070,.T.);
#6638=ORIENTED_EDGE('',*,*,#5071,.T.);
#6639=ORIENTED_EDGE('',*,*,#5067,.F.);
#6640=ORIENTED_EDGE('',*,*,#5072,.F.);
#6641=ORIENTED_EDGE('',*,*,#5073,.F.);
#6642=ORIENTED_EDGE('',*,*,#5074,.F.);
#6643=ORIENTED_EDGE('',*,*,#5075,.F.);
#6644=ORIENTED_EDGE('',*,*,#5076,.T.);
#6645=ORIENTED_EDGE('',*,*,#5077,.T.);
#6646=ORIENTED_EDGE('',*,*,#5078,.T.);
#6647=ORIENTED_EDGE('',*,*,#5079,.T.);
#6648=ORIENTED_EDGE('',*,*,#5080,.T.);
#6649=ORIENTED_EDGE('',*,*,#5081,.T.);
#6650=ORIENTED_EDGE('',*,*,#5082,.T.);
#6651=ORIENTED_EDGE('',*,*,#5081,.F.);
#6652=ORIENTED_EDGE('',*,*,#5083,.T.);
#6653=ORIENTED_EDGE('',*,*,#5084,.T.);
#6654=ORIENTED_EDGE('',*,*,#5085,.T.);
#6655=ORIENTED_EDGE('',*,*,#5077,.F.);
#6656=ORIENTED_EDGE('',*,*,#5086,.T.);
#6657=ORIENTED_EDGE('',*,*,#5087,.T.);
#6658=ORIENTED_EDGE('',*,*,#5088,.T.);
#6659=ORIENTED_EDGE('',*,*,#5084,.F.);
#6660=ORIENTED_EDGE('',*,*,#5089,.T.);
#6661=ORIENTED_EDGE('',*,*,#5090,.T.);
#6662=ORIENTED_EDGE('',*,*,#5091,.T.);
#6663=ORIENTED_EDGE('',*,*,#5087,.F.);
#6664=ORIENTED_EDGE('',*,*,#5092,.T.);
#6665=ORIENTED_EDGE('',*,*,#5093,.T.);
#6666=ORIENTED_EDGE('',*,*,#5094,.T.);
#6667=ORIENTED_EDGE('',*,*,#5090,.F.);
#6668=ORIENTED_EDGE('',*,*,#5095,.T.);
#6669=ORIENTED_EDGE('',*,*,#5096,.T.);
#6670=ORIENTED_EDGE('',*,*,#5097,.T.);
#6671=ORIENTED_EDGE('',*,*,#5093,.F.);
#6672=ORIENTED_EDGE('',*,*,#5098,.T.);
#6673=ORIENTED_EDGE('',*,*,#5099,.T.);
#6674=ORIENTED_EDGE('',*,*,#5100,.T.);
#6675=ORIENTED_EDGE('',*,*,#5096,.F.);
#6676=ORIENTED_EDGE('',*,*,#5101,.T.);
#6677=ORIENTED_EDGE('',*,*,#5102,.T.);
#6678=ORIENTED_EDGE('',*,*,#5103,.T.);
#6679=ORIENTED_EDGE('',*,*,#5099,.F.);
#6680=ORIENTED_EDGE('',*,*,#5104,.T.);
#6681=ORIENTED_EDGE('',*,*,#5105,.T.);
#6682=ORIENTED_EDGE('',*,*,#5106,.T.);
#6683=ORIENTED_EDGE('',*,*,#5102,.F.);
#6684=ORIENTED_EDGE('',*,*,#5107,.T.);
#6685=ORIENTED_EDGE('',*,*,#5108,.T.);
#6686=ORIENTED_EDGE('',*,*,#5109,.T.);
#6687=ORIENTED_EDGE('',*,*,#5105,.F.);
#6688=ORIENTED_EDGE('',*,*,#5110,.T.);
#6689=ORIENTED_EDGE('',*,*,#5111,.T.);
#6690=ORIENTED_EDGE('',*,*,#5112,.T.);
#6691=ORIENTED_EDGE('',*,*,#5108,.F.);
#6692=ORIENTED_EDGE('',*,*,#5113,.T.);
#6693=ORIENTED_EDGE('',*,*,#5114,.T.);
#6694=ORIENTED_EDGE('',*,*,#5115,.T.);
#6695=ORIENTED_EDGE('',*,*,#5111,.F.);
#6696=ORIENTED_EDGE('',*,*,#5116,.T.);
#6697=ORIENTED_EDGE('',*,*,#5117,.T.);
#6698=ORIENTED_EDGE('',*,*,#5118,.T.);
#6699=ORIENTED_EDGE('',*,*,#5114,.F.);
#6700=ORIENTED_EDGE('',*,*,#5119,.T.);
#6701=ORIENTED_EDGE('',*,*,#5120,.T.);
#6702=ORIENTED_EDGE('',*,*,#5121,.T.);
#6703=ORIENTED_EDGE('',*,*,#5117,.F.);
#6704=ORIENTED_EDGE('',*,*,#5122,.T.);
#6705=ORIENTED_EDGE('',*,*,#5123,.F.);
#6706=ORIENTED_EDGE('',*,*,#5124,.T.);
#6707=ORIENTED_EDGE('',*,*,#5125,.F.);
#6708=ORIENTED_EDGE('',*,*,#5126,.T.);
#6709=ORIENTED_EDGE('',*,*,#5127,.T.);
#6710=ORIENTED_EDGE('',*,*,#5128,.T.);
#6711=ORIENTED_EDGE('',*,*,#5129,.F.);
#6712=ORIENTED_EDGE('',*,*,#5130,.F.);
#6713=ORIENTED_EDGE('',*,*,#5131,.T.);
#6714=ORIENTED_EDGE('',*,*,#5132,.T.);
#6715=ORIENTED_EDGE('',*,*,#5127,.F.);
#6716=ORIENTED_EDGE('',*,*,#5133,.F.);
#6717=ORIENTED_EDGE('',*,*,#5134,.T.);
#6718=ORIENTED_EDGE('',*,*,#5135,.T.);
#6719=ORIENTED_EDGE('',*,*,#5131,.F.);
#6720=ORIENTED_EDGE('',*,*,#5136,.F.);
#6721=ORIENTED_EDGE('',*,*,#5137,.T.);
#6722=ORIENTED_EDGE('',*,*,#5138,.T.);
#6723=ORIENTED_EDGE('',*,*,#5134,.F.);
#6724=ORIENTED_EDGE('',*,*,#5139,.F.);
#6725=ORIENTED_EDGE('',*,*,#5140,.T.);
#6726=ORIENTED_EDGE('',*,*,#5141,.T.);
#6727=ORIENTED_EDGE('',*,*,#5137,.F.);
#6728=ORIENTED_EDGE('',*,*,#5142,.F.);
#6729=ORIENTED_EDGE('',*,*,#5143,.T.);
#6730=ORIENTED_EDGE('',*,*,#5144,.T.);
#6731=ORIENTED_EDGE('',*,*,#5140,.F.);
#6732=ORIENTED_EDGE('',*,*,#5145,.F.);
#6733=ORIENTED_EDGE('',*,*,#5146,.T.);
#6734=ORIENTED_EDGE('',*,*,#5147,.T.);
#6735=ORIENTED_EDGE('',*,*,#5143,.F.);
#6736=ORIENTED_EDGE('',*,*,#5148,.F.);
#6737=ORIENTED_EDGE('',*,*,#5149,.T.);
#6738=ORIENTED_EDGE('',*,*,#5150,.T.);
#6739=ORIENTED_EDGE('',*,*,#5146,.F.);
#6740=ORIENTED_EDGE('',*,*,#5151,.F.);
#6741=ORIENTED_EDGE('',*,*,#5152,.T.);
#6742=ORIENTED_EDGE('',*,*,#5153,.T.);
#6743=ORIENTED_EDGE('',*,*,#5149,.F.);
#6744=ORIENTED_EDGE('',*,*,#5154,.F.);
#6745=ORIENTED_EDGE('',*,*,#5155,.T.);
#6746=ORIENTED_EDGE('',*,*,#5156,.T.);
#6747=ORIENTED_EDGE('',*,*,#5152,.F.);
#6748=ORIENTED_EDGE('',*,*,#5157,.F.);
#6749=ORIENTED_EDGE('',*,*,#5158,.T.);
#6750=ORIENTED_EDGE('',*,*,#5159,.T.);
#6751=ORIENTED_EDGE('',*,*,#5155,.F.);
#6752=ORIENTED_EDGE('',*,*,#5160,.F.);
#6753=ORIENTED_EDGE('',*,*,#5161,.T.);
#6754=ORIENTED_EDGE('',*,*,#5162,.T.);
#6755=ORIENTED_EDGE('',*,*,#5158,.F.);
#6756=ORIENTED_EDGE('',*,*,#5163,.F.);
#6757=ORIENTED_EDGE('',*,*,#5164,.T.);
#6758=ORIENTED_EDGE('',*,*,#5165,.T.);
#6759=ORIENTED_EDGE('',*,*,#5161,.F.);
#6760=ORIENTED_EDGE('',*,*,#5166,.F.);
#6761=ORIENTED_EDGE('',*,*,#5167,.T.);
#6762=ORIENTED_EDGE('',*,*,#5168,.T.);
#6763=ORIENTED_EDGE('',*,*,#5164,.F.);
#6764=ORIENTED_EDGE('',*,*,#5169,.F.);
#6765=ORIENTED_EDGE('',*,*,#5170,.T.);
#6766=ORIENTED_EDGE('',*,*,#5171,.T.);
#6767=ORIENTED_EDGE('',*,*,#5167,.F.);
#6768=ORIENTED_EDGE('',*,*,#5172,.F.);
#6769=ORIENTED_EDGE('',*,*,#5173,.F.);
#6770=ORIENTED_EDGE('',*,*,#5174,.F.);
#6771=ORIENTED_EDGE('',*,*,#5175,.F.);
#6772=ORIENTED_EDGE('',*,*,#5176,.T.);
#6773=ORIENTED_EDGE('',*,*,#5177,.T.);
#6774=ORIENTED_EDGE('',*,*,#5178,.T.);
#6775=ORIENTED_EDGE('',*,*,#5179,.T.);
#6776=ORIENTED_EDGE('',*,*,#5180,.T.);
#6777=ORIENTED_EDGE('',*,*,#5181,.T.);
#6778=ORIENTED_EDGE('',*,*,#5182,.T.);
#6779=ORIENTED_EDGE('',*,*,#5181,.F.);
#6780=ORIENTED_EDGE('',*,*,#5183,.T.);
#6781=ORIENTED_EDGE('',*,*,#5184,.T.);
#6782=ORIENTED_EDGE('',*,*,#5185,.T.);
#6783=ORIENTED_EDGE('',*,*,#5177,.F.);
#6784=ORIENTED_EDGE('',*,*,#5186,.T.);
#6785=ORIENTED_EDGE('',*,*,#5187,.T.);
#6786=ORIENTED_EDGE('',*,*,#5188,.T.);
#6787=ORIENTED_EDGE('',*,*,#5184,.F.);
#6788=ORIENTED_EDGE('',*,*,#5189,.T.);
#6789=ORIENTED_EDGE('',*,*,#5190,.T.);
#6790=ORIENTED_EDGE('',*,*,#5191,.T.);
#6791=ORIENTED_EDGE('',*,*,#5187,.F.);
#6792=ORIENTED_EDGE('',*,*,#5192,.T.);
#6793=ORIENTED_EDGE('',*,*,#5193,.T.);
#6794=ORIENTED_EDGE('',*,*,#5194,.T.);
#6795=ORIENTED_EDGE('',*,*,#5190,.F.);
#6796=ORIENTED_EDGE('',*,*,#5195,.T.);
#6797=ORIENTED_EDGE('',*,*,#5196,.T.);
#6798=ORIENTED_EDGE('',*,*,#5197,.T.);
#6799=ORIENTED_EDGE('',*,*,#5193,.F.);
#6800=ORIENTED_EDGE('',*,*,#5198,.T.);
#6801=ORIENTED_EDGE('',*,*,#5199,.T.);
#6802=ORIENTED_EDGE('',*,*,#5200,.T.);
#6803=ORIENTED_EDGE('',*,*,#5196,.F.);
#6804=ORIENTED_EDGE('',*,*,#5201,.T.);
#6805=ORIENTED_EDGE('',*,*,#5202,.T.);
#6806=ORIENTED_EDGE('',*,*,#5203,.T.);
#6807=ORIENTED_EDGE('',*,*,#5199,.F.);
#6808=ORIENTED_EDGE('',*,*,#5204,.T.);
#6809=ORIENTED_EDGE('',*,*,#5205,.T.);
#6810=ORIENTED_EDGE('',*,*,#5206,.T.);
#6811=ORIENTED_EDGE('',*,*,#5202,.F.);
#6812=ORIENTED_EDGE('',*,*,#5207,.T.);
#6813=ORIENTED_EDGE('',*,*,#5208,.T.);
#6814=ORIENTED_EDGE('',*,*,#5209,.T.);
#6815=ORIENTED_EDGE('',*,*,#5205,.F.);
#6816=ORIENTED_EDGE('',*,*,#5210,.T.);
#6817=ORIENTED_EDGE('',*,*,#5211,.T.);
#6818=ORIENTED_EDGE('',*,*,#5212,.T.);
#6819=ORIENTED_EDGE('',*,*,#5208,.F.);
#6820=ORIENTED_EDGE('',*,*,#5213,.T.);
#6821=ORIENTED_EDGE('',*,*,#5214,.T.);
#6822=ORIENTED_EDGE('',*,*,#5215,.T.);
#6823=ORIENTED_EDGE('',*,*,#5211,.F.);
#6824=ORIENTED_EDGE('',*,*,#5216,.T.);
#6825=ORIENTED_EDGE('',*,*,#5217,.T.);
#6826=ORIENTED_EDGE('',*,*,#5218,.T.);
#6827=ORIENTED_EDGE('',*,*,#5214,.F.);
#6828=ORIENTED_EDGE('',*,*,#5219,.T.);
#6829=ORIENTED_EDGE('',*,*,#5220,.T.);
#6830=ORIENTED_EDGE('',*,*,#5221,.T.);
#6831=ORIENTED_EDGE('',*,*,#5217,.F.);
#6832=ORIENTED_EDGE('',*,*,#5222,.T.);
#6833=ORIENTED_EDGE('',*,*,#5223,.F.);
#6834=ORIENTED_EDGE('',*,*,#5224,.T.);
#6835=ORIENTED_EDGE('',*,*,#5225,.F.);
#6836=ORIENTED_EDGE('',*,*,#5226,.T.);
#6837=ORIENTED_EDGE('',*,*,#5227,.T.);
#6838=ORIENTED_EDGE('',*,*,#5228,.T.);
#6839=ORIENTED_EDGE('',*,*,#5229,.F.);
#6840=ORIENTED_EDGE('',*,*,#5230,.F.);
#6841=ORIENTED_EDGE('',*,*,#5231,.T.);
#6842=ORIENTED_EDGE('',*,*,#5232,.T.);
#6843=ORIENTED_EDGE('',*,*,#5227,.F.);
#6844=ORIENTED_EDGE('',*,*,#5233,.F.);
#6845=ORIENTED_EDGE('',*,*,#5234,.T.);
#6846=ORIENTED_EDGE('',*,*,#5235,.T.);
#6847=ORIENTED_EDGE('',*,*,#5231,.F.);
#6848=ORIENTED_EDGE('',*,*,#5236,.F.);
#6849=ORIENTED_EDGE('',*,*,#5237,.T.);
#6850=ORIENTED_EDGE('',*,*,#5238,.T.);
#6851=ORIENTED_EDGE('',*,*,#5234,.F.);
#6852=ORIENTED_EDGE('',*,*,#5239,.F.);
#6853=ORIENTED_EDGE('',*,*,#5240,.T.);
#6854=ORIENTED_EDGE('',*,*,#5241,.T.);
#6855=ORIENTED_EDGE('',*,*,#5237,.F.);
#6856=ORIENTED_EDGE('',*,*,#5242,.F.);
#6857=ORIENTED_EDGE('',*,*,#5243,.T.);
#6858=ORIENTED_EDGE('',*,*,#5244,.T.);
#6859=ORIENTED_EDGE('',*,*,#5240,.F.);
#6860=ORIENTED_EDGE('',*,*,#5245,.F.);
#6861=ORIENTED_EDGE('',*,*,#5246,.T.);
#6862=ORIENTED_EDGE('',*,*,#5247,.T.);
#6863=ORIENTED_EDGE('',*,*,#5243,.F.);
#6864=ORIENTED_EDGE('',*,*,#5248,.F.);
#6865=ORIENTED_EDGE('',*,*,#5249,.T.);
#6866=ORIENTED_EDGE('',*,*,#5250,.T.);
#6867=ORIENTED_EDGE('',*,*,#5246,.F.);
#6868=ORIENTED_EDGE('',*,*,#5251,.F.);
#6869=ORIENTED_EDGE('',*,*,#5252,.T.);
#6870=ORIENTED_EDGE('',*,*,#5253,.T.);
#6871=ORIENTED_EDGE('',*,*,#5249,.F.);
#6872=ORIENTED_EDGE('',*,*,#5254,.F.);
#6873=ORIENTED_EDGE('',*,*,#5255,.T.);
#6874=ORIENTED_EDGE('',*,*,#5256,.T.);
#6875=ORIENTED_EDGE('',*,*,#5252,.F.);
#6876=ORIENTED_EDGE('',*,*,#5257,.F.);
#6877=ORIENTED_EDGE('',*,*,#5258,.T.);
#6878=ORIENTED_EDGE('',*,*,#5259,.T.);
#6879=ORIENTED_EDGE('',*,*,#5255,.F.);
#6880=ORIENTED_EDGE('',*,*,#5260,.F.);
#6881=ORIENTED_EDGE('',*,*,#5261,.T.);
#6882=ORIENTED_EDGE('',*,*,#5262,.T.);
#6883=ORIENTED_EDGE('',*,*,#5258,.F.);
#6884=ORIENTED_EDGE('',*,*,#5263,.F.);
#6885=ORIENTED_EDGE('',*,*,#5264,.T.);
#6886=ORIENTED_EDGE('',*,*,#5265,.T.);
#6887=ORIENTED_EDGE('',*,*,#5261,.F.);
#6888=ORIENTED_EDGE('',*,*,#5266,.F.);
#6889=ORIENTED_EDGE('',*,*,#5267,.T.);
#6890=ORIENTED_EDGE('',*,*,#5268,.T.);
#6891=ORIENTED_EDGE('',*,*,#5264,.F.);
#6892=ORIENTED_EDGE('',*,*,#5269,.F.);
#6893=ORIENTED_EDGE('',*,*,#5270,.T.);
#6894=ORIENTED_EDGE('',*,*,#5271,.T.);
#6895=ORIENTED_EDGE('',*,*,#5267,.F.);
#6896=ORIENTED_EDGE('',*,*,#5272,.F.);
#6897=ORIENTED_EDGE('',*,*,#5273,.F.);
#6898=ORIENTED_EDGE('',*,*,#5274,.F.);
#6899=ORIENTED_EDGE('',*,*,#5275,.F.);
#6900=ORIENTED_EDGE('',*,*,#5276,.T.);
#6901=ORIENTED_EDGE('',*,*,#5277,.T.);
#6902=ORIENTED_EDGE('',*,*,#5278,.T.);
#6903=ORIENTED_EDGE('',*,*,#5279,.T.);
#6904=ORIENTED_EDGE('',*,*,#5280,.F.);
#6905=ORIENTED_EDGE('',*,*,#5281,.T.);
#6906=ORIENTED_EDGE('',*,*,#5282,.T.);
#6907=ORIENTED_EDGE('',*,*,#5283,.T.);
#6908=ORIENTED_EDGE('',*,*,#5284,.T.);
#6909=ORIENTED_EDGE('',*,*,#5277,.F.);
#6910=ORIENTED_EDGE('',*,*,#5285,.T.);
#6911=ORIENTED_EDGE('',*,*,#5286,.T.);
#6912=ORIENTED_EDGE('',*,*,#5287,.T.);
#6913=ORIENTED_EDGE('',*,*,#5283,.F.);
#6914=ORIENTED_EDGE('',*,*,#5288,.T.);
#6915=ORIENTED_EDGE('',*,*,#5289,.T.);
#6916=ORIENTED_EDGE('',*,*,#5290,.T.);
#6917=ORIENTED_EDGE('',*,*,#5286,.F.);
#6918=ORIENTED_EDGE('',*,*,#5291,.T.);
#6919=ORIENTED_EDGE('',*,*,#5292,.T.);
#6920=ORIENTED_EDGE('',*,*,#5293,.T.);
#6921=ORIENTED_EDGE('',*,*,#5289,.F.);
#6922=ORIENTED_EDGE('',*,*,#5294,.T.);
#6923=ORIENTED_EDGE('',*,*,#5295,.T.);
#6924=ORIENTED_EDGE('',*,*,#5296,.T.);
#6925=ORIENTED_EDGE('',*,*,#5292,.F.);
#6926=ORIENTED_EDGE('',*,*,#5297,.T.);
#6927=ORIENTED_EDGE('',*,*,#5298,.T.);
#6928=ORIENTED_EDGE('',*,*,#5299,.T.);
#6929=ORIENTED_EDGE('',*,*,#5295,.F.);
#6930=ORIENTED_EDGE('',*,*,#5300,.T.);
#6931=ORIENTED_EDGE('',*,*,#5301,.T.);
#6932=ORIENTED_EDGE('',*,*,#5302,.T.);
#6933=ORIENTED_EDGE('',*,*,#5298,.F.);
#6934=ORIENTED_EDGE('',*,*,#5303,.T.);
#6935=ORIENTED_EDGE('',*,*,#5304,.T.);
#6936=ORIENTED_EDGE('',*,*,#5305,.T.);
#6937=ORIENTED_EDGE('',*,*,#5301,.F.);
#6938=ORIENTED_EDGE('',*,*,#5306,.T.);
#6939=ORIENTED_EDGE('',*,*,#5307,.T.);
#6940=ORIENTED_EDGE('',*,*,#5308,.T.);
#6941=ORIENTED_EDGE('',*,*,#5304,.F.);
#6942=ORIENTED_EDGE('',*,*,#5309,.T.);
#6943=ORIENTED_EDGE('',*,*,#5310,.T.);
#6944=ORIENTED_EDGE('',*,*,#5311,.T.);
#6945=ORIENTED_EDGE('',*,*,#5307,.F.);
#6946=ORIENTED_EDGE('',*,*,#5312,.T.);
#6947=ORIENTED_EDGE('',*,*,#5313,.T.);
#6948=ORIENTED_EDGE('',*,*,#5314,.T.);
#6949=ORIENTED_EDGE('',*,*,#5310,.F.);
#6950=ORIENTED_EDGE('',*,*,#5315,.T.);
#6951=ORIENTED_EDGE('',*,*,#5316,.T.);
#6952=ORIENTED_EDGE('',*,*,#5317,.T.);
#6953=ORIENTED_EDGE('',*,*,#5313,.F.);
#6954=ORIENTED_EDGE('',*,*,#5318,.T.);
#6955=ORIENTED_EDGE('',*,*,#5319,.T.);
#6956=ORIENTED_EDGE('',*,*,#5320,.T.);
#6957=ORIENTED_EDGE('',*,*,#5316,.F.);
#6958=ORIENTED_EDGE('',*,*,#5321,.T.);
#6959=ORIENTED_EDGE('',*,*,#5322,.F.);
#6960=ORIENTED_EDGE('',*,*,#5323,.T.);
#6961=ORIENTED_EDGE('',*,*,#5324,.F.);
#6962=ORIENTED_EDGE('',*,*,#5325,.T.);
#6963=ORIENTED_EDGE('',*,*,#5326,.T.);
#6964=ORIENTED_EDGE('',*,*,#5327,.T.);
#6965=ORIENTED_EDGE('',*,*,#5328,.T.);
#6966=ORIENTED_EDGE('',*,*,#5329,.F.);
#6967=ORIENTED_EDGE('',*,*,#5330,.T.);
#6968=ORIENTED_EDGE('',*,*,#5331,.T.);
#6969=ORIENTED_EDGE('',*,*,#5332,.T.);
#6970=ORIENTED_EDGE('',*,*,#5333,.T.);
#6971=ORIENTED_EDGE('',*,*,#5326,.F.);
#6972=ORIENTED_EDGE('',*,*,#5334,.T.);
#6973=ORIENTED_EDGE('',*,*,#5335,.T.);
#6974=ORIENTED_EDGE('',*,*,#5336,.T.);
#6975=ORIENTED_EDGE('',*,*,#5332,.F.);
#6976=ORIENTED_EDGE('',*,*,#5337,.T.);
#6977=ORIENTED_EDGE('',*,*,#5338,.T.);
#6978=ORIENTED_EDGE('',*,*,#5339,.T.);
#6979=ORIENTED_EDGE('',*,*,#5335,.F.);
#6980=ORIENTED_EDGE('',*,*,#5340,.T.);
#6981=ORIENTED_EDGE('',*,*,#5341,.T.);
#6982=ORIENTED_EDGE('',*,*,#5342,.T.);
#6983=ORIENTED_EDGE('',*,*,#5338,.F.);
#6984=ORIENTED_EDGE('',*,*,#5343,.T.);
#6985=ORIENTED_EDGE('',*,*,#5344,.T.);
#6986=ORIENTED_EDGE('',*,*,#5345,.T.);
#6987=ORIENTED_EDGE('',*,*,#5341,.F.);
#6988=ORIENTED_EDGE('',*,*,#5346,.T.);
#6989=ORIENTED_EDGE('',*,*,#5347,.T.);
#6990=ORIENTED_EDGE('',*,*,#5348,.T.);
#6991=ORIENTED_EDGE('',*,*,#5344,.F.);
#6992=ORIENTED_EDGE('',*,*,#5349,.T.);
#6993=ORIENTED_EDGE('',*,*,#5350,.T.);
#6994=ORIENTED_EDGE('',*,*,#5351,.T.);
#6995=ORIENTED_EDGE('',*,*,#5347,.F.);
#6996=ORIENTED_EDGE('',*,*,#5352,.T.);
#6997=ORIENTED_EDGE('',*,*,#5353,.T.);
#6998=ORIENTED_EDGE('',*,*,#5354,.T.);
#6999=ORIENTED_EDGE('',*,*,#5350,.F.);
#7000=ORIENTED_EDGE('',*,*,#5355,.T.);
#7001=ORIENTED_EDGE('',*,*,#5356,.T.);
#7002=ORIENTED_EDGE('',*,*,#5357,.T.);
#7003=ORIENTED_EDGE('',*,*,#5353,.F.);
#7004=ORIENTED_EDGE('',*,*,#5358,.T.);
#7005=ORIENTED_EDGE('',*,*,#5359,.T.);
#7006=ORIENTED_EDGE('',*,*,#5360,.T.);
#7007=ORIENTED_EDGE('',*,*,#5356,.F.);
#7008=ORIENTED_EDGE('',*,*,#5361,.T.);
#7009=ORIENTED_EDGE('',*,*,#5362,.T.);
#7010=ORIENTED_EDGE('',*,*,#5363,.T.);
#7011=ORIENTED_EDGE('',*,*,#5359,.F.);
#7012=ORIENTED_EDGE('',*,*,#5364,.T.);
#7013=ORIENTED_EDGE('',*,*,#5365,.T.);
#7014=ORIENTED_EDGE('',*,*,#5366,.T.);
#7015=ORIENTED_EDGE('',*,*,#5362,.F.);
#7016=ORIENTED_EDGE('',*,*,#5367,.T.);
#7017=ORIENTED_EDGE('',*,*,#5368,.T.);
#7018=ORIENTED_EDGE('',*,*,#5369,.T.);
#7019=ORIENTED_EDGE('',*,*,#5365,.F.);
#7020=ORIENTED_EDGE('',*,*,#5370,.T.);
#7021=ORIENTED_EDGE('',*,*,#5371,.F.);
#7022=ORIENTED_EDGE('',*,*,#5372,.T.);
#7023=ORIENTED_EDGE('',*,*,#5373,.F.);
#7024=ORIENTED_EDGE('',*,*,#5374,.T.);
#7025=ORIENTED_EDGE('',*,*,#5375,.T.);
#7026=ORIENTED_EDGE('',*,*,#5376,.T.);
#7027=ORIENTED_EDGE('',*,*,#5377,.F.);
#7028=ORIENTED_EDGE('',*,*,#5378,.F.);
#7029=ORIENTED_EDGE('',*,*,#5379,.T.);
#7030=ORIENTED_EDGE('',*,*,#5380,.T.);
#7031=ORIENTED_EDGE('',*,*,#5375,.F.);
#7032=ORIENTED_EDGE('',*,*,#5381,.F.);
#7033=ORIENTED_EDGE('',*,*,#5382,.T.);
#7034=ORIENTED_EDGE('',*,*,#5383,.T.);
#7035=ORIENTED_EDGE('',*,*,#5379,.F.);
#7036=ORIENTED_EDGE('',*,*,#5384,.F.);
#7037=ORIENTED_EDGE('',*,*,#5385,.T.);
#7038=ORIENTED_EDGE('',*,*,#5386,.T.);
#7039=ORIENTED_EDGE('',*,*,#5382,.F.);
#7040=ORIENTED_EDGE('',*,*,#5387,.F.);
#7041=ORIENTED_EDGE('',*,*,#5388,.T.);
#7042=ORIENTED_EDGE('',*,*,#5389,.T.);
#7043=ORIENTED_EDGE('',*,*,#5385,.F.);
#7044=ORIENTED_EDGE('',*,*,#5390,.F.);
#7045=ORIENTED_EDGE('',*,*,#5391,.T.);
#7046=ORIENTED_EDGE('',*,*,#5392,.T.);
#7047=ORIENTED_EDGE('',*,*,#5388,.F.);
#7048=ORIENTED_EDGE('',*,*,#5393,.F.);
#7049=ORIENTED_EDGE('',*,*,#5394,.T.);
#7050=ORIENTED_EDGE('',*,*,#5395,.T.);
#7051=ORIENTED_EDGE('',*,*,#5391,.F.);
#7052=ORIENTED_EDGE('',*,*,#5396,.F.);
#7053=ORIENTED_EDGE('',*,*,#5397,.T.);
#7054=ORIENTED_EDGE('',*,*,#5398,.T.);
#7055=ORIENTED_EDGE('',*,*,#5394,.F.);
#7056=ORIENTED_EDGE('',*,*,#5399,.F.);
#7057=ORIENTED_EDGE('',*,*,#5400,.T.);
#7058=ORIENTED_EDGE('',*,*,#5401,.T.);
#7059=ORIENTED_EDGE('',*,*,#5397,.F.);
#7060=ORIENTED_EDGE('',*,*,#5402,.F.);
#7061=ORIENTED_EDGE('',*,*,#5403,.T.);
#7062=ORIENTED_EDGE('',*,*,#5404,.T.);
#7063=ORIENTED_EDGE('',*,*,#5400,.F.);
#7064=ORIENTED_EDGE('',*,*,#5405,.F.);
#7065=ORIENTED_EDGE('',*,*,#5406,.T.);
#7066=ORIENTED_EDGE('',*,*,#5407,.T.);
#7067=ORIENTED_EDGE('',*,*,#5403,.F.);
#7068=ORIENTED_EDGE('',*,*,#5408,.F.);
#7069=ORIENTED_EDGE('',*,*,#5409,.T.);
#7070=ORIENTED_EDGE('',*,*,#5410,.T.);
#7071=ORIENTED_EDGE('',*,*,#5406,.F.);
#7072=ORIENTED_EDGE('',*,*,#5411,.F.);
#7073=ORIENTED_EDGE('',*,*,#5412,.T.);
#7074=ORIENTED_EDGE('',*,*,#5413,.T.);
#7075=ORIENTED_EDGE('',*,*,#5409,.F.);
#7076=ORIENTED_EDGE('',*,*,#5414,.F.);
#7077=ORIENTED_EDGE('',*,*,#5415,.T.);
#7078=ORIENTED_EDGE('',*,*,#5416,.T.);
#7079=ORIENTED_EDGE('',*,*,#5412,.F.);
#7080=ORIENTED_EDGE('',*,*,#5417,.F.);
#7081=ORIENTED_EDGE('',*,*,#5418,.F.);
#7082=ORIENTED_EDGE('',*,*,#5419,.F.);
#7083=ORIENTED_EDGE('',*,*,#5420,.F.);
#7084=ORIENTED_EDGE('',*,*,#5421,.T.);
#7085=ORIENTED_EDGE('',*,*,#5422,.T.);
#7086=ORIENTED_EDGE('',*,*,#5423,.T.);
#7087=ORIENTED_EDGE('',*,*,#5424,.F.);
#7088=ORIENTED_EDGE('',*,*,#5425,.F.);
#7089=ORIENTED_EDGE('',*,*,#5426,.T.);
#7090=ORIENTED_EDGE('',*,*,#5427,.T.);
#7091=ORIENTED_EDGE('',*,*,#5422,.F.);
#7092=ORIENTED_EDGE('',*,*,#5428,.F.);
#7093=ORIENTED_EDGE('',*,*,#5429,.T.);
#7094=ORIENTED_EDGE('',*,*,#5430,.T.);
#7095=ORIENTED_EDGE('',*,*,#5426,.F.);
#7096=ORIENTED_EDGE('',*,*,#5431,.F.);
#7097=ORIENTED_EDGE('',*,*,#5432,.T.);
#7098=ORIENTED_EDGE('',*,*,#5433,.T.);
#7099=ORIENTED_EDGE('',*,*,#5429,.F.);
#7100=ORIENTED_EDGE('',*,*,#5434,.F.);
#7101=ORIENTED_EDGE('',*,*,#5435,.T.);
#7102=ORIENTED_EDGE('',*,*,#5436,.T.);
#7103=ORIENTED_EDGE('',*,*,#5432,.F.);
#7104=ORIENTED_EDGE('',*,*,#5437,.F.);
#7105=ORIENTED_EDGE('',*,*,#5438,.T.);
#7106=ORIENTED_EDGE('',*,*,#5439,.T.);
#7107=ORIENTED_EDGE('',*,*,#5435,.F.);
#7108=ORIENTED_EDGE('',*,*,#5440,.F.);
#7109=ORIENTED_EDGE('',*,*,#5441,.T.);
#7110=ORIENTED_EDGE('',*,*,#5442,.T.);
#7111=ORIENTED_EDGE('',*,*,#5438,.F.);
#7112=ORIENTED_EDGE('',*,*,#5443,.F.);
#7113=ORIENTED_EDGE('',*,*,#5444,.T.);
#7114=ORIENTED_EDGE('',*,*,#5445,.T.);
#7115=ORIENTED_EDGE('',*,*,#5441,.F.);
#7116=ORIENTED_EDGE('',*,*,#5446,.F.);
#7117=ORIENTED_EDGE('',*,*,#5447,.T.);
#7118=ORIENTED_EDGE('',*,*,#5448,.T.);
#7119=ORIENTED_EDGE('',*,*,#5444,.F.);
#7120=ORIENTED_EDGE('',*,*,#5449,.F.);
#7121=ORIENTED_EDGE('',*,*,#5450,.T.);
#7122=ORIENTED_EDGE('',*,*,#5451,.T.);
#7123=ORIENTED_EDGE('',*,*,#5447,.F.);
#7124=ORIENTED_EDGE('',*,*,#5452,.F.);
#7125=ORIENTED_EDGE('',*,*,#5453,.T.);
#7126=ORIENTED_EDGE('',*,*,#5454,.T.);
#7127=ORIENTED_EDGE('',*,*,#5450,.F.);
#7128=ORIENTED_EDGE('',*,*,#5455,.F.);
#7129=ORIENTED_EDGE('',*,*,#5456,.T.);
#7130=ORIENTED_EDGE('',*,*,#5457,.T.);
#7131=ORIENTED_EDGE('',*,*,#5453,.F.);
#7132=ORIENTED_EDGE('',*,*,#5458,.F.);
#7133=ORIENTED_EDGE('',*,*,#5459,.T.);
#7134=ORIENTED_EDGE('',*,*,#5460,.T.);
#7135=ORIENTED_EDGE('',*,*,#5456,.F.);
#7136=ORIENTED_EDGE('',*,*,#5461,.F.);
#7137=ORIENTED_EDGE('',*,*,#5462,.T.);
#7138=ORIENTED_EDGE('',*,*,#5463,.T.);
#7139=ORIENTED_EDGE('',*,*,#5459,.F.);
#7140=ORIENTED_EDGE('',*,*,#5464,.F.);
#7141=ORIENTED_EDGE('',*,*,#5465,.F.);
#7142=ORIENTED_EDGE('',*,*,#5466,.F.);
#7143=ORIENTED_EDGE('',*,*,#5467,.F.);
#7144=ORIENTED_EDGE('',*,*,#5468,.T.);
#7145=ORIENTED_EDGE('',*,*,#5469,.T.);
#7146=ORIENTED_EDGE('',*,*,#5470,.T.);
#7147=ORIENTED_EDGE('',*,*,#5471,.T.);
#7148=ORIENTED_EDGE('',*,*,#5472,.T.);
#7149=ORIENTED_EDGE('',*,*,#5473,.T.);
#7150=ORIENTED_EDGE('',*,*,#5472,.F.);
#7151=ORIENTED_EDGE('',*,*,#5474,.T.);
#7152=ORIENTED_EDGE('',*,*,#5475,.T.);
#7153=ORIENTED_EDGE('',*,*,#5476,.T.);
#7154=ORIENTED_EDGE('',*,*,#5477,.T.);
#7155=ORIENTED_EDGE('',*,*,#5469,.F.);
#7156=ORIENTED_EDGE('',*,*,#5478,.T.);
#7157=ORIENTED_EDGE('',*,*,#5479,.T.);
#7158=ORIENTED_EDGE('',*,*,#5480,.T.);
#7159=ORIENTED_EDGE('',*,*,#5476,.F.);
#7160=ORIENTED_EDGE('',*,*,#5481,.T.);
#7161=ORIENTED_EDGE('',*,*,#5482,.T.);
#7162=ORIENTED_EDGE('',*,*,#5483,.T.);
#7163=ORIENTED_EDGE('',*,*,#5479,.F.);
#7164=ORIENTED_EDGE('',*,*,#5484,.T.);
#7165=ORIENTED_EDGE('',*,*,#5485,.T.);
#7166=ORIENTED_EDGE('',*,*,#5486,.T.);
#7167=ORIENTED_EDGE('',*,*,#5482,.F.);
#7168=ORIENTED_EDGE('',*,*,#5487,.T.);
#7169=ORIENTED_EDGE('',*,*,#5488,.T.);
#7170=ORIENTED_EDGE('',*,*,#5489,.T.);
#7171=ORIENTED_EDGE('',*,*,#5485,.F.);
#7172=ORIENTED_EDGE('',*,*,#5490,.T.);
#7173=ORIENTED_EDGE('',*,*,#5491,.T.);
#7174=ORIENTED_EDGE('',*,*,#5492,.T.);
#7175=ORIENTED_EDGE('',*,*,#5488,.F.);
#7176=ORIENTED_EDGE('',*,*,#5493,.T.);
#7177=ORIENTED_EDGE('',*,*,#5494,.T.);
#7178=ORIENTED_EDGE('',*,*,#5495,.T.);
#7179=ORIENTED_EDGE('',*,*,#5491,.F.);
#7180=ORIENTED_EDGE('',*,*,#5496,.T.);
#7181=ORIENTED_EDGE('',*,*,#5497,.T.);
#7182=ORIENTED_EDGE('',*,*,#5498,.T.);
#7183=ORIENTED_EDGE('',*,*,#5494,.F.);
#7184=ORIENTED_EDGE('',*,*,#5499,.T.);
#7185=ORIENTED_EDGE('',*,*,#5500,.T.);
#7186=ORIENTED_EDGE('',*,*,#5501,.T.);
#7187=ORIENTED_EDGE('',*,*,#5497,.F.);
#7188=ORIENTED_EDGE('',*,*,#5502,.T.);
#7189=ORIENTED_EDGE('',*,*,#5503,.T.);
#7190=ORIENTED_EDGE('',*,*,#5504,.T.);
#7191=ORIENTED_EDGE('',*,*,#5500,.F.);
#7192=ORIENTED_EDGE('',*,*,#5505,.T.);
#7193=ORIENTED_EDGE('',*,*,#5506,.T.);
#7194=ORIENTED_EDGE('',*,*,#5507,.T.);
#7195=ORIENTED_EDGE('',*,*,#5503,.F.);
#7196=ORIENTED_EDGE('',*,*,#5508,.T.);
#7197=ORIENTED_EDGE('',*,*,#5509,.T.);
#7198=ORIENTED_EDGE('',*,*,#5510,.T.);
#7199=ORIENTED_EDGE('',*,*,#5506,.F.);
#7200=ORIENTED_EDGE('',*,*,#5511,.T.);
#7201=ORIENTED_EDGE('',*,*,#5512,.T.);
#7202=ORIENTED_EDGE('',*,*,#5513,.T.);
#7203=ORIENTED_EDGE('',*,*,#5509,.F.);
#7204=ORIENTED_EDGE('',*,*,#5514,.T.);
#7205=ORIENTED_EDGE('',*,*,#5515,.F.);
#7206=ORIENTED_EDGE('',*,*,#5516,.T.);
#7207=ORIENTED_EDGE('',*,*,#5517,.F.);
#7208=ORIENTED_EDGE('',*,*,#5518,.T.);
#7209=ORIENTED_EDGE('',*,*,#5519,.T.);
#7210=ORIENTED_EDGE('',*,*,#5520,.T.);
#7211=ORIENTED_EDGE('',*,*,#5521,.F.);
#7212=ORIENTED_EDGE('',*,*,#5522,.F.);
#7213=ORIENTED_EDGE('',*,*,#5523,.T.);
#7214=ORIENTED_EDGE('',*,*,#5524,.T.);
#7215=ORIENTED_EDGE('',*,*,#5519,.F.);
#7216=ORIENTED_EDGE('',*,*,#5525,.F.);
#7217=ORIENTED_EDGE('',*,*,#5526,.T.);
#7218=ORIENTED_EDGE('',*,*,#5527,.T.);
#7219=ORIENTED_EDGE('',*,*,#5523,.F.);
#7220=ORIENTED_EDGE('',*,*,#5528,.F.);
#7221=ORIENTED_EDGE('',*,*,#5529,.T.);
#7222=ORIENTED_EDGE('',*,*,#5530,.T.);
#7223=ORIENTED_EDGE('',*,*,#5526,.F.);
#7224=ORIENTED_EDGE('',*,*,#5531,.F.);
#7225=ORIENTED_EDGE('',*,*,#5532,.T.);
#7226=ORIENTED_EDGE('',*,*,#5533,.T.);
#7227=ORIENTED_EDGE('',*,*,#5529,.F.);
#7228=ORIENTED_EDGE('',*,*,#5534,.F.);
#7229=ORIENTED_EDGE('',*,*,#5535,.T.);
#7230=ORIENTED_EDGE('',*,*,#5536,.T.);
#7231=ORIENTED_EDGE('',*,*,#5532,.F.);
#7232=ORIENTED_EDGE('',*,*,#5537,.F.);
#7233=ORIENTED_EDGE('',*,*,#5538,.T.);
#7234=ORIENTED_EDGE('',*,*,#5539,.T.);
#7235=ORIENTED_EDGE('',*,*,#5535,.F.);
#7236=ORIENTED_EDGE('',*,*,#5540,.F.);
#7237=ORIENTED_EDGE('',*,*,#5541,.T.);
#7238=ORIENTED_EDGE('',*,*,#5542,.T.);
#7239=ORIENTED_EDGE('',*,*,#5538,.F.);
#7240=ORIENTED_EDGE('',*,*,#5543,.F.);
#7241=ORIENTED_EDGE('',*,*,#5544,.T.);
#7242=ORIENTED_EDGE('',*,*,#5545,.T.);
#7243=ORIENTED_EDGE('',*,*,#5541,.F.);
#7244=ORIENTED_EDGE('',*,*,#5546,.F.);
#7245=ORIENTED_EDGE('',*,*,#5547,.T.);
#7246=ORIENTED_EDGE('',*,*,#5548,.T.);
#7247=ORIENTED_EDGE('',*,*,#5544,.F.);
#7248=ORIENTED_EDGE('',*,*,#5549,.F.);
#7249=ORIENTED_EDGE('',*,*,#5550,.T.);
#7250=ORIENTED_EDGE('',*,*,#5551,.T.);
#7251=ORIENTED_EDGE('',*,*,#5547,.F.);
#7252=ORIENTED_EDGE('',*,*,#5552,.F.);
#7253=ORIENTED_EDGE('',*,*,#5553,.T.);
#7254=ORIENTED_EDGE('',*,*,#5554,.T.);
#7255=ORIENTED_EDGE('',*,*,#5550,.F.);
#7256=ORIENTED_EDGE('',*,*,#5555,.F.);
#7257=ORIENTED_EDGE('',*,*,#5556,.T.);
#7258=ORIENTED_EDGE('',*,*,#5557,.T.);
#7259=ORIENTED_EDGE('',*,*,#5553,.F.);
#7260=ORIENTED_EDGE('',*,*,#5558,.F.);
#7261=ORIENTED_EDGE('',*,*,#5559,.T.);
#7262=ORIENTED_EDGE('',*,*,#5560,.T.);
#7263=ORIENTED_EDGE('',*,*,#5556,.F.);
#7264=ORIENTED_EDGE('',*,*,#5561,.F.);
#7265=ORIENTED_EDGE('',*,*,#5562,.F.);
#7266=ORIENTED_EDGE('',*,*,#5563,.F.);
#7267=ORIENTED_EDGE('',*,*,#5564,.F.);
#7268=ORIENTED_EDGE('',*,*,#5565,.T.);
#7269=ORIENTED_EDGE('',*,*,#5566,.T.);
#7270=ORIENTED_EDGE('',*,*,#5567,.T.);
#7271=ORIENTED_EDGE('',*,*,#5568,.T.);
#7272=ORIENTED_EDGE('',*,*,#5569,.T.);
#7273=ORIENTED_EDGE('',*,*,#5570,.T.);
#7274=ORIENTED_EDGE('',*,*,#5569,.F.);
#7275=ORIENTED_EDGE('',*,*,#5571,.T.);
#7276=ORIENTED_EDGE('',*,*,#5572,.T.);
#7277=ORIENTED_EDGE('',*,*,#5573,.T.);
#7278=ORIENTED_EDGE('',*,*,#5574,.T.);
#7279=ORIENTED_EDGE('',*,*,#5566,.F.);
#7280=ORIENTED_EDGE('',*,*,#5575,.T.);
#7281=ORIENTED_EDGE('',*,*,#5576,.T.);
#7282=ORIENTED_EDGE('',*,*,#5577,.T.);
#7283=ORIENTED_EDGE('',*,*,#5573,.F.);
#7284=ORIENTED_EDGE('',*,*,#5578,.T.);
#7285=ORIENTED_EDGE('',*,*,#5579,.T.);
#7286=ORIENTED_EDGE('',*,*,#5580,.T.);
#7287=ORIENTED_EDGE('',*,*,#5576,.F.);
#7288=ORIENTED_EDGE('',*,*,#5581,.T.);
#7289=ORIENTED_EDGE('',*,*,#5582,.T.);
#7290=ORIENTED_EDGE('',*,*,#5583,.T.);
#7291=ORIENTED_EDGE('',*,*,#5579,.F.);
#7292=ORIENTED_EDGE('',*,*,#5584,.T.);
#7293=ORIENTED_EDGE('',*,*,#5585,.T.);
#7294=ORIENTED_EDGE('',*,*,#5586,.T.);
#7295=ORIENTED_EDGE('',*,*,#5582,.F.);
#7296=ORIENTED_EDGE('',*,*,#5587,.T.);
#7297=ORIENTED_EDGE('',*,*,#5588,.T.);
#7298=ORIENTED_EDGE('',*,*,#5589,.T.);
#7299=ORIENTED_EDGE('',*,*,#5585,.F.);
#7300=ORIENTED_EDGE('',*,*,#5590,.T.);
#7301=ORIENTED_EDGE('',*,*,#5591,.T.);
#7302=ORIENTED_EDGE('',*,*,#5592,.T.);
#7303=ORIENTED_EDGE('',*,*,#5588,.F.);
#7304=ORIENTED_EDGE('',*,*,#5593,.T.);
#7305=ORIENTED_EDGE('',*,*,#5594,.T.);
#7306=ORIENTED_EDGE('',*,*,#5595,.T.);
#7307=ORIENTED_EDGE('',*,*,#5591,.F.);
#7308=ORIENTED_EDGE('',*,*,#5596,.T.);
#7309=ORIENTED_EDGE('',*,*,#5597,.T.);
#7310=ORIENTED_EDGE('',*,*,#5598,.T.);
#7311=ORIENTED_EDGE('',*,*,#5594,.F.);
#7312=ORIENTED_EDGE('',*,*,#5599,.T.);
#7313=ORIENTED_EDGE('',*,*,#5600,.T.);
#7314=ORIENTED_EDGE('',*,*,#5601,.T.);
#7315=ORIENTED_EDGE('',*,*,#5597,.F.);
#7316=ORIENTED_EDGE('',*,*,#5602,.T.);
#7317=ORIENTED_EDGE('',*,*,#5603,.T.);
#7318=ORIENTED_EDGE('',*,*,#5604,.T.);
#7319=ORIENTED_EDGE('',*,*,#5600,.F.);
#7320=ORIENTED_EDGE('',*,*,#5605,.T.);
#7321=ORIENTED_EDGE('',*,*,#5606,.T.);
#7322=ORIENTED_EDGE('',*,*,#5607,.T.);
#7323=ORIENTED_EDGE('',*,*,#5603,.F.);
#7324=ORIENTED_EDGE('',*,*,#5608,.T.);
#7325=ORIENTED_EDGE('',*,*,#5609,.T.);
#7326=ORIENTED_EDGE('',*,*,#5610,.T.);
#7327=ORIENTED_EDGE('',*,*,#5606,.F.);
#7328=ORIENTED_EDGE('',*,*,#5611,.T.);
#7329=ORIENTED_EDGE('',*,*,#5612,.F.);
#7330=ORIENTED_EDGE('',*,*,#5613,.T.);
#7331=ORIENTED_EDGE('',*,*,#5614,.F.);
#7332=ORIENTED_EDGE('',*,*,#5615,.T.);
#7333=ORIENTED_EDGE('',*,*,#5616,.T.);
#7334=ORIENTED_EDGE('',*,*,#5617,.T.);
#7335=ORIENTED_EDGE('',*,*,#5618,.F.);
#7336=ORIENTED_EDGE('',*,*,#5619,.F.);
#7337=ORIENTED_EDGE('',*,*,#5620,.T.);
#7338=ORIENTED_EDGE('',*,*,#5621,.T.);
#7339=ORIENTED_EDGE('',*,*,#5616,.F.);
#7340=ORIENTED_EDGE('',*,*,#5622,.F.);
#7341=ORIENTED_EDGE('',*,*,#5623,.T.);
#7342=ORIENTED_EDGE('',*,*,#5624,.T.);
#7343=ORIENTED_EDGE('',*,*,#5620,.F.);
#7344=ORIENTED_EDGE('',*,*,#5625,.F.);
#7345=ORIENTED_EDGE('',*,*,#5626,.T.);
#7346=ORIENTED_EDGE('',*,*,#5627,.T.);
#7347=ORIENTED_EDGE('',*,*,#5623,.F.);
#7348=ORIENTED_EDGE('',*,*,#5628,.F.);
#7349=ORIENTED_EDGE('',*,*,#5629,.T.);
#7350=ORIENTED_EDGE('',*,*,#5630,.T.);
#7351=ORIENTED_EDGE('',*,*,#5626,.F.);
#7352=ORIENTED_EDGE('',*,*,#5631,.F.);
#7353=ORIENTED_EDGE('',*,*,#5632,.T.);
#7354=ORIENTED_EDGE('',*,*,#5633,.T.);
#7355=ORIENTED_EDGE('',*,*,#5629,.F.);
#7356=ORIENTED_EDGE('',*,*,#5634,.F.);
#7357=ORIENTED_EDGE('',*,*,#5635,.T.);
#7358=ORIENTED_EDGE('',*,*,#5636,.T.);
#7359=ORIENTED_EDGE('',*,*,#5632,.F.);
#7360=ORIENTED_EDGE('',*,*,#5637,.F.);
#7361=ORIENTED_EDGE('',*,*,#5638,.T.);
#7362=ORIENTED_EDGE('',*,*,#5639,.T.);
#7363=ORIENTED_EDGE('',*,*,#5635,.F.);
#7364=ORIENTED_EDGE('',*,*,#5640,.F.);
#7365=ORIENTED_EDGE('',*,*,#5641,.T.);
#7366=ORIENTED_EDGE('',*,*,#5642,.T.);
#7367=ORIENTED_EDGE('',*,*,#5638,.F.);
#7368=ORIENTED_EDGE('',*,*,#5643,.F.);
#7369=ORIENTED_EDGE('',*,*,#5644,.T.);
#7370=ORIENTED_EDGE('',*,*,#5645,.T.);
#7371=ORIENTED_EDGE('',*,*,#5641,.F.);
#7372=ORIENTED_EDGE('',*,*,#5646,.F.);
#7373=ORIENTED_EDGE('',*,*,#5647,.T.);
#7374=ORIENTED_EDGE('',*,*,#5648,.T.);
#7375=ORIENTED_EDGE('',*,*,#5644,.F.);
#7376=ORIENTED_EDGE('',*,*,#5649,.F.);
#7377=ORIENTED_EDGE('',*,*,#5650,.T.);
#7378=ORIENTED_EDGE('',*,*,#5651,.T.);
#7379=ORIENTED_EDGE('',*,*,#5647,.F.);
#7380=ORIENTED_EDGE('',*,*,#5652,.F.);
#7381=ORIENTED_EDGE('',*,*,#5653,.T.);
#7382=ORIENTED_EDGE('',*,*,#5654,.T.);
#7383=ORIENTED_EDGE('',*,*,#5650,.F.);
#7384=ORIENTED_EDGE('',*,*,#5655,.F.);
#7385=ORIENTED_EDGE('',*,*,#5656,.T.);
#7386=ORIENTED_EDGE('',*,*,#5657,.T.);
#7387=ORIENTED_EDGE('',*,*,#5653,.F.);
#7388=ORIENTED_EDGE('',*,*,#5658,.F.);
#7389=ORIENTED_EDGE('',*,*,#5659,.F.);
#7390=ORIENTED_EDGE('',*,*,#5660,.F.);
#7391=ORIENTED_EDGE('',*,*,#5661,.F.);
#7392=ORIENTED_EDGE('',*,*,#5662,.T.);
#7393=ORIENTED_EDGE('',*,*,#5663,.T.);
#7394=ORIENTED_EDGE('',*,*,#5664,.T.);
#7395=ORIENTED_EDGE('',*,*,#5665,.T.);
#7396=ORIENTED_EDGE('',*,*,#5666,.T.);
#7397=ORIENTED_EDGE('',*,*,#5667,.T.);
#7398=ORIENTED_EDGE('',*,*,#5668,.T.);
#7399=ORIENTED_EDGE('',*,*,#5663,.F.);
#7400=ORIENTED_EDGE('',*,*,#5669,.T.);
#7401=ORIENTED_EDGE('',*,*,#5670,.T.);
#7402=ORIENTED_EDGE('',*,*,#5671,.T.);
#7403=ORIENTED_EDGE('',*,*,#5667,.F.);
#7404=ORIENTED_EDGE('',*,*,#5672,.T.);
#7405=ORIENTED_EDGE('',*,*,#5673,.T.);
#7406=ORIENTED_EDGE('',*,*,#5674,.T.);
#7407=ORIENTED_EDGE('',*,*,#5670,.F.);
#7408=ORIENTED_EDGE('',*,*,#5675,.T.);
#7409=ORIENTED_EDGE('',*,*,#5676,.T.);
#7410=ORIENTED_EDGE('',*,*,#5677,.T.);
#7411=ORIENTED_EDGE('',*,*,#5673,.F.);
#7412=ORIENTED_EDGE('',*,*,#5678,.T.);
#7413=ORIENTED_EDGE('',*,*,#5679,.T.);
#7414=ORIENTED_EDGE('',*,*,#5680,.T.);
#7415=ORIENTED_EDGE('',*,*,#5676,.F.);
#7416=ORIENTED_EDGE('',*,*,#5681,.T.);
#7417=ORIENTED_EDGE('',*,*,#5682,.T.);
#7418=ORIENTED_EDGE('',*,*,#5683,.T.);
#7419=ORIENTED_EDGE('',*,*,#5679,.F.);
#7420=ORIENTED_EDGE('',*,*,#5684,.T.);
#7421=ORIENTED_EDGE('',*,*,#5685,.F.);
#7422=ORIENTED_EDGE('',*,*,#5686,.T.);
#7423=ORIENTED_EDGE('',*,*,#5687,.F.);
#7424=ORIENTED_EDGE('',*,*,#5688,.T.);
#7425=ORIENTED_EDGE('',*,*,#5689,.T.);
#7426=ORIENTED_EDGE('',*,*,#5690,.T.);
#7427=ORIENTED_EDGE('',*,*,#5691,.F.);
#7428=ORIENTED_EDGE('',*,*,#5692,.F.);
#7429=ORIENTED_EDGE('',*,*,#5693,.T.);
#7430=ORIENTED_EDGE('',*,*,#5694,.T.);
#7431=ORIENTED_EDGE('',*,*,#5689,.F.);
#7432=ORIENTED_EDGE('',*,*,#5695,.F.);
#7433=ORIENTED_EDGE('',*,*,#5696,.T.);
#7434=ORIENTED_EDGE('',*,*,#5697,.T.);
#7435=ORIENTED_EDGE('',*,*,#5693,.F.);
#7436=ORIENTED_EDGE('',*,*,#5698,.F.);
#7437=ORIENTED_EDGE('',*,*,#5699,.T.);
#7438=ORIENTED_EDGE('',*,*,#5700,.T.);
#7439=ORIENTED_EDGE('',*,*,#5696,.F.);
#7440=ORIENTED_EDGE('',*,*,#5701,.F.);
#7441=ORIENTED_EDGE('',*,*,#5702,.T.);
#7442=ORIENTED_EDGE('',*,*,#5703,.T.);
#7443=ORIENTED_EDGE('',*,*,#5699,.F.);
#7444=ORIENTED_EDGE('',*,*,#5704,.F.);
#7445=ORIENTED_EDGE('',*,*,#5705,.T.);
#7446=ORIENTED_EDGE('',*,*,#5706,.T.);
#7447=ORIENTED_EDGE('',*,*,#5702,.F.);
#7448=ORIENTED_EDGE('',*,*,#5707,.F.);
#7449=ORIENTED_EDGE('',*,*,#5708,.T.);
#7450=ORIENTED_EDGE('',*,*,#5709,.T.);
#7451=ORIENTED_EDGE('',*,*,#5705,.F.);
#7452=ORIENTED_EDGE('',*,*,#5710,.F.);
#7453=ORIENTED_EDGE('',*,*,#5711,.F.);
#7454=ORIENTED_EDGE('',*,*,#5712,.F.);
#7455=ORIENTED_EDGE('',*,*,#5713,.F.);
#7456=ORIENTED_EDGE('',*,*,#5714,.T.);
#7457=ORIENTED_EDGE('',*,*,#5711,.T.);
#7458=ORIENTED_EDGE('',*,*,#5715,.T.);
#7459=ORIENTED_EDGE('',*,*,#5708,.F.);
#7460=ORIENTED_EDGE('',*,*,#5716,.F.);
#7461=ORIENTED_EDGE('',*,*,#5717,.F.);
#7462=ORIENTED_EDGE('',*,*,#5690,.F.);
#7463=ORIENTED_EDGE('',*,*,#5694,.F.);
#7464=ORIENTED_EDGE('',*,*,#5697,.F.);
#7465=ORIENTED_EDGE('',*,*,#5700,.F.);
#7466=ORIENTED_EDGE('',*,*,#5703,.F.);
#7467=ORIENTED_EDGE('',*,*,#5706,.F.);
#7468=ORIENTED_EDGE('',*,*,#5709,.F.);
#7469=ORIENTED_EDGE('',*,*,#5715,.F.);
#7470=ORIENTED_EDGE('',*,*,#5714,.F.);
#7471=ORIENTED_EDGE('',*,*,#5718,.F.);
#7472=ORIENTED_EDGE('',*,*,#5664,.F.);
#7473=ORIENTED_EDGE('',*,*,#5668,.F.);
#7474=ORIENTED_EDGE('',*,*,#5671,.F.);
#7475=ORIENTED_EDGE('',*,*,#5674,.F.);
#7476=ORIENTED_EDGE('',*,*,#5677,.F.);
#7477=ORIENTED_EDGE('',*,*,#5680,.F.);
#7478=ORIENTED_EDGE('',*,*,#5683,.F.);
#7479=ORIENTED_EDGE('',*,*,#5719,.F.);
#7480=ORIENTED_EDGE('',*,*,#5688,.F.);
#7481=ORIENTED_EDGE('',*,*,#5720,.F.);
#7482=ORIENTED_EDGE('',*,*,#5686,.F.);
#7483=ORIENTED_EDGE('',*,*,#5721,.F.);
#7484=ORIENTED_EDGE('',*,*,#5684,.F.);
#7485=ORIENTED_EDGE('',*,*,#5681,.F.);
#7486=ORIENTED_EDGE('',*,*,#5678,.F.);
#7487=ORIENTED_EDGE('',*,*,#5675,.F.);
#7488=ORIENTED_EDGE('',*,*,#5672,.F.);
#7489=ORIENTED_EDGE('',*,*,#5669,.F.);
#7490=ORIENTED_EDGE('',*,*,#5666,.F.);
#7491=ORIENTED_EDGE('',*,*,#5722,.F.);
#7492=ORIENTED_EDGE('',*,*,#5712,.T.);
#7493=ORIENTED_EDGE('',*,*,#5716,.T.);
#7494=ORIENTED_EDGE('',*,*,#5710,.T.);
#7495=ORIENTED_EDGE('',*,*,#5707,.T.);
#7496=ORIENTED_EDGE('',*,*,#5704,.T.);
#7497=ORIENTED_EDGE('',*,*,#5701,.T.);
#7498=ORIENTED_EDGE('',*,*,#5698,.T.);
#7499=ORIENTED_EDGE('',*,*,#5695,.T.);
#7500=ORIENTED_EDGE('',*,*,#5692,.T.);
#7501=ORIENTED_EDGE('',*,*,#5723,.F.);
#7502=ORIENTED_EDGE('',*,*,#5718,.T.);
#7503=ORIENTED_EDGE('',*,*,#5713,.T.);
#7504=ORIENTED_EDGE('',*,*,#5722,.T.);
#7505=ORIENTED_EDGE('',*,*,#5665,.F.);
#7506=ORIENTED_EDGE('',*,*,#5685,.T.);
#7507=ORIENTED_EDGE('',*,*,#5719,.T.);
#7508=ORIENTED_EDGE('',*,*,#5682,.F.);
#7509=ORIENTED_EDGE('',*,*,#5721,.T.);
#7510=ORIENTED_EDGE('',*,*,#5724,.F.);
#7511=ORIENTED_EDGE('',*,*,#5725,.T.);
#7512=ORIENTED_EDGE('',*,*,#5723,.T.);
#7513=ORIENTED_EDGE('',*,*,#5725,.F.);
#7514=ORIENTED_EDGE('',*,*,#5726,.F.);
#7515=ORIENTED_EDGE('',*,*,#5727,.F.);
#7516=ORIENTED_EDGE('',*,*,#5728,.F.);
#7517=ORIENTED_EDGE('',*,*,#5729,.F.);
#7518=ORIENTED_EDGE('',*,*,#5730,.T.);
#7519=ORIENTED_EDGE('',*,*,#5373,.T.);
#7520=ORIENTED_EDGE('',*,*,#5731,.T.);
#7521=ORIENTED_EDGE('',*,*,#5420,.T.);
#7522=ORIENTED_EDGE('',*,*,#5732,.T.);
#7523=ORIENTED_EDGE('',*,*,#5324,.T.);
#7524=ORIENTED_EDGE('',*,*,#5733,.T.);
#7525=ORIENTED_EDGE('',*,*,#5467,.T.);
#7526=ORIENTED_EDGE('',*,*,#5734,.T.);
#7527=ORIENTED_EDGE('',*,*,#5517,.T.);
#7528=ORIENTED_EDGE('',*,*,#5735,.T.);
#7529=ORIENTED_EDGE('',*,*,#5564,.T.);
#7530=ORIENTED_EDGE('',*,*,#5736,.T.);
#7531=ORIENTED_EDGE('',*,*,#5614,.T.);
#7532=ORIENTED_EDGE('',*,*,#5737,.T.);
#7533=ORIENTED_EDGE('',*,*,#5661,.T.);
#7534=ORIENTED_EDGE('',*,*,#5724,.T.);
#7535=ORIENTED_EDGE('',*,*,#5568,.F.);
#7536=ORIENTED_EDGE('',*,*,#5738,.T.);
#7537=ORIENTED_EDGE('',*,*,#5618,.T.);
#7538=ORIENTED_EDGE('',*,*,#5739,.T.);
#7539=ORIENTED_EDGE('',*,*,#5571,.F.);
#7540=ORIENTED_EDGE('',*,*,#5659,.T.);
#7541=ORIENTED_EDGE('',*,*,#5740,.T.);
#7542=ORIENTED_EDGE('',*,*,#5656,.F.);
#7543=ORIENTED_EDGE('',*,*,#5741,.F.);
#7544=ORIENTED_EDGE('',*,*,#5739,.F.);
#7545=ORIENTED_EDGE('',*,*,#5617,.F.);
#7546=ORIENTED_EDGE('',*,*,#5621,.F.);
#7547=ORIENTED_EDGE('',*,*,#5624,.F.);
#7548=ORIENTED_EDGE('',*,*,#5627,.F.);
#7549=ORIENTED_EDGE('',*,*,#5630,.F.);
#7550=ORIENTED_EDGE('',*,*,#5633,.F.);
#7551=ORIENTED_EDGE('',*,*,#5636,.F.);
#7552=ORIENTED_EDGE('',*,*,#5639,.F.);
#7553=ORIENTED_EDGE('',*,*,#5642,.F.);
#7554=ORIENTED_EDGE('',*,*,#5645,.F.);
#7555=ORIENTED_EDGE('',*,*,#5648,.F.);
#7556=ORIENTED_EDGE('',*,*,#5651,.F.);
#7557=ORIENTED_EDGE('',*,*,#5654,.F.);
#7558=ORIENTED_EDGE('',*,*,#5657,.F.);
#7559=ORIENTED_EDGE('',*,*,#5740,.F.);
#7560=ORIENTED_EDGE('',*,*,#5662,.F.);
#7561=ORIENTED_EDGE('',*,*,#5737,.F.);
#7562=ORIENTED_EDGE('',*,*,#5613,.F.);
#7563=ORIENTED_EDGE('',*,*,#5742,.F.);
#7564=ORIENTED_EDGE('',*,*,#5611,.F.);
#7565=ORIENTED_EDGE('',*,*,#5608,.F.);
#7566=ORIENTED_EDGE('',*,*,#5605,.F.);
#7567=ORIENTED_EDGE('',*,*,#5602,.F.);
#7568=ORIENTED_EDGE('',*,*,#5599,.F.);
#7569=ORIENTED_EDGE('',*,*,#5596,.F.);
#7570=ORIENTED_EDGE('',*,*,#5593,.F.);
#7571=ORIENTED_EDGE('',*,*,#5590,.F.);
#7572=ORIENTED_EDGE('',*,*,#5587,.F.);
#7573=ORIENTED_EDGE('',*,*,#5584,.F.);
#7574=ORIENTED_EDGE('',*,*,#5581,.F.);
#7575=ORIENTED_EDGE('',*,*,#5578,.F.);
#7576=ORIENTED_EDGE('',*,*,#5575,.F.);
#7577=ORIENTED_EDGE('',*,*,#5572,.F.);
#7578=ORIENTED_EDGE('',*,*,#5738,.F.);
#7579=ORIENTED_EDGE('',*,*,#5567,.F.);
#7580=ORIENTED_EDGE('',*,*,#5574,.F.);
#7581=ORIENTED_EDGE('',*,*,#5577,.F.);
#7582=ORIENTED_EDGE('',*,*,#5580,.F.);
#7583=ORIENTED_EDGE('',*,*,#5583,.F.);
#7584=ORIENTED_EDGE('',*,*,#5586,.F.);
#7585=ORIENTED_EDGE('',*,*,#5589,.F.);
#7586=ORIENTED_EDGE('',*,*,#5592,.F.);
#7587=ORIENTED_EDGE('',*,*,#5595,.F.);
#7588=ORIENTED_EDGE('',*,*,#5598,.F.);
#7589=ORIENTED_EDGE('',*,*,#5601,.F.);
#7590=ORIENTED_EDGE('',*,*,#5604,.F.);
#7591=ORIENTED_EDGE('',*,*,#5607,.F.);
#7592=ORIENTED_EDGE('',*,*,#5610,.F.);
#7593=ORIENTED_EDGE('',*,*,#5743,.F.);
#7594=ORIENTED_EDGE('',*,*,#5615,.F.);
#7595=ORIENTED_EDGE('',*,*,#5736,.F.);
#7596=ORIENTED_EDGE('',*,*,#5660,.T.);
#7597=ORIENTED_EDGE('',*,*,#5741,.T.);
#7598=ORIENTED_EDGE('',*,*,#5658,.T.);
#7599=ORIENTED_EDGE('',*,*,#5655,.T.);
#7600=ORIENTED_EDGE('',*,*,#5652,.T.);
#7601=ORIENTED_EDGE('',*,*,#5649,.T.);
#7602=ORIENTED_EDGE('',*,*,#5646,.T.);
#7603=ORIENTED_EDGE('',*,*,#5643,.T.);
#7604=ORIENTED_EDGE('',*,*,#5640,.T.);
#7605=ORIENTED_EDGE('',*,*,#5637,.T.);
#7606=ORIENTED_EDGE('',*,*,#5634,.T.);
#7607=ORIENTED_EDGE('',*,*,#5631,.T.);
#7608=ORIENTED_EDGE('',*,*,#5628,.T.);
#7609=ORIENTED_EDGE('',*,*,#5625,.T.);
#7610=ORIENTED_EDGE('',*,*,#5622,.T.);
#7611=ORIENTED_EDGE('',*,*,#5619,.T.);
#7612=ORIENTED_EDGE('',*,*,#5612,.T.);
#7613=ORIENTED_EDGE('',*,*,#5743,.T.);
#7614=ORIENTED_EDGE('',*,*,#5609,.F.);
#7615=ORIENTED_EDGE('',*,*,#5742,.T.);
#7616=ORIENTED_EDGE('',*,*,#5471,.F.);
#7617=ORIENTED_EDGE('',*,*,#5744,.T.);
#7618=ORIENTED_EDGE('',*,*,#5521,.T.);
#7619=ORIENTED_EDGE('',*,*,#5745,.T.);
#7620=ORIENTED_EDGE('',*,*,#5474,.F.);
#7621=ORIENTED_EDGE('',*,*,#5562,.T.);
#7622=ORIENTED_EDGE('',*,*,#5746,.T.);
#7623=ORIENTED_EDGE('',*,*,#5559,.F.);
#7624=ORIENTED_EDGE('',*,*,#5747,.F.);
#7625=ORIENTED_EDGE('',*,*,#5745,.F.);
#7626=ORIENTED_EDGE('',*,*,#5520,.F.);
#7627=ORIENTED_EDGE('',*,*,#5524,.F.);
#7628=ORIENTED_EDGE('',*,*,#5527,.F.);
#7629=ORIENTED_EDGE('',*,*,#5530,.F.);
#7630=ORIENTED_EDGE('',*,*,#5533,.F.);
#7631=ORIENTED_EDGE('',*,*,#5536,.F.);
#7632=ORIENTED_EDGE('',*,*,#5539,.F.);
#7633=ORIENTED_EDGE('',*,*,#5542,.F.);
#7634=ORIENTED_EDGE('',*,*,#5545,.F.);
#7635=ORIENTED_EDGE('',*,*,#5548,.F.);
#7636=ORIENTED_EDGE('',*,*,#5551,.F.);
#7637=ORIENTED_EDGE('',*,*,#5554,.F.);
#7638=ORIENTED_EDGE('',*,*,#5557,.F.);
#7639=ORIENTED_EDGE('',*,*,#5560,.F.);
#7640=ORIENTED_EDGE('',*,*,#5746,.F.);
#7641=ORIENTED_EDGE('',*,*,#5565,.F.);
#7642=ORIENTED_EDGE('',*,*,#5735,.F.);
#7643=ORIENTED_EDGE('',*,*,#5516,.F.);
#7644=ORIENTED_EDGE('',*,*,#5748,.F.);
#7645=ORIENTED_EDGE('',*,*,#5514,.F.);
#7646=ORIENTED_EDGE('',*,*,#5511,.F.);
#7647=ORIENTED_EDGE('',*,*,#5508,.F.);
#7648=ORIENTED_EDGE('',*,*,#5505,.F.);
#7649=ORIENTED_EDGE('',*,*,#5502,.F.);
#7650=ORIENTED_EDGE('',*,*,#5499,.F.);
#7651=ORIENTED_EDGE('',*,*,#5496,.F.);
#7652=ORIENTED_EDGE('',*,*,#5493,.F.);
#7653=ORIENTED_EDGE('',*,*,#5490,.F.);
#7654=ORIENTED_EDGE('',*,*,#5487,.F.);
#7655=ORIENTED_EDGE('',*,*,#5484,.F.);
#7656=ORIENTED_EDGE('',*,*,#5481,.F.);
#7657=ORIENTED_EDGE('',*,*,#5478,.F.);
#7658=ORIENTED_EDGE('',*,*,#5475,.F.);
#7659=ORIENTED_EDGE('',*,*,#5744,.F.);
#7660=ORIENTED_EDGE('',*,*,#5470,.F.);
#7661=ORIENTED_EDGE('',*,*,#5477,.F.);
#7662=ORIENTED_EDGE('',*,*,#5480,.F.);
#7663=ORIENTED_EDGE('',*,*,#5483,.F.);
#7664=ORIENTED_EDGE('',*,*,#5486,.F.);
#7665=ORIENTED_EDGE('',*,*,#5489,.F.);
#7666=ORIENTED_EDGE('',*,*,#5492,.F.);
#7667=ORIENTED_EDGE('',*,*,#5495,.F.);
#7668=ORIENTED_EDGE('',*,*,#5498,.F.);
#7669=ORIENTED_EDGE('',*,*,#5501,.F.);
#7670=ORIENTED_EDGE('',*,*,#5504,.F.);
#7671=ORIENTED_EDGE('',*,*,#5507,.F.);
#7672=ORIENTED_EDGE('',*,*,#5510,.F.);
#7673=ORIENTED_EDGE('',*,*,#5513,.F.);
#7674=ORIENTED_EDGE('',*,*,#5749,.F.);
#7675=ORIENTED_EDGE('',*,*,#5518,.F.);
#7676=ORIENTED_EDGE('',*,*,#5734,.F.);
#7677=ORIENTED_EDGE('',*,*,#5563,.T.);
#7678=ORIENTED_EDGE('',*,*,#5747,.T.);
#7679=ORIENTED_EDGE('',*,*,#5561,.T.);
#7680=ORIENTED_EDGE('',*,*,#5558,.T.);
#7681=ORIENTED_EDGE('',*,*,#5555,.T.);
#7682=ORIENTED_EDGE('',*,*,#5552,.T.);
#7683=ORIENTED_EDGE('',*,*,#5549,.T.);
#7684=ORIENTED_EDGE('',*,*,#5546,.T.);
#7685=ORIENTED_EDGE('',*,*,#5543,.T.);
#7686=ORIENTED_EDGE('',*,*,#5540,.T.);
#7687=ORIENTED_EDGE('',*,*,#5537,.T.);
#7688=ORIENTED_EDGE('',*,*,#5534,.T.);
#7689=ORIENTED_EDGE('',*,*,#5531,.T.);
#7690=ORIENTED_EDGE('',*,*,#5528,.T.);
#7691=ORIENTED_EDGE('',*,*,#5525,.T.);
#7692=ORIENTED_EDGE('',*,*,#5522,.T.);
#7693=ORIENTED_EDGE('',*,*,#5515,.T.);
#7694=ORIENTED_EDGE('',*,*,#5749,.T.);
#7695=ORIENTED_EDGE('',*,*,#5512,.F.);
#7696=ORIENTED_EDGE('',*,*,#5748,.T.);
#7697=ORIENTED_EDGE('',*,*,#5750,.F.);
#7698=ORIENTED_EDGE('',*,*,#5751,.T.);
#7699=ORIENTED_EDGE('',*,*,#5281,.F.);
#7700=ORIENTED_EDGE('',*,*,#5752,.T.);
#7701=ORIENTED_EDGE('',*,*,#5753,.T.);
#7702=ORIENTED_EDGE('',*,*,#5424,.T.);
#7703=ORIENTED_EDGE('',*,*,#5754,.T.);
#7704=ORIENTED_EDGE('',*,*,#5755,.T.);
#7705=ORIENTED_EDGE('',*,*,#5756,.F.);
#7706=ORIENTED_EDGE('',*,*,#5757,.F.);
#7707=ORIENTED_EDGE('',*,*,#5279,.F.);
#7708=ORIENTED_EDGE('',*,*,#5758,.T.);
#7709=ORIENTED_EDGE('',*,*,#5465,.T.);
#7710=ORIENTED_EDGE('',*,*,#5759,.T.);
#7711=ORIENTED_EDGE('',*,*,#5462,.F.);
#7712=ORIENTED_EDGE('',*,*,#5760,.F.);
#7713=ORIENTED_EDGE('',*,*,#5754,.F.);
#7714=ORIENTED_EDGE('',*,*,#5423,.F.);
#7715=ORIENTED_EDGE('',*,*,#5427,.F.);
#7716=ORIENTED_EDGE('',*,*,#5430,.F.);
#7717=ORIENTED_EDGE('',*,*,#5433,.F.);
#7718=ORIENTED_EDGE('',*,*,#5436,.F.);
#7719=ORIENTED_EDGE('',*,*,#5439,.F.);
#7720=ORIENTED_EDGE('',*,*,#5442,.F.);
#7721=ORIENTED_EDGE('',*,*,#5445,.F.);
#7722=ORIENTED_EDGE('',*,*,#5448,.F.);
#7723=ORIENTED_EDGE('',*,*,#5451,.F.);
#7724=ORIENTED_EDGE('',*,*,#5454,.F.);
#7725=ORIENTED_EDGE('',*,*,#5457,.F.);
#7726=ORIENTED_EDGE('',*,*,#5460,.F.);
#7727=ORIENTED_EDGE('',*,*,#5463,.F.);
#7728=ORIENTED_EDGE('',*,*,#5759,.F.);
#7729=ORIENTED_EDGE('',*,*,#5468,.F.);
#7730=ORIENTED_EDGE('',*,*,#5733,.F.);
#7731=ORIENTED_EDGE('',*,*,#5323,.F.);
#7732=ORIENTED_EDGE('',*,*,#5761,.F.);
#7733=ORIENTED_EDGE('',*,*,#5321,.F.);
#7734=ORIENTED_EDGE('',*,*,#5318,.F.);
#7735=ORIENTED_EDGE('',*,*,#5315,.F.);
#7736=ORIENTED_EDGE('',*,*,#5312,.F.);
#7737=ORIENTED_EDGE('',*,*,#5309,.F.);
#7738=ORIENTED_EDGE('',*,*,#5306,.F.);
#7739=ORIENTED_EDGE('',*,*,#5303,.F.);
#7740=ORIENTED_EDGE('',*,*,#5300,.F.);
#7741=ORIENTED_EDGE('',*,*,#5297,.F.);
#7742=ORIENTED_EDGE('',*,*,#5294,.F.);
#7743=ORIENTED_EDGE('',*,*,#5291,.F.);
#7744=ORIENTED_EDGE('',*,*,#5288,.F.);
#7745=ORIENTED_EDGE('',*,*,#5285,.F.);
#7746=ORIENTED_EDGE('',*,*,#5282,.F.);
#7747=ORIENTED_EDGE('',*,*,#5751,.F.);
#7748=ORIENTED_EDGE('',*,*,#5758,.F.);
#7749=ORIENTED_EDGE('',*,*,#5278,.F.);
#7750=ORIENTED_EDGE('',*,*,#5284,.F.);
#7751=ORIENTED_EDGE('',*,*,#5287,.F.);
#7752=ORIENTED_EDGE('',*,*,#5290,.F.);
#7753=ORIENTED_EDGE('',*,*,#5293,.F.);
#7754=ORIENTED_EDGE('',*,*,#5296,.F.);
#7755=ORIENTED_EDGE('',*,*,#5299,.F.);
#7756=ORIENTED_EDGE('',*,*,#5302,.F.);
#7757=ORIENTED_EDGE('',*,*,#5305,.F.);
#7758=ORIENTED_EDGE('',*,*,#5308,.F.);
#7759=ORIENTED_EDGE('',*,*,#5311,.F.);
#7760=ORIENTED_EDGE('',*,*,#5314,.F.);
#7761=ORIENTED_EDGE('',*,*,#5317,.F.);
#7762=ORIENTED_EDGE('',*,*,#5320,.F.);
#7763=ORIENTED_EDGE('',*,*,#5762,.F.);
#7764=ORIENTED_EDGE('',*,*,#5325,.F.);
#7765=ORIENTED_EDGE('',*,*,#5732,.F.);
#7766=ORIENTED_EDGE('',*,*,#5466,.T.);
#7767=ORIENTED_EDGE('',*,*,#5760,.T.);
#7768=ORIENTED_EDGE('',*,*,#5464,.T.);
#7769=ORIENTED_EDGE('',*,*,#5461,.T.);
#7770=ORIENTED_EDGE('',*,*,#5458,.T.);
#7771=ORIENTED_EDGE('',*,*,#5455,.T.);
#7772=ORIENTED_EDGE('',*,*,#5452,.T.);
#7773=ORIENTED_EDGE('',*,*,#5449,.T.);
#7774=ORIENTED_EDGE('',*,*,#5446,.T.);
#7775=ORIENTED_EDGE('',*,*,#5443,.T.);
#7776=ORIENTED_EDGE('',*,*,#5440,.T.);
#7777=ORIENTED_EDGE('',*,*,#5437,.T.);
#7778=ORIENTED_EDGE('',*,*,#5434,.T.);
#7779=ORIENTED_EDGE('',*,*,#5431,.T.);
#7780=ORIENTED_EDGE('',*,*,#5428,.T.);
#7781=ORIENTED_EDGE('',*,*,#5425,.T.);
#7782=ORIENTED_EDGE('',*,*,#5753,.F.);
#7783=ORIENTED_EDGE('',*,*,#5756,.T.);
#7784=ORIENTED_EDGE('',*,*,#5763,.F.);
#7785=ORIENTED_EDGE('',*,*,#5764,.F.);
#7786=ORIENTED_EDGE('',*,*,#5765,.F.);
#7787=ORIENTED_EDGE('',*,*,#5766,.T.);
#7788=ORIENTED_EDGE('',*,*,#5330,.F.);
#7789=ORIENTED_EDGE('',*,*,#5767,.T.);
#7790=ORIENTED_EDGE('',*,*,#5768,.T.);
#7791=ORIENTED_EDGE('',*,*,#5377,.T.);
#7792=ORIENTED_EDGE('',*,*,#5769,.T.);
#7793=ORIENTED_EDGE('',*,*,#5770,.T.);
#7794=ORIENTED_EDGE('',*,*,#5771,.F.);
#7795=ORIENTED_EDGE('',*,*,#5772,.F.);
#7796=ORIENTED_EDGE('',*,*,#5328,.F.);
#7797=ORIENTED_EDGE('',*,*,#5773,.T.);
#7798=ORIENTED_EDGE('',*,*,#5418,.T.);
#7799=ORIENTED_EDGE('',*,*,#5774,.T.);
#7800=ORIENTED_EDGE('',*,*,#5415,.F.);
#7801=ORIENTED_EDGE('',*,*,#5775,.F.);
#7802=ORIENTED_EDGE('',*,*,#5769,.F.);
#7803=ORIENTED_EDGE('',*,*,#5376,.F.);
#7804=ORIENTED_EDGE('',*,*,#5380,.F.);
#7805=ORIENTED_EDGE('',*,*,#5383,.F.);
#7806=ORIENTED_EDGE('',*,*,#5386,.F.);
#7807=ORIENTED_EDGE('',*,*,#5389,.F.);
#7808=ORIENTED_EDGE('',*,*,#5392,.F.);
#7809=ORIENTED_EDGE('',*,*,#5395,.F.);
#7810=ORIENTED_EDGE('',*,*,#5398,.F.);
#7811=ORIENTED_EDGE('',*,*,#5401,.F.);
#7812=ORIENTED_EDGE('',*,*,#5404,.F.);
#7813=ORIENTED_EDGE('',*,*,#5407,.F.);
#7814=ORIENTED_EDGE('',*,*,#5410,.F.);
#7815=ORIENTED_EDGE('',*,*,#5413,.F.);
#7816=ORIENTED_EDGE('',*,*,#5416,.F.);
#7817=ORIENTED_EDGE('',*,*,#5774,.F.);
#7818=ORIENTED_EDGE('',*,*,#5421,.F.);
#7819=ORIENTED_EDGE('',*,*,#5731,.F.);
#7820=ORIENTED_EDGE('',*,*,#5372,.F.);
#7821=ORIENTED_EDGE('',*,*,#5776,.F.);
#7822=ORIENTED_EDGE('',*,*,#5370,.F.);
#7823=ORIENTED_EDGE('',*,*,#5367,.F.);
#7824=ORIENTED_EDGE('',*,*,#5364,.F.);
#7825=ORIENTED_EDGE('',*,*,#5361,.F.);
#7826=ORIENTED_EDGE('',*,*,#5358,.F.);
#7827=ORIENTED_EDGE('',*,*,#5355,.F.);
#7828=ORIENTED_EDGE('',*,*,#5352,.F.);
#7829=ORIENTED_EDGE('',*,*,#5349,.F.);
#7830=ORIENTED_EDGE('',*,*,#5346,.F.);
#7831=ORIENTED_EDGE('',*,*,#5343,.F.);
#7832=ORIENTED_EDGE('',*,*,#5340,.F.);
#7833=ORIENTED_EDGE('',*,*,#5337,.F.);
#7834=ORIENTED_EDGE('',*,*,#5334,.F.);
#7835=ORIENTED_EDGE('',*,*,#5331,.F.);
#7836=ORIENTED_EDGE('',*,*,#5766,.F.);
#7837=ORIENTED_EDGE('',*,*,#5773,.F.);
#7838=ORIENTED_EDGE('',*,*,#5327,.F.);
#7839=ORIENTED_EDGE('',*,*,#5333,.F.);
#7840=ORIENTED_EDGE('',*,*,#5336,.F.);
#7841=ORIENTED_EDGE('',*,*,#5339,.F.);
#7842=ORIENTED_EDGE('',*,*,#5342,.F.);
#7843=ORIENTED_EDGE('',*,*,#5345,.F.);
#7844=ORIENTED_EDGE('',*,*,#5348,.F.);
#7845=ORIENTED_EDGE('',*,*,#5351,.F.);
#7846=ORIENTED_EDGE('',*,*,#5354,.F.);
#7847=ORIENTED_EDGE('',*,*,#5357,.F.);
#7848=ORIENTED_EDGE('',*,*,#5360,.F.);
#7849=ORIENTED_EDGE('',*,*,#5363,.F.);
#7850=ORIENTED_EDGE('',*,*,#5366,.F.);
#7851=ORIENTED_EDGE('',*,*,#5369,.F.);
#7852=ORIENTED_EDGE('',*,*,#5777,.F.);
#7853=ORIENTED_EDGE('',*,*,#5374,.F.);
#7854=ORIENTED_EDGE('',*,*,#5730,.F.);
#7855=ORIENTED_EDGE('',*,*,#5419,.T.);
#7856=ORIENTED_EDGE('',*,*,#5775,.T.);
#7857=ORIENTED_EDGE('',*,*,#5417,.T.);
#7858=ORIENTED_EDGE('',*,*,#5414,.T.);
#7859=ORIENTED_EDGE('',*,*,#5411,.T.);
#7860=ORIENTED_EDGE('',*,*,#5408,.T.);
#7861=ORIENTED_EDGE('',*,*,#5405,.T.);
#7862=ORIENTED_EDGE('',*,*,#5402,.T.);
#7863=ORIENTED_EDGE('',*,*,#5399,.T.);
#7864=ORIENTED_EDGE('',*,*,#5396,.T.);
#7865=ORIENTED_EDGE('',*,*,#5393,.T.);
#7866=ORIENTED_EDGE('',*,*,#5390,.T.);
#7867=ORIENTED_EDGE('',*,*,#5387,.T.);
#7868=ORIENTED_EDGE('',*,*,#5384,.T.);
#7869=ORIENTED_EDGE('',*,*,#5381,.T.);
#7870=ORIENTED_EDGE('',*,*,#5378,.T.);
#7871=ORIENTED_EDGE('',*,*,#5768,.F.);
#7872=ORIENTED_EDGE('',*,*,#5771,.T.);
#7873=ORIENTED_EDGE('',*,*,#5778,.F.);
#7874=ORIENTED_EDGE('',*,*,#5779,.F.);
#7875=ORIENTED_EDGE('',*,*,#5371,.T.);
#7876=ORIENTED_EDGE('',*,*,#5777,.T.);
#7877=ORIENTED_EDGE('',*,*,#5368,.F.);
#7878=ORIENTED_EDGE('',*,*,#5776,.T.);
#7879=ORIENTED_EDGE('',*,*,#5570,.F.);
#7880=ORIENTED_EDGE('',*,*,#5473,.F.);
#7881=ORIENTED_EDGE('',*,*,#5322,.T.);
#7882=ORIENTED_EDGE('',*,*,#5762,.T.);
#7883=ORIENTED_EDGE('',*,*,#5319,.F.);
#7884=ORIENTED_EDGE('',*,*,#5761,.T.);
#7885=ORIENTED_EDGE('',*,*,#5179,.F.);
#7886=ORIENTED_EDGE('',*,*,#5780,.T.);
#7887=ORIENTED_EDGE('',*,*,#5229,.T.);
#7888=ORIENTED_EDGE('',*,*,#5781,.T.);
#7889=ORIENTED_EDGE('',*,*,#5273,.T.);
#7890=ORIENTED_EDGE('',*,*,#5782,.T.);
#7891=ORIENTED_EDGE('',*,*,#5270,.F.);
#7892=ORIENTED_EDGE('',*,*,#5783,.F.);
#7893=ORIENTED_EDGE('',*,*,#5781,.F.);
#7894=ORIENTED_EDGE('',*,*,#5228,.F.);
#7895=ORIENTED_EDGE('',*,*,#5232,.F.);
#7896=ORIENTED_EDGE('',*,*,#5235,.F.);
#7897=ORIENTED_EDGE('',*,*,#5238,.F.);
#7898=ORIENTED_EDGE('',*,*,#5241,.F.);
#7899=ORIENTED_EDGE('',*,*,#5244,.F.);
#7900=ORIENTED_EDGE('',*,*,#5247,.F.);
#7901=ORIENTED_EDGE('',*,*,#5250,.F.);
#7902=ORIENTED_EDGE('',*,*,#5253,.F.);
#7903=ORIENTED_EDGE('',*,*,#5256,.F.);
#7904=ORIENTED_EDGE('',*,*,#5259,.F.);
#7905=ORIENTED_EDGE('',*,*,#5262,.F.);
#7906=ORIENTED_EDGE('',*,*,#5265,.F.);
#7907=ORIENTED_EDGE('',*,*,#5268,.F.);
#7908=ORIENTED_EDGE('',*,*,#5271,.F.);
#7909=ORIENTED_EDGE('',*,*,#5782,.F.);
#7910=ORIENTED_EDGE('',*,*,#5276,.F.);
#7911=ORIENTED_EDGE('',*,*,#5784,.F.);
#7912=ORIENTED_EDGE('',*,*,#5224,.F.);
#7913=ORIENTED_EDGE('',*,*,#5785,.F.);
#7914=ORIENTED_EDGE('',*,*,#5222,.F.);
#7915=ORIENTED_EDGE('',*,*,#5219,.F.);
#7916=ORIENTED_EDGE('',*,*,#5216,.F.);
#7917=ORIENTED_EDGE('',*,*,#5213,.F.);
#7918=ORIENTED_EDGE('',*,*,#5210,.F.);
#7919=ORIENTED_EDGE('',*,*,#5207,.F.);
#7920=ORIENTED_EDGE('',*,*,#5204,.F.);
#7921=ORIENTED_EDGE('',*,*,#5201,.F.);
#7922=ORIENTED_EDGE('',*,*,#5198,.F.);
#7923=ORIENTED_EDGE('',*,*,#5195,.F.);
#7924=ORIENTED_EDGE('',*,*,#5192,.F.);
#7925=ORIENTED_EDGE('',*,*,#5189,.F.);
#7926=ORIENTED_EDGE('',*,*,#5186,.F.);
#7927=ORIENTED_EDGE('',*,*,#5183,.F.);
#7928=ORIENTED_EDGE('',*,*,#5180,.F.);
#7929=ORIENTED_EDGE('',*,*,#5780,.F.);
#7930=ORIENTED_EDGE('',*,*,#5178,.F.);
#7931=ORIENTED_EDGE('',*,*,#5185,.F.);
#7932=ORIENTED_EDGE('',*,*,#5188,.F.);
#7933=ORIENTED_EDGE('',*,*,#5191,.F.);
#7934=ORIENTED_EDGE('',*,*,#5194,.F.);
#7935=ORIENTED_EDGE('',*,*,#5197,.F.);
#7936=ORIENTED_EDGE('',*,*,#5200,.F.);
#7937=ORIENTED_EDGE('',*,*,#5203,.F.);
#7938=ORIENTED_EDGE('',*,*,#5206,.F.);
#7939=ORIENTED_EDGE('',*,*,#5209,.F.);
#7940=ORIENTED_EDGE('',*,*,#5212,.F.);
#7941=ORIENTED_EDGE('',*,*,#5215,.F.);
#7942=ORIENTED_EDGE('',*,*,#5218,.F.);
#7943=ORIENTED_EDGE('',*,*,#5221,.F.);
#7944=ORIENTED_EDGE('',*,*,#5786,.F.);
#7945=ORIENTED_EDGE('',*,*,#5226,.F.);
#7946=ORIENTED_EDGE('',*,*,#5787,.F.);
#7947=ORIENTED_EDGE('',*,*,#5274,.T.);
#7948=ORIENTED_EDGE('',*,*,#5783,.T.);
#7949=ORIENTED_EDGE('',*,*,#5272,.T.);
#7950=ORIENTED_EDGE('',*,*,#5269,.T.);
#7951=ORIENTED_EDGE('',*,*,#5266,.T.);
#7952=ORIENTED_EDGE('',*,*,#5263,.T.);
#7953=ORIENTED_EDGE('',*,*,#5260,.T.);
#7954=ORIENTED_EDGE('',*,*,#5257,.T.);
#7955=ORIENTED_EDGE('',*,*,#5254,.T.);
#7956=ORIENTED_EDGE('',*,*,#5251,.T.);
#7957=ORIENTED_EDGE('',*,*,#5248,.T.);
#7958=ORIENTED_EDGE('',*,*,#5245,.T.);
#7959=ORIENTED_EDGE('',*,*,#5242,.T.);
#7960=ORIENTED_EDGE('',*,*,#5239,.T.);
#7961=ORIENTED_EDGE('',*,*,#5236,.T.);
#7962=ORIENTED_EDGE('',*,*,#5233,.T.);
#7963=ORIENTED_EDGE('',*,*,#5230,.T.);
#7964=ORIENTED_EDGE('',*,*,#5223,.T.);
#7965=ORIENTED_EDGE('',*,*,#5786,.T.);
#7966=ORIENTED_EDGE('',*,*,#5220,.F.);
#7967=ORIENTED_EDGE('',*,*,#5785,.T.);
#7968=ORIENTED_EDGE('',*,*,#5079,.F.);
#7969=ORIENTED_EDGE('',*,*,#5788,.T.);
#7970=ORIENTED_EDGE('',*,*,#5129,.T.);
#7971=ORIENTED_EDGE('',*,*,#5789,.T.);
#7972=ORIENTED_EDGE('',*,*,#5173,.T.);
#7973=ORIENTED_EDGE('',*,*,#5790,.T.);
#7974=ORIENTED_EDGE('',*,*,#5170,.F.);
#7975=ORIENTED_EDGE('',*,*,#5791,.F.);
#7976=ORIENTED_EDGE('',*,*,#5789,.F.);
#7977=ORIENTED_EDGE('',*,*,#5128,.F.);
#7978=ORIENTED_EDGE('',*,*,#5132,.F.);
#7979=ORIENTED_EDGE('',*,*,#5135,.F.);
#7980=ORIENTED_EDGE('',*,*,#5138,.F.);
#7981=ORIENTED_EDGE('',*,*,#5141,.F.);
#7982=ORIENTED_EDGE('',*,*,#5144,.F.);
#7983=ORIENTED_EDGE('',*,*,#5147,.F.);
#7984=ORIENTED_EDGE('',*,*,#5150,.F.);
#7985=ORIENTED_EDGE('',*,*,#5153,.F.);
#7986=ORIENTED_EDGE('',*,*,#5156,.F.);
#7987=ORIENTED_EDGE('',*,*,#5159,.F.);
#7988=ORIENTED_EDGE('',*,*,#5162,.F.);
#7989=ORIENTED_EDGE('',*,*,#5165,.F.);
#7990=ORIENTED_EDGE('',*,*,#5168,.F.);
#7991=ORIENTED_EDGE('',*,*,#5171,.F.);
#7992=ORIENTED_EDGE('',*,*,#5790,.F.);
#7993=ORIENTED_EDGE('',*,*,#5176,.F.);
#7994=ORIENTED_EDGE('',*,*,#5792,.F.);
#7995=ORIENTED_EDGE('',*,*,#5124,.F.);
#7996=ORIENTED_EDGE('',*,*,#5793,.F.);
#7997=ORIENTED_EDGE('',*,*,#5122,.F.);
#7998=ORIENTED_EDGE('',*,*,#5119,.F.);
#7999=ORIENTED_EDGE('',*,*,#5116,.F.);
#8000=ORIENTED_EDGE('',*,*,#5113,.F.);
#8001=ORIENTED_EDGE('',*,*,#5110,.F.);
#8002=ORIENTED_EDGE('',*,*,#5107,.F.);
#8003=ORIENTED_EDGE('',*,*,#5104,.F.);
#8004=ORIENTED_EDGE('',*,*,#5101,.F.);
#8005=ORIENTED_EDGE('',*,*,#5098,.F.);
#8006=ORIENTED_EDGE('',*,*,#5095,.F.);
#8007=ORIENTED_EDGE('',*,*,#5092,.F.);
#8008=ORIENTED_EDGE('',*,*,#5089,.F.);
#8009=ORIENTED_EDGE('',*,*,#5086,.F.);
#8010=ORIENTED_EDGE('',*,*,#5083,.F.);
#8011=ORIENTED_EDGE('',*,*,#5080,.F.);
#8012=ORIENTED_EDGE('',*,*,#5788,.F.);
#8013=ORIENTED_EDGE('',*,*,#5078,.F.);
#8014=ORIENTED_EDGE('',*,*,#5085,.F.);
#8015=ORIENTED_EDGE('',*,*,#5088,.F.);
#8016=ORIENTED_EDGE('',*,*,#5091,.F.);
#8017=ORIENTED_EDGE('',*,*,#5094,.F.);
#8018=ORIENTED_EDGE('',*,*,#5097,.F.);
#8019=ORIENTED_EDGE('',*,*,#5100,.F.);
#8020=ORIENTED_EDGE('',*,*,#5103,.F.);
#8021=ORIENTED_EDGE('',*,*,#5106,.F.);
#8022=ORIENTED_EDGE('',*,*,#5109,.F.);
#8023=ORIENTED_EDGE('',*,*,#5112,.F.);
#8024=ORIENTED_EDGE('',*,*,#5115,.F.);
#8025=ORIENTED_EDGE('',*,*,#5118,.F.);
#8026=ORIENTED_EDGE('',*,*,#5121,.F.);
#8027=ORIENTED_EDGE('',*,*,#5794,.F.);
#8028=ORIENTED_EDGE('',*,*,#5126,.F.);
#8029=ORIENTED_EDGE('',*,*,#5795,.F.);
#8030=ORIENTED_EDGE('',*,*,#5174,.T.);
#8031=ORIENTED_EDGE('',*,*,#5791,.T.);
#8032=ORIENTED_EDGE('',*,*,#5172,.T.);
#8033=ORIENTED_EDGE('',*,*,#5169,.T.);
#8034=ORIENTED_EDGE('',*,*,#5166,.T.);
#8035=ORIENTED_EDGE('',*,*,#5163,.T.);
#8036=ORIENTED_EDGE('',*,*,#5160,.T.);
#8037=ORIENTED_EDGE('',*,*,#5157,.T.);
#8038=ORIENTED_EDGE('',*,*,#5154,.T.);
#8039=ORIENTED_EDGE('',*,*,#5151,.T.);
#8040=ORIENTED_EDGE('',*,*,#5148,.T.);
#8041=ORIENTED_EDGE('',*,*,#5145,.T.);
#8042=ORIENTED_EDGE('',*,*,#5142,.T.);
#8043=ORIENTED_EDGE('',*,*,#5139,.T.);
#8044=ORIENTED_EDGE('',*,*,#5136,.T.);
#8045=ORIENTED_EDGE('',*,*,#5133,.T.);
#8046=ORIENTED_EDGE('',*,*,#5130,.T.);
#8047=ORIENTED_EDGE('',*,*,#5123,.T.);
#8048=ORIENTED_EDGE('',*,*,#5794,.T.);
#8049=ORIENTED_EDGE('',*,*,#5120,.F.);
#8050=ORIENTED_EDGE('',*,*,#5793,.T.);
#8051=ORIENTED_EDGE('',*,*,#4979,.F.);
#8052=ORIENTED_EDGE('',*,*,#5796,.T.);
#8053=ORIENTED_EDGE('',*,*,#5029,.T.);
#8054=ORIENTED_EDGE('',*,*,#5797,.T.);
#8055=ORIENTED_EDGE('',*,*,#5073,.T.);
#8056=ORIENTED_EDGE('',*,*,#5798,.T.);
#8057=ORIENTED_EDGE('',*,*,#5070,.F.);
#8058=ORIENTED_EDGE('',*,*,#5799,.F.);
#8059=ORIENTED_EDGE('',*,*,#5797,.F.);
#8060=ORIENTED_EDGE('',*,*,#5028,.F.);
#8061=ORIENTED_EDGE('',*,*,#5032,.F.);
#8062=ORIENTED_EDGE('',*,*,#5035,.F.);
#8063=ORIENTED_EDGE('',*,*,#5038,.F.);
#8064=ORIENTED_EDGE('',*,*,#5041,.F.);
#8065=ORIENTED_EDGE('',*,*,#5044,.F.);
#8066=ORIENTED_EDGE('',*,*,#5047,.F.);
#8067=ORIENTED_EDGE('',*,*,#5050,.F.);
#8068=ORIENTED_EDGE('',*,*,#5053,.F.);
#8069=ORIENTED_EDGE('',*,*,#5056,.F.);
#8070=ORIENTED_EDGE('',*,*,#5059,.F.);
#8071=ORIENTED_EDGE('',*,*,#5062,.F.);
#8072=ORIENTED_EDGE('',*,*,#5065,.F.);
#8073=ORIENTED_EDGE('',*,*,#5068,.F.);
#8074=ORIENTED_EDGE('',*,*,#5071,.F.);
#8075=ORIENTED_EDGE('',*,*,#5798,.F.);
#8076=ORIENTED_EDGE('',*,*,#5076,.F.);
#8077=ORIENTED_EDGE('',*,*,#5800,.F.);
#8078=ORIENTED_EDGE('',*,*,#5024,.F.);
#8079=ORIENTED_EDGE('',*,*,#5801,.F.);
#8080=ORIENTED_EDGE('',*,*,#5022,.F.);
#8081=ORIENTED_EDGE('',*,*,#5019,.F.);
#8082=ORIENTED_EDGE('',*,*,#5016,.F.);
#8083=ORIENTED_EDGE('',*,*,#5013,.F.);
#8084=ORIENTED_EDGE('',*,*,#5010,.F.);
#8085=ORIENTED_EDGE('',*,*,#5007,.F.);
#8086=ORIENTED_EDGE('',*,*,#5004,.F.);
#8087=ORIENTED_EDGE('',*,*,#5001,.F.);
#8088=ORIENTED_EDGE('',*,*,#4998,.F.);
#8089=ORIENTED_EDGE('',*,*,#4995,.F.);
#8090=ORIENTED_EDGE('',*,*,#4992,.F.);
#8091=ORIENTED_EDGE('',*,*,#4989,.F.);
#8092=ORIENTED_EDGE('',*,*,#4986,.F.);
#8093=ORIENTED_EDGE('',*,*,#4983,.F.);
#8094=ORIENTED_EDGE('',*,*,#4980,.F.);
#8095=ORIENTED_EDGE('',*,*,#5796,.F.);
#8096=ORIENTED_EDGE('',*,*,#4978,.F.);
#8097=ORIENTED_EDGE('',*,*,#4985,.F.);
#8098=ORIENTED_EDGE('',*,*,#4988,.F.);
#8099=ORIENTED_EDGE('',*,*,#4991,.F.);
#8100=ORIENTED_EDGE('',*,*,#4994,.F.);
#8101=ORIENTED_EDGE('',*,*,#4997,.F.);
#8102=ORIENTED_EDGE('',*,*,#5000,.F.);
#8103=ORIENTED_EDGE('',*,*,#5003,.F.);
#8104=ORIENTED_EDGE('',*,*,#5006,.F.);
#8105=ORIENTED_EDGE('',*,*,#5009,.F.);
#8106=ORIENTED_EDGE('',*,*,#5012,.F.);
#8107=ORIENTED_EDGE('',*,*,#5015,.F.);
#8108=ORIENTED_EDGE('',*,*,#5018,.F.);
#8109=ORIENTED_EDGE('',*,*,#5021,.F.);
#8110=ORIENTED_EDGE('',*,*,#5802,.F.);
#8111=ORIENTED_EDGE('',*,*,#5026,.F.);
#8112=ORIENTED_EDGE('',*,*,#5803,.F.);
#8113=ORIENTED_EDGE('',*,*,#5074,.T.);
#8114=ORIENTED_EDGE('',*,*,#5799,.T.);
#8115=ORIENTED_EDGE('',*,*,#5072,.T.);
#8116=ORIENTED_EDGE('',*,*,#5069,.T.);
#8117=ORIENTED_EDGE('',*,*,#5066,.T.);
#8118=ORIENTED_EDGE('',*,*,#5063,.T.);
#8119=ORIENTED_EDGE('',*,*,#5060,.T.);
#8120=ORIENTED_EDGE('',*,*,#5057,.T.);
#8121=ORIENTED_EDGE('',*,*,#5054,.T.);
#8122=ORIENTED_EDGE('',*,*,#5051,.T.);
#8123=ORIENTED_EDGE('',*,*,#5048,.T.);
#8124=ORIENTED_EDGE('',*,*,#5045,.T.);
#8125=ORIENTED_EDGE('',*,*,#5042,.T.);
#8126=ORIENTED_EDGE('',*,*,#5039,.T.);
#8127=ORIENTED_EDGE('',*,*,#5036,.T.);
#8128=ORIENTED_EDGE('',*,*,#5033,.T.);
#8129=ORIENTED_EDGE('',*,*,#5030,.T.);
#8130=ORIENTED_EDGE('',*,*,#5023,.T.);
#8131=ORIENTED_EDGE('',*,*,#5802,.T.);
#8132=ORIENTED_EDGE('',*,*,#5020,.F.);
#8133=ORIENTED_EDGE('',*,*,#5801,.T.);
#8134=ORIENTED_EDGE('',*,*,#4879,.F.);
#8135=ORIENTED_EDGE('',*,*,#5804,.T.);
#8136=ORIENTED_EDGE('',*,*,#4929,.T.);
#8137=ORIENTED_EDGE('',*,*,#5805,.T.);
#8138=ORIENTED_EDGE('',*,*,#4973,.T.);
#8139=ORIENTED_EDGE('',*,*,#5806,.T.);
#8140=ORIENTED_EDGE('',*,*,#4970,.F.);
#8141=ORIENTED_EDGE('',*,*,#5807,.F.);
#8142=ORIENTED_EDGE('',*,*,#5805,.F.);
#8143=ORIENTED_EDGE('',*,*,#4928,.F.);
#8144=ORIENTED_EDGE('',*,*,#4932,.F.);
#8145=ORIENTED_EDGE('',*,*,#4935,.F.);
#8146=ORIENTED_EDGE('',*,*,#4938,.F.);
#8147=ORIENTED_EDGE('',*,*,#4941,.F.);
#8148=ORIENTED_EDGE('',*,*,#4944,.F.);
#8149=ORIENTED_EDGE('',*,*,#4947,.F.);
#8150=ORIENTED_EDGE('',*,*,#4950,.F.);
#8151=ORIENTED_EDGE('',*,*,#4953,.F.);
#8152=ORIENTED_EDGE('',*,*,#4956,.F.);
#8153=ORIENTED_EDGE('',*,*,#4959,.F.);
#8154=ORIENTED_EDGE('',*,*,#4962,.F.);
#8155=ORIENTED_EDGE('',*,*,#4965,.F.);
#8156=ORIENTED_EDGE('',*,*,#4968,.F.);
#8157=ORIENTED_EDGE('',*,*,#4971,.F.);
#8158=ORIENTED_EDGE('',*,*,#5806,.F.);
#8159=ORIENTED_EDGE('',*,*,#4976,.F.);
#8160=ORIENTED_EDGE('',*,*,#5808,.F.);
#8161=ORIENTED_EDGE('',*,*,#4924,.F.);
#8162=ORIENTED_EDGE('',*,*,#5809,.F.);
#8163=ORIENTED_EDGE('',*,*,#4922,.F.);
#8164=ORIENTED_EDGE('',*,*,#4919,.F.);
#8165=ORIENTED_EDGE('',*,*,#4916,.F.);
#8166=ORIENTED_EDGE('',*,*,#4913,.F.);
#8167=ORIENTED_EDGE('',*,*,#4910,.F.);
#8168=ORIENTED_EDGE('',*,*,#4907,.F.);
#8169=ORIENTED_EDGE('',*,*,#4904,.F.);
#8170=ORIENTED_EDGE('',*,*,#4901,.F.);
#8171=ORIENTED_EDGE('',*,*,#4898,.F.);
#8172=ORIENTED_EDGE('',*,*,#4895,.F.);
#8173=ORIENTED_EDGE('',*,*,#4892,.F.);
#8174=ORIENTED_EDGE('',*,*,#4889,.F.);
#8175=ORIENTED_EDGE('',*,*,#4886,.F.);
#8176=ORIENTED_EDGE('',*,*,#4883,.F.);
#8177=ORIENTED_EDGE('',*,*,#4880,.F.);
#8178=ORIENTED_EDGE('',*,*,#5804,.F.);
#8179=ORIENTED_EDGE('',*,*,#4878,.F.);
#8180=ORIENTED_EDGE('',*,*,#4885,.F.);
#8181=ORIENTED_EDGE('',*,*,#4888,.F.);
#8182=ORIENTED_EDGE('',*,*,#4891,.F.);
#8183=ORIENTED_EDGE('',*,*,#4894,.F.);
#8184=ORIENTED_EDGE('',*,*,#4897,.F.);
#8185=ORIENTED_EDGE('',*,*,#4900,.F.);
#8186=ORIENTED_EDGE('',*,*,#4903,.F.);
#8187=ORIENTED_EDGE('',*,*,#4906,.F.);
#8188=ORIENTED_EDGE('',*,*,#4909,.F.);
#8189=ORIENTED_EDGE('',*,*,#4912,.F.);
#8190=ORIENTED_EDGE('',*,*,#4915,.F.);
#8191=ORIENTED_EDGE('',*,*,#4918,.F.);
#8192=ORIENTED_EDGE('',*,*,#4921,.F.);
#8193=ORIENTED_EDGE('',*,*,#5810,.F.);
#8194=ORIENTED_EDGE('',*,*,#4926,.F.);
#8195=ORIENTED_EDGE('',*,*,#5811,.F.);
#8196=ORIENTED_EDGE('',*,*,#4974,.T.);
#8197=ORIENTED_EDGE('',*,*,#5807,.T.);
#8198=ORIENTED_EDGE('',*,*,#4972,.T.);
#8199=ORIENTED_EDGE('',*,*,#4969,.T.);
#8200=ORIENTED_EDGE('',*,*,#4966,.T.);
#8201=ORIENTED_EDGE('',*,*,#4963,.T.);
#8202=ORIENTED_EDGE('',*,*,#4960,.T.);
#8203=ORIENTED_EDGE('',*,*,#4957,.T.);
#8204=ORIENTED_EDGE('',*,*,#4954,.T.);
#8205=ORIENTED_EDGE('',*,*,#4951,.T.);
#8206=ORIENTED_EDGE('',*,*,#4948,.T.);
#8207=ORIENTED_EDGE('',*,*,#4945,.T.);
#8208=ORIENTED_EDGE('',*,*,#4942,.T.);
#8209=ORIENTED_EDGE('',*,*,#4939,.T.);
#8210=ORIENTED_EDGE('',*,*,#4936,.T.);
#8211=ORIENTED_EDGE('',*,*,#4933,.T.);
#8212=ORIENTED_EDGE('',*,*,#4930,.T.);
#8213=ORIENTED_EDGE('',*,*,#4923,.T.);
#8214=ORIENTED_EDGE('',*,*,#5810,.T.);
#8215=ORIENTED_EDGE('',*,*,#4920,.F.);
#8216=ORIENTED_EDGE('',*,*,#5809,.T.);
#8217=ORIENTED_EDGE('',*,*,#4982,.F.);
#8218=ORIENTED_EDGE('',*,*,#4882,.F.);
#8219=ORIENTED_EDGE('',*,*,#5082,.F.);
#8220=ORIENTED_EDGE('',*,*,#5182,.F.);
#8221=ORIENTED_EDGE('',*,*,#5812,.F.);
#8222=ORIENTED_EDGE('',*,*,#5813,.T.);
#8223=ORIENTED_EDGE('',*,*,#5814,.F.);
#8224=ORIENTED_EDGE('',*,*,#5813,.F.);
#8225=ORIENTED_EDGE('',*,*,#5815,.F.);
#8226=ORIENTED_EDGE('',*,*,#5816,.T.);
#8227=ORIENTED_EDGE('',*,*,#5817,.F.);
#8228=ORIENTED_EDGE('',*,*,#5816,.F.);
#8229=ORIENTED_EDGE('',*,*,#5818,.F.);
#8230=ORIENTED_EDGE('',*,*,#5819,.T.);
#8231=ORIENTED_EDGE('',*,*,#5820,.F.);
#8232=ORIENTED_EDGE('',*,*,#5819,.F.);
#8233=ORIENTED_EDGE('',*,*,#5821,.F.);
#8234=ORIENTED_EDGE('',*,*,#5822,.T.);
#8235=ORIENTED_EDGE('',*,*,#5823,.F.);
#8236=ORIENTED_EDGE('',*,*,#5822,.F.);
#8237=ORIENTED_EDGE('',*,*,#5824,.F.);
#8238=ORIENTED_EDGE('',*,*,#5825,.T.);
#8239=ORIENTED_EDGE('',*,*,#5826,.F.);
#8240=ORIENTED_EDGE('',*,*,#5825,.F.);
#8241=ORIENTED_EDGE('',*,*,#5827,.F.);
#8242=ORIENTED_EDGE('',*,*,#5828,.T.);
#8243=ORIENTED_EDGE('',*,*,#5829,.F.);
#8244=ORIENTED_EDGE('',*,*,#5828,.F.);
#8245=ORIENTED_EDGE('',*,*,#5830,.F.);
#8246=ORIENTED_EDGE('',*,*,#5831,.T.);
#8247=ORIENTED_EDGE('',*,*,#5832,.F.);
#8248=ORIENTED_EDGE('',*,*,#5831,.F.);
#8249=ORIENTED_EDGE('',*,*,#5833,.F.);
#8250=ORIENTED_EDGE('',*,*,#5834,.T.);
#8251=ORIENTED_EDGE('',*,*,#5835,.F.);
#8252=ORIENTED_EDGE('',*,*,#5834,.F.);
#8253=ORIENTED_EDGE('',*,*,#5836,.F.);
#8254=ORIENTED_EDGE('',*,*,#5837,.T.);
#8255=ORIENTED_EDGE('',*,*,#5767,.F.);
#8256=ORIENTED_EDGE('',*,*,#5779,.T.);
#8257=ORIENTED_EDGE('',*,*,#5778,.T.);
#8258=ORIENTED_EDGE('',*,*,#5770,.F.);
#8259=ORIENTED_EDGE('',*,*,#5838,.T.);
#8260=ORIENTED_EDGE('',*,*,#5839,.F.);
#8261=ORIENTED_EDGE('',*,*,#5838,.F.);
#8262=ORIENTED_EDGE('',*,*,#5765,.T.);
#8263=ORIENTED_EDGE('',*,*,#5329,.T.);
#8264=ORIENTED_EDGE('',*,*,#5772,.T.);
#8265=ORIENTED_EDGE('',*,*,#5837,.F.);
#8266=ORIENTED_EDGE('',*,*,#5840,.F.);
#8267=ORIENTED_EDGE('',*,*,#5841,.T.);
#8268=ORIENTED_EDGE('',*,*,#5842,.F.);
#8269=ORIENTED_EDGE('',*,*,#5841,.F.);
#8270=ORIENTED_EDGE('',*,*,#5843,.F.);
#8271=ORIENTED_EDGE('',*,*,#5844,.T.);
#8272=ORIENTED_EDGE('',*,*,#5845,.F.);
#8273=ORIENTED_EDGE('',*,*,#5844,.F.);
#8274=ORIENTED_EDGE('',*,*,#5846,.F.);
#8275=ORIENTED_EDGE('',*,*,#5847,.T.);
#8276=ORIENTED_EDGE('',*,*,#5848,.F.);
#8277=ORIENTED_EDGE('',*,*,#5847,.F.);
#8278=ORIENTED_EDGE('',*,*,#5849,.F.);
#8279=ORIENTED_EDGE('',*,*,#5850,.T.);
#8280=ORIENTED_EDGE('',*,*,#5851,.F.);
#8281=ORIENTED_EDGE('',*,*,#5850,.F.);
#8282=ORIENTED_EDGE('',*,*,#5852,.F.);
#8283=ORIENTED_EDGE('',*,*,#5853,.T.);
#8284=ORIENTED_EDGE('',*,*,#5854,.F.);
#8285=ORIENTED_EDGE('',*,*,#5853,.F.);
#8286=ORIENTED_EDGE('',*,*,#5855,.F.);
#8287=ORIENTED_EDGE('',*,*,#5856,.T.);
#8288=ORIENTED_EDGE('',*,*,#5857,.F.);
#8289=ORIENTED_EDGE('',*,*,#5856,.F.);
#8290=ORIENTED_EDGE('',*,*,#5858,.F.);
#8291=ORIENTED_EDGE('',*,*,#5859,.T.);
#8292=ORIENTED_EDGE('',*,*,#5860,.F.);
#8293=ORIENTED_EDGE('',*,*,#5859,.F.);
#8294=ORIENTED_EDGE('',*,*,#5861,.F.);
#8295=ORIENTED_EDGE('',*,*,#5862,.T.);
#8296=ORIENTED_EDGE('',*,*,#5752,.F.);
#8297=ORIENTED_EDGE('',*,*,#5764,.T.);
#8298=ORIENTED_EDGE('',*,*,#5763,.T.);
#8299=ORIENTED_EDGE('',*,*,#5755,.F.);
#8300=ORIENTED_EDGE('',*,*,#5863,.T.);
#8301=ORIENTED_EDGE('',*,*,#5864,.F.);
#8302=ORIENTED_EDGE('',*,*,#5863,.F.);
#8303=ORIENTED_EDGE('',*,*,#5750,.T.);
#8304=ORIENTED_EDGE('',*,*,#5280,.T.);
#8305=ORIENTED_EDGE('',*,*,#5757,.T.);
#8306=ORIENTED_EDGE('',*,*,#5862,.F.);
#8307=ORIENTED_EDGE('',*,*,#5865,.F.);
#8308=ORIENTED_EDGE('',*,*,#5866,.T.);
#8309=ORIENTED_EDGE('',*,*,#5867,.F.);
#8310=ORIENTED_EDGE('',*,*,#5866,.F.);
#8311=ORIENTED_EDGE('',*,*,#5868,.F.);
#8312=ORIENTED_EDGE('',*,*,#5869,.T.);
#8313=ORIENTED_EDGE('',*,*,#5870,.T.);
#8314=ORIENTED_EDGE('',*,*,#5871,.F.);
#8315=ORIENTED_EDGE('',*,*,#5872,.F.);
#8316=ORIENTED_EDGE('',*,*,#5873,.T.);
#8317=ORIENTED_EDGE('',*,*,#5874,.T.);
#8318=ORIENTED_EDGE('',*,*,#5869,.F.);
#8319=ORIENTED_EDGE('',*,*,#5867,.T.);
#8320=ORIENTED_EDGE('',*,*,#5864,.T.);
#8321=ORIENTED_EDGE('',*,*,#5860,.T.);
#8322=ORIENTED_EDGE('',*,*,#5857,.T.);
#8323=ORIENTED_EDGE('',*,*,#5854,.T.);
#8324=ORIENTED_EDGE('',*,*,#5851,.T.);
#8325=ORIENTED_EDGE('',*,*,#5848,.T.);
#8326=ORIENTED_EDGE('',*,*,#5845,.T.);
#8327=ORIENTED_EDGE('',*,*,#5842,.T.);
#8328=ORIENTED_EDGE('',*,*,#5839,.T.);
#8329=ORIENTED_EDGE('',*,*,#5835,.T.);
#8330=ORIENTED_EDGE('',*,*,#5832,.T.);
#8331=ORIENTED_EDGE('',*,*,#5829,.T.);
#8332=ORIENTED_EDGE('',*,*,#5826,.T.);
#8333=ORIENTED_EDGE('',*,*,#5823,.T.);
#8334=ORIENTED_EDGE('',*,*,#5820,.T.);
#8335=ORIENTED_EDGE('',*,*,#5817,.T.);
#8336=ORIENTED_EDGE('',*,*,#5814,.T.);
#8337=ORIENTED_EDGE('',*,*,#5875,.F.);
#8338=ORIENTED_EDGE('',*,*,#5876,.T.);
#8339=ORIENTED_EDGE('',*,*,#5877,.T.);
#8340=ORIENTED_EDGE('',*,*,#5873,.F.);
#8341=ORIENTED_EDGE('',*,*,#5878,.F.);
#8342=ORIENTED_EDGE('',*,*,#5871,.T.);
#8343=ORIENTED_EDGE('',*,*,#5879,.T.);
#8344=ORIENTED_EDGE('',*,*,#5876,.F.);
#8345=ORIENTED_EDGE('',*,*,#5879,.F.);
#8346=ORIENTED_EDGE('',*,*,#5870,.F.);
#8347=ORIENTED_EDGE('',*,*,#5874,.F.);
#8348=ORIENTED_EDGE('',*,*,#5877,.F.);
#8349=ORIENTED_EDGE('',*,*,#5717,.T.);
#8350=ORIENTED_EDGE('',*,*,#5687,.T.);
#8351=ORIENTED_EDGE('',*,*,#5720,.T.);
#8352=ORIENTED_EDGE('',*,*,#5691,.T.);
#8353=ORIENTED_EDGE('',*,*,#5727,.T.);
#8354=ORIENTED_EDGE('',*,*,#5880,.T.);
#8355=ORIENTED_EDGE('',*,*,#5881,.F.);
#8356=ORIENTED_EDGE('',*,*,#5882,.F.);
#8357=ORIENTED_EDGE('',*,*,#5728,.T.);
#8358=ORIENTED_EDGE('',*,*,#5882,.T.);
#8359=ORIENTED_EDGE('',*,*,#5883,.F.);
#8360=ORIENTED_EDGE('',*,*,#5884,.F.);
#8361=ORIENTED_EDGE('',*,*,#5865,.T.);
#8362=ORIENTED_EDGE('',*,*,#5861,.T.);
#8363=ORIENTED_EDGE('',*,*,#5858,.T.);
#8364=ORIENTED_EDGE('',*,*,#5855,.T.);
#8365=ORIENTED_EDGE('',*,*,#5852,.T.);
#8366=ORIENTED_EDGE('',*,*,#5849,.T.);
#8367=ORIENTED_EDGE('',*,*,#5846,.T.);
#8368=ORIENTED_EDGE('',*,*,#5843,.T.);
#8369=ORIENTED_EDGE('',*,*,#5840,.T.);
#8370=ORIENTED_EDGE('',*,*,#5836,.T.);
#8371=ORIENTED_EDGE('',*,*,#5833,.T.);
#8372=ORIENTED_EDGE('',*,*,#5830,.T.);
#8373=ORIENTED_EDGE('',*,*,#5827,.T.);
#8374=ORIENTED_EDGE('',*,*,#5824,.T.);
#8375=ORIENTED_EDGE('',*,*,#5821,.T.);
#8376=ORIENTED_EDGE('',*,*,#5818,.T.);
#8377=ORIENTED_EDGE('',*,*,#5815,.T.);
#8378=ORIENTED_EDGE('',*,*,#5812,.T.);
#8379=ORIENTED_EDGE('',*,*,#5729,.T.);
#8380=ORIENTED_EDGE('',*,*,#5884,.T.);
#8381=ORIENTED_EDGE('',*,*,#5885,.F.);
#8382=ORIENTED_EDGE('',*,*,#5886,.F.);
#8383=ORIENTED_EDGE('',*,*,#5726,.T.);
#8384=ORIENTED_EDGE('',*,*,#5886,.T.);
#8385=ORIENTED_EDGE('',*,*,#5887,.F.);
#8386=ORIENTED_EDGE('',*,*,#5880,.F.);
#8387=ORIENTED_EDGE('',*,*,#5887,.T.);
#8388=ORIENTED_EDGE('',*,*,#5885,.T.);
#8389=ORIENTED_EDGE('',*,*,#5883,.T.);
#8390=ORIENTED_EDGE('',*,*,#5881,.T.);
#8391=ORIENTED_EDGE('',*,*,#5787,.T.);
#8392=ORIENTED_EDGE('',*,*,#5225,.T.);
#8393=ORIENTED_EDGE('',*,*,#5784,.T.);
#8394=ORIENTED_EDGE('',*,*,#5275,.T.);
#8395=ORIENTED_EDGE('',*,*,#5795,.T.);
#8396=ORIENTED_EDGE('',*,*,#5125,.T.);
#8397=ORIENTED_EDGE('',*,*,#5792,.T.);
#8398=ORIENTED_EDGE('',*,*,#5175,.T.);
#8399=ORIENTED_EDGE('',*,*,#5803,.T.);
#8400=ORIENTED_EDGE('',*,*,#5025,.T.);
#8401=ORIENTED_EDGE('',*,*,#5800,.T.);
#8402=ORIENTED_EDGE('',*,*,#5075,.T.);
#8403=ORIENTED_EDGE('',*,*,#5811,.T.);
#8404=ORIENTED_EDGE('',*,*,#4925,.T.);
#8405=ORIENTED_EDGE('',*,*,#5808,.T.);
#8406=ORIENTED_EDGE('',*,*,#4975,.T.);
#8407=ORIENTED_EDGE('',*,*,#5868,.T.);
#8408=ORIENTED_EDGE('',*,*,#5878,.T.);
#8409=ORIENTED_EDGE('',*,*,#5875,.T.);
#8410=ORIENTED_EDGE('',*,*,#5872,.T.);
#9413=CYLINDRICAL_SURFACE('',#10506,1.666);
#9414=CYLINDRICAL_SURFACE('',#10509,1.666);
#9415=CYLINDRICAL_SURFACE('',#10510,1.666);
#9416=CYLINDRICAL_SURFACE('',#10511,1.666);
#9417=CYLINDRICAL_SURFACE('',#10512,1.666);
#9418=CYLINDRICAL_SURFACE('',#10513,1.666);
#9419=CYLINDRICAL_SURFACE('',#10514,1.666);
#9420=CYLINDRICAL_SURFACE('',#10515,1.666);
#9421=CYLINDRICAL_SURFACE('',#10516,1.666);
#9422=CYLINDRICAL_SURFACE('',#10517,1.666);
#9423=CYLINDRICAL_SURFACE('',#10518,1.666);
#9424=CYLINDRICAL_SURFACE('',#10519,1.666);
#9425=CYLINDRICAL_SURFACE('',#10520,1.666);
#9426=CYLINDRICAL_SURFACE('',#10521,1.666);
#9427=CYLINDRICAL_SURFACE('',#10522,1.666);
#9428=CYLINDRICAL_SURFACE('',#10524,2.05475000000001);
#9429=CYLINDRICAL_SURFACE('',#10526,2.05475000000001);
#9430=CYLINDRICAL_SURFACE('',#10527,2.05475000000001);
#9431=CYLINDRICAL_SURFACE('',#10528,2.05475000000001);
#9432=CYLINDRICAL_SURFACE('',#10529,2.05475000000001);
#9433=CYLINDRICAL_SURFACE('',#10530,2.05475000000001);
#9434=CYLINDRICAL_SURFACE('',#10531,2.05475000000001);
#9435=CYLINDRICAL_SURFACE('',#10532,2.05475000000001);
#9436=CYLINDRICAL_SURFACE('',#10533,2.05475000000001);
#9437=CYLINDRICAL_SURFACE('',#10534,2.05475000000001);
#9438=CYLINDRICAL_SURFACE('',#10535,2.05475000000001);
#9439=CYLINDRICAL_SURFACE('',#10536,2.05475000000001);
#9440=CYLINDRICAL_SURFACE('',#10537,2.05475000000001);
#9441=CYLINDRICAL_SURFACE('',#10538,2.05475000000001);
#9442=CYLINDRICAL_SURFACE('',#10539,2.05475000000001);
#9443=CYLINDRICAL_SURFACE('',#10540,2.05475000000001);
#9444=CYLINDRICAL_SURFACE('',#10542,1.666);
#9445=CYLINDRICAL_SURFACE('',#10545,1.666);
#9446=CYLINDRICAL_SURFACE('',#10546,1.666);
#9447=CYLINDRICAL_SURFACE('',#10547,1.666);
#9448=CYLINDRICAL_SURFACE('',#10548,1.666);
#9449=CYLINDRICAL_SURFACE('',#10549,1.666);
#9450=CYLINDRICAL_SURFACE('',#10550,1.666);
#9451=CYLINDRICAL_SURFACE('',#10551,1.666);
#9452=CYLINDRICAL_SURFACE('',#10552,1.666);
#9453=CYLINDRICAL_SURFACE('',#10553,1.666);
#9454=CYLINDRICAL_SURFACE('',#10554,1.666);
#9455=CYLINDRICAL_SURFACE('',#10555,1.666);
#9456=CYLINDRICAL_SURFACE('',#10556,1.666);
#9457=CYLINDRICAL_SURFACE('',#10557,1.666);
#9458=CYLINDRICAL_SURFACE('',#10558,1.666);
#9459=CYLINDRICAL_SURFACE('',#10560,2.05475);
#9460=CYLINDRICAL_SURFACE('',#10562,2.05475);
#9461=CYLINDRICAL_SURFACE('',#10563,2.05475);
#9462=CYLINDRICAL_SURFACE('',#10564,2.05475);
#9463=CYLINDRICAL_SURFACE('',#10565,2.05475);
#9464=CYLINDRICAL_SURFACE('',#10566,2.05475);
#9465=CYLINDRICAL_SURFACE('',#10567,2.05475);
#9466=CYLINDRICAL_SURFACE('',#10568,2.05475);
#9467=CYLINDRICAL_SURFACE('',#10569,2.05475);
#9468=CYLINDRICAL_SURFACE('',#10570,2.05475);
#9469=CYLINDRICAL_SURFACE('',#10571,2.05475);
#9470=CYLINDRICAL_SURFACE('',#10572,2.05475);
#9471=CYLINDRICAL_SURFACE('',#10573,2.05475);
#9472=CYLINDRICAL_SURFACE('',#10574,2.05475);
#9473=CYLINDRICAL_SURFACE('',#10575,2.05475);
#9474=CYLINDRICAL_SURFACE('',#10576,2.05475);
#9475=CYLINDRICAL_SURFACE('',#10578,1.666);
#9476=CYLINDRICAL_SURFACE('',#10581,1.666);
#9477=CYLINDRICAL_SURFACE('',#10582,1.666);
#9478=CYLINDRICAL_SURFACE('',#10583,1.666);
#9479=CYLINDRICAL_SURFACE('',#10584,1.666);
#9480=CYLINDRICAL_SURFACE('',#10585,1.666);
#9481=CYLINDRICAL_SURFACE('',#10586,1.666);
#9482=CYLINDRICAL_SURFACE('',#10587,1.666);
#9483=CYLINDRICAL_SURFACE('',#10588,1.666);
#9484=CYLINDRICAL_SURFACE('',#10589,1.666);
#9485=CYLINDRICAL_SURFACE('',#10590,1.666);
#9486=CYLINDRICAL_SURFACE('',#10591,1.666);
#9487=CYLINDRICAL_SURFACE('',#10592,1.666);
#9488=CYLINDRICAL_SURFACE('',#10593,1.666);
#9489=CYLINDRICAL_SURFACE('',#10594,1.666);
#9490=CYLINDRICAL_SURFACE('',#10596,2.05475000000001);
#9491=CYLINDRICAL_SURFACE('',#10598,2.05475000000001);
#9492=CYLINDRICAL_SURFACE('',#10599,2.05475000000001);
#9493=CYLINDRICAL_SURFACE('',#10600,2.05475000000001);
#9494=CYLINDRICAL_SURFACE('',#10601,2.05475000000001);
#9495=CYLINDRICAL_SURFACE('',#10602,2.05475000000001);
#9496=CYLINDRICAL_SURFACE('',#10603,2.05475000000001);
#9497=CYLINDRICAL_SURFACE('',#10604,2.05475000000001);
#9498=CYLINDRICAL_SURFACE('',#10605,2.05475000000001);
#9499=CYLINDRICAL_SURFACE('',#10606,2.05475000000001);
#9500=CYLINDRICAL_SURFACE('',#10607,2.05475000000001);
#9501=CYLINDRICAL_SURFACE('',#10608,2.05475000000001);
#9502=CYLINDRICAL_SURFACE('',#10609,2.05475000000001);
#9503=CYLINDRICAL_SURFACE('',#10610,2.05475000000001);
#9504=CYLINDRICAL_SURFACE('',#10611,2.05475000000001);
#9505=CYLINDRICAL_SURFACE('',#10612,2.05475000000001);
#9506=CYLINDRICAL_SURFACE('',#10614,1.666);
#9507=CYLINDRICAL_SURFACE('',#10617,1.666);
#9508=CYLINDRICAL_SURFACE('',#10618,1.666);
#9509=CYLINDRICAL_SURFACE('',#10619,1.666);
#9510=CYLINDRICAL_SURFACE('',#10620,1.666);
#9511=CYLINDRICAL_SURFACE('',#10621,1.666);
#9512=CYLINDRICAL_SURFACE('',#10622,1.666);
#9513=CYLINDRICAL_SURFACE('',#10623,1.666);
#9514=CYLINDRICAL_SURFACE('',#10624,1.666);
#9515=CYLINDRICAL_SURFACE('',#10625,1.666);
#9516=CYLINDRICAL_SURFACE('',#10626,1.666);
#9517=CYLINDRICAL_SURFACE('',#10627,1.666);
#9518=CYLINDRICAL_SURFACE('',#10628,1.666);
#9519=CYLINDRICAL_SURFACE('',#10629,1.666);
#9520=CYLINDRICAL_SURFACE('',#10630,1.666);
#9521=CYLINDRICAL_SURFACE('',#10632,2.05475);
#9522=CYLINDRICAL_SURFACE('',#10634,2.05475);
#9523=CYLINDRICAL_SURFACE('',#10635,2.05475);
#9524=CYLINDRICAL_SURFACE('',#10636,2.05475);
#9525=CYLINDRICAL_SURFACE('',#10637,2.05475);
#9526=CYLINDRICAL_SURFACE('',#10638,2.05475);
#9527=CYLINDRICAL_SURFACE('',#10639,2.05475);
#9528=CYLINDRICAL_SURFACE('',#10640,2.05475);
#9529=CYLINDRICAL_SURFACE('',#10641,2.05475);
#9530=CYLINDRICAL_SURFACE('',#10642,2.05475);
#9531=CYLINDRICAL_SURFACE('',#10643,2.05475);
#9532=CYLINDRICAL_SURFACE('',#10644,2.05475);
#9533=CYLINDRICAL_SURFACE('',#10645,2.05475);
#9534=CYLINDRICAL_SURFACE('',#10646,2.05475);
#9535=CYLINDRICAL_SURFACE('',#10647,2.05475);
#9536=CYLINDRICAL_SURFACE('',#10648,2.05475);
#9537=CYLINDRICAL_SURFACE('',#10650,2.5175);
#9538=CYLINDRICAL_SURFACE('',#10653,2.5175);
#9539=CYLINDRICAL_SURFACE('',#10654,2.5175);
#9540=CYLINDRICAL_SURFACE('',#10655,2.5175);
#9541=CYLINDRICAL_SURFACE('',#10656,2.5175);
#9542=CYLINDRICAL_SURFACE('',#10657,2.5175);
#9543=CYLINDRICAL_SURFACE('',#10658,2.5175);
#9544=CYLINDRICAL_SURFACE('',#10659,2.5175);
#9545=CYLINDRICAL_SURFACE('',#10660,2.5175);
#9546=CYLINDRICAL_SURFACE('',#10661,2.5175);
#9547=CYLINDRICAL_SURFACE('',#10662,2.5175);
#9548=CYLINDRICAL_SURFACE('',#10663,2.5175);
#9549=CYLINDRICAL_SURFACE('',#10664,2.5175);
#9550=CYLINDRICAL_SURFACE('',#10665,2.5175);
#9551=CYLINDRICAL_SURFACE('',#10666,2.5175);
#9552=CYLINDRICAL_SURFACE('',#10668,2.5175);
#9553=CYLINDRICAL_SURFACE('',#10671,2.5175);
#9554=CYLINDRICAL_SURFACE('',#10672,2.5175);
#9555=CYLINDRICAL_SURFACE('',#10673,2.5175);
#9556=CYLINDRICAL_SURFACE('',#10674,2.5175);
#9557=CYLINDRICAL_SURFACE('',#10675,2.5175);
#9558=CYLINDRICAL_SURFACE('',#10676,2.5175);
#9559=CYLINDRICAL_SURFACE('',#10677,2.5175);
#9560=CYLINDRICAL_SURFACE('',#10678,2.5175);
#9561=CYLINDRICAL_SURFACE('',#10679,2.5175);
#9562=CYLINDRICAL_SURFACE('',#10680,2.5175);
#9563=CYLINDRICAL_SURFACE('',#10681,2.5175);
#9564=CYLINDRICAL_SURFACE('',#10682,2.5175);
#9565=CYLINDRICAL_SURFACE('',#10683,2.5175);
#9566=CYLINDRICAL_SURFACE('',#10684,2.5175);
#9567=CYLINDRICAL_SURFACE('',#10686,3.0735);
#9568=CYLINDRICAL_SURFACE('',#10688,3.0735);
#9569=CYLINDRICAL_SURFACE('',#10689,3.0735);
#9570=CYLINDRICAL_SURFACE('',#10690,3.0735);
#9571=CYLINDRICAL_SURFACE('',#10691,3.0735);
#9572=CYLINDRICAL_SURFACE('',#10692,3.0735);
#9573=CYLINDRICAL_SURFACE('',#10693,3.0735);
#9574=CYLINDRICAL_SURFACE('',#10694,3.0735);
#9575=CYLINDRICAL_SURFACE('',#10695,3.0735);
#9576=CYLINDRICAL_SURFACE('',#10696,3.0735);
#9577=CYLINDRICAL_SURFACE('',#10697,3.0735);
#9578=CYLINDRICAL_SURFACE('',#10698,3.0735);
#9579=CYLINDRICAL_SURFACE('',#10699,3.0735);
#9580=CYLINDRICAL_SURFACE('',#10700,3.0735);
#9581=CYLINDRICAL_SURFACE('',#10701,3.0735);
#9582=CYLINDRICAL_SURFACE('',#10703,3.0735);
#9583=CYLINDRICAL_SURFACE('',#10705,3.0735);
#9584=CYLINDRICAL_SURFACE('',#10706,3.0735);
#9585=CYLINDRICAL_SURFACE('',#10707,3.0735);
#9586=CYLINDRICAL_SURFACE('',#10708,3.0735);
#9587=CYLINDRICAL_SURFACE('',#10709,3.0735);
#9588=CYLINDRICAL_SURFACE('',#10710,3.0735);
#9589=CYLINDRICAL_SURFACE('',#10711,3.0735);
#9590=CYLINDRICAL_SURFACE('',#10712,3.0735);
#9591=CYLINDRICAL_SURFACE('',#10713,3.0735);
#9592=CYLINDRICAL_SURFACE('',#10714,3.0735);
#9593=CYLINDRICAL_SURFACE('',#10715,3.0735);
#9594=CYLINDRICAL_SURFACE('',#10716,3.0735);
#9595=CYLINDRICAL_SURFACE('',#10717,3.0735);
#9596=CYLINDRICAL_SURFACE('',#10718,3.07350000000001);
#9597=CYLINDRICAL_SURFACE('',#10720,2.5175);
#9598=CYLINDRICAL_SURFACE('',#10724,2.5175);
#9599=CYLINDRICAL_SURFACE('',#10725,2.5175);
#9600=CYLINDRICAL_SURFACE('',#10726,2.5175);
#9601=CYLINDRICAL_SURFACE('',#10727,2.5175);
#9602=CYLINDRICAL_SURFACE('',#10728,2.5175);
#9603=CYLINDRICAL_SURFACE('',#10729,2.5175);
#9604=CYLINDRICAL_SURFACE('',#10730,2.5175);
#9605=CYLINDRICAL_SURFACE('',#10731,2.5175);
#9606=CYLINDRICAL_SURFACE('',#10732,2.5175);
#9607=CYLINDRICAL_SURFACE('',#10733,2.5175);
#9608=CYLINDRICAL_SURFACE('',#10734,2.5175);
#9609=CYLINDRICAL_SURFACE('',#10735,2.5175);
#9610=CYLINDRICAL_SURFACE('',#10736,2.5175);
#9611=CYLINDRICAL_SURFACE('',#10737,2.5175);
#9612=CYLINDRICAL_SURFACE('',#10739,3.0735);
#9613=CYLINDRICAL_SURFACE('',#10741,3.0735);
#9614=CYLINDRICAL_SURFACE('',#10742,3.0735);
#9615=CYLINDRICAL_SURFACE('',#10743,3.0735);
#9616=CYLINDRICAL_SURFACE('',#10744,3.0735);
#9617=CYLINDRICAL_SURFACE('',#10745,3.0735);
#9618=CYLINDRICAL_SURFACE('',#10746,3.0735);
#9619=CYLINDRICAL_SURFACE('',#10747,3.0735);
#9620=CYLINDRICAL_SURFACE('',#10748,3.0735);
#9621=CYLINDRICAL_SURFACE('',#10749,3.0735);
#9622=CYLINDRICAL_SURFACE('',#10750,3.0735);
#9623=CYLINDRICAL_SURFACE('',#10751,3.0735);
#9624=CYLINDRICAL_SURFACE('',#10752,3.0735);
#9625=CYLINDRICAL_SURFACE('',#10753,3.0735);
#9626=CYLINDRICAL_SURFACE('',#10754,3.0735);
#9627=CYLINDRICAL_SURFACE('',#10756,2.5175);
#9628=CYLINDRICAL_SURFACE('',#10760,2.5175);
#9629=CYLINDRICAL_SURFACE('',#10761,2.5175);
#9630=CYLINDRICAL_SURFACE('',#10762,2.5175);
#9631=CYLINDRICAL_SURFACE('',#10763,2.5175);
#9632=CYLINDRICAL_SURFACE('',#10764,2.5175);
#9633=CYLINDRICAL_SURFACE('',#10765,2.5175);
#9634=CYLINDRICAL_SURFACE('',#10766,2.5175);
#9635=CYLINDRICAL_SURFACE('',#10767,2.5175);
#9636=CYLINDRICAL_SURFACE('',#10768,2.5175);
#9637=CYLINDRICAL_SURFACE('',#10769,2.5175);
#9638=CYLINDRICAL_SURFACE('',#10770,2.5175);
#9639=CYLINDRICAL_SURFACE('',#10771,2.5175);
#9640=CYLINDRICAL_SURFACE('',#10772,2.5175);
#9641=CYLINDRICAL_SURFACE('',#10773,2.5175);
#9642=CYLINDRICAL_SURFACE('',#10775,3.0735);
#9643=CYLINDRICAL_SURFACE('',#10777,3.0735);
#9644=CYLINDRICAL_SURFACE('',#10778,3.0735);
#9645=CYLINDRICAL_SURFACE('',#10779,3.0735);
#9646=CYLINDRICAL_SURFACE('',#10780,3.0735);
#9647=CYLINDRICAL_SURFACE('',#10781,3.0735);
#9648=CYLINDRICAL_SURFACE('',#10782,3.0735);
#9649=CYLINDRICAL_SURFACE('',#10783,3.0735);
#9650=CYLINDRICAL_SURFACE('',#10784,3.0735);
#9651=CYLINDRICAL_SURFACE('',#10785,3.0735);
#9652=CYLINDRICAL_SURFACE('',#10786,3.0735);
#9653=CYLINDRICAL_SURFACE('',#10787,3.0735);
#9654=CYLINDRICAL_SURFACE('',#10788,3.0735);
#9655=CYLINDRICAL_SURFACE('',#10789,3.0735);
#9656=CYLINDRICAL_SURFACE('',#10790,3.0735);
#9657=CYLINDRICAL_SURFACE('',#10792,7.263);
#9658=CYLINDRICAL_SURFACE('',#10794,7.263);
#9659=CYLINDRICAL_SURFACE('',#10795,7.263);
#9660=CYLINDRICAL_SURFACE('',#10796,7.263);
#9661=CYLINDRICAL_SURFACE('',#10797,7.263);
#9662=CYLINDRICAL_SURFACE('',#10798,7.263);
#9663=CYLINDRICAL_SURFACE('',#10799,7.263);
#9664=CYLINDRICAL_SURFACE('',#10800,7.263);
#9665=CYLINDRICAL_SURFACE('',#10802,8.1015);
#9666=CYLINDRICAL_SURFACE('',#10804,8.1015);
#9667=CYLINDRICAL_SURFACE('',#10805,8.1015);
#9668=CYLINDRICAL_SURFACE('',#10806,8.1015);
#9669=CYLINDRICAL_SURFACE('',#10807,8.1015);
#9670=CYLINDRICAL_SURFACE('',#10808,8.1015);
#9671=CYLINDRICAL_SURFACE('',#10809,8.1015);
#9672=CYLINDRICAL_SURFACE('',#10810,8.1015);
#9673=CYLINDRICAL_SURFACE('',#10812,8.1015);
#9674=CYLINDRICAL_SURFACE('',#10815,7.263);
#9675=CYLINDRICAL_SURFACE('',#10816,12.);
#9676=CYLINDRICAL_SURFACE('',#10820,3.0735);
#9677=CYLINDRICAL_SURFACE('',#10821,2.5175);
#9678=CYLINDRICAL_SURFACE('',#10823,3.0735);
#9679=CYLINDRICAL_SURFACE('',#10824,2.5175);
#9680=CYLINDRICAL_SURFACE('',#10829,3.0735);
#9681=CYLINDRICAL_SURFACE('',#10830,2.5175);
#9682=CYLINDRICAL_SURFACE('',#10835,3.0735);
#9683=CYLINDRICAL_SURFACE('',#10836,2.5175);
#9684=CYLINDRICAL_SURFACE('',#10837,2.5175);
#9685=CYLINDRICAL_SURFACE('',#10840,2.5175);
#9686=CYLINDRICAL_SURFACE('',#10842,2.05475);
#9687=CYLINDRICAL_SURFACE('',#10843,1.666);
#9688=CYLINDRICAL_SURFACE('',#10845,2.05475000000001);
#9689=CYLINDRICAL_SURFACE('',#10846,1.666);
#9690=CYLINDRICAL_SURFACE('',#10848,2.05475);
#9691=CYLINDRICAL_SURFACE('',#10849,1.666);
#9692=CYLINDRICAL_SURFACE('',#10851,2.05475000000001);
#9693=CYLINDRICAL_SURFACE('',#10852,1.666);
#9694=CYLINDRICAL_SURFACE('',#10857,5.);
#9695=CYLINDRICAL_SURFACE('',#10860,5.);
#9696=CYLINDRICAL_SURFACE('',#10863,5.);
#9697=CYLINDRICAL_SURFACE('',#10866,5.);
#9698=CYLINDRICAL_SURFACE('',#10869,5.);
#9699=CYLINDRICAL_SURFACE('',#10872,5.);
#9700=CYLINDRICAL_SURFACE('',#10875,5.);
#9701=CYLINDRICAL_SURFACE('',#10878,5.);
#9702=CYLINDRICAL_SURFACE('',#10881,5.);
#9703=CYLINDRICAL_SURFACE('',#10884,5.);
#9704=CYLINDRICAL_SURFACE('',#10887,5.);
#9705=CYLINDRICAL_SURFACE('',#10890,5.);
#9706=CYLINDRICAL_SURFACE('',#10893,5.);
#9707=CYLINDRICAL_SURFACE('',#10896,5.);
#9708=CYLINDRICAL_SURFACE('',#10899,5.);
#9709=CYLINDRICAL_SURFACE('',#10902,5.);
#9710=CYLINDRICAL_SURFACE('',#10905,5.);
#9711=CYLINDRICAL_SURFACE('',#10908,5.);
#9839=ADVANCED_FACE('',(#603),#9413,.F.);
#9840=ADVANCED_FACE('',(#604),#9414,.F.);
#9841=ADVANCED_FACE('',(#605),#9415,.F.);
#9842=ADVANCED_FACE('',(#606),#9416,.F.);
#9843=ADVANCED_FACE('',(#607),#9417,.F.);
#9844=ADVANCED_FACE('',(#608),#9418,.F.);
#9845=ADVANCED_FACE('',(#609),#9419,.F.);
#9846=ADVANCED_FACE('',(#610),#9420,.F.);
#9847=ADVANCED_FACE('',(#611),#9421,.F.);
#9848=ADVANCED_FACE('',(#612),#9422,.F.);
#9849=ADVANCED_FACE('',(#613),#9423,.F.);
#9850=ADVANCED_FACE('',(#614),#9424,.F.);
#9851=ADVANCED_FACE('',(#615),#9425,.F.);
#9852=ADVANCED_FACE('',(#616),#9426,.F.);
#9853=ADVANCED_FACE('',(#617),#9427,.F.);
#9854=ADVANCED_FACE('',(#618),#9428,.F.);
#9855=ADVANCED_FACE('',(#619),#9429,.F.);
#9856=ADVANCED_FACE('',(#620),#9430,.F.);
#9857=ADVANCED_FACE('',(#621),#9431,.F.);
#9858=ADVANCED_FACE('',(#622),#9432,.F.);
#9859=ADVANCED_FACE('',(#623),#9433,.F.);
#9860=ADVANCED_FACE('',(#624),#9434,.F.);
#9861=ADVANCED_FACE('',(#625),#9435,.F.);
#9862=ADVANCED_FACE('',(#626),#9436,.F.);
#9863=ADVANCED_FACE('',(#627),#9437,.F.);
#9864=ADVANCED_FACE('',(#628),#9438,.F.);
#9865=ADVANCED_FACE('',(#629),#9439,.F.);
#9866=ADVANCED_FACE('',(#630),#9440,.F.);
#9867=ADVANCED_FACE('',(#631),#9441,.F.);
#9868=ADVANCED_FACE('',(#632),#9442,.F.);
#9869=ADVANCED_FACE('',(#633),#9443,.F.);
#9870=ADVANCED_FACE('',(#634),#9444,.F.);
#9871=ADVANCED_FACE('',(#635),#9445,.F.);
#9872=ADVANCED_FACE('',(#636),#9446,.F.);
#9873=ADVANCED_FACE('',(#637),#9447,.F.);
#9874=ADVANCED_FACE('',(#638),#9448,.F.);
#9875=ADVANCED_FACE('',(#639),#9449,.F.);
#9876=ADVANCED_FACE('',(#640),#9450,.F.);
#9877=ADVANCED_FACE('',(#641),#9451,.F.);
#9878=ADVANCED_FACE('',(#642),#9452,.F.);
#9879=ADVANCED_FACE('',(#643),#9453,.F.);
#9880=ADVANCED_FACE('',(#644),#9454,.F.);
#9881=ADVANCED_FACE('',(#645),#9455,.F.);
#9882=ADVANCED_FACE('',(#646),#9456,.F.);
#9883=ADVANCED_FACE('',(#647),#9457,.F.);
#9884=ADVANCED_FACE('',(#648),#9458,.F.);
#9885=ADVANCED_FACE('',(#649),#9459,.F.);
#9886=ADVANCED_FACE('',(#650),#9460,.F.);
#9887=ADVANCED_FACE('',(#651),#9461,.F.);
#9888=ADVANCED_FACE('',(#652),#9462,.F.);
#9889=ADVANCED_FACE('',(#653),#9463,.F.);
#9890=ADVANCED_FACE('',(#654),#9464,.F.);
#9891=ADVANCED_FACE('',(#655),#9465,.F.);
#9892=ADVANCED_FACE('',(#656),#9466,.F.);
#9893=ADVANCED_FACE('',(#657),#9467,.F.);
#9894=ADVANCED_FACE('',(#658),#9468,.F.);
#9895=ADVANCED_FACE('',(#659),#9469,.F.);
#9896=ADVANCED_FACE('',(#660),#9470,.F.);
#9897=ADVANCED_FACE('',(#661),#9471,.F.);
#9898=ADVANCED_FACE('',(#662),#9472,.F.);
#9899=ADVANCED_FACE('',(#663),#9473,.F.);
#9900=ADVANCED_FACE('',(#664),#9474,.F.);
#9901=ADVANCED_FACE('',(#665),#9475,.F.);
#9902=ADVANCED_FACE('',(#666),#9476,.F.);
#9903=ADVANCED_FACE('',(#667),#9477,.F.);
#9904=ADVANCED_FACE('',(#668),#9478,.F.);
#9905=ADVANCED_FACE('',(#669),#9479,.F.);
#9906=ADVANCED_FACE('',(#670),#9480,.F.);
#9907=ADVANCED_FACE('',(#671),#9481,.F.);
#9908=ADVANCED_FACE('',(#672),#9482,.F.);
#9909=ADVANCED_FACE('',(#673),#9483,.F.);
#9910=ADVANCED_FACE('',(#674),#9484,.F.);
#9911=ADVANCED_FACE('',(#675),#9485,.F.);
#9912=ADVANCED_FACE('',(#676),#9486,.F.);
#9913=ADVANCED_FACE('',(#677),#9487,.F.);
#9914=ADVANCED_FACE('',(#678),#9488,.F.);
#9915=ADVANCED_FACE('',(#679),#9489,.F.);
#9916=ADVANCED_FACE('',(#680),#9490,.F.);
#9917=ADVANCED_FACE('',(#681),#9491,.F.);
#9918=ADVANCED_FACE('',(#682),#9492,.F.);
#9919=ADVANCED_FACE('',(#683),#9493,.F.);
#9920=ADVANCED_FACE('',(#684),#9494,.F.);
#9921=ADVANCED_FACE('',(#685),#9495,.F.);
#9922=ADVANCED_FACE('',(#686),#9496,.F.);
#9923=ADVANCED_FACE('',(#687),#9497,.F.);
#9924=ADVANCED_FACE('',(#688),#9498,.F.);
#9925=ADVANCED_FACE('',(#689),#9499,.F.);
#9926=ADVANCED_FACE('',(#690),#9500,.F.);
#9927=ADVANCED_FACE('',(#691),#9501,.F.);
#9928=ADVANCED_FACE('',(#692),#9502,.F.);
#9929=ADVANCED_FACE('',(#693),#9503,.F.);
#9930=ADVANCED_FACE('',(#694),#9504,.F.);
#9931=ADVANCED_FACE('',(#695),#9505,.F.);
#9932=ADVANCED_FACE('',(#696),#9506,.F.);
#9933=ADVANCED_FACE('',(#697),#9507,.F.);
#9934=ADVANCED_FACE('',(#698),#9508,.F.);
#9935=ADVANCED_FACE('',(#699),#9509,.F.);
#9936=ADVANCED_FACE('',(#700),#9510,.F.);
#9937=ADVANCED_FACE('',(#701),#9511,.F.);
#9938=ADVANCED_FACE('',(#702),#9512,.F.);
#9939=ADVANCED_FACE('',(#703),#9513,.F.);
#9940=ADVANCED_FACE('',(#704),#9514,.F.);
#9941=ADVANCED_FACE('',(#705),#9515,.F.);
#9942=ADVANCED_FACE('',(#706),#9516,.F.);
#9943=ADVANCED_FACE('',(#707),#9517,.F.);
#9944=ADVANCED_FACE('',(#708),#9518,.F.);
#9945=ADVANCED_FACE('',(#709),#9519,.F.);
#9946=ADVANCED_FACE('',(#710),#9520,.F.);
#9947=ADVANCED_FACE('',(#711),#9521,.F.);
#9948=ADVANCED_FACE('',(#712),#9522,.F.);
#9949=ADVANCED_FACE('',(#713),#9523,.F.);
#9950=ADVANCED_FACE('',(#714),#9524,.F.);
#9951=ADVANCED_FACE('',(#715),#9525,.F.);
#9952=ADVANCED_FACE('',(#716),#9526,.F.);
#9953=ADVANCED_FACE('',(#717),#9527,.F.);
#9954=ADVANCED_FACE('',(#718),#9528,.F.);
#9955=ADVANCED_FACE('',(#719),#9529,.F.);
#9956=ADVANCED_FACE('',(#720),#9530,.F.);
#9957=ADVANCED_FACE('',(#721),#9531,.F.);
#9958=ADVANCED_FACE('',(#722),#9532,.F.);
#9959=ADVANCED_FACE('',(#723),#9533,.F.);
#9960=ADVANCED_FACE('',(#724),#9534,.F.);
#9961=ADVANCED_FACE('',(#725),#9535,.F.);
#9962=ADVANCED_FACE('',(#726),#9536,.F.);
#9963=ADVANCED_FACE('',(#727),#9537,.F.);
#9964=ADVANCED_FACE('',(#728),#9538,.F.);
#9965=ADVANCED_FACE('',(#729),#9539,.F.);
#9966=ADVANCED_FACE('',(#730),#9540,.F.);
#9967=ADVANCED_FACE('',(#731),#9541,.F.);
#9968=ADVANCED_FACE('',(#732),#9542,.F.);
#9969=ADVANCED_FACE('',(#733),#9543,.F.);
#9970=ADVANCED_FACE('',(#734),#9544,.F.);
#9971=ADVANCED_FACE('',(#735),#9545,.F.);
#9972=ADVANCED_FACE('',(#736),#9546,.F.);
#9973=ADVANCED_FACE('',(#737),#9547,.F.);
#9974=ADVANCED_FACE('',(#738),#9548,.F.);
#9975=ADVANCED_FACE('',(#739),#9549,.F.);
#9976=ADVANCED_FACE('',(#740),#9550,.F.);
#9977=ADVANCED_FACE('',(#741),#9551,.F.);
#9978=ADVANCED_FACE('',(#742),#9552,.F.);
#9979=ADVANCED_FACE('',(#743),#9553,.F.);
#9980=ADVANCED_FACE('',(#744),#9554,.F.);
#9981=ADVANCED_FACE('',(#745),#9555,.F.);
#9982=ADVANCED_FACE('',(#746),#9556,.F.);
#9983=ADVANCED_FACE('',(#747),#9557,.F.);
#9984=ADVANCED_FACE('',(#748),#9558,.F.);
#9985=ADVANCED_FACE('',(#749),#9559,.F.);
#9986=ADVANCED_FACE('',(#750),#9560,.F.);
#9987=ADVANCED_FACE('',(#751),#9561,.F.);
#9988=ADVANCED_FACE('',(#752),#9562,.F.);
#9989=ADVANCED_FACE('',(#753),#9563,.F.);
#9990=ADVANCED_FACE('',(#754),#9564,.F.);
#9991=ADVANCED_FACE('',(#755),#9565,.F.);
#9992=ADVANCED_FACE('',(#756),#9566,.F.);
#9993=ADVANCED_FACE('',(#757),#9567,.F.);
#9994=ADVANCED_FACE('',(#758),#9568,.F.);
#9995=ADVANCED_FACE('',(#759),#9569,.F.);
#9996=ADVANCED_FACE('',(#760),#9570,.F.);
#9997=ADVANCED_FACE('',(#761),#9571,.F.);
#9998=ADVANCED_FACE('',(#762),#9572,.F.);
#9999=ADVANCED_FACE('',(#763),#9573,.F.);
#10000=ADVANCED_FACE('',(#764),#9574,.F.);
#10001=ADVANCED_FACE('',(#765),#9575,.F.);
#10002=ADVANCED_FACE('',(#766),#9576,.F.);
#10003=ADVANCED_FACE('',(#767),#9577,.F.);
#10004=ADVANCED_FACE('',(#768),#9578,.F.);
#10005=ADVANCED_FACE('',(#769),#9579,.F.);
#10006=ADVANCED_FACE('',(#770),#9580,.F.);
#10007=ADVANCED_FACE('',(#771),#9581,.F.);
#10008=ADVANCED_FACE('',(#772),#9582,.F.);
#10009=ADVANCED_FACE('',(#773),#9583,.F.);
#10010=ADVANCED_FACE('',(#774),#9584,.F.);
#10011=ADVANCED_FACE('',(#775),#9585,.F.);
#10012=ADVANCED_FACE('',(#776),#9586,.F.);
#10013=ADVANCED_FACE('',(#777),#9587,.F.);
#10014=ADVANCED_FACE('',(#778),#9588,.F.);
#10015=ADVANCED_FACE('',(#779),#9589,.F.);
#10016=ADVANCED_FACE('',(#780),#9590,.F.);
#10017=ADVANCED_FACE('',(#781),#9591,.F.);
#10018=ADVANCED_FACE('',(#782),#9592,.F.);
#10019=ADVANCED_FACE('',(#783),#9593,.F.);
#10020=ADVANCED_FACE('',(#784),#9594,.F.);
#10021=ADVANCED_FACE('',(#785),#9595,.F.);
#10022=ADVANCED_FACE('',(#786),#9596,.F.);
#10023=ADVANCED_FACE('',(#787),#9597,.F.);
#10024=ADVANCED_FACE('',(#788),#9598,.F.);
#10025=ADVANCED_FACE('',(#789),#9599,.F.);
#10026=ADVANCED_FACE('',(#790),#9600,.F.);
#10027=ADVANCED_FACE('',(#791),#9601,.F.);
#10028=ADVANCED_FACE('',(#792),#9602,.F.);
#10029=ADVANCED_FACE('',(#793),#9603,.F.);
#10030=ADVANCED_FACE('',(#794),#9604,.F.);
#10031=ADVANCED_FACE('',(#795),#9605,.F.);
#10032=ADVANCED_FACE('',(#796),#9606,.F.);
#10033=ADVANCED_FACE('',(#797),#9607,.F.);
#10034=ADVANCED_FACE('',(#798),#9608,.F.);
#10035=ADVANCED_FACE('',(#799),#9609,.F.);
#10036=ADVANCED_FACE('',(#800),#9610,.F.);
#10037=ADVANCED_FACE('',(#801),#9611,.F.);
#10038=ADVANCED_FACE('',(#802),#9612,.F.);
#10039=ADVANCED_FACE('',(#803),#9613,.F.);
#10040=ADVANCED_FACE('',(#804),#9614,.F.);
#10041=ADVANCED_FACE('',(#805),#9615,.F.);
#10042=ADVANCED_FACE('',(#806),#9616,.F.);
#10043=ADVANCED_FACE('',(#807),#9617,.F.);
#10044=ADVANCED_FACE('',(#808),#9618,.F.);
#10045=ADVANCED_FACE('',(#809),#9619,.F.);
#10046=ADVANCED_FACE('',(#810),#9620,.F.);
#10047=ADVANCED_FACE('',(#811),#9621,.F.);
#10048=ADVANCED_FACE('',(#812),#9622,.F.);
#10049=ADVANCED_FACE('',(#813),#9623,.F.);
#10050=ADVANCED_FACE('',(#814),#9624,.F.);
#10051=ADVANCED_FACE('',(#815),#9625,.F.);
#10052=ADVANCED_FACE('',(#816),#9626,.F.);
#10053=ADVANCED_FACE('',(#817),#9627,.F.);
#10054=ADVANCED_FACE('',(#818),#9628,.F.);
#10055=ADVANCED_FACE('',(#819),#9629,.F.);
#10056=ADVANCED_FACE('',(#820),#9630,.F.);
#10057=ADVANCED_FACE('',(#821),#9631,.F.);
#10058=ADVANCED_FACE('',(#822),#9632,.F.);
#10059=ADVANCED_FACE('',(#823),#9633,.F.);
#10060=ADVANCED_FACE('',(#824),#9634,.F.);
#10061=ADVANCED_FACE('',(#825),#9635,.F.);
#10062=ADVANCED_FACE('',(#826),#9636,.F.);
#10063=ADVANCED_FACE('',(#827),#9637,.F.);
#10064=ADVANCED_FACE('',(#828),#9638,.F.);
#10065=ADVANCED_FACE('',(#829),#9639,.F.);
#10066=ADVANCED_FACE('',(#830),#9640,.F.);
#10067=ADVANCED_FACE('',(#831),#9641,.F.);
#10068=ADVANCED_FACE('',(#832),#9642,.F.);
#10069=ADVANCED_FACE('',(#833),#9643,.F.);
#10070=ADVANCED_FACE('',(#834),#9644,.F.);
#10071=ADVANCED_FACE('',(#835),#9645,.F.);
#10072=ADVANCED_FACE('',(#836),#9646,.F.);
#10073=ADVANCED_FACE('',(#837),#9647,.F.);
#10074=ADVANCED_FACE('',(#838),#9648,.F.);
#10075=ADVANCED_FACE('',(#839),#9649,.F.);
#10076=ADVANCED_FACE('',(#840),#9650,.F.);
#10077=ADVANCED_FACE('',(#841),#9651,.F.);
#10078=ADVANCED_FACE('',(#842),#9652,.F.);
#10079=ADVANCED_FACE('',(#843),#9653,.F.);
#10080=ADVANCED_FACE('',(#844),#9654,.F.);
#10081=ADVANCED_FACE('',(#845),#9655,.F.);
#10082=ADVANCED_FACE('',(#846),#9656,.F.);
#10083=ADVANCED_FACE('',(#847),#9657,.F.);
#10084=ADVANCED_FACE('',(#848),#9658,.F.);
#10085=ADVANCED_FACE('',(#849),#9659,.F.);
#10086=ADVANCED_FACE('',(#850),#9660,.F.);
#10087=ADVANCED_FACE('',(#851),#9661,.F.);
#10088=ADVANCED_FACE('',(#852),#9662,.F.);
#10089=ADVANCED_FACE('',(#853),#9663,.F.);
#10090=ADVANCED_FACE('',(#854),#9664,.F.);
#10091=ADVANCED_FACE('',(#855),#9665,.F.);
#10092=ADVANCED_FACE('',(#856),#9666,.F.);
#10093=ADVANCED_FACE('',(#857),#9667,.F.);
#10094=ADVANCED_FACE('',(#858),#9668,.F.);
#10095=ADVANCED_FACE('',(#859),#9669,.F.);
#10096=ADVANCED_FACE('',(#860),#9670,.F.);
#10097=ADVANCED_FACE('',(#861),#9671,.F.);
#10098=ADVANCED_FACE('',(#862),#9672,.F.);
#10099=ADVANCED_FACE('',(#863),#9673,.F.);
#10100=ADVANCED_FACE('',(#864),#579,.F.);
#10101=ADVANCED_FACE('',(#865),#580,.F.);
#10102=ADVANCED_FACE('',(#866,#353),#487,.F.);
#10103=ADVANCED_FACE('',(#867),#9674,.F.);
#10104=ADVANCED_FACE('',(#868),#9675,.T.);
#10105=ADVANCED_FACE('',(#869,#354,#355,#356,#357,#358),#488,.F.);
#10106=ADVANCED_FACE('',(#870),#489,.F.);
#10107=ADVANCED_FACE('',(#871),#9676,.F.);
#10108=ADVANCED_FACE('',(#872),#581,.F.);
#10109=ADVANCED_FACE('',(#873),#582,.F.);
#10110=ADVANCED_FACE('',(#874),#9677,.F.);
#10111=ADVANCED_FACE('',(#875),#490,.F.);
#10112=ADVANCED_FACE('',(#876),#9678,.F.);
#10113=ADVANCED_FACE('',(#877),#583,.F.);
#10114=ADVANCED_FACE('',(#878),#584,.F.);
#10115=ADVANCED_FACE('',(#879),#9679,.F.);
#10116=ADVANCED_FACE('',(#880),#491,.F.);
#10117=ADVANCED_FACE('',(#881),#492,.F.);
#10118=ADVANCED_FACE('',(#882),#493,.F.);
#10119=ADVANCED_FACE('',(#883),#9680,.F.);
#10120=ADVANCED_FACE('',(#884),#585,.F.);
#10121=ADVANCED_FACE('',(#885),#586,.F.);
#10122=ADVANCED_FACE('',(#886),#9681,.F.);
#10123=ADVANCED_FACE('',(#887),#494,.F.);
#10124=ADVANCED_FACE('',(#888),#495,.F.);
#10125=ADVANCED_FACE('',(#889),#496,.F.);
#10126=ADVANCED_FACE('',(#890),#9682,.F.);
#10127=ADVANCED_FACE('',(#891),#587,.F.);
#10128=ADVANCED_FACE('',(#892),#588,.F.);
#10129=ADVANCED_FACE('',(#893),#9683,.F.);
#10130=ADVANCED_FACE('',(#894),#9684,.F.);
#10131=ADVANCED_FACE('',(#895),#497,.F.);
#10132=ADVANCED_FACE('',(#896),#498,.F.);
#10133=ADVANCED_FACE('',(#897),#9685,.F.);
#10134=ADVANCED_FACE('',(#898),#499,.T.);
#10135=ADVANCED_FACE('',(#899),#9686,.F.);
#10136=ADVANCED_FACE('',(#900),#589,.F.);
#10137=ADVANCED_FACE('',(#901),#590,.F.);
#10138=ADVANCED_FACE('',(#902),#9687,.F.);
#10139=ADVANCED_FACE('',(#903),#500,.T.);
#10140=ADVANCED_FACE('',(#904),#9688,.F.);
#10141=ADVANCED_FACE('',(#905),#591,.F.);
#10142=ADVANCED_FACE('',(#906),#592,.F.);
#10143=ADVANCED_FACE('',(#907),#9689,.F.);
#10144=ADVANCED_FACE('',(#908),#501,.T.);
#10145=ADVANCED_FACE('',(#909),#9690,.F.);
#10146=ADVANCED_FACE('',(#910),#593,.F.);
#10147=ADVANCED_FACE('',(#911),#594,.F.);
#10148=ADVANCED_FACE('',(#912),#9691,.F.);
#10149=ADVANCED_FACE('',(#913),#502,.T.);
#10150=ADVANCED_FACE('',(#914),#9692,.F.);
#10151=ADVANCED_FACE('',(#915),#595,.F.);
#10152=ADVANCED_FACE('',(#916),#596,.F.);
#10153=ADVANCED_FACE('',(#917),#9693,.F.);
#10154=ADVANCED_FACE('',(#918),#503,.F.);
#10155=ADVANCED_FACE('',(#919),#504,.F.);
#10156=ADVANCED_FACE('',(#920),#505,.F.);
#10157=ADVANCED_FACE('',(#921),#506,.F.);
#10158=ADVANCED_FACE('',(#922),#9694,.F.);
#10159=ADVANCED_FACE('',(#923),#9695,.F.);
#10160=ADVANCED_FACE('',(#924),#9696,.F.);
#10161=ADVANCED_FACE('',(#925),#9697,.F.);
#10162=ADVANCED_FACE('',(#926),#9698,.F.);
#10163=ADVANCED_FACE('',(#927),#9699,.F.);
#10164=ADVANCED_FACE('',(#928),#9700,.F.);
#10165=ADVANCED_FACE('',(#929),#9701,.F.);
#10166=ADVANCED_FACE('',(#930),#9702,.F.);
#10167=ADVANCED_FACE('',(#931),#9703,.F.);
#10168=ADVANCED_FACE('',(#932),#9704,.F.);
#10169=ADVANCED_FACE('',(#933),#9705,.F.);
#10170=ADVANCED_FACE('',(#934),#9706,.F.);
#10171=ADVANCED_FACE('',(#935),#9707,.F.);
#10172=ADVANCED_FACE('',(#936),#9708,.F.);
#10173=ADVANCED_FACE('',(#937),#9709,.F.);
#10174=ADVANCED_FACE('',(#938),#9710,.F.);
#10175=ADVANCED_FACE('',(#939),#9711,.F.);
#10176=ADVANCED_FACE('',(#940),#507,.F.);
#10177=ADVANCED_FACE('',(#941,#359,#360,#361,#362,#363,#364,#365,#366,#367,
#368,#369,#370,#371,#372,#373,#374,#375,#376),#508,.F.);
#10178=ADVANCED_FACE('',(#942),#509,.F.);
#10179=ADVANCED_FACE('',(#943),#510,.F.);
#10180=ADVANCED_FACE('',(#944,#377),#511,.F.);
#10181=ADVANCED_FACE('',(#945),#512,.T.);
#10182=ADVANCED_FACE('',(#946,#378,#379,#380,#381,#382,#383,#384,#385,#386,
#387,#388,#389,#390,#391,#392,#393,#394,#395),#513,.T.);
#10183=ADVANCED_FACE('',(#947),#514,.T.);
#10184=ADVANCED_FACE('',(#948),#515,.T.);
#10185=ADVANCED_FACE('',(#949,#396,#397,#398,#399,#400),#516,.T.);
#10383=CLOSED_SHELL('',(#9839,#9840,#9841,#9842,#9843,#9844,#9845,#9846,
#9847,#9848,#9849,#9850,#9851,#9852,#9853,#9854,#9855,#9856,#9857,#9858,
#9859,#9860,#9861,#9862,#9863,#9864,#9865,#9866,#9867,#9868,#9869,#9870,
#9871,#9872,#9873,#9874,#9875,#9876,#9877,#9878,#9879,#9880,#9881,#9882,
#9883,#9884,#9885,#9886,#9887,#9888,#9889,#9890,#9891,#9892,#9893,#9894,
#9895,#9896,#9897,#9898,#9899,#9900,#9901,#9902,#9903,#9904,#9905,#9906,
#9907,#9908,#9909,#9910,#9911,#9912,#9913,#9914,#9915,#9916,#9917,#9918,
#9919,#9920,#9921,#9922,#9923,#9924,#9925,#9926,#9927,#9928,#9929,#9930,
#9931,#9932,#9933,#9934,#9935,#9936,#9937,#9938,#9939,#9940,#9941,#9942,
#9943,#9944,#9945,#9946,#9947,#9948,#9949,#9950,#9951,#9952,#9953,#9954,
#9955,#9956,#9957,#9958,#9959,#9960,#9961,#9962,#9963,#9964,#9965,#9966,
#9967,#9968,#9969,#9970,#9971,#9972,#9973,#9974,#9975,#9976,#9977,#9978,
#9979,#9980,#9981,#9982,#9983,#9984,#9985,#9986,#9987,#9988,#9989,#9990,
#9991,#9992,#9993,#9994,#9995,#9996,#9997,#9998,#9999,#10000,#10001,#10002,
#10003,#10004,#10005,#10006,#10007,#10008,#10009,#10010,#10011,#10012,#10013,
#10014,#10015,#10016,#10017,#10018,#10019,#10020,#10021,#10022,#10023,#10024,
#10025,#10026,#10027,#10028,#10029,#10030,#10031,#10032,#10033,#10034,#10035,
#10036,#10037,#10038,#10039,#10040,#10041,#10042,#10043,#10044,#10045,#10046,
#10047,#10048,#10049,#10050,#10051,#10052,#10053,#10054,#10055,#10056,#10057,
#10058,#10059,#10060,#10061,#10062,#10063,#10064,#10065,#10066,#10067,#10068,
#10069,#10070,#10071,#10072,#10073,#10074,#10075,#10076,#10077,#10078,#10079,
#10080,#10081,#10082,#10083,#10084,#10085,#10086,#10087,#10088,#10089,#10090,
#10091,#10092,#10093,#10094,#10095,#10096,#10097,#10098,#10099,#10100,#10101,
#10102,#10103,#10104,#10105,#10106,#10107,#10108,#10109,#10110,#10111,#10112,
#10113,#10114,#10115,#10116,#10117,#10118,#10119,#10120,#10121,#10122,#10123,
#10124,#10125,#10126,#10127,#10128,#10129,#10130,#10131,#10132,#10133,#10134,
#10135,#10136,#10137,#10138,#10139,#10140,#10141,#10142,#10143,#10144,#10145,
#10146,#10147,#10148,#10149,#10150,#10151,#10152,#10153,#10154,#10155,#10156,
#10157,#10158,#10159,#10160,#10161,#10162,#10163,#10164,#10165,#10166,#10167,
#10168,#10169,#10170,#10171,#10172,#10173,#10174,#10175,#10176,#10177,#10178,
#10179,#10180,#10181,#10182,#10183,#10184,#10185));
#10505=AXIS2_PLACEMENT_3D('',#13449,#11308,#11309);
#10506=AXIS2_PLACEMENT_3D('',#13450,#11310,#11311);
#10507=AXIS2_PLACEMENT_3D('',#13475,#11313,#11314);
#10508=AXIS2_PLACEMENT_3D('',#13483,#11316,#11317);
#10509=AXIS2_PLACEMENT_3D('',#13506,#11318,#11319);
#10510=AXIS2_PLACEMENT_3D('',#13557,#11321,#11322);
#10511=AXIS2_PLACEMENT_3D('',#13605,#11324,#11325);
#10512=AXIS2_PLACEMENT_3D('',#13656,#11327,#11328);
#10513=AXIS2_PLACEMENT_3D('',#13707,#11330,#11331);
#10514=AXIS2_PLACEMENT_3D('',#13755,#11333,#11334);
#10515=AXIS2_PLACEMENT_3D('',#13803,#11336,#11337);
#10516=AXIS2_PLACEMENT_3D('',#13854,#11339,#11340);
#10517=AXIS2_PLACEMENT_3D('',#13902,#11342,#11343);
#10518=AXIS2_PLACEMENT_3D('',#13950,#11345,#11346);
#10519=AXIS2_PLACEMENT_3D('',#14001,#11348,#11349);
#10520=AXIS2_PLACEMENT_3D('',#14052,#11351,#11352);
#10521=AXIS2_PLACEMENT_3D('',#14100,#11354,#11355);
#10522=AXIS2_PLACEMENT_3D('',#14151,#11357,#11358);
#10523=AXIS2_PLACEMENT_3D('',#14170,#11360,#11361);
#10524=AXIS2_PLACEMENT_3D('',#14190,#11362,#11363);
#10525=AXIS2_PLACEMENT_3D('',#14202,#11365,#11366);
#10526=AXIS2_PLACEMENT_3D('',#14210,#11367,#11368);
#10527=AXIS2_PLACEMENT_3D('',#14234,#11370,#11371);
#10528=AXIS2_PLACEMENT_3D('',#14259,#11373,#11374);
#10529=AXIS2_PLACEMENT_3D('',#14284,#11376,#11377);
#10530=AXIS2_PLACEMENT_3D('',#14308,#11379,#11380);
#10531=AXIS2_PLACEMENT_3D('',#14333,#11382,#11383);
#10532=AXIS2_PLACEMENT_3D('',#14357,#11385,#11386);
#10533=AXIS2_PLACEMENT_3D('',#14382,#11388,#11389);
#10534=AXIS2_PLACEMENT_3D('',#14407,#11391,#11392);
#10535=AXIS2_PLACEMENT_3D('',#14431,#11394,#11395);
#10536=AXIS2_PLACEMENT_3D('',#14456,#11397,#11398);
#10537=AXIS2_PLACEMENT_3D('',#14480,#11400,#11401);
#10538=AXIS2_PLACEMENT_3D('',#14505,#11403,#11404);
#10539=AXIS2_PLACEMENT_3D('',#14530,#11406,#11407);
#10540=AXIS2_PLACEMENT_3D('',#14554,#11409,#11410);
#10541=AXIS2_PLACEMENT_3D('',#14565,#11412,#11413);
#10542=AXIS2_PLACEMENT_3D('',#14571,#11414,#11415);
#10543=AXIS2_PLACEMENT_3D('',#14596,#11417,#11418);
#10544=AXIS2_PLACEMENT_3D('',#14604,#11420,#11421);
#10545=AXIS2_PLACEMENT_3D('',#14627,#11422,#11423);
#10546=AXIS2_PLACEMENT_3D('',#14678,#11425,#11426);
#10547=AXIS2_PLACEMENT_3D('',#14726,#11428,#11429);
#10548=AXIS2_PLACEMENT_3D('',#14777,#11431,#11432);
#10549=AXIS2_PLACEMENT_3D('',#14828,#11434,#11435);
#10550=AXIS2_PLACEMENT_3D('',#14876,#11437,#11438);
#10551=AXIS2_PLACEMENT_3D('',#14924,#11440,#11441);
#10552=AXIS2_PLACEMENT_3D('',#14975,#11443,#11444);
#10553=AXIS2_PLACEMENT_3D('',#15023,#11446,#11447);
#10554=AXIS2_PLACEMENT_3D('',#15071,#11449,#11450);
#10555=AXIS2_PLACEMENT_3D('',#15122,#11452,#11453);
#10556=AXIS2_PLACEMENT_3D('',#15173,#11455,#11456);
#10557=AXIS2_PLACEMENT_3D('',#15221,#11458,#11459);
#10558=AXIS2_PLACEMENT_3D('',#15272,#11461,#11462);
#10559=AXIS2_PLACEMENT_3D('',#15291,#11464,#11465);
#10560=AXIS2_PLACEMENT_3D('',#15311,#11466,#11467);
#10561=AXIS2_PLACEMENT_3D('',#15323,#11469,#11470);
#10562=AXIS2_PLACEMENT_3D('',#15331,#11471,#11472);
#10563=AXIS2_PLACEMENT_3D('',#15355,#11474,#11475);
#10564=AXIS2_PLACEMENT_3D('',#15380,#11477,#11478);
#10565=AXIS2_PLACEMENT_3D('',#15405,#11480,#11481);
#10566=AXIS2_PLACEMENT_3D('',#15429,#11483,#11484);
#10567=AXIS2_PLACEMENT_3D('',#15454,#11486,#11487);
#10568=AXIS2_PLACEMENT_3D('',#15478,#11489,#11490);
#10569=AXIS2_PLACEMENT_3D('',#15503,#11492,#11493);
#10570=AXIS2_PLACEMENT_3D('',#15528,#11495,#11496);
#10571=AXIS2_PLACEMENT_3D('',#15552,#11498,#11499);
#10572=AXIS2_PLACEMENT_3D('',#15577,#11501,#11502);
#10573=AXIS2_PLACEMENT_3D('',#15601,#11504,#11505);
#10574=AXIS2_PLACEMENT_3D('',#15626,#11507,#11508);
#10575=AXIS2_PLACEMENT_3D('',#15651,#11510,#11511);
#10576=AXIS2_PLACEMENT_3D('',#15675,#11513,#11514);
#10577=AXIS2_PLACEMENT_3D('',#15686,#11516,#11517);
#10578=AXIS2_PLACEMENT_3D('',#15692,#11518,#11519);
#10579=AXIS2_PLACEMENT_3D('',#15717,#11521,#11522);
#10580=AXIS2_PLACEMENT_3D('',#15725,#11524,#11525);
#10581=AXIS2_PLACEMENT_3D('',#15748,#11526,#11527);
#10582=AXIS2_PLACEMENT_3D('',#15799,#11529,#11530);
#10583=AXIS2_PLACEMENT_3D('',#15847,#11532,#11533);
#10584=AXIS2_PLACEMENT_3D('',#15898,#11535,#11536);
#10585=AXIS2_PLACEMENT_3D('',#15949,#11538,#11539);
#10586=AXIS2_PLACEMENT_3D('',#15997,#11541,#11542);
#10587=AXIS2_PLACEMENT_3D('',#16045,#11544,#11545);
#10588=AXIS2_PLACEMENT_3D('',#16096,#11547,#11548);
#10589=AXIS2_PLACEMENT_3D('',#16144,#11550,#11551);
#10590=AXIS2_PLACEMENT_3D('',#16192,#11553,#11554);
#10591=AXIS2_PLACEMENT_3D('',#16243,#11556,#11557);
#10592=AXIS2_PLACEMENT_3D('',#16294,#11559,#11560);
#10593=AXIS2_PLACEMENT_3D('',#16342,#11562,#11563);
#10594=AXIS2_PLACEMENT_3D('',#16393,#11565,#11566);
#10595=AXIS2_PLACEMENT_3D('',#16412,#11568,#11569);
#10596=AXIS2_PLACEMENT_3D('',#16432,#11570,#11571);
#10597=AXIS2_PLACEMENT_3D('',#16444,#11573,#11574);
#10598=AXIS2_PLACEMENT_3D('',#16452,#11575,#11576);
#10599=AXIS2_PLACEMENT_3D('',#16476,#11578,#11579);
#10600=AXIS2_PLACEMENT_3D('',#16501,#11581,#11582);
#10601=AXIS2_PLACEMENT_3D('',#16526,#11584,#11585);
#10602=AXIS2_PLACEMENT_3D('',#16550,#11587,#11588);
#10603=AXIS2_PLACEMENT_3D('',#16575,#11590,#11591);
#10604=AXIS2_PLACEMENT_3D('',#16599,#11593,#11594);
#10605=AXIS2_PLACEMENT_3D('',#16624,#11596,#11597);
#10606=AXIS2_PLACEMENT_3D('',#16649,#11599,#11600);
#10607=AXIS2_PLACEMENT_3D('',#16673,#11602,#11603);
#10608=AXIS2_PLACEMENT_3D('',#16698,#11605,#11606);
#10609=AXIS2_PLACEMENT_3D('',#16722,#11608,#11609);
#10610=AXIS2_PLACEMENT_3D('',#16747,#11611,#11612);
#10611=AXIS2_PLACEMENT_3D('',#16772,#11614,#11615);
#10612=AXIS2_PLACEMENT_3D('',#16796,#11617,#11618);
#10613=AXIS2_PLACEMENT_3D('',#16807,#11620,#11621);
#10614=AXIS2_PLACEMENT_3D('',#16813,#11622,#11623);
#10615=AXIS2_PLACEMENT_3D('',#16838,#11625,#11626);
#10616=AXIS2_PLACEMENT_3D('',#16846,#11628,#11629);
#10617=AXIS2_PLACEMENT_3D('',#16869,#11630,#11631);
#10618=AXIS2_PLACEMENT_3D('',#16920,#11633,#11634);
#10619=AXIS2_PLACEMENT_3D('',#16968,#11636,#11637);
#10620=AXIS2_PLACEMENT_3D('',#17019,#11639,#11640);
#10621=AXIS2_PLACEMENT_3D('',#17070,#11642,#11643);
#10622=AXIS2_PLACEMENT_3D('',#17118,#11645,#11646);
#10623=AXIS2_PLACEMENT_3D('',#17166,#11648,#11649);
#10624=AXIS2_PLACEMENT_3D('',#17217,#11651,#11652);
#10625=AXIS2_PLACEMENT_3D('',#17265,#11654,#11655);
#10626=AXIS2_PLACEMENT_3D('',#17313,#11657,#11658);
#10627=AXIS2_PLACEMENT_3D('',#17364,#11660,#11661);
#10628=AXIS2_PLACEMENT_3D('',#17415,#11663,#11664);
#10629=AXIS2_PLACEMENT_3D('',#17463,#11666,#11667);
#10630=AXIS2_PLACEMENT_3D('',#17514,#11669,#11670);
#10631=AXIS2_PLACEMENT_3D('',#17533,#11672,#11673);
#10632=AXIS2_PLACEMENT_3D('',#17553,#11674,#11675);
#10633=AXIS2_PLACEMENT_3D('',#17565,#11677,#11678);
#10634=AXIS2_PLACEMENT_3D('',#17573,#11679,#11680);
#10635=AXIS2_PLACEMENT_3D('',#17597,#11682,#11683);
#10636=AXIS2_PLACEMENT_3D('',#17622,#11685,#11686);
#10637=AXIS2_PLACEMENT_3D('',#17647,#11688,#11689);
#10638=AXIS2_PLACEMENT_3D('',#17671,#11691,#11692);
#10639=AXIS2_PLACEMENT_3D('',#17696,#11694,#11695);
#10640=AXIS2_PLACEMENT_3D('',#17720,#11697,#11698);
#10641=AXIS2_PLACEMENT_3D('',#17745,#11700,#11701);
#10642=AXIS2_PLACEMENT_3D('',#17770,#11703,#11704);
#10643=AXIS2_PLACEMENT_3D('',#17794,#11706,#11707);
#10644=AXIS2_PLACEMENT_3D('',#17819,#11709,#11710);
#10645=AXIS2_PLACEMENT_3D('',#17843,#11712,#11713);
#10646=AXIS2_PLACEMENT_3D('',#17868,#11715,#11716);
#10647=AXIS2_PLACEMENT_3D('',#17893,#11718,#11719);
#10648=AXIS2_PLACEMENT_3D('',#17917,#11721,#11722);
#10649=AXIS2_PLACEMENT_3D('',#17928,#11724,#11725);
#10650=AXIS2_PLACEMENT_3D('',#17934,#11726,#11727);
#10651=AXIS2_PLACEMENT_3D('',#17944,#11729,#11730);
#10652=AXIS2_PLACEMENT_3D('',#17966,#11731,#11732);
#10653=AXIS2_PLACEMENT_3D('',#17977,#11733,#11734);
#10654=AXIS2_PLACEMENT_3D('',#18028,#11736,#11737);
#10655=AXIS2_PLACEMENT_3D('',#18079,#11739,#11740);
#10656=AXIS2_PLACEMENT_3D('',#18127,#11742,#11743);
#10657=AXIS2_PLACEMENT_3D('',#18178,#11745,#11746);
#10658=AXIS2_PLACEMENT_3D('',#18229,#11748,#11749);
#10659=AXIS2_PLACEMENT_3D('',#18277,#11751,#11752);
#10660=AXIS2_PLACEMENT_3D('',#18328,#11754,#11755);
#10661=AXIS2_PLACEMENT_3D('',#18379,#11757,#11758);
#10662=AXIS2_PLACEMENT_3D('',#18427,#11760,#11761);
#10663=AXIS2_PLACEMENT_3D('',#18478,#11763,#11764);
#10664=AXIS2_PLACEMENT_3D('',#18529,#11766,#11767);
#10665=AXIS2_PLACEMENT_3D('',#18577,#11769,#11770);
#10666=AXIS2_PLACEMENT_3D('',#18628,#11772,#11773);
#10667=AXIS2_PLACEMENT_3D('',#18647,#11775,#11776);
#10668=AXIS2_PLACEMENT_3D('',#18667,#11777,#11778);
#10669=AXIS2_PLACEMENT_3D('',#18677,#11780,#11781);
#10670=AXIS2_PLACEMENT_3D('',#18699,#11782,#11783);
#10671=AXIS2_PLACEMENT_3D('',#18710,#11784,#11785);
#10672=AXIS2_PLACEMENT_3D('',#18761,#11787,#11788);
#10673=AXIS2_PLACEMENT_3D('',#18812,#11790,#11791);
#10674=AXIS2_PLACEMENT_3D('',#18860,#11793,#11794);
#10675=AXIS2_PLACEMENT_3D('',#18911,#11796,#11797);
#10676=AXIS2_PLACEMENT_3D('',#18962,#11799,#11800);
#10677=AXIS2_PLACEMENT_3D('',#19010,#11802,#11803);
#10678=AXIS2_PLACEMENT_3D('',#19061,#11805,#11806);
#10679=AXIS2_PLACEMENT_3D('',#19112,#11808,#11809);
#10680=AXIS2_PLACEMENT_3D('',#19160,#11811,#11812);
#10681=AXIS2_PLACEMENT_3D('',#19211,#11814,#11815);
#10682=AXIS2_PLACEMENT_3D('',#19262,#11817,#11818);
#10683=AXIS2_PLACEMENT_3D('',#19310,#11820,#11821);
#10684=AXIS2_PLACEMENT_3D('',#19361,#11823,#11824);
#10685=AXIS2_PLACEMENT_3D('',#19380,#11826,#11827);
#10686=AXIS2_PLACEMENT_3D('',#19400,#11828,#11829);
#10687=AXIS2_PLACEMENT_3D('',#19414,#11831,#11832);
#10688=AXIS2_PLACEMENT_3D('',#19424,#11833,#11834);
#10689=AXIS2_PLACEMENT_3D('',#19448,#11836,#11837);
#10690=AXIS2_PLACEMENT_3D('',#19473,#11839,#11840);
#10691=AXIS2_PLACEMENT_3D('',#19498,#11842,#11843);
#10692=AXIS2_PLACEMENT_3D('',#19522,#11845,#11846);
#10693=AXIS2_PLACEMENT_3D('',#19547,#11848,#11849);
#10694=AXIS2_PLACEMENT_3D('',#19572,#11851,#11852);
#10695=AXIS2_PLACEMENT_3D('',#19596,#11854,#11855);
#10696=AXIS2_PLACEMENT_3D('',#19621,#11857,#11858);
#10697=AXIS2_PLACEMENT_3D('',#19646,#11860,#11861);
#10698=AXIS2_PLACEMENT_3D('',#19670,#11863,#11864);
#10699=AXIS2_PLACEMENT_3D('',#19695,#11866,#11867);
#10700=AXIS2_PLACEMENT_3D('',#19720,#11869,#11870);
#10701=AXIS2_PLACEMENT_3D('',#19744,#11872,#11873);
#10702=AXIS2_PLACEMENT_3D('',#19755,#11875,#11876);
#10703=AXIS2_PLACEMENT_3D('',#19761,#11877,#11878);
#10704=AXIS2_PLACEMENT_3D('',#19775,#11880,#11881);
#10705=AXIS2_PLACEMENT_3D('',#19785,#11882,#11883);
#10706=AXIS2_PLACEMENT_3D('',#19809,#11885,#11886);
#10707=AXIS2_PLACEMENT_3D('',#19834,#11888,#11889);
#10708=AXIS2_PLACEMENT_3D('',#19859,#11891,#11892);
#10709=AXIS2_PLACEMENT_3D('',#19883,#11894,#11895);
#10710=AXIS2_PLACEMENT_3D('',#19908,#11897,#11898);
#10711=AXIS2_PLACEMENT_3D('',#19933,#11900,#11901);
#10712=AXIS2_PLACEMENT_3D('',#19957,#11903,#11904);
#10713=AXIS2_PLACEMENT_3D('',#19982,#11906,#11907);
#10714=AXIS2_PLACEMENT_3D('',#20007,#11909,#11910);
#10715=AXIS2_PLACEMENT_3D('',#20031,#11912,#11913);
#10716=AXIS2_PLACEMENT_3D('',#20056,#11915,#11916);
#10717=AXIS2_PLACEMENT_3D('',#20081,#11918,#11919);
#10718=AXIS2_PLACEMENT_3D('',#20105,#11921,#11922);
#10719=AXIS2_PLACEMENT_3D('',#20116,#11924,#11925);
#10720=AXIS2_PLACEMENT_3D('',#20122,#11926,#11927);
#10721=AXIS2_PLACEMENT_3D('',#20132,#11929,#11930);
#10722=AXIS2_PLACEMENT_3D('',#20135,#11932,#11933);
#10723=AXIS2_PLACEMENT_3D('',#20137,#11934,#11935);
#10724=AXIS2_PLACEMENT_3D('',#20148,#11936,#11937);
#10725=AXIS2_PLACEMENT_3D('',#20199,#11939,#11940);
#10726=AXIS2_PLACEMENT_3D('',#20250,#11942,#11943);
#10727=AXIS2_PLACEMENT_3D('',#20298,#11945,#11946);
#10728=AXIS2_PLACEMENT_3D('',#20349,#11948,#11949);
#10729=AXIS2_PLACEMENT_3D('',#20400,#11951,#11952);
#10730=AXIS2_PLACEMENT_3D('',#20448,#11954,#11955);
#10731=AXIS2_PLACEMENT_3D('',#20499,#11957,#11958);
#10732=AXIS2_PLACEMENT_3D('',#20550,#11960,#11961);
#10733=AXIS2_PLACEMENT_3D('',#20598,#11963,#11964);
#10734=AXIS2_PLACEMENT_3D('',#20649,#11966,#11967);
#10735=AXIS2_PLACEMENT_3D('',#20700,#11969,#11970);
#10736=AXIS2_PLACEMENT_3D('',#20748,#11972,#11973);
#10737=AXIS2_PLACEMENT_3D('',#20799,#11975,#11976);
#10738=AXIS2_PLACEMENT_3D('',#20818,#11978,#11979);
#10739=AXIS2_PLACEMENT_3D('',#20838,#11980,#11981);
#10740=AXIS2_PLACEMENT_3D('',#20852,#11983,#11984);
#10741=AXIS2_PLACEMENT_3D('',#20862,#11985,#11986);
#10742=AXIS2_PLACEMENT_3D('',#20886,#11988,#11989);
#10743=AXIS2_PLACEMENT_3D('',#20911,#11991,#11992);
#10744=AXIS2_PLACEMENT_3D('',#20936,#11994,#11995);
#10745=AXIS2_PLACEMENT_3D('',#20960,#11997,#11998);
#10746=AXIS2_PLACEMENT_3D('',#20985,#12000,#12001);
#10747=AXIS2_PLACEMENT_3D('',#21010,#12003,#12004);
#10748=AXIS2_PLACEMENT_3D('',#21034,#12006,#12007);
#10749=AXIS2_PLACEMENT_3D('',#21059,#12009,#12010);
#10750=AXIS2_PLACEMENT_3D('',#21084,#12012,#12013);
#10751=AXIS2_PLACEMENT_3D('',#21108,#12015,#12016);
#10752=AXIS2_PLACEMENT_3D('',#21133,#12018,#12019);
#10753=AXIS2_PLACEMENT_3D('',#21158,#12021,#12022);
#10754=AXIS2_PLACEMENT_3D('',#21182,#12024,#12025);
#10755=AXIS2_PLACEMENT_3D('',#21193,#12027,#12028);
#10756=AXIS2_PLACEMENT_3D('',#21199,#12029,#12030);
#10757=AXIS2_PLACEMENT_3D('',#21209,#12032,#12033);
#10758=AXIS2_PLACEMENT_3D('',#21212,#12035,#12036);
#10759=AXIS2_PLACEMENT_3D('',#21214,#12037,#12038);
#10760=AXIS2_PLACEMENT_3D('',#21225,#12039,#12040);
#10761=AXIS2_PLACEMENT_3D('',#21276,#12042,#12043);
#10762=AXIS2_PLACEMENT_3D('',#21327,#12045,#12046);
#10763=AXIS2_PLACEMENT_3D('',#21375,#12048,#12049);
#10764=AXIS2_PLACEMENT_3D('',#21426,#12051,#12052);
#10765=AXIS2_PLACEMENT_3D('',#21477,#12054,#12055);
#10766=AXIS2_PLACEMENT_3D('',#21525,#12057,#12058);
#10767=AXIS2_PLACEMENT_3D('',#21576,#12060,#12061);
#10768=AXIS2_PLACEMENT_3D('',#21627,#12063,#12064);
#10769=AXIS2_PLACEMENT_3D('',#21675,#12066,#12067);
#10770=AXIS2_PLACEMENT_3D('',#21726,#12069,#12070);
#10771=AXIS2_PLACEMENT_3D('',#21777,#12072,#12073);
#10772=AXIS2_PLACEMENT_3D('',#21825,#12075,#12076);
#10773=AXIS2_PLACEMENT_3D('',#21876,#12078,#12079);
#10774=AXIS2_PLACEMENT_3D('',#21895,#12081,#12082);
#10775=AXIS2_PLACEMENT_3D('',#21915,#12083,#12084);
#10776=AXIS2_PLACEMENT_3D('',#21929,#12086,#12087);
#10777=AXIS2_PLACEMENT_3D('',#21939,#12088,#12089);
#10778=AXIS2_PLACEMENT_3D('',#21963,#12091,#12092);
#10779=AXIS2_PLACEMENT_3D('',#21988,#12094,#12095);
#10780=AXIS2_PLACEMENT_3D('',#22013,#12097,#12098);
#10781=AXIS2_PLACEMENT_3D('',#22037,#12100,#12101);
#10782=AXIS2_PLACEMENT_3D('',#22062,#12103,#12104);
#10783=AXIS2_PLACEMENT_3D('',#22087,#12106,#12107);
#10784=AXIS2_PLACEMENT_3D('',#22111,#12109,#12110);
#10785=AXIS2_PLACEMENT_3D('',#22136,#12112,#12113);
#10786=AXIS2_PLACEMENT_3D('',#22161,#12115,#12116);
#10787=AXIS2_PLACEMENT_3D('',#22185,#12118,#12119);
#10788=AXIS2_PLACEMENT_3D('',#22210,#12121,#12122);
#10789=AXIS2_PLACEMENT_3D('',#22235,#12124,#12125);
#10790=AXIS2_PLACEMENT_3D('',#22259,#12127,#12128);
#10791=AXIS2_PLACEMENT_3D('',#22270,#12130,#12131);
#10792=AXIS2_PLACEMENT_3D('',#22276,#12132,#12133);
#10793=AXIS2_PLACEMENT_3D('',#22307,#12135,#12136);
#10794=AXIS2_PLACEMENT_3D('',#22345,#12137,#12138);
#10795=AXIS2_PLACEMENT_3D('',#22435,#12140,#12141);
#10796=AXIS2_PLACEMENT_3D('',#22522,#12143,#12144);
#10797=AXIS2_PLACEMENT_3D('',#22612,#12146,#12147);
#10798=AXIS2_PLACEMENT_3D('',#22699,#12149,#12150);
#10799=AXIS2_PLACEMENT_3D('',#22789,#12152,#12153);
#10800=AXIS2_PLACEMENT_3D('',#22876,#12155,#12156);
#10801=AXIS2_PLACEMENT_3D('',#22889,#12158,#12159);
#10802=AXIS2_PLACEMENT_3D('',#22909,#12160,#12161);
#10803=AXIS2_PLACEMENT_3D('',#22928,#12163,#12164);
#10804=AXIS2_PLACEMENT_3D('',#22943,#12165,#12166);
#10805=AXIS2_PLACEMENT_3D('',#22979,#12168,#12169);
#10806=AXIS2_PLACEMENT_3D('',#23017,#12171,#12172);
#10807=AXIS2_PLACEMENT_3D('',#23055,#12174,#12175);
#10808=AXIS2_PLACEMENT_3D('',#23092,#12177,#12178);
#10809=AXIS2_PLACEMENT_3D('',#23129,#12180,#12181);
#10810=AXIS2_PLACEMENT_3D('',#23167,#12183,#12184);
#10811=AXIS2_PLACEMENT_3D('',#23179,#12186,#12187);
#10812=AXIS2_PLACEMENT_3D('',#23187,#12188,#12189);
#10813=AXIS2_PLACEMENT_3D('',#24643,#12190,#12191);
#10814=AXIS2_PLACEMENT_3D('',#24645,#12192,#12193);
#10815=AXIS2_PLACEMENT_3D('',#24646,#12194,#12195);
#10816=AXIS2_PLACEMENT_3D('',#24647,#12196,#12197);
#10817=AXIS2_PLACEMENT_3D('',#24649,#12198,#12199);
#10818=AXIS2_PLACEMENT_3D('',#24651,#12201,#12202);
#10819=AXIS2_PLACEMENT_3D('',#25400,#12207,#12208);
#10820=AXIS2_PLACEMENT_3D('',#25589,#12209,#12210);
#10821=AXIS2_PLACEMENT_3D('',#26458,#12211,#12212);
#10822=AXIS2_PLACEMENT_3D('',#26459,#12213,#12214);
#10823=AXIS2_PLACEMENT_3D('',#26648,#12215,#12216);
#10824=AXIS2_PLACEMENT_3D('',#27517,#12217,#12218);
#10825=AXIS2_PLACEMENT_3D('',#27518,#12219,#12220);
#10826=AXIS2_PLACEMENT_3D('',#27552,#12222,#12223);
#10827=AXIS2_PLACEMENT_3D('',#27684,#12226,#12227);
#10828=AXIS2_PLACEMENT_3D('',#27685,#12228,#12229);
#10829=AXIS2_PLACEMENT_3D('',#27721,#12231,#12232);
#10830=AXIS2_PLACEMENT_3D('',#28590,#12233,#12234);
#10831=AXIS2_PLACEMENT_3D('',#28612,#12235,#12236);
#10832=AXIS2_PLACEMENT_3D('',#28646,#12238,#12239);
#10833=AXIS2_PLACEMENT_3D('',#28778,#12242,#12243);
#10834=AXIS2_PLACEMENT_3D('',#28779,#12244,#12245);
#10835=AXIS2_PLACEMENT_3D('',#28815,#12247,#12248);
#10836=AXIS2_PLACEMENT_3D('',#29684,#12249,#12250);
#10837=AXIS2_PLACEMENT_3D('',#29706,#12251,#12252);
#10838=AXIS2_PLACEMENT_3D('',#29707,#12253,#12254);
#10839=AXIS2_PLACEMENT_3D('',#29708,#12255,#12256);
#10840=AXIS2_PLACEMENT_3D('',#29709,#12257,#12258);
#10841=AXIS2_PLACEMENT_3D('',#29710,#12259,#12260);
#10842=AXIS2_PLACEMENT_3D('',#29884,#12261,#12262);
#10843=AXIS2_PLACEMENT_3D('',#30952,#12263,#12264);
#10844=AXIS2_PLACEMENT_3D('',#30953,#12265,#12266);
#10845=AXIS2_PLACEMENT_3D('',#31127,#12267,#12268);
#10846=AXIS2_PLACEMENT_3D('',#32195,#12269,#12270);
#10847=AXIS2_PLACEMENT_3D('',#32196,#12271,#12272);
#10848=AXIS2_PLACEMENT_3D('',#32370,#12273,#12274);
#10849=AXIS2_PLACEMENT_3D('',#33438,#12275,#12276);
#10850=AXIS2_PLACEMENT_3D('',#33439,#12277,#12278);
#10851=AXIS2_PLACEMENT_3D('',#33613,#12279,#12280);
#10852=AXIS2_PLACEMENT_3D('',#34681,#12281,#12282);
#10853=AXIS2_PLACEMENT_3D('',#34682,#12283,#12284);
#10854=AXIS2_PLACEMENT_3D('',#34683,#12285,#12286);
#10855=AXIS2_PLACEMENT_3D('',#34684,#12287,#12288);
#10856=AXIS2_PLACEMENT_3D('',#34685,#12289,#12290);
#10857=AXIS2_PLACEMENT_3D('',#34686,#12291,#12292);
#10858=AXIS2_PLACEMENT_3D('',#34688,#12293,#12294);
#10859=AXIS2_PLACEMENT_3D('',#34691,#12296,#12297);
#10860=AXIS2_PLACEMENT_3D('',#34692,#12298,#12299);
#10861=AXIS2_PLACEMENT_3D('',#34694,#12300,#12301);
#10862=AXIS2_PLACEMENT_3D('',#34697,#12303,#12304);
#10863=AXIS2_PLACEMENT_3D('',#34698,#12305,#12306);
#10864=AXIS2_PLACEMENT_3D('',#34700,#12307,#12308);
#10865=AXIS2_PLACEMENT_3D('',#34703,#12310,#12311);
#10866=AXIS2_PLACEMENT_3D('',#34704,#12312,#12313);
#10867=AXIS2_PLACEMENT_3D('',#34706,#12314,#12315);
#10868=AXIS2_PLACEMENT_3D('',#34709,#12317,#12318);
#10869=AXIS2_PLACEMENT_3D('',#34710,#12319,#12320);
#10870=AXIS2_PLACEMENT_3D('',#34712,#12321,#12322);
#10871=AXIS2_PLACEMENT_3D('',#34715,#12324,#12325);
#10872=AXIS2_PLACEMENT_3D('',#34716,#12326,#12327);
#10873=AXIS2_PLACEMENT_3D('',#34718,#12328,#12329);
#10874=AXIS2_PLACEMENT_3D('',#34721,#12331,#12332);
#10875=AXIS2_PLACEMENT_3D('',#34722,#12333,#12334);
#10876=AXIS2_PLACEMENT_3D('',#34724,#12335,#12336);
#10877=AXIS2_PLACEMENT_3D('',#34727,#12338,#12339);
#10878=AXIS2_PLACEMENT_3D('',#34728,#12340,#12341);
#10879=AXIS2_PLACEMENT_3D('',#34730,#12342,#12343);
#10880=AXIS2_PLACEMENT_3D('',#34733,#12345,#12346);
#10881=AXIS2_PLACEMENT_3D('',#34734,#12347,#12348);
#10882=AXIS2_PLACEMENT_3D('',#34736,#12349,#12350);
#10883=AXIS2_PLACEMENT_3D('',#34740,#12353,#12354);
#10884=AXIS2_PLACEMENT_3D('',#34741,#12355,#12356);
#10885=AXIS2_PLACEMENT_3D('',#34743,#12357,#12358);
#10886=AXIS2_PLACEMENT_3D('',#34746,#12360,#12361);
#10887=AXIS2_PLACEMENT_3D('',#34747,#12362,#12363);
#10888=AXIS2_PLACEMENT_3D('',#34749,#12364,#12365);
#10889=AXIS2_PLACEMENT_3D('',#34752,#12367,#12368);
#10890=AXIS2_PLACEMENT_3D('',#34753,#12369,#12370);
#10891=AXIS2_PLACEMENT_3D('',#34755,#12371,#12372);
#10892=AXIS2_PLACEMENT_3D('',#34758,#12374,#12375);
#10893=AXIS2_PLACEMENT_3D('',#34759,#12376,#12377);
#10894=AXIS2_PLACEMENT_3D('',#34761,#12378,#12379);
#10895=AXIS2_PLACEMENT_3D('',#34764,#12381,#12382);
#10896=AXIS2_PLACEMENT_3D('',#34765,#12383,#12384);
#10897=AXIS2_PLACEMENT_3D('',#34767,#12385,#12386);
#10898=AXIS2_PLACEMENT_3D('',#34770,#12388,#12389);
#10899=AXIS2_PLACEMENT_3D('',#34771,#12390,#12391);
#10900=AXIS2_PLACEMENT_3D('',#34773,#12392,#12393);
#10901=AXIS2_PLACEMENT_3D('',#34776,#12395,#12396);
#10902=AXIS2_PLACEMENT_3D('',#34777,#12397,#12398);
#10903=AXIS2_PLACEMENT_3D('',#34779,#12399,#12400);
#10904=AXIS2_PLACEMENT_3D('',#34782,#12402,#12403);
#10905=AXIS2_PLACEMENT_3D('',#34783,#12404,#12405);
#10906=AXIS2_PLACEMENT_3D('',#34785,#12406,#12407);
#10907=AXIS2_PLACEMENT_3D('',#34789,#12410,#12411);
#10908=AXIS2_PLACEMENT_3D('',#34790,#12412,#12413);
#10909=AXIS2_PLACEMENT_3D('',#34792,#12414,#12415);
#10910=AXIS2_PLACEMENT_3D('',#34795,#12417,#12418);
#10911=AXIS2_PLACEMENT_3D('',#34796,#12419,#12420);
#10912=AXIS2_PLACEMENT_3D('',#34805,#12425,#12426);
#10913=AXIS2_PLACEMENT_3D('',#34811,#12430,#12431);
#10914=AXIS2_PLACEMENT_3D('',#34817,#12435,#12436);
#10915=AXIS2_PLACEMENT_3D('',#34820,#12439,#12440);
#10916=AXIS2_PLACEMENT_3D('',#34821,#12441,#12442);
#10917=AXIS2_PLACEMENT_3D('',#34827,#12446,#12447);
#10918=AXIS2_PLACEMENT_3D('',#34831,#12450,#12451);
#10919=AXIS2_PLACEMENT_3D('',#34835,#12454,#12455);
#10920=AXIS2_PLACEMENT_3D('',#34837,#12457,#12458);
#11308=DIRECTION('axis',(0.,0.,1.));
#11309=DIRECTION('refdir',(1.,0.,0.));
#11310=DIRECTION('center_axis',(0.,0.,-1.));
#11311=DIRECTION('ref_axis',(1.,0.,0.));
#11312=DIRECTION('',(0.,0.,-1.));
#11313=DIRECTION('center_axis',(0.,0.,1.));
#11314=DIRECTION('ref_axis',(1.,0.,0.));
#11315=DIRECTION('',(0.,0.,-1.));
#11316=DIRECTION('center_axis',(0.,0.,1.));
#11317=DIRECTION('ref_axis',(1.,0.,0.));
#11318=DIRECTION('center_axis',(0.,0.,-1.));
#11319=DIRECTION('ref_axis',(1.,0.,0.));
#11320=DIRECTION('',(0.,0.,-1.));
#11321=DIRECTION('center_axis',(0.,0.,-1.));
#11322=DIRECTION('ref_axis',(1.,0.,0.));
#11323=DIRECTION('',(0.,0.,-1.));
#11324=DIRECTION('center_axis',(0.,0.,-1.));
#11325=DIRECTION('ref_axis',(1.,0.,0.));
#11326=DIRECTION('',(0.,0.,-1.));
#11327=DIRECTION('center_axis',(0.,0.,-1.));
#11328=DIRECTION('ref_axis',(1.,0.,0.));
#11329=DIRECTION('',(0.,0.,-1.));
#11330=DIRECTION('center_axis',(0.,0.,-1.));
#11331=DIRECTION('ref_axis',(1.,0.,0.));
#11332=DIRECTION('',(0.,0.,-1.));
#11333=DIRECTION('center_axis',(0.,0.,-1.));
#11334=DIRECTION('ref_axis',(1.,0.,0.));
#11335=DIRECTION('',(0.,0.,-1.));
#11336=DIRECTION('center_axis',(0.,0.,-1.));
#11337=DIRECTION('ref_axis',(1.,0.,0.));
#11338=DIRECTION('',(0.,0.,-1.));
#11339=DIRECTION('center_axis',(0.,0.,-1.));
#11340=DIRECTION('ref_axis',(1.,0.,0.));
#11341=DIRECTION('',(0.,0.,-1.));
#11342=DIRECTION('center_axis',(0.,0.,-1.));
#11343=DIRECTION('ref_axis',(1.,0.,0.));
#11344=DIRECTION('',(0.,0.,-1.));
#11345=DIRECTION('center_axis',(0.,0.,-1.));
#11346=DIRECTION('ref_axis',(1.,0.,0.));
#11347=DIRECTION('',(0.,0.,-1.));
#11348=DIRECTION('center_axis',(0.,0.,-1.));
#11349=DIRECTION('ref_axis',(1.,0.,0.));
#11350=DIRECTION('',(0.,0.,-1.));
#11351=DIRECTION('center_axis',(0.,0.,-1.));
#11352=DIRECTION('ref_axis',(1.,0.,0.));
#11353=DIRECTION('',(0.,0.,-1.));
#11354=DIRECTION('center_axis',(0.,0.,-1.));
#11355=DIRECTION('ref_axis',(1.,0.,0.));
#11356=DIRECTION('',(0.,0.,-1.));
#11357=DIRECTION('center_axis',(0.,0.,-1.));
#11358=DIRECTION('ref_axis',(0.938438521500727,-0.345446293023284,0.));
#11359=DIRECTION('',(0.,0.,-1.));
#11360=DIRECTION('center_axis',(0.,0.,-1.));
#11361=DIRECTION('ref_axis',(1.,0.,0.));
#11362=DIRECTION('center_axis',(0.,0.,-1.));
#11363=DIRECTION('ref_axis',(0.0179642919149216,0.999838629087712,0.));
#11364=DIRECTION('',(1.22464679914735E-16,-9.01413744397708E-30,-1.));
#11365=DIRECTION('center_axis',(0.,0.,1.));
#11366=DIRECTION('ref_axis',(1.,-7.34835534001804E-14,0.));
#11367=DIRECTION('center_axis',(0.,0.,-1.));
#11368=DIRECTION('ref_axis',(1.,-7.34835534001804E-14,0.));
#11369=DIRECTION('',(1.22464679914735E-16,-9.01413744397708E-30,-1.));
#11370=DIRECTION('center_axis',(0.,0.,-1.));
#11371=DIRECTION('ref_axis',(1.,-7.34835534001804E-14,0.));
#11372=DIRECTION('',(1.22464679914735E-16,-9.01413744397708E-30,-1.));
#11373=DIRECTION('center_axis',(0.,0.,-1.));
#11374=DIRECTION('ref_axis',(1.,-7.34835534001804E-14,0.));
#11375=DIRECTION('',(1.22464679914735E-16,-9.01413744397708E-30,-1.));
#11376=DIRECTION('center_axis',(0.,0.,-1.));
#11377=DIRECTION('ref_axis',(1.,-7.34835534001804E-14,0.));
#11378=DIRECTION('',(1.22464679914735E-16,-9.01413744397708E-30,-1.));
#11379=DIRECTION('center_axis',(0.,0.,-1.));
#11380=DIRECTION('ref_axis',(1.,-7.34835534001804E-14,0.));
#11381=DIRECTION('',(1.22464679914735E-16,-9.01413744397708E-30,-1.));
#11382=DIRECTION('center_axis',(0.,0.,-1.));
#11383=DIRECTION('ref_axis',(1.,-7.34835534001804E-14,0.));
#11384=DIRECTION('',(1.22464679914735E-16,-9.01413744397708E-30,-1.));
#11385=DIRECTION('center_axis',(0.,0.,-1.));
#11386=DIRECTION('ref_axis',(1.,-7.34835534001804E-14,0.));
#11387=DIRECTION('',(1.22464679914735E-16,-9.01413744397708E-30,-1.));
#11388=DIRECTION('center_axis',(0.,0.,-1.));
#11389=DIRECTION('ref_axis',(1.,-7.34835534001804E-14,0.));
#11390=DIRECTION('',(1.22464679914735E-16,-9.01413744397708E-30,-1.));
#11391=DIRECTION('center_axis',(0.,0.,-1.));
#11392=DIRECTION('ref_axis',(1.,-7.34835534001804E-14,0.));
#11393=DIRECTION('',(1.22464679914735E-16,-9.01413744397708E-30,-1.));
#11394=DIRECTION('center_axis',(0.,0.,-1.));
#11395=DIRECTION('ref_axis',(1.,-7.34835534001804E-14,0.));
#11396=DIRECTION('',(1.22464679914735E-16,-9.01413744397708E-30,-1.));
#11397=DIRECTION('center_axis',(0.,0.,-1.));
#11398=DIRECTION('ref_axis',(1.,-7.34835534001804E-14,0.));
#11399=DIRECTION('',(1.22464679914735E-16,-9.01413744397708E-30,-1.));
#11400=DIRECTION('center_axis',(0.,0.,-1.));
#11401=DIRECTION('ref_axis',(1.,-7.34835534001804E-14,0.));
#11402=DIRECTION('',(1.22464679914735E-16,-9.01413744397708E-30,-1.));
#11403=DIRECTION('center_axis',(0.,0.,-1.));
#11404=DIRECTION('ref_axis',(1.,-7.34835534001804E-14,0.));
#11405=DIRECTION('',(1.22464679914735E-16,-9.01413744397708E-30,-1.));
#11406=DIRECTION('center_axis',(0.,0.,-1.));
#11407=DIRECTION('ref_axis',(1.,-7.34835534001804E-14,0.));
#11408=DIRECTION('',(1.22464679914735E-16,-9.01413744397708E-30,-1.));
#11409=DIRECTION('center_axis',(0.,0.,-1.));
#11410=DIRECTION('ref_axis',(-0.609341740308203,-0.792907714376755,0.));
#11411=DIRECTION('',(1.22464679914735E-16,-9.01413744397708E-30,-1.));
#11412=DIRECTION('center_axis',(0.,0.,-1.));
#11413=DIRECTION('ref_axis',(1.,-7.34835534001804E-14,0.));
#11414=DIRECTION('center_axis',(0.,0.,-1.));
#11415=DIRECTION('ref_axis',(1.,0.,0.));
#11416=DIRECTION('',(0.,0.,-1.));
#11417=DIRECTION('center_axis',(0.,0.,1.));
#11418=DIRECTION('ref_axis',(1.,0.,0.));
#11419=DIRECTION('',(0.,0.,-1.));
#11420=DIRECTION('center_axis',(0.,0.,1.));
#11421=DIRECTION('ref_axis',(1.,0.,0.));
#11422=DIRECTION('center_axis',(0.,0.,-1.));
#11423=DIRECTION('ref_axis',(1.,0.,0.));
#11424=DIRECTION('',(0.,0.,-1.));
#11425=DIRECTION('center_axis',(0.,0.,-1.));
#11426=DIRECTION('ref_axis',(1.,0.,0.));
#11427=DIRECTION('',(0.,0.,-1.));
#11428=DIRECTION('center_axis',(0.,0.,-1.));
#11429=DIRECTION('ref_axis',(1.,0.,0.));
#11430=DIRECTION('',(0.,0.,-1.));
#11431=DIRECTION('center_axis',(0.,0.,-1.));
#11432=DIRECTION('ref_axis',(1.,0.,0.));
#11433=DIRECTION('',(0.,0.,-1.));
#11434=DIRECTION('center_axis',(0.,0.,-1.));
#11435=DIRECTION('ref_axis',(1.,0.,0.));
#11436=DIRECTION('',(0.,0.,-1.));
#11437=DIRECTION('center_axis',(0.,0.,-1.));
#11438=DIRECTION('ref_axis',(1.,0.,0.));
#11439=DIRECTION('',(0.,0.,-1.));
#11440=DIRECTION('center_axis',(0.,0.,-1.));
#11441=DIRECTION('ref_axis',(1.,0.,0.));
#11442=DIRECTION('',(0.,0.,-1.));
#11443=DIRECTION('center_axis',(0.,0.,-1.));
#11444=DIRECTION('ref_axis',(1.,0.,0.));
#11445=DIRECTION('',(0.,0.,-1.));
#11446=DIRECTION('center_axis',(0.,0.,-1.));
#11447=DIRECTION('ref_axis',(1.,0.,0.));
#11448=DIRECTION('',(0.,0.,-1.));
#11449=DIRECTION('center_axis',(0.,0.,-1.));
#11450=DIRECTION('ref_axis',(1.,0.,0.));
#11451=DIRECTION('',(0.,0.,-1.));
#11452=DIRECTION('center_axis',(0.,0.,-1.));
#11453=DIRECTION('ref_axis',(1.,0.,0.));
#11454=DIRECTION('',(0.,0.,-1.));
#11455=DIRECTION('center_axis',(0.,0.,-1.));
#11456=DIRECTION('ref_axis',(1.,0.,0.));
#11457=DIRECTION('',(0.,0.,-1.));
#11458=DIRECTION('center_axis',(0.,0.,-1.));
#11459=DIRECTION('ref_axis',(1.,0.,0.));
#11460=DIRECTION('',(0.,0.,-1.));
#11461=DIRECTION('center_axis',(0.,0.,-1.));
#11462=DIRECTION('ref_axis',(0.93843850099312,-0.345446348734193,0.));
#11463=DIRECTION('',(0.,0.,-1.));
#11464=DIRECTION('center_axis',(0.,0.,-1.));
#11465=DIRECTION('ref_axis',(1.,0.,0.));
#11466=DIRECTION('center_axis',(0.,0.,-1.));
#11467=DIRECTION('ref_axis',(0.0179642417346127,0.99983862998931,0.));
#11468=DIRECTION('',(1.22464679914735E-16,-7.95541510913586E-30,-1.));
#11469=DIRECTION('center_axis',(0.,0.,1.));
#11470=DIRECTION('ref_axis',(1.,-6.48384294707476E-14,0.));
#11471=DIRECTION('center_axis',(0.,0.,-1.));
#11472=DIRECTION('ref_axis',(1.,-6.48384294707476E-14,0.));
#11473=DIRECTION('',(1.22464679914735E-16,-7.95541510913586E-30,-1.));
#11474=DIRECTION('center_axis',(0.,0.,-1.));
#11475=DIRECTION('ref_axis',(1.,-6.48384294707476E-14,0.));
#11476=DIRECTION('',(1.22464679914735E-16,-7.95541510913586E-30,-1.));
#11477=DIRECTION('center_axis',(0.,0.,-1.));
#11478=DIRECTION('ref_axis',(1.,-6.48384294707476E-14,0.));
#11479=DIRECTION('',(1.22464679914735E-16,-7.95541510913586E-30,-1.));
#11480=DIRECTION('center_axis',(0.,0.,-1.));
#11481=DIRECTION('ref_axis',(1.,-6.48384294707476E-14,0.));
#11482=DIRECTION('',(1.22464679914735E-16,-7.95541510913586E-30,-1.));
#11483=DIRECTION('center_axis',(0.,0.,-1.));
#11484=DIRECTION('ref_axis',(1.,-6.48384294707476E-14,0.));
#11485=DIRECTION('',(1.22464679914735E-16,-7.95541510913586E-30,-1.));
#11486=DIRECTION('center_axis',(0.,0.,-1.));
#11487=DIRECTION('ref_axis',(1.,-6.48384294707476E-14,0.));
#11488=DIRECTION('',(1.22464679914735E-16,-7.95541510913586E-30,-1.));
#11489=DIRECTION('center_axis',(0.,0.,-1.));
#11490=DIRECTION('ref_axis',(1.,-6.48384294707476E-14,0.));
#11491=DIRECTION('',(1.22464679914735E-16,-7.95541510913586E-30,-1.));
#11492=DIRECTION('center_axis',(0.,0.,-1.));
#11493=DIRECTION('ref_axis',(1.,-6.48384294707476E-14,0.));
#11494=DIRECTION('',(1.22464679914735E-16,-7.95541510913586E-30,-1.));
#11495=DIRECTION('center_axis',(0.,0.,-1.));
#11496=DIRECTION('ref_axis',(1.,-6.48384294707476E-14,0.));
#11497=DIRECTION('',(1.22464679914735E-16,-7.95541510913586E-30,-1.));
#11498=DIRECTION('center_axis',(0.,0.,-1.));
#11499=DIRECTION('ref_axis',(1.,-6.48384294707476E-14,0.));
#11500=DIRECTION('',(1.22464679914735E-16,-7.95541510913586E-30,-1.));
#11501=DIRECTION('center_axis',(0.,0.,-1.));
#11502=DIRECTION('ref_axis',(1.,-6.48384294707476E-14,0.));
#11503=DIRECTION('',(1.22464679914735E-16,-7.95541510913586E-30,-1.));
#11504=DIRECTION('center_axis',(0.,0.,-1.));
#11505=DIRECTION('ref_axis',(1.,-6.48384294707476E-14,0.));
#11506=DIRECTION('',(1.22464679914735E-16,-7.95541510913586E-30,-1.));
#11507=DIRECTION('center_axis',(0.,0.,-1.));
#11508=DIRECTION('ref_axis',(1.,-6.48384294707476E-14,0.));
#11509=DIRECTION('',(1.22464679914735E-16,-7.95541510913586E-30,-1.));
#11510=DIRECTION('center_axis',(0.,0.,-1.));
#11511=DIRECTION('ref_axis',(1.,-6.48384294707476E-14,0.));
#11512=DIRECTION('',(1.22464679914735E-16,-7.95541510913586E-30,-1.));
#11513=DIRECTION('center_axis',(0.,0.,-1.));
#11514=DIRECTION('ref_axis',(-0.609341731077546,-0.792907721470424,0.));
#11515=DIRECTION('',(1.22464679914735E-16,-7.95541510913586E-30,-1.));
#11516=DIRECTION('center_axis',(0.,0.,-1.));
#11517=DIRECTION('ref_axis',(1.,-6.48384294707476E-14,0.));
#11518=DIRECTION('center_axis',(0.,0.,-1.));
#11519=DIRECTION('ref_axis',(1.,0.,0.));
#11520=DIRECTION('',(0.,0.,-1.));
#11521=DIRECTION('center_axis',(0.,0.,1.));
#11522=DIRECTION('ref_axis',(1.,0.,0.));
#11523=DIRECTION('',(0.,0.,-1.));
#11524=DIRECTION('center_axis',(0.,0.,1.));
#11525=DIRECTION('ref_axis',(1.,0.,0.));
#11526=DIRECTION('center_axis',(0.,0.,-1.));
#11527=DIRECTION('ref_axis',(1.,0.,0.));
#11528=DIRECTION('',(0.,0.,-1.));
#11529=DIRECTION('center_axis',(0.,0.,-1.));
#11530=DIRECTION('ref_axis',(1.,0.,0.));
#11531=DIRECTION('',(0.,0.,-1.));
#11532=DIRECTION('center_axis',(0.,0.,-1.));
#11533=DIRECTION('ref_axis',(1.,0.,0.));
#11534=DIRECTION('',(0.,0.,-1.));
#11535=DIRECTION('center_axis',(0.,0.,-1.));
#11536=DIRECTION('ref_axis',(1.,0.,0.));
#11537=DIRECTION('',(0.,0.,-1.));
#11538=DIRECTION('center_axis',(0.,0.,-1.));
#11539=DIRECTION('ref_axis',(1.,0.,0.));
#11540=DIRECTION('',(0.,0.,-1.));
#11541=DIRECTION('center_axis',(0.,0.,-1.));
#11542=DIRECTION('ref_axis',(1.,0.,0.));
#11543=DIRECTION('',(0.,0.,-1.));
#11544=DIRECTION('center_axis',(0.,0.,-1.));
#11545=DIRECTION('ref_axis',(1.,0.,0.));
#11546=DIRECTION('',(0.,0.,-1.));
#11547=DIRECTION('center_axis',(0.,0.,-1.));
#11548=DIRECTION('ref_axis',(1.,0.,0.));
#11549=DIRECTION('',(0.,0.,-1.));
#11550=DIRECTION('center_axis',(0.,0.,-1.));
#11551=DIRECTION('ref_axis',(1.,0.,0.));
#11552=DIRECTION('',(0.,0.,-1.));
#11553=DIRECTION('center_axis',(0.,0.,-1.));
#11554=DIRECTION('ref_axis',(1.,0.,0.));
#11555=DIRECTION('',(0.,0.,-1.));
#11556=DIRECTION('center_axis',(0.,0.,-1.));
#11557=DIRECTION('ref_axis',(1.,0.,0.));
#11558=DIRECTION('',(0.,0.,-1.));
#11559=DIRECTION('center_axis',(0.,0.,-1.));
#11560=DIRECTION('ref_axis',(1.,0.,0.));
#11561=DIRECTION('',(0.,0.,-1.));
#11562=DIRECTION('center_axis',(0.,0.,-1.));
#11563=DIRECTION('ref_axis',(1.,0.,0.));
#11564=DIRECTION('',(0.,0.,-1.));
#11565=DIRECTION('center_axis',(0.,0.,-1.));
#11566=DIRECTION('ref_axis',(0.938438517397114,-0.345446304171149,0.));
#11567=DIRECTION('',(0.,0.,-1.));
#11568=DIRECTION('center_axis',(0.,0.,-1.));
#11569=DIRECTION('ref_axis',(1.,0.,0.));
#11570=DIRECTION('center_axis',(0.,0.,-1.));
#11571=DIRECTION('ref_axis',(0.0179642700006831,0.999838629481449,0.));
#11572=DIRECTION('',(1.22464679914735E-16,-1.00728597788183E-29,-1.));
#11573=DIRECTION('center_axis',(0.,0.,1.));
#11574=DIRECTION('ref_axis',(1.,-8.21286773296134E-14,0.));
#11575=DIRECTION('center_axis',(0.,0.,-1.));
#11576=DIRECTION('ref_axis',(1.,-8.21286773296134E-14,0.));
#11577=DIRECTION('',(1.22464679914735E-16,-1.00728597788183E-29,-1.));
#11578=DIRECTION('center_axis',(0.,0.,-1.));
#11579=DIRECTION('ref_axis',(1.,-8.21286773296134E-14,0.));
#11580=DIRECTION('',(1.22464679914735E-16,-1.00728597788183E-29,-1.));
#11581=DIRECTION('center_axis',(0.,0.,-1.));
#11582=DIRECTION('ref_axis',(1.,-8.21286773296134E-14,0.));
#11583=DIRECTION('',(1.22464679914735E-16,-1.00728597788183E-29,-1.));
#11584=DIRECTION('center_axis',(0.,0.,-1.));
#11585=DIRECTION('ref_axis',(1.,-8.21286773296134E-14,0.));
#11586=DIRECTION('',(1.22464679914735E-16,-1.00728597788183E-29,-1.));
#11587=DIRECTION('center_axis',(0.,0.,-1.));
#11588=DIRECTION('ref_axis',(1.,-8.21286773296134E-14,0.));
#11589=DIRECTION('',(1.22464679914735E-16,-1.00728597788183E-29,-1.));
#11590=DIRECTION('center_axis',(0.,0.,-1.));
#11591=DIRECTION('ref_axis',(1.,-8.21286773296134E-14,0.));
#11592=DIRECTION('',(1.22464679914735E-16,-1.00728597788183E-29,-1.));
#11593=DIRECTION('center_axis',(0.,0.,-1.));
#11594=DIRECTION('ref_axis',(1.,-8.21286773296134E-14,0.));
#11595=DIRECTION('',(1.22464679914735E-16,-1.00728597788183E-29,-1.));
#11596=DIRECTION('center_axis',(0.,0.,-1.));
#11597=DIRECTION('ref_axis',(1.,-8.21286773296134E-14,0.));
#11598=DIRECTION('',(1.22464679914735E-16,-1.00728597788183E-29,-1.));
#11599=DIRECTION('center_axis',(0.,0.,-1.));
#11600=DIRECTION('ref_axis',(1.,-8.21286773296134E-14,0.));
#11601=DIRECTION('',(1.22464679914735E-16,-1.00728597788183E-29,-1.));
#11602=DIRECTION('center_axis',(0.,0.,-1.));
#11603=DIRECTION('ref_axis',(1.,-8.21286773296134E-14,0.));
#11604=DIRECTION('',(1.22464679914735E-16,-1.00728597788183E-29,-1.));
#11605=DIRECTION('center_axis',(0.,0.,-1.));
#11606=DIRECTION('ref_axis',(1.,-8.21286773296134E-14,0.));
#11607=DIRECTION('',(1.22464679914735E-16,-1.00728597788183E-29,-1.));
#11608=DIRECTION('center_axis',(0.,0.,-1.));
#11609=DIRECTION('ref_axis',(1.,-8.21286773296134E-14,0.));
#11610=DIRECTION('',(1.22464679914735E-16,-1.00728597788183E-29,-1.));
#11611=DIRECTION('center_axis',(0.,0.,-1.));
#11612=DIRECTION('ref_axis',(1.,-8.21286773296134E-14,0.));
#11613=DIRECTION('',(1.22464679914735E-16,-1.00728597788183E-29,-1.));
#11614=DIRECTION('center_axis',(0.,0.,-1.));
#11615=DIRECTION('ref_axis',(1.,-8.21286773296134E-14,0.));
#11616=DIRECTION('',(1.22464679914735E-16,-1.00728597788183E-29,-1.));
#11617=DIRECTION('center_axis',(0.,0.,-1.));
#11618=DIRECTION('ref_axis',(-0.609341750416278,-0.792907706608799,0.));
#11619=DIRECTION('',(1.22464679914735E-16,-1.00728597788183E-29,-1.));
#11620=DIRECTION('center_axis',(0.,0.,-1.));
#11621=DIRECTION('ref_axis',(1.,-8.21286773296134E-14,0.));
#11622=DIRECTION('center_axis',(0.,0.,-1.));
#11623=DIRECTION('ref_axis',(1.,0.,0.));
#11624=DIRECTION('',(0.,0.,-1.));
#11625=DIRECTION('center_axis',(0.,0.,1.));
#11626=DIRECTION('ref_axis',(1.,0.,0.));
#11627=DIRECTION('',(0.,0.,-1.));
#11628=DIRECTION('center_axis',(0.,0.,1.));
#11629=DIRECTION('ref_axis',(1.,0.,0.));
#11630=DIRECTION('center_axis',(0.,0.,-1.));
#11631=DIRECTION('ref_axis',(1.,0.,0.));
#11632=DIRECTION('',(0.,0.,-1.));
#11633=DIRECTION('center_axis',(0.,0.,-1.));
#11634=DIRECTION('ref_axis',(1.,0.,0.));
#11635=DIRECTION('',(0.,0.,-1.));
#11636=DIRECTION('center_axis',(0.,0.,-1.));
#11637=DIRECTION('ref_axis',(1.,0.,0.));
#11638=DIRECTION('',(0.,0.,-1.));
#11639=DIRECTION('center_axis',(0.,0.,-1.));
#11640=DIRECTION('ref_axis',(1.,0.,0.));
#11641=DIRECTION('',(0.,0.,-1.));
#11642=DIRECTION('center_axis',(0.,0.,-1.));
#11643=DIRECTION('ref_axis',(1.,0.,0.));
#11644=DIRECTION('',(0.,0.,-1.));
#11645=DIRECTION('center_axis',(0.,0.,-1.));
#11646=DIRECTION('ref_axis',(1.,0.,0.));
#11647=DIRECTION('',(0.,0.,-1.));
#11648=DIRECTION('center_axis',(0.,0.,-1.));
#11649=DIRECTION('ref_axis',(1.,0.,0.));
#11650=DIRECTION('',(0.,0.,-1.));
#11651=DIRECTION('center_axis',(0.,0.,-1.));
#11652=DIRECTION('ref_axis',(1.,0.,0.));
#11653=DIRECTION('',(0.,0.,-1.));
#11654=DIRECTION('center_axis',(0.,0.,-1.));
#11655=DIRECTION('ref_axis',(1.,0.,0.));
#11656=DIRECTION('',(0.,0.,-1.));
#11657=DIRECTION('center_axis',(0.,0.,-1.));
#11658=DIRECTION('ref_axis',(1.,0.,0.));
#11659=DIRECTION('',(0.,0.,-1.));
#11660=DIRECTION('center_axis',(0.,0.,-1.));
#11661=DIRECTION('ref_axis',(1.,0.,0.));
#11662=DIRECTION('',(0.,0.,-1.));
#11663=DIRECTION('center_axis',(0.,0.,-1.));
#11664=DIRECTION('ref_axis',(1.,0.,0.));
#11665=DIRECTION('',(0.,0.,-1.));
#11666=DIRECTION('center_axis',(0.,0.,-1.));
#11667=DIRECTION('ref_axis',(1.,0.,0.));
#11668=DIRECTION('',(0.,0.,-1.));
#11669=DIRECTION('center_axis',(0.,0.,-1.));
#11670=DIRECTION('ref_axis',(0.93843850644045,-0.345446333935992,0.));
#11671=DIRECTION('',(0.,0.,-1.));
#11672=DIRECTION('center_axis',(0.,0.,-1.));
#11673=DIRECTION('ref_axis',(1.,0.,0.));
#11674=DIRECTION('center_axis',(0.,0.,-1.));
#11675=DIRECTION('ref_axis',(0.0179642658157032,0.999838629556641,0.));
#11676=DIRECTION('',(1.22464679914735E-16,-1.00728597788183E-29,-1.));
#11677=DIRECTION('center_axis',(0.,0.,1.));
#11678=DIRECTION('ref_axis',(1.,-8.21286773296138E-14,0.));
#11679=DIRECTION('center_axis',(0.,0.,-1.));
#11680=DIRECTION('ref_axis',(1.,-8.21286773296138E-14,0.));
#11681=DIRECTION('',(1.22464679914735E-16,-1.00728597788183E-29,-1.));
#11682=DIRECTION('center_axis',(0.,0.,-1.));
#11683=DIRECTION('ref_axis',(1.,-8.21286773296138E-14,0.));
#11684=DIRECTION('',(1.22464679914735E-16,-1.00728597788183E-29,-1.));
#11685=DIRECTION('center_axis',(0.,0.,-1.));
#11686=DIRECTION('ref_axis',(1.,-8.21286773296138E-14,0.));
#11687=DIRECTION('',(1.22464679914735E-16,-1.00728597788183E-29,-1.));
#11688=DIRECTION('center_axis',(0.,0.,-1.));
#11689=DIRECTION('ref_axis',(1.,-8.21286773296138E-14,0.));
#11690=DIRECTION('',(1.22464679914735E-16,-1.00728597788183E-29,-1.));
#11691=DIRECTION('center_axis',(0.,0.,-1.));
#11692=DIRECTION('ref_axis',(1.,-8.21286773296138E-14,0.));
#11693=DIRECTION('',(1.22464679914735E-16,-1.00728597788183E-29,-1.));
#11694=DIRECTION('center_axis',(0.,0.,-1.));
#11695=DIRECTION('ref_axis',(1.,-8.21286773296138E-14,0.));
#11696=DIRECTION('',(1.22464679914735E-16,-1.00728597788183E-29,-1.));
#11697=DIRECTION('center_axis',(0.,0.,-1.));
#11698=DIRECTION('ref_axis',(1.,-8.21286773296138E-14,0.));
#11699=DIRECTION('',(1.22464679914735E-16,-1.00728597788183E-29,-1.));
#11700=DIRECTION('center_axis',(0.,0.,-1.));
#11701=DIRECTION('ref_axis',(1.,-8.21286773296138E-14,0.));
#11702=DIRECTION('',(1.22464679914735E-16,-1.00728597788183E-29,-1.));
#11703=DIRECTION('center_axis',(0.,0.,-1.));
#11704=DIRECTION('ref_axis',(1.,-8.21286773296138E-14,0.));
#11705=DIRECTION('',(1.22464679914735E-16,-1.00728597788183E-29,-1.));
#11706=DIRECTION('center_axis',(0.,0.,-1.));
#11707=DIRECTION('ref_axis',(1.,-8.21286773296138E-14,0.));
#11708=DIRECTION('',(1.22464679914735E-16,-1.00728597788183E-29,-1.));
#11709=DIRECTION('center_axis',(0.,0.,-1.));
#11710=DIRECTION('ref_axis',(1.,-8.21286773296138E-14,0.));
#11711=DIRECTION('',(1.22464679914735E-16,-1.00728597788183E-29,-1.));
#11712=DIRECTION('center_axis',(0.,0.,-1.));
#11713=DIRECTION('ref_axis',(1.,-8.21286773296138E-14,0.));
#11714=DIRECTION('',(1.22464679914735E-16,-1.00728597788183E-29,-1.));
#11715=DIRECTION('center_axis',(0.,0.,-1.));
#11716=DIRECTION('ref_axis',(1.,-8.21286773296138E-14,0.));
#11717=DIRECTION('',(1.22464679914735E-16,-1.00728597788183E-29,-1.));
#11718=DIRECTION('center_axis',(0.,0.,-1.));
#11719=DIRECTION('ref_axis',(1.,-8.21286773296138E-14,0.));
#11720=DIRECTION('',(1.22464679914735E-16,-1.00728597788183E-29,-1.));
#11721=DIRECTION('center_axis',(0.,0.,-1.));
#11722=DIRECTION('ref_axis',(-0.609341722721044,-0.792907727892313,0.));
#11723=DIRECTION('',(1.22464679914735E-16,-1.00728597788183E-29,-1.));
#11724=DIRECTION('center_axis',(0.,0.,-1.));
#11725=DIRECTION('ref_axis',(1.,-8.21286773296138E-14,0.));
#11726=DIRECTION('center_axis',(0.,0.,1.));
#11727=DIRECTION('ref_axis',(0.000672283037009468,0.999999774017734,0.));
#11728=DIRECTION('',(0.,0.,1.));
#11729=DIRECTION('center_axis',(0.,0.,-1.));
#11730=DIRECTION('ref_axis',(-1.,0.,0.));
#11731=DIRECTION('center_axis',(0.,0.,-1.));
#11732=DIRECTION('ref_axis',(-1.,0.,0.));
#11733=DIRECTION('center_axis',(0.,0.,1.));
#11734=DIRECTION('ref_axis',(-1.,0.,0.));
#11735=DIRECTION('',(0.,0.,1.));
#11736=DIRECTION('center_axis',(0.,0.,1.));
#11737=DIRECTION('ref_axis',(-1.,0.,0.));
#11738=DIRECTION('',(0.,0.,1.));
#11739=DIRECTION('center_axis',(0.,0.,1.));
#11740=DIRECTION('ref_axis',(-1.,0.,0.));
#11741=DIRECTION('',(0.,0.,1.));
#11742=DIRECTION('center_axis',(0.,0.,1.));
#11743=DIRECTION('ref_axis',(-1.,0.,0.));
#11744=DIRECTION('',(0.,0.,1.));
#11745=DIRECTION('center_axis',(0.,0.,1.));
#11746=DIRECTION('ref_axis',(-1.,0.,0.));
#11747=DIRECTION('',(0.,0.,1.));
#11748=DIRECTION('center_axis',(0.,0.,1.));
#11749=DIRECTION('ref_axis',(-1.,0.,0.));
#11750=DIRECTION('',(0.,0.,1.));
#11751=DIRECTION('center_axis',(0.,0.,1.));
#11752=DIRECTION('ref_axis',(-1.,0.,0.));
#11753=DIRECTION('',(0.,0.,1.));
#11754=DIRECTION('center_axis',(0.,0.,1.));
#11755=DIRECTION('ref_axis',(-1.,0.,0.));
#11756=DIRECTION('',(0.,0.,1.));
#11757=DIRECTION('center_axis',(0.,0.,1.));
#11758=DIRECTION('ref_axis',(-1.,0.,0.));
#11759=DIRECTION('',(0.,0.,1.));
#11760=DIRECTION('center_axis',(0.,0.,1.));
#11761=DIRECTION('ref_axis',(-1.,0.,0.));
#11762=DIRECTION('',(0.,0.,1.));
#11763=DIRECTION('center_axis',(0.,0.,1.));
#11764=DIRECTION('ref_axis',(-1.,0.,0.));
#11765=DIRECTION('',(0.,0.,1.));
#11766=DIRECTION('center_axis',(0.,0.,1.));
#11767=DIRECTION('ref_axis',(-1.,0.,0.));
#11768=DIRECTION('',(0.,0.,1.));
#11769=DIRECTION('center_axis',(0.,0.,1.));
#11770=DIRECTION('ref_axis',(-1.,0.,0.));
#11771=DIRECTION('',(0.,0.,1.));
#11772=DIRECTION('center_axis',(0.,0.,1.));
#11773=DIRECTION('ref_axis',(-0.938007161567557,-0.346615875066297,0.));
#11774=DIRECTION('',(0.,0.,1.));
#11775=DIRECTION('center_axis',(0.,0.,-1.));
#11776=DIRECTION('ref_axis',(-1.,0.,0.));
#11777=DIRECTION('center_axis',(0.,0.,1.));
#11778=DIRECTION('ref_axis',(0.000672370108301728,0.999999773959193,0.));
#11779=DIRECTION('',(0.,0.,1.));
#11780=DIRECTION('center_axis',(0.,0.,-1.));
#11781=DIRECTION('ref_axis',(-1.,0.,0.));
#11782=DIRECTION('center_axis',(0.,0.,-1.));
#11783=DIRECTION('ref_axis',(-1.,0.,0.));
#11784=DIRECTION('center_axis',(0.,0.,1.));
#11785=DIRECTION('ref_axis',(-1.,0.,0.));
#11786=DIRECTION('',(0.,0.,1.));
#11787=DIRECTION('center_axis',(0.,0.,1.));
#11788=DIRECTION('ref_axis',(-1.,0.,0.));
#11789=DIRECTION('',(0.,0.,1.));
#11790=DIRECTION('center_axis',(0.,0.,1.));
#11791=DIRECTION('ref_axis',(-1.,0.,0.));
#11792=DIRECTION('',(0.,0.,1.));
#11793=DIRECTION('center_axis',(0.,0.,1.));
#11794=DIRECTION('ref_axis',(-1.,0.,0.));
#11795=DIRECTION('',(0.,0.,1.));
#11796=DIRECTION('center_axis',(0.,0.,1.));
#11797=DIRECTION('ref_axis',(-1.,0.,0.));
#11798=DIRECTION('',(0.,0.,1.));
#11799=DIRECTION('center_axis',(0.,0.,1.));
#11800=DIRECTION('ref_axis',(-1.,0.,0.));
#11801=DIRECTION('',(0.,0.,1.));
#11802=DIRECTION('center_axis',(0.,0.,1.));
#11803=DIRECTION('ref_axis',(-1.,0.,0.));
#11804=DIRECTION('',(0.,0.,1.));
#11805=DIRECTION('center_axis',(0.,0.,1.));
#11806=DIRECTION('ref_axis',(-1.,0.,0.));
#11807=DIRECTION('',(0.,0.,1.));
#11808=DIRECTION('center_axis',(0.,0.,1.));
#11809=DIRECTION('ref_axis',(-1.,0.,0.));
#11810=DIRECTION('',(0.,0.,1.));
#11811=DIRECTION('center_axis',(0.,0.,1.));
#11812=DIRECTION('ref_axis',(-1.,0.,0.));
#11813=DIRECTION('',(0.,0.,1.));
#11814=DIRECTION('center_axis',(0.,0.,1.));
#11815=DIRECTION('ref_axis',(-1.,0.,0.));
#11816=DIRECTION('',(0.,0.,1.));
#11817=DIRECTION('center_axis',(0.,0.,1.));
#11818=DIRECTION('ref_axis',(-1.,0.,0.));
#11819=DIRECTION('',(0.,0.,1.));
#11820=DIRECTION('center_axis',(0.,0.,1.));
#11821=DIRECTION('ref_axis',(-1.,0.,0.));
#11822=DIRECTION('',(0.,0.,1.));
#11823=DIRECTION('center_axis',(0.,0.,1.));
#11824=DIRECTION('ref_axis',(-0.938007170856739,-0.346615849928038,0.));
#11825=DIRECTION('',(0.,0.,1.));
#11826=DIRECTION('center_axis',(0.,0.,-1.));
#11827=DIRECTION('ref_axis',(-1.,0.,0.));
#11828=DIRECTION('center_axis',(0.,0.,1.));
#11829=DIRECTION('ref_axis',(-1.,-7.80244585388103E-14,0.));
#11830=DIRECTION('',(-1.22464679914735E-16,-9.57023793830256E-30,1.));
#11831=DIRECTION('center_axis',(0.,0.,-1.));
#11832=DIRECTION('ref_axis',(-1.,-7.80244585388103E-14,0.));
#11833=DIRECTION('center_axis',(0.,0.,1.));
#11834=DIRECTION('ref_axis',(-1.,-7.80244585388103E-14,0.));
#11835=DIRECTION('',(-1.22464679914735E-16,-9.57023793830256E-30,1.));
#11836=DIRECTION('center_axis',(0.,0.,1.));
#11837=DIRECTION('ref_axis',(-1.,-7.80244585388103E-14,0.));
#11838=DIRECTION('',(-1.22464679914735E-16,-9.57023793830256E-30,1.));
#11839=DIRECTION('center_axis',(0.,0.,1.));
#11840=DIRECTION('ref_axis',(-1.,-7.80244585388103E-14,0.));
#11841=DIRECTION('',(-1.22464679914735E-16,-9.57023793830256E-30,1.));
#11842=DIRECTION('center_axis',(0.,0.,1.));
#11843=DIRECTION('ref_axis',(-1.,-7.80244585388103E-14,0.));
#11844=DIRECTION('',(-1.22464679914735E-16,-9.57023793830256E-30,1.));
#11845=DIRECTION('center_axis',(0.,0.,1.));
#11846=DIRECTION('ref_axis',(-1.,-7.80244585388103E-14,0.));
#11847=DIRECTION('',(-1.22464679914735E-16,-9.57023793830256E-30,1.));
#11848=DIRECTION('center_axis',(0.,0.,1.));
#11849=DIRECTION('ref_axis',(-1.,-7.80244585388103E-14,0.));
#11850=DIRECTION('',(-1.22464679914735E-16,-9.57023793830256E-30,1.));
#11851=DIRECTION('center_axis',(0.,0.,1.));
#11852=DIRECTION('ref_axis',(-1.,-7.80244585388103E-14,0.));
#11853=DIRECTION('',(-1.22464679914735E-16,-9.57023793830256E-30,1.));
#11854=DIRECTION('center_axis',(0.,0.,1.));
#11855=DIRECTION('ref_axis',(-1.,-7.80244585388103E-14,0.));
#11856=DIRECTION('',(-1.22464679914735E-16,-9.57023793830256E-30,1.));
#11857=DIRECTION('center_axis',(0.,0.,1.));
#11858=DIRECTION('ref_axis',(-1.,-7.80244585388103E-14,0.));
#11859=DIRECTION('',(-1.22464679914735E-16,-9.57023793830256E-30,1.));
#11860=DIRECTION('center_axis',(0.,0.,1.));
#11861=DIRECTION('ref_axis',(-1.,-7.80244585388103E-14,0.));
#11862=DIRECTION('',(-1.22464679914735E-16,-9.57023793830256E-30,1.));
#11863=DIRECTION('center_axis',(0.,0.,1.));
#11864=DIRECTION('ref_axis',(-1.,-7.80244585388103E-14,0.));
#11865=DIRECTION('',(-1.22464679914735E-16,-9.57023793830256E-30,1.));
#11866=DIRECTION('center_axis',(0.,0.,1.));
#11867=DIRECTION('ref_axis',(-1.,-7.80244585388103E-14,0.));
#11868=DIRECTION('',(-1.22464679914735E-16,-9.57023793830256E-30,1.));
#11869=DIRECTION('center_axis',(0.,0.,1.));
#11870=DIRECTION('ref_axis',(-1.,-7.80244585388103E-14,0.));
#11871=DIRECTION('',(-1.22464679914735E-16,-9.57023793830256E-30,1.));
#11872=DIRECTION('center_axis',(0.,0.,1.));
#11873=DIRECTION('ref_axis',(0.609168748886822,-0.793040626563144,0.));
#11874=DIRECTION('',(-1.22464679914735E-16,-9.57023793830256E-30,1.));
#11875=DIRECTION('center_axis',(0.,0.,1.));
#11876=DIRECTION('ref_axis',(-1.,-7.80244585388103E-14,0.));
#11877=DIRECTION('center_axis',(0.,0.,1.));
#11878=DIRECTION('ref_axis',(-1.,-7.80244585388103E-14,0.));
#11879=DIRECTION('',(-1.22464679914735E-16,-9.57023793830256E-30,1.));
#11880=DIRECTION('center_axis',(0.,0.,-1.));
#11881=DIRECTION('ref_axis',(-1.,-7.80244585388103E-14,0.));
#11882=DIRECTION('center_axis',(0.,0.,1.));
#11883=DIRECTION('ref_axis',(-1.,-7.80244585388103E-14,0.));
#11884=DIRECTION('',(-1.22464679914735E-16,-9.57023793830256E-30,1.));
#11885=DIRECTION('center_axis',(0.,0.,1.));
#11886=DIRECTION('ref_axis',(-1.,-7.80244585388103E-14,0.));
#11887=DIRECTION('',(-1.22464679914735E-16,-9.57023793830256E-30,1.));
#11888=DIRECTION('center_axis',(0.,0.,1.));
#11889=DIRECTION('ref_axis',(-1.,-7.80244585388103E-14,0.));
#11890=DIRECTION('',(-1.22464679914735E-16,-9.57023793830256E-30,1.));
#11891=DIRECTION('center_axis',(0.,0.,1.));
#11892=DIRECTION('ref_axis',(-1.,-7.80244585388103E-14,0.));
#11893=DIRECTION('',(-1.22464679914735E-16,-9.57023793830256E-30,1.));
#11894=DIRECTION('center_axis',(0.,0.,1.));
#11895=DIRECTION('ref_axis',(-1.,-7.80244585388103E-14,0.));
#11896=DIRECTION('',(-1.22464679914735E-16,-9.57023793830256E-30,1.));
#11897=DIRECTION('center_axis',(0.,0.,1.));
#11898=DIRECTION('ref_axis',(-1.,-7.80244585388103E-14,0.));
#11899=DIRECTION('',(-1.22464679914735E-16,-9.57023793830256E-30,1.));
#11900=DIRECTION('center_axis',(0.,0.,1.));
#11901=DIRECTION('ref_axis',(-1.,-7.80244585388103E-14,0.));
#11902=DIRECTION('',(-1.22464679914735E-16,-9.57023793830256E-30,1.));
#11903=DIRECTION('center_axis',(0.,0.,1.));
#11904=DIRECTION('ref_axis',(-1.,-7.80244585388103E-14,0.));
#11905=DIRECTION('',(-1.22464679914735E-16,-9.57023793830256E-30,1.));
#11906=DIRECTION('center_axis',(0.,0.,1.));
#11907=DIRECTION('ref_axis',(-1.,-7.80244585388103E-14,0.));
#11908=DIRECTION('',(-1.22464679914735E-16,-9.57023793830256E-30,1.));
#11909=DIRECTION('center_axis',(0.,0.,1.));
#11910=DIRECTION('ref_axis',(-1.,-7.80244585388103E-14,0.));
#11911=DIRECTION('',(-1.22464679914735E-16,-9.57023793830256E-30,1.));
#11912=DIRECTION('center_axis',(0.,0.,1.));
#11913=DIRECTION('ref_axis',(-1.,-7.80244585388103E-14,0.));
#11914=DIRECTION('',(-1.22464679914735E-16,-9.57023793830256E-30,1.));
#11915=DIRECTION('center_axis',(0.,0.,1.));
#11916=DIRECTION('ref_axis',(-1.,-7.80244585388103E-14,0.));
#11917=DIRECTION('',(-1.22464679914735E-16,-9.57023793830256E-30,1.));
#11918=DIRECTION('center_axis',(0.,0.,1.));
#11919=DIRECTION('ref_axis',(-1.,-7.80244585388103E-14,0.));
#11920=DIRECTION('',(-1.22464679914735E-16,-9.57023793830256E-30,1.));
#11921=DIRECTION('center_axis',(0.,0.,1.));
#11922=DIRECTION('ref_axis',(0.609168765471054,-0.793040613824079,0.));
#11923=DIRECTION('',(-1.22464679914735E-16,-9.57023793830256E-30,1.));
#11924=DIRECTION('center_axis',(0.,0.,1.));
#11925=DIRECTION('ref_axis',(-1.,-7.80244585388103E-14,0.));
#11926=DIRECTION('center_axis',(0.,0.,1.));
#11927=DIRECTION('ref_axis',(-1.,0.,0.));
#11928=DIRECTION('',(0.,0.,1.));
#11929=DIRECTION('center_axis',(0.,0.,-1.));
#11930=DIRECTION('ref_axis',(-1.,0.,0.));
#11931=DIRECTION('',(0.,0.,1.));
#11932=DIRECTION('center_axis',(0.,0.,-1.));
#11933=DIRECTION('ref_axis',(-1.,0.,0.));
#11934=DIRECTION('center_axis',(0.,0.,-1.));
#11935=DIRECTION('ref_axis',(-1.,0.,0.));
#11936=DIRECTION('center_axis',(0.,0.,1.));
#11937=DIRECTION('ref_axis',(-1.,0.,0.));
#11938=DIRECTION('',(0.,0.,1.));
#11939=DIRECTION('center_axis',(0.,0.,1.));
#11940=DIRECTION('ref_axis',(-1.,0.,0.));
#11941=DIRECTION('',(0.,0.,1.));
#11942=DIRECTION('center_axis',(0.,0.,1.));
#11943=DIRECTION('ref_axis',(-1.,0.,0.));
#11944=DIRECTION('',(0.,0.,1.));
#11945=DIRECTION('center_axis',(0.,0.,1.));
#11946=DIRECTION('ref_axis',(-1.,0.,0.));
#11947=DIRECTION('',(0.,0.,1.));
#11948=DIRECTION('center_axis',(0.,0.,1.));
#11949=DIRECTION('ref_axis',(-1.,0.,0.));
#11950=DIRECTION('',(0.,0.,1.));
#11951=DIRECTION('center_axis',(0.,0.,1.));
#11952=DIRECTION('ref_axis',(-1.,0.,0.));
#11953=DIRECTION('',(0.,0.,1.));
#11954=DIRECTION('center_axis',(0.,0.,1.));
#11955=DIRECTION('ref_axis',(-1.,0.,0.));
#11956=DIRECTION('',(0.,0.,1.));
#11957=DIRECTION('center_axis',(0.,0.,1.));
#11958=DIRECTION('ref_axis',(-1.,0.,0.));
#11959=DIRECTION('',(0.,0.,1.));
#11960=DIRECTION('center_axis',(0.,0.,1.));
#11961=DIRECTION('ref_axis',(-1.,0.,0.));
#11962=DIRECTION('',(0.,0.,1.));
#11963=DIRECTION('center_axis',(0.,0.,1.));
#11964=DIRECTION('ref_axis',(-1.,0.,0.));
#11965=DIRECTION('',(0.,0.,1.));
#11966=DIRECTION('center_axis',(0.,0.,1.));
#11967=DIRECTION('ref_axis',(-1.,0.,0.));
#11968=DIRECTION('',(0.,0.,1.));
#11969=DIRECTION('center_axis',(0.,0.,1.));
#11970=DIRECTION('ref_axis',(-1.,0.,0.));
#11971=DIRECTION('',(0.,0.,1.));
#11972=DIRECTION('center_axis',(0.,0.,1.));
#11973=DIRECTION('ref_axis',(-1.,0.,0.));
#11974=DIRECTION('',(0.,0.,1.));
#11975=DIRECTION('center_axis',(0.,0.,1.));
#11976=DIRECTION('ref_axis',(-0.938007151213456,-0.346615903086422,0.));
#11977=DIRECTION('',(0.,0.,1.));
#11978=DIRECTION('center_axis',(0.,0.,-1.));
#11979=DIRECTION('ref_axis',(-1.,0.,0.));
#11980=DIRECTION('center_axis',(0.,0.,1.));
#11981=DIRECTION('ref_axis',(-1.,-7.80244585388104E-14,0.));
#11982=DIRECTION('',(-1.22464679914735E-16,-9.57023793830257E-30,1.));
#11983=DIRECTION('center_axis',(0.,0.,-1.));
#11984=DIRECTION('ref_axis',(-1.,-7.80244585388104E-14,0.));
#11985=DIRECTION('center_axis',(0.,0.,1.));
#11986=DIRECTION('ref_axis',(-1.,-7.80244585388104E-14,0.));
#11987=DIRECTION('',(-1.22464679914735E-16,-9.57023793830257E-30,1.));
#11988=DIRECTION('center_axis',(0.,0.,1.));
#11989=DIRECTION('ref_axis',(-1.,-7.80244585388104E-14,0.));
#11990=DIRECTION('',(-1.22464679914735E-16,-9.57023793830257E-30,1.));
#11991=DIRECTION('center_axis',(0.,0.,1.));
#11992=DIRECTION('ref_axis',(-1.,-7.80244585388104E-14,0.));
#11993=DIRECTION('',(-1.22464679914735E-16,-9.57023793830257E-30,1.));
#11994=DIRECTION('center_axis',(0.,0.,1.));
#11995=DIRECTION('ref_axis',(-1.,-7.80244585388104E-14,0.));
#11996=DIRECTION('',(-1.22464679914735E-16,-9.57023793830257E-30,1.));
#11997=DIRECTION('center_axis',(0.,0.,1.));
#11998=DIRECTION('ref_axis',(-1.,-7.80244585388104E-14,0.));
#11999=DIRECTION('',(-1.22464679914735E-16,-9.57023793830257E-30,1.));
#12000=DIRECTION('center_axis',(0.,0.,1.));
#12001=DIRECTION('ref_axis',(-1.,-7.80244585388104E-14,0.));
#12002=DIRECTION('',(-1.22464679914735E-16,-9.57023793830257E-30,1.));
#12003=DIRECTION('center_axis',(0.,0.,1.));
#12004=DIRECTION('ref_axis',(-1.,-7.80244585388104E-14,0.));
#12005=DIRECTION('',(-1.22464679914735E-16,-9.57023793830257E-30,1.));
#12006=DIRECTION('center_axis',(0.,0.,1.));
#12007=DIRECTION('ref_axis',(-1.,-7.80244585388104E-14,0.));
#12008=DIRECTION('',(-1.22464679914735E-16,-9.57023793830257E-30,1.));
#12009=DIRECTION('center_axis',(0.,0.,1.));
#12010=DIRECTION('ref_axis',(-1.,-7.80244585388104E-14,0.));
#12011=DIRECTION('',(-1.22464679914735E-16,-9.57023793830257E-30,1.));
#12012=DIRECTION('center_axis',(0.,0.,1.));
#12013=DIRECTION('ref_axis',(-1.,-7.80244585388104E-14,0.));
#12014=DIRECTION('',(-1.22464679914735E-16,-9.57023793830257E-30,1.));
#12015=DIRECTION('center_axis',(0.,0.,1.));
#12016=DIRECTION('ref_axis',(-1.,-7.80244585388104E-14,0.));
#12017=DIRECTION('',(-1.22464679914735E-16,-9.57023793830257E-30,1.));
#12018=DIRECTION('center_axis',(0.,0.,1.));
#12019=DIRECTION('ref_axis',(-1.,-7.80244585388104E-14,0.));
#12020=DIRECTION('',(-1.22464679914735E-16,-9.57023793830257E-30,1.));
#12021=DIRECTION('center_axis',(0.,0.,1.));
#12022=DIRECTION('ref_axis',(-1.,-7.80244585388104E-14,0.));
#12023=DIRECTION('',(-1.22464679914735E-16,-9.57023793830257E-30,1.));
#12024=DIRECTION('center_axis',(0.,0.,1.));
#12025=DIRECTION('ref_axis',(0.609168720998191,-0.793040647985605,0.));
#12026=DIRECTION('',(-1.22464679914735E-16,-9.57023793830257E-30,1.));
#12027=DIRECTION('center_axis',(0.,0.,1.));
#12028=DIRECTION('ref_axis',(-1.,-7.80244585388104E-14,0.));
#12029=DIRECTION('center_axis',(0.,0.,1.));
#12030=DIRECTION('ref_axis',(-1.,0.,0.));
#12031=DIRECTION('',(0.,0.,1.));
#12032=DIRECTION('center_axis',(0.,0.,-1.));
#12033=DIRECTION('ref_axis',(-1.,0.,0.));
#12034=DIRECTION('',(0.,0.,1.));
#12035=DIRECTION('center_axis',(0.,0.,-1.));
#12036=DIRECTION('ref_axis',(-1.,0.,0.));
#12037=DIRECTION('center_axis',(0.,0.,-1.));
#12038=DIRECTION('ref_axis',(-1.,0.,0.));
#12039=DIRECTION('center_axis',(0.,0.,1.));
#12040=DIRECTION('ref_axis',(-1.,0.,0.));
#12041=DIRECTION('',(0.,0.,1.));
#12042=DIRECTION('center_axis',(0.,0.,1.));
#12043=DIRECTION('ref_axis',(-1.,0.,0.));
#12044=DIRECTION('',(0.,0.,1.));
#12045=DIRECTION('center_axis',(0.,0.,1.));
#12046=DIRECTION('ref_axis',(-1.,0.,0.));
#12047=DIRECTION('',(0.,0.,1.));
#12048=DIRECTION('center_axis',(0.,0.,1.));
#12049=DIRECTION('ref_axis',(-1.,0.,0.));
#12050=DIRECTION('',(0.,0.,1.));
#12051=DIRECTION('center_axis',(0.,0.,1.));
#12052=DIRECTION('ref_axis',(-1.,0.,0.));
#12053=DIRECTION('',(0.,0.,1.));
#12054=DIRECTION('center_axis',(0.,0.,1.));
#12055=DIRECTION('ref_axis',(-1.,0.,0.));
#12056=DIRECTION('',(0.,0.,1.));
#12057=DIRECTION('center_axis',(0.,0.,1.));
#12058=DIRECTION('ref_axis',(-1.,0.,0.));
#12059=DIRECTION('',(0.,0.,1.));
#12060=DIRECTION('center_axis',(0.,0.,1.));
#12061=DIRECTION('ref_axis',(-1.,0.,0.));
#12062=DIRECTION('',(0.,0.,1.));
#12063=DIRECTION('center_axis',(0.,0.,1.));
#12064=DIRECTION('ref_axis',(-1.,0.,0.));
#12065=DIRECTION('',(0.,0.,1.));
#12066=DIRECTION('center_axis',(0.,0.,1.));
#12067=DIRECTION('ref_axis',(-1.,0.,0.));
#12068=DIRECTION('',(0.,0.,1.));
#12069=DIRECTION('center_axis',(0.,0.,1.));
#12070=DIRECTION('ref_axis',(-1.,0.,0.));
#12071=DIRECTION('',(0.,0.,1.));
#12072=DIRECTION('center_axis',(0.,0.,1.));
#12073=DIRECTION('ref_axis',(-1.,0.,0.));
#12074=DIRECTION('',(0.,0.,1.));
#12075=DIRECTION('center_axis',(0.,0.,1.));
#12076=DIRECTION('ref_axis',(-1.,0.,0.));
#12077=DIRECTION('',(0.,0.,1.));
#12078=DIRECTION('center_axis',(0.,0.,1.));
#12079=DIRECTION('ref_axis',(-0.938007139797982,-0.346615933978819,0.));
#12080=DIRECTION('',(0.,0.,1.));
#12081=DIRECTION('center_axis',(0.,0.,-1.));
#12082=DIRECTION('ref_axis',(-1.,0.,0.));
#12083=DIRECTION('center_axis',(0.,0.,1.));
#12084=DIRECTION('ref_axis',(-1.,-7.2244869017417E-14,0.));
#12085=DIRECTION('',(-1.22464679914735E-16,-8.86244235752658E-30,1.));
#12086=DIRECTION('center_axis',(0.,0.,-1.));
#12087=DIRECTION('ref_axis',(-1.,-7.22448690174171E-14,0.));
#12088=DIRECTION('center_axis',(0.,0.,1.));
#12089=DIRECTION('ref_axis',(-1.,-7.2244869017417E-14,0.));
#12090=DIRECTION('',(-1.22464679914735E-16,-8.86244235752658E-30,1.));
#12091=DIRECTION('center_axis',(0.,0.,1.));
#12092=DIRECTION('ref_axis',(-1.,-7.2244869017417E-14,0.));
#12093=DIRECTION('',(-1.22464679914735E-16,-8.86244235752658E-30,1.));
#12094=DIRECTION('center_axis',(0.,0.,1.));
#12095=DIRECTION('ref_axis',(-1.,-7.2244869017417E-14,0.));
#12096=DIRECTION('',(-1.22464679914735E-16,-8.86244235752658E-30,1.));
#12097=DIRECTION('center_axis',(0.,0.,1.));
#12098=DIRECTION('ref_axis',(-1.,-7.2244869017417E-14,0.));
#12099=DIRECTION('',(-1.22464679914735E-16,-8.86244235752658E-30,1.));
#12100=DIRECTION('center_axis',(0.,0.,1.));
#12101=DIRECTION('ref_axis',(-1.,-7.2244869017417E-14,0.));
#12102=DIRECTION('',(-1.22464679914735E-16,-8.86244235752658E-30,1.));
#12103=DIRECTION('center_axis',(0.,0.,1.));
#12104=DIRECTION('ref_axis',(-1.,-7.2244869017417E-14,0.));
#12105=DIRECTION('',(-1.22464679914735E-16,-8.86244235752658E-30,1.));
#12106=DIRECTION('center_axis',(0.,0.,1.));
#12107=DIRECTION('ref_axis',(-1.,-7.2244869017417E-14,0.));
#12108=DIRECTION('',(-1.22464679914735E-16,-8.86244235752658E-30,1.));
#12109=DIRECTION('center_axis',(0.,0.,1.));
#12110=DIRECTION('ref_axis',(-1.,-7.2244869017417E-14,0.));
#12111=DIRECTION('',(-1.22464679914735E-16,-8.86244235752658E-30,1.));
#12112=DIRECTION('center_axis',(0.,0.,1.));
#12113=DIRECTION('ref_axis',(-1.,-7.2244869017417E-14,0.));
#12114=DIRECTION('',(-1.22464679914735E-16,-8.86244235752658E-30,1.));
#12115=DIRECTION('center_axis',(0.,0.,1.));
#12116=DIRECTION('ref_axis',(-1.,-7.2244869017417E-14,0.));
#12117=DIRECTION('',(-1.22464679914735E-16,-8.86244235752658E-30,1.));
#12118=DIRECTION('center_axis',(0.,0.,1.));
#12119=DIRECTION('ref_axis',(-1.,-7.2244869017417E-14,0.));
#12120=DIRECTION('',(-1.22464679914735E-16,-8.86244235752658E-30,1.));
#12121=DIRECTION('center_axis',(0.,0.,1.));
#12122=DIRECTION('ref_axis',(-1.,-7.2244869017417E-14,0.));
#12123=DIRECTION('',(-1.22464679914735E-16,-8.86244235752658E-30,1.));
#12124=DIRECTION('center_axis',(0.,0.,1.));
#12125=DIRECTION('ref_axis',(-1.,-7.2244869017417E-14,0.));
#12126=DIRECTION('',(-1.22464679914735E-16,-8.86244235752658E-30,1.));
#12127=DIRECTION('center_axis',(0.,0.,1.));
#12128=DIRECTION('ref_axis',(0.609168734065488,-0.79304063794805,0.));
#12129=DIRECTION('',(-1.22464679914735E-16,-8.86244235752658E-30,1.));
#12130=DIRECTION('center_axis',(0.,0.,1.));
#12131=DIRECTION('ref_axis',(-1.,-7.2244869017417E-14,0.));
#12132=DIRECTION('center_axis',(0.,0.,1.));
#12133=DIRECTION('ref_axis',(0.935988336829059,0.352031011872493,0.));
#12134=DIRECTION('',(0.,0.,-1.));
#12135=DIRECTION('center_axis',(0.,0.,1.));
#12136=DIRECTION('ref_axis',(1.,0.,0.));
#12137=DIRECTION('center_axis',(0.,0.,1.));
#12138=DIRECTION('ref_axis',(1.,0.,0.));
#12139=DIRECTION('',(0.,0.,-1.));
#12140=DIRECTION('center_axis',(0.,0.,1.));
#12141=DIRECTION('ref_axis',(1.,0.,0.));
#12142=DIRECTION('',(0.,0.,-1.));
#12143=DIRECTION('center_axis',(0.,0.,1.));
#12144=DIRECTION('ref_axis',(1.,0.,0.));
#12145=DIRECTION('',(0.,0.,-1.));
#12146=DIRECTION('center_axis',(0.,0.,1.));
#12147=DIRECTION('ref_axis',(1.,0.,0.));
#12148=DIRECTION('',(0.,0.,-1.));
#12149=DIRECTION('center_axis',(0.,0.,1.));
#12150=DIRECTION('ref_axis',(1.,0.,0.));
#12151=DIRECTION('',(0.,0.,-1.));
#12152=DIRECTION('center_axis',(0.,0.,1.));
#12153=DIRECTION('ref_axis',(1.,0.,0.));
#12154=DIRECTION('',(0.,0.,-1.));
#12155=DIRECTION('center_axis',(0.,0.,1.));
#12156=DIRECTION('ref_axis',(1.,0.,0.));
#12157=DIRECTION('',(0.,0.,-1.));
#12158=DIRECTION('center_axis',(0.,0.,-1.));
#12159=DIRECTION('ref_axis',(1.,0.,0.));
#12160=DIRECTION('center_axis',(0.,0.,1.));
#12161=DIRECTION('ref_axis',(1.,2.7012746630748E-14,0.));
#12162=DIRECTION('',(1.22464679914735E-16,3.32310496757901E-30,1.));
#12163=DIRECTION('center_axis',(0.,0.,-1.));
#12164=DIRECTION('ref_axis',(1.,2.7012746630748E-14,0.));
#12165=DIRECTION('center_axis',(0.,0.,1.));
#12166=DIRECTION('ref_axis',(1.,2.7012746630748E-14,0.));
#12167=DIRECTION('',(1.22464679914735E-16,3.32310496757901E-30,1.));
#12168=DIRECTION('center_axis',(0.,0.,1.));
#12169=DIRECTION('ref_axis',(1.,2.7012746630748E-14,0.));
#12170=DIRECTION('',(1.22464679914735E-16,3.32310496757901E-30,1.));
#12171=DIRECTION('center_axis',(0.,0.,1.));
#12172=DIRECTION('ref_axis',(1.,2.7012746630748E-14,0.));
#12173=DIRECTION('',(1.22464679914735E-16,3.32310496757901E-30,1.));
#12174=DIRECTION('center_axis',(0.,0.,1.));
#12175=DIRECTION('ref_axis',(1.,2.7012746630748E-14,0.));
#12176=DIRECTION('',(1.22464679914735E-16,3.32310496757901E-30,1.));
#12177=DIRECTION('center_axis',(0.,0.,1.));
#12178=DIRECTION('ref_axis',(1.,2.7012746630748E-14,0.));
#12179=DIRECTION('',(1.22464679914735E-16,3.32310496757901E-30,1.));
#12180=DIRECTION('center_axis',(0.,0.,1.));
#12181=DIRECTION('ref_axis',(1.,2.7012746630748E-14,0.));
#12182=DIRECTION('',(1.22464679914735E-16,3.32310496757901E-30,1.));
#12183=DIRECTION('center_axis',(0.,0.,1.));
#12184=DIRECTION('ref_axis',(-0.608508919018736,0.79354703419183,0.));
#12185=DIRECTION('',(1.22464679914735E-16,3.32310496757901E-30,1.));
#12186=DIRECTION('center_axis',(0.,0.,1.));
#12187=DIRECTION('ref_axis',(1.,2.7012746630748E-14,0.));
#12188=DIRECTION('center_axis',(0.,0.,1.));
#12189=DIRECTION('ref_axis',(1.,2.7012746630748E-14,0.));
#12190=DIRECTION('center_axis',(0.,0.,1.));
#12191=DIRECTION('ref_axis',(1.,0.,0.));
#12192=DIRECTION('center_axis',(0.,0.,1.));
#12193=DIRECTION('ref_axis',(1.,0.,0.));
#12194=DIRECTION('center_axis',(0.,0.,1.));
#12195=DIRECTION('ref_axis',(1.,0.,0.));
#12196=DIRECTION('center_axis',(0.,0.,1.));
#12197=DIRECTION('ref_axis',(1.,0.,0.));
#12198=DIRECTION('center_axis',(0.,0.,1.));
#12199=DIRECTION('ref_axis',(1.,0.,0.));
#12200=DIRECTION('',(0.,0.,-1.));
#12201=DIRECTION('center_axis',(0.,0.,1.));
#12202=DIRECTION('ref_axis',(1.,0.,0.));
#12203=DIRECTION('',(0.,1.,0.));
#12204=DIRECTION('',(1.,0.,0.));
#12205=DIRECTION('',(0.,1.,0.));
#12206=DIRECTION('',(-1.,0.,0.));
#12207=DIRECTION('center_axis',(0.,0.,1.));
#12208=DIRECTION('ref_axis',(1.,0.,0.));
#12209=DIRECTION('center_axis',(0.,0.,1.));
#12210=DIRECTION('ref_axis',(-1.,-7.2244869017417E-14,0.));
#12211=DIRECTION('center_axis',(0.,0.,1.));
#12212=DIRECTION('ref_axis',(-1.,0.,0.));
#12213=DIRECTION('center_axis',(0.,0.,1.));
#12214=DIRECTION('ref_axis',(1.,0.,0.));
#12215=DIRECTION('center_axis',(0.,0.,1.));
#12216=DIRECTION('ref_axis',(-1.,-7.80244585388104E-14,0.));
#12217=DIRECTION('center_axis',(0.,0.,1.));
#12218=DIRECTION('ref_axis',(-1.,0.,0.));
#12219=DIRECTION('center_axis',(0.,0.,1.));
#12220=DIRECTION('ref_axis',(1.,0.,0.));
#12221=DIRECTION('',(1.,0.,0.));
#12222=DIRECTION('center_axis',(0.,0.,1.));
#12223=DIRECTION('ref_axis',(1.,0.,0.));
#12224=DIRECTION('',(1.,0.,0.));
#12225=DIRECTION('',(1.,0.,0.));
#12226=DIRECTION('center_axis',(0.,0.,-1.));
#12227=DIRECTION('ref_axis',(-1.,0.,0.));
#12228=DIRECTION('center_axis',(0.,0.,1.));
#12229=DIRECTION('ref_axis',(1.,0.,0.));
#12230=DIRECTION('',(1.,0.,0.));
#12231=DIRECTION('center_axis',(0.,0.,1.));
#12232=DIRECTION('ref_axis',(-1.,-7.80244585388103E-14,0.));
#12233=DIRECTION('center_axis',(0.,0.,1.));
#12234=DIRECTION('ref_axis',(-1.,0.,0.));
#12235=DIRECTION('center_axis',(0.,0.,1.));
#12236=DIRECTION('ref_axis',(1.,0.,0.));
#12237=DIRECTION('',(1.,0.,0.));
#12238=DIRECTION('center_axis',(0.,0.,1.));
#12239=DIRECTION('ref_axis',(1.,0.,0.));
#12240=DIRECTION('',(1.,0.,0.));
#12241=DIRECTION('',(1.,0.,0.));
#12242=DIRECTION('center_axis',(0.,0.,-1.));
#12243=DIRECTION('ref_axis',(-1.,0.,0.));
#12244=DIRECTION('center_axis',(0.,0.,1.));
#12245=DIRECTION('ref_axis',(1.,0.,0.));
#12246=DIRECTION('',(1.,0.,0.));
#12247=DIRECTION('center_axis',(0.,0.,1.));
#12248=DIRECTION('ref_axis',(-1.,-7.80244585388103E-14,0.));
#12249=DIRECTION('center_axis',(0.,0.,1.));
#12250=DIRECTION('ref_axis',(-1.,0.,0.));
#12251=DIRECTION('center_axis',(0.,0.,1.));
#12252=DIRECTION('ref_axis',(-1.,0.,0.));
#12253=DIRECTION('center_axis',(0.,0.,1.));
#12254=DIRECTION('ref_axis',(-1.,0.,0.));
#12255=DIRECTION('center_axis',(0.,0.,1.));
#12256=DIRECTION('ref_axis',(-1.,0.,0.));
#12257=DIRECTION('center_axis',(0.,0.,1.));
#12258=DIRECTION('ref_axis',(-1.,0.,0.));
#12259=DIRECTION('center_axis',(0.,0.,1.));
#12260=DIRECTION('ref_axis',(1.,0.,0.));
#12261=DIRECTION('center_axis',(0.,0.,-1.));
#12262=DIRECTION('ref_axis',(1.,-8.21286773296138E-14,0.));
#12263=DIRECTION('center_axis',(0.,0.,-1.));
#12264=DIRECTION('ref_axis',(1.,0.,0.));
#12265=DIRECTION('center_axis',(0.,0.,1.));
#12266=DIRECTION('ref_axis',(1.,0.,0.));
#12267=DIRECTION('center_axis',(0.,0.,-1.));
#12268=DIRECTION('ref_axis',(1.,-8.21286773296134E-14,0.));
#12269=DIRECTION('center_axis',(0.,0.,-1.));
#12270=DIRECTION('ref_axis',(1.,0.,0.));
#12271=DIRECTION('center_axis',(0.,0.,1.));
#12272=DIRECTION('ref_axis',(1.,0.,0.));
#12273=DIRECTION('center_axis',(0.,0.,-1.));
#12274=DIRECTION('ref_axis',(1.,-6.48384294707476E-14,0.));
#12275=DIRECTION('center_axis',(0.,0.,-1.));
#12276=DIRECTION('ref_axis',(1.,0.,0.));
#12277=DIRECTION('center_axis',(0.,0.,1.));
#12278=DIRECTION('ref_axis',(1.,0.,0.));
#12279=DIRECTION('center_axis',(0.,0.,-1.));
#12280=DIRECTION('ref_axis',(1.,-7.34835534001804E-14,0.));
#12281=DIRECTION('center_axis',(0.,0.,-1.));
#12282=DIRECTION('ref_axis',(1.,0.,0.));
#12283=DIRECTION('center_axis',(0.,0.,-1.));
#12284=DIRECTION('ref_axis',(1.,0.,0.));
#12285=DIRECTION('center_axis',(0.,0.,-1.));
#12286=DIRECTION('ref_axis',(1.,0.,0.));
#12287=DIRECTION('center_axis',(0.,0.,-1.));
#12288=DIRECTION('ref_axis',(1.,0.,0.));
#12289=DIRECTION('center_axis',(0.,0.,-1.));
#12290=DIRECTION('ref_axis',(1.,0.,0.));
#12291=DIRECTION('center_axis',(-1.,0.,0.));
#12292=DIRECTION('ref_axis',(0.,1.,0.));
#12293=DIRECTION('center_axis',(-1.,0.,0.));
#12294=DIRECTION('ref_axis',(0.,1.,0.));
#12295=DIRECTION('',(-1.,0.,0.));
#12296=DIRECTION('center_axis',(1.,0.,0.));
#12297=DIRECTION('ref_axis',(0.,1.,0.));
#12298=DIRECTION('center_axis',(-1.,0.,0.));
#12299=DIRECTION('ref_axis',(0.,1.,0.));
#12300=DIRECTION('center_axis',(-1.,0.,0.));
#12301=DIRECTION('ref_axis',(0.,1.,0.));
#12302=DIRECTION('',(-1.,0.,0.));
#12303=DIRECTION('center_axis',(1.,0.,0.));
#12304=DIRECTION('ref_axis',(0.,1.,0.));
#12305=DIRECTION('center_axis',(-1.,0.,0.));
#12306=DIRECTION('ref_axis',(0.,1.,0.));
#12307=DIRECTION('center_axis',(-1.,0.,0.));
#12308=DIRECTION('ref_axis',(0.,1.,0.));
#12309=DIRECTION('',(-1.,0.,0.));
#12310=DIRECTION('center_axis',(1.,0.,0.));
#12311=DIRECTION('ref_axis',(0.,1.,0.));
#12312=DIRECTION('center_axis',(-1.,0.,0.));
#12313=DIRECTION('ref_axis',(0.,1.,0.));
#12314=DIRECTION('center_axis',(-1.,0.,0.));
#12315=DIRECTION('ref_axis',(0.,1.,0.));
#12316=DIRECTION('',(-1.,0.,0.));
#12317=DIRECTION('center_axis',(1.,0.,0.));
#12318=DIRECTION('ref_axis',(0.,1.,0.));
#12319=DIRECTION('center_axis',(-1.,0.,0.));
#12320=DIRECTION('ref_axis',(0.,1.,0.));
#12321=DIRECTION('center_axis',(-1.,0.,0.));
#12322=DIRECTION('ref_axis',(0.,1.,0.));
#12323=DIRECTION('',(-1.,0.,0.));
#12324=DIRECTION('center_axis',(1.,0.,0.));
#12325=DIRECTION('ref_axis',(0.,1.,0.));
#12326=DIRECTION('center_axis',(-1.,0.,0.));
#12327=DIRECTION('ref_axis',(0.,1.,0.));
#12328=DIRECTION('center_axis',(-1.,0.,0.));
#12329=DIRECTION('ref_axis',(0.,1.,0.));
#12330=DIRECTION('',(-1.,0.,0.));
#12331=DIRECTION('center_axis',(1.,0.,0.));
#12332=DIRECTION('ref_axis',(0.,1.,0.));
#12333=DIRECTION('center_axis',(-1.,0.,0.));
#12334=DIRECTION('ref_axis',(0.,1.,0.));
#12335=DIRECTION('center_axis',(-1.,0.,0.));
#12336=DIRECTION('ref_axis',(0.,1.,0.));
#12337=DIRECTION('',(-1.,0.,0.));
#12338=DIRECTION('center_axis',(1.,0.,0.));
#12339=DIRECTION('ref_axis',(0.,1.,0.));
#12340=DIRECTION('center_axis',(-1.,0.,0.));
#12341=DIRECTION('ref_axis',(0.,1.,0.));
#12342=DIRECTION('center_axis',(-1.,0.,0.));
#12343=DIRECTION('ref_axis',(0.,1.,0.));
#12344=DIRECTION('',(-1.,0.,0.));
#12345=DIRECTION('center_axis',(1.,0.,0.));
#12346=DIRECTION('ref_axis',(0.,1.,0.));
#12347=DIRECTION('center_axis',(-1.,0.,0.));
#12348=DIRECTION('ref_axis',(0.,3.3690166589284E-15,1.));
#12349=DIRECTION('center_axis',(-1.,0.,0.));
#12350=DIRECTION('ref_axis',(0.,1.,0.));
#12351=DIRECTION('',(-1.,0.,0.));
#12352=DIRECTION('',(-1.,0.,0.));
#12353=DIRECTION('center_axis',(1.,0.,0.));
#12354=DIRECTION('ref_axis',(0.,1.,0.));
#12355=DIRECTION('center_axis',(-1.,0.,0.));
#12356=DIRECTION('ref_axis',(0.,1.,0.));
#12357=DIRECTION('center_axis',(-1.,0.,0.));
#12358=DIRECTION('ref_axis',(0.,1.,0.));
#12359=DIRECTION('',(-1.,0.,0.));
#12360=DIRECTION('center_axis',(1.,0.,0.));
#12361=DIRECTION('ref_axis',(0.,1.,0.));
#12362=DIRECTION('center_axis',(-1.,0.,0.));
#12363=DIRECTION('ref_axis',(0.,1.,0.));
#12364=DIRECTION('center_axis',(-1.,0.,0.));
#12365=DIRECTION('ref_axis',(0.,1.,0.));
#12366=DIRECTION('',(-1.,0.,0.));
#12367=DIRECTION('center_axis',(1.,0.,0.));
#12368=DIRECTION('ref_axis',(0.,1.,0.));
#12369=DIRECTION('center_axis',(-1.,0.,0.));
#12370=DIRECTION('ref_axis',(0.,1.,0.));
#12371=DIRECTION('center_axis',(-1.,0.,0.));
#12372=DIRECTION('ref_axis',(0.,1.,0.));
#12373=DIRECTION('',(-1.,0.,0.));
#12374=DIRECTION('center_axis',(1.,0.,0.));
#12375=DIRECTION('ref_axis',(0.,1.,0.));
#12376=DIRECTION('center_axis',(-1.,0.,0.));
#12377=DIRECTION('ref_axis',(0.,1.,0.));
#12378=DIRECTION('center_axis',(-1.,0.,0.));
#12379=DIRECTION('ref_axis',(0.,1.,0.));
#12380=DIRECTION('',(-1.,0.,0.));
#12381=DIRECTION('center_axis',(1.,0.,0.));
#12382=DIRECTION('ref_axis',(0.,1.,0.));
#12383=DIRECTION('center_axis',(-1.,0.,0.));
#12384=DIRECTION('ref_axis',(0.,1.,0.));
#12385=DIRECTION('center_axis',(-1.,0.,0.));
#12386=DIRECTION('ref_axis',(0.,1.,0.));
#12387=DIRECTION('',(-1.,0.,0.));
#12388=DIRECTION('center_axis',(1.,0.,0.));
#12389=DIRECTION('ref_axis',(0.,1.,0.));
#12390=DIRECTION('center_axis',(-1.,0.,0.));
#12391=DIRECTION('ref_axis',(0.,1.,0.));
#12392=DIRECTION('center_axis',(-1.,0.,0.));
#12393=DIRECTION('ref_axis',(0.,1.,0.));
#12394=DIRECTION('',(-1.,0.,0.));
#12395=DIRECTION('center_axis',(1.,0.,0.));
#12396=DIRECTION('ref_axis',(0.,1.,0.));
#12397=DIRECTION('center_axis',(-1.,0.,0.));
#12398=DIRECTION('ref_axis',(0.,1.,0.));
#12399=DIRECTION('center_axis',(-1.,0.,0.));
#12400=DIRECTION('ref_axis',(0.,1.,0.));
#12401=DIRECTION('',(-1.,0.,0.));
#12402=DIRECTION('center_axis',(1.,0.,0.));
#12403=DIRECTION('ref_axis',(0.,1.,0.));
#12404=DIRECTION('center_axis',(-1.,0.,0.));
#12405=DIRECTION('ref_axis',(0.,-3.7364106986726E-15,1.));
#12406=DIRECTION('center_axis',(-1.,0.,0.));
#12407=DIRECTION('ref_axis',(0.,1.,0.));
#12408=DIRECTION('',(-1.,0.,0.));
#12409=DIRECTION('',(-1.,0.,0.));
#12410=DIRECTION('center_axis',(1.,0.,0.));
#12411=DIRECTION('ref_axis',(0.,1.,0.));
#12412=DIRECTION('center_axis',(-1.,0.,0.));
#12413=DIRECTION('ref_axis',(0.,1.,0.));
#12414=DIRECTION('center_axis',(-1.,0.,0.));
#12415=DIRECTION('ref_axis',(0.,1.,0.));
#12416=DIRECTION('',(-1.,0.,0.));
#12417=DIRECTION('center_axis',(1.,0.,0.));
#12418=DIRECTION('ref_axis',(0.,1.,0.));
#12419=DIRECTION('center_axis',(0.,-1.,0.));
#12420=DIRECTION('ref_axis',(-1.,0.,0.));
#12421=DIRECTION('',(-1.,0.,0.));
#12422=DIRECTION('',(0.,0.,-1.));
#12423=DIRECTION('',(-1.,0.,0.));
#12424=DIRECTION('',(0.,0.,-1.));
#12425=DIRECTION('center_axis',(1.,0.,0.));
#12426=DIRECTION('ref_axis',(0.,-1.,0.));
#12427=DIRECTION('',(0.,-1.,0.));
#12428=DIRECTION('',(0.,0.,-1.));
#12429=DIRECTION('',(0.,-1.,0.));
#12430=DIRECTION('center_axis',(0.,1.,0.));
#12431=DIRECTION('ref_axis',(1.,0.,0.));
#12432=DIRECTION('',(1.,0.,0.));
#12433=DIRECTION('',(0.,0.,-1.));
#12434=DIRECTION('',(1.,0.,0.));
#12435=DIRECTION('center_axis',(-1.,0.,0.));
#12436=DIRECTION('ref_axis',(0.,1.,0.));
#12437=DIRECTION('',(0.,1.,0.));
#12438=DIRECTION('',(0.,1.,0.));
#12439=DIRECTION('center_axis',(0.,0.,-1.));
#12440=DIRECTION('ref_axis',(-1.,0.,0.));
#12441=DIRECTION('center_axis',(0.,1.,0.));
#12442=DIRECTION('ref_axis',(-1.,0.,0.));
#12443=DIRECTION('',(0.,0.,1.));
#12444=DIRECTION('',(1.,0.,0.));
#12445=DIRECTION('',(0.,0.,-1.));
#12446=DIRECTION('center_axis',(1.,0.,0.));
#12447=DIRECTION('ref_axis',(0.,1.,0.));
#12448=DIRECTION('',(0.,1.,0.));
#12449=DIRECTION('',(0.,0.,1.));
#12450=DIRECTION('center_axis',(0.,-1.,0.));
#12451=DIRECTION('ref_axis',(1.,0.,0.));
#12452=DIRECTION('',(-1.,0.,0.));
#12453=DIRECTION('',(0.,0.,-1.));
#12454=DIRECTION('center_axis',(-1.,0.,0.));
#12455=DIRECTION('ref_axis',(0.,-1.,0.));
#12456=DIRECTION('',(0.,1.,0.));
#12457=DIRECTION('center_axis',(0.,0.,1.));
#12458=DIRECTION('ref_axis',(1.,0.,0.));
#13449=CARTESIAN_POINT('',(0.,0.,0.));
#13450=CARTESIAN_POINT('Origin',(-20.,-66.,30.));
#13451=CARTESIAN_POINT('',(-21.6686463164215,-66.0003916927953,25.7714803633902));
#13452=CARTESIAN_POINT('',(-21.6665334720122,-65.9985218171631,25.5785196366098));
#13453=CARTESIAN_POINT('',(-21.666,-66.,30.));
#13454=CARTESIAN_POINT('',(-20.7699020406705,-67.4774325188554,25.));
#13455=CARTESIAN_POINT('Ctrl Pts',(-21.6665334720122,-65.9985218171631,
25.5785196366098));
#13456=CARTESIAN_POINT('Ctrl Pts',(-21.6675831226457,-65.8847144663257,
25.5709016210591));
#13457=CARTESIAN_POINT('Ctrl Pts',(-21.6569164284924,-65.7711020348436,
25.5632836055085));
#13458=CARTESIAN_POINT('Ctrl Pts',(-21.6338086330613,-65.6600764397889,
25.5556655899578));
#13459=CARTESIAN_POINT('Ctrl Pts',(-21.5214416026058,-65.1201886578488,
25.5186212172939));
#13460=CARTESIAN_POINT('Ctrl Pts',(-21.1148901954472,-64.6414696458604,
25.4815768446301));
#13461=CARTESIAN_POINT('Ctrl Pts',(-20.6004654912914,-64.4430320689214,
25.4445324719662));
#13462=CARTESIAN_POINT('Ctrl Pts',(-20.0860407871355,-64.2445944919823,
25.4074880993024));
#13463=CARTESIAN_POINT('Ctrl Pts',(-19.4637427859824,-64.3264383500926,
25.3704437266385));
#13464=CARTESIAN_POINT('Ctrl Pts',(-19.0178170303308,-64.6510266230413,
25.3333993539747));
#13465=CARTESIAN_POINT('Ctrl Pts',(-18.5718912746792,-64.9756148959899,
25.2963549813108));
#13466=CARTESIAN_POINT('Ctrl Pts',(-18.3023377645291,-65.5429475837768,
25.259310608647));
#13467=CARTESIAN_POINT('Ctrl Pts',(-18.3335864161634,-66.0935813146395,
25.2222662359831));
#13468=CARTESIAN_POINT('Ctrl Pts',(-18.3648350677978,-66.6442150455023,
25.1852218633193));
#13469=CARTESIAN_POINT('Ctrl Pts',(-18.6968858812165,-67.1781498194408,
25.1481774906554));
#13470=CARTESIAN_POINT('Ctrl Pts',(-19.1753375331628,-67.4504541256366,
25.1111331179916));
#13471=CARTESIAN_POINT('Ctrl Pts',(-19.653789185109,-67.7227584318323,25.0740887453277));
#13472=CARTESIAN_POINT('Ctrl Pts',(-20.2786416755828,-67.7334322702853,
25.0370443726639));
#13473=CARTESIAN_POINT('Ctrl Pts',(-20.7699020406704,-67.4774325188554,
25.));
#13474=CARTESIAN_POINT('',(-21.3370260554501,-65.0009970088504,25.));
#13475=CARTESIAN_POINT('Origin',(-20.,-66.,25.));
#13476=CARTESIAN_POINT('',(-21.6645215840113,-66.0012211302689,25.0714803633902));
#13477=CARTESIAN_POINT('Ctrl Pts',(-21.3370274731509,-65.0009958365549,
25.));
#13478=CARTESIAN_POINT('Ctrl Pts',(-21.5489927408181,-65.2854500014782,
25.0238267877967));
#13479=CARTESIAN_POINT('Ctrl Pts',(-21.6621689009854,-65.6440627477619,
25.0476535755935));
#13480=CARTESIAN_POINT('Ctrl Pts',(-21.6645215840113,-66.0012211302689,
25.0714803633902));
#13481=CARTESIAN_POINT('',(-21.666,-66.,24.));
#13482=CARTESIAN_POINT('',(-21.666,-66.,30.));
#13483=CARTESIAN_POINT('Origin',(-20.,-66.,24.));
#13484=CARTESIAN_POINT('Ctrl Pts',(-21.6645215840113,-66.0012211302689,
25.0714803633902));
#13485=CARTESIAN_POINT('Ctrl Pts',(-21.6657549943118,-66.188463875268,25.0839717212025));
#13486=CARTESIAN_POINT('Ctrl Pts',(-21.6365290935638,-66.3753068952287,
25.0964630790149));
#13487=CARTESIAN_POINT('Ctrl Pts',(-21.5751098549791,-66.5508551556528,
25.1089544368272));
#13488=CARTESIAN_POINT('Ctrl Pts',(-21.3929649515153,-67.0714611039685,
25.1459988094911));
#13489=CARTESIAN_POINT('Ctrl Pts',(-20.9276865865547,-67.492732078676,25.1830431821549));
#13490=CARTESIAN_POINT('Ctrl Pts',(-20.3917115249228,-67.6221189802502,
25.2200875548188));
#13491=CARTESIAN_POINT('Ctrl Pts',(-19.8557364632908,-67.7515058818244,
25.2571319274826));
#13492=CARTESIAN_POINT('Ctrl Pts',(-19.2490647049875,-67.5890087102653,
25.2941763001465));
#13493=CARTESIAN_POINT('Ctrl Pts',(-18.8495628612421,-67.2088726273032,
25.3312206728103));
#13494=CARTESIAN_POINT('Ctrl Pts',(-18.4500610174968,-66.8287365443411,
25.3682650454742));
#13495=CARTESIAN_POINT('Ctrl Pts',(-18.2577290883093,-66.230961549976,25.405309418138));
#13496=CARTESIAN_POINT('Ctrl Pts',(-18.3604608102357,-65.6891597965066,
25.4423537908019));
#13497=CARTESIAN_POINT('Ctrl Pts',(-18.4631925321622,-65.1473580430372,
25.4793981634657));
#13498=CARTESIAN_POINT('Ctrl Pts',(-18.8609879052027,-64.6615295304635,
25.5164425361296));
#13499=CARTESIAN_POINT('Ctrl Pts',(-19.3718686901783,-64.453969580922,25.5534869087934));
#13500=CARTESIAN_POINT('Ctrl Pts',(-19.8827494751539,-64.2464096313805,
25.5905312814573));
#13501=CARTESIAN_POINT('Ctrl Pts',(-20.5067156720646,-64.3171182448712,
25.6275756541212));
#13502=CARTESIAN_POINT('Ctrl Pts',(-20.9581975997172,-64.6337524970504,
25.664620026785));
#13503=CARTESIAN_POINT('Ctrl Pts',(-21.3923212132001,-64.9382129799389,
25.7002401389867));
#13504=CARTESIAN_POINT('Ctrl Pts',(-21.6669687399304,-65.4700522183443,
25.7358602511885));
#13505=CARTESIAN_POINT('Ctrl Pts',(-21.6686463164215,-66.0003916927953,
25.7714803633902));
#13506=CARTESIAN_POINT('Origin',(-20.,-66.,30.));
#13507=CARTESIAN_POINT('',(-21.6655732814929,-65.9984874577248,26.4714803633902));
#13508=CARTESIAN_POINT('',(-21.6632974926259,-66.0000402088307,26.2785196366098));
#13509=CARTESIAN_POINT('',(-21.666,-66.,30.));
#13510=CARTESIAN_POINT('Ctrl Pts',(-21.6632974926259,-66.0000402088307,
26.2785196366098));
#13511=CARTESIAN_POINT('Ctrl Pts',(-21.6632374792194,-65.7195428093862,
26.2598345237089));
#13512=CARTESIAN_POINT('Ctrl Pts',(-21.5960668066056,-65.4390182789714,
26.241149410808));
#13513=CARTESIAN_POINT('Ctrl Pts',(-21.4619469193729,-65.1953423902613,
26.2224642979072));
#13514=CARTESIAN_POINT('Ctrl Pts',(-21.1960460864137,-64.7122401217089,
26.1854199252433));
#13515=CARTESIAN_POINT('Ctrl Pts',(-20.6669981929564,-64.3739731854776,
26.1483755525794));
#13516=CARTESIAN_POINT('Ctrl Pts',(-20.1169101847181,-64.3353398464244,
26.1113311799156));
#13517=CARTESIAN_POINT('Ctrl Pts',(-19.5668221764797,-64.2967065073713,
26.0742868072517));
#13518=CARTESIAN_POINT('Ctrl Pts',(-18.9956940534603,-64.5577067654963,
26.0372424345879));
#13519=CARTESIAN_POINT('Ctrl Pts',(-18.6648768742022,-64.9989004546789,
26.000198061924));
#13520=CARTESIAN_POINT('Ctrl Pts',(-18.3340596949442,-65.4400941438616,
25.9631536892602));
#13521=CARTESIAN_POINT('Ctrl Pts',(-18.2435534594475,-66.0614812641019,
25.9261093165963));
#13522=CARTESIAN_POINT('Ctrl Pts',(-18.4347923709177,-66.5787054554592,
25.8890649439325));
#13523=CARTESIAN_POINT('Ctrl Pts',(-18.6260312823879,-67.0959296468164,
25.8520205712686));
#13524=CARTESIAN_POINT('Ctrl Pts',(-19.099015340825,-67.5089909092908,25.8149761986048));
#13525=CARTESIAN_POINT('Ctrl Pts',(-19.6372642986701,-67.6288590661524,
25.7779318259409));
#13526=CARTESIAN_POINT('Ctrl Pts',(-20.1755132565153,-67.7487272230141,
25.7408874532771));
#13527=CARTESIAN_POINT('Ctrl Pts',(-20.7790271137684,-67.5754022742632,
25.7038430806132));
#13528=CARTESIAN_POINT('Ctrl Pts',(-21.1716927155188,-67.1882115239419,
25.6667987079494));
#13529=CARTESIAN_POINT('Ctrl Pts',(-21.4836083289379,-66.880644882356,25.6373723508362));
#13530=CARTESIAN_POINT('Ctrl Pts',(-21.6624789522782,-66.4381291828313,
25.607945993723));
#13531=CARTESIAN_POINT('Ctrl Pts',(-21.6665334720122,-65.9985218171631,
25.5785196366098));
#13532=CARTESIAN_POINT('Ctrl Pts',(-21.6686463164215,-66.0003916927953,
25.7714803633902));
#13533=CARTESIAN_POINT('Ctrl Pts',(-21.6687133938595,-66.0215971718989,
25.7729046238523));
#13534=CARTESIAN_POINT('Ctrl Pts',(-21.6683440528391,-66.0428002532123,
25.7743288843144));
#13535=CARTESIAN_POINT('Ctrl Pts',(-21.66753103807,-66.0639863052831,25.7757531447765));
#13536=CARTESIAN_POINT('Ctrl Pts',(-21.6463848903759,-66.6150259704687,
25.8127975174404));
#13537=CARTESIAN_POINT('Ctrl Pts',(-21.3250949365933,-67.1545454099721,
25.8498418901043));
#13538=CARTESIAN_POINT('Ctrl Pts',(-20.8506821176263,-67.4356536157318,
25.8868862627681));
#13539=CARTESIAN_POINT('Ctrl Pts',(-20.3762692986592,-67.7167618214914,
25.923930635432));
#13540=CARTESIAN_POINT('Ctrl Pts',(-19.7487336145077,-67.7394587935073,
25.9609750080958));
#13541=CARTESIAN_POINT('Ctrl Pts',(-19.2552515883631,-67.4933560924105,
25.9980193807597));
#13542=CARTESIAN_POINT('Ctrl Pts',(-18.7617695622185,-67.2472533913136,
26.0350637534235));
#13543=CARTESIAN_POINT('Ctrl Pts',(-18.4023411940809,-66.732351017104,26.0721081260874));
#13544=CARTESIAN_POINT('Ctrl Pts',(-18.3414460505489,-66.1842793614378,
26.1091524987512));
#13545=CARTESIAN_POINT('Ctrl Pts',(-18.2805509070169,-65.6362077057716,
26.1461968714151));
#13546=CARTESIAN_POINT('Ctrl Pts',(-18.5181889880905,-65.0549667686488,
26.1832412440789));
#13547=CARTESIAN_POINT('Ctrl Pts',(-18.9456133982649,-64.7065433741402,
26.2202856167428));
#13548=CARTESIAN_POINT('Ctrl Pts',(-19.3730378084393,-64.3581199796316,
26.2573299894066));
#13549=CARTESIAN_POINT('Ctrl Pts',(-19.9902485477144,-64.2425141277373,
26.2943743620705));
#13550=CARTESIAN_POINT('Ctrl Pts',(-20.5147973501738,-64.4126295658445,
26.3314187347344));
#13551=CARTESIAN_POINT('Ctrl Pts',(-21.0393461526331,-64.5827450039518,
26.3684631073982));
#13552=CARTESIAN_POINT('Ctrl Pts',(-21.4712330182765,-65.0385817320607,
26.4055074800621));
#13553=CARTESIAN_POINT('Ctrl Pts',(-21.6128182612061,-65.5715397750152,
26.4425518527259));
#13554=CARTESIAN_POINT('Ctrl Pts',(-21.649673613454,-65.7102714394179,26.452194689614));
#13555=CARTESIAN_POINT('Ctrl Pts',(-21.6668585011999,-65.8542287449032,
26.4618375265021));
#13556=CARTESIAN_POINT('Ctrl Pts',(-21.6655732814929,-65.9984874577248,
26.4714803633902));
#13557=CARTESIAN_POINT('Origin',(-20.,-66.,30.));
#13558=CARTESIAN_POINT('',(-21.6634529485587,-66.0005281517982,27.1714803633902));
#13559=CARTESIAN_POINT('',(-21.6666334680486,-66.0014645810993,26.9785196366098));
#13560=CARTESIAN_POINT('',(-21.666,-66.,30.));
#13561=CARTESIAN_POINT('Ctrl Pts',(-21.6666334680486,-66.0014645810993,
26.9785196366098));
#13562=CARTESIAN_POINT('Ctrl Pts',(-21.6625547837736,-65.5570900696918,
26.9487674263587));
#13563=CARTESIAN_POINT('Ctrl Pts',(-21.4793116087742,-65.1097459698003,
26.9190152161076));
#13564=CARTESIAN_POINT('Ctrl Pts',(-21.1612403596529,-64.8015501984858,
26.8892630058565));
#13565=CARTESIAN_POINT('Ctrl Pts',(-20.765210962621,-64.417816724245,26.8522186331926));
#13566=CARTESIAN_POINT('Ctrl Pts',(-20.1601622836896,-64.2498000723804,
26.8151742605288));
#13567=CARTESIAN_POINT('Ctrl Pts',(-19.6229765727187,-64.3743879797908,
26.7781298878649));
#13568=CARTESIAN_POINT('Ctrl Pts',(-19.0857908617477,-64.4989758872013,
26.7410855152011));
#13569=CARTESIAN_POINT('Ctrl Pts',(-18.6164681187371,-64.9161683538868,
26.7040411425372));
#13570=CARTESIAN_POINT('Ctrl Pts',(-18.4297795332059,-65.4350498759485,
26.6669967698734));
#13571=CARTESIAN_POINT('Ctrl Pts',(-18.2430909476747,-65.9539313980101,
26.6299523972095));
#13572=CARTESIAN_POINT('Ctrl Pts',(-18.3390365196228,-66.5745019754479,
26.5929080245457));
#13573=CARTESIAN_POINT('Ctrl Pts',(-18.6737099340405,-67.0127763409396,
26.5558636518818));
#13574=CARTESIAN_POINT('Ctrl Pts',(-19.0083833484582,-67.4510507064314,
26.518819279218));
#13575=CARTESIAN_POINT('Ctrl Pts',(-19.5817846053455,-67.7070288599771,
26.4817749065541));
#13576=CARTESIAN_POINT('Ctrl Pts',(-20.1315134729593,-67.663570077923,26.4447305338903));
#13577=CARTESIAN_POINT('Ctrl Pts',(-20.6812423405732,-67.6201112958688,
26.4076861612264));
#13578=CARTESIAN_POINT('Ctrl Pts',(-21.2072988189137,-67.2772155782147,
26.3706417885626));
#13579=CARTESIAN_POINT('Ctrl Pts',(-21.4689501718534,-66.7917989189509,
26.3335974158987));
#13580=CARTESIAN_POINT('Ctrl Pts',(-21.5986250674048,-66.5512255227818,
26.3152381561357));
#13581=CARTESIAN_POINT('Ctrl Pts',(-21.6633564594476,-66.275645962275,26.2968788963728));
#13582=CARTESIAN_POINT('Ctrl Pts',(-21.6632974926259,-66.0000402088307,
26.2785196366098));
#13583=CARTESIAN_POINT('Ctrl Pts',(-21.6655732814929,-65.9984874577248,
26.4714803633902));
#13584=CARTESIAN_POINT('Ctrl Pts',(-21.6619211411332,-66.4084197552654,
26.498881899166));
#13585=CARTESIAN_POINT('Ctrl Pts',(-21.5091236946976,-66.8207859038016,
26.5262834349417));
#13586=CARTESIAN_POINT('Ctrl Pts',(-21.2347245419387,-67.1225935870211,
26.5536849707175));
#13587=CARTESIAN_POINT('Ctrl Pts',(-20.8637619595262,-67.5306099982724,
26.5907293433813));
#13588=CARTESIAN_POINT('Ctrl Pts',(-20.2705531744855,-67.7365634629749,
26.6277737160452));
#13589=CARTESIAN_POINT('Ctrl Pts',(-19.7265622622826,-67.6462055929746,
26.664818088709));
#13590=CARTESIAN_POINT('Ctrl Pts',(-19.1825713500797,-67.5558477229742,
26.7018624613729));
#13591=CARTESIAN_POINT('Ctrl Pts',(-18.6877983107146,-67.1691785182711,
26.7389068340367));
#13592=CARTESIAN_POINT('Ctrl Pts',(-18.4686609933462,-66.6631454313498,
26.7759512067006));
#13593=CARTESIAN_POINT('Ctrl Pts',(-18.2495236759778,-66.1571123444284,
26.8129955793644));
#13594=CARTESIAN_POINT('Ctrl Pts',(-18.306022080606,-65.5317153752889,26.8500399520283));
#13595=CARTESIAN_POINT('Ctrl Pts',(-18.6123014407894,-65.0731484772605,
26.8870843246922));
#13596=CARTESIAN_POINT('Ctrl Pts',(-18.9185808009729,-64.6145815792321,
26.924128697356));
#13597=CARTESIAN_POINT('Ctrl Pts',(-19.4746411167116,-64.3228447523148,
26.9611730700199));
#13598=CARTESIAN_POINT('Ctrl Pts',(-20.0260182366421,-64.3314425135629,
26.9982174426837));
#13599=CARTESIAN_POINT('Ctrl Pts',(-20.5773953565726,-64.3400402748111,
27.0352618153476));
#13600=CARTESIAN_POINT('Ctrl Pts',(-21.124089280695,-64.6489726242249,27.0723061880114));
#13601=CARTESIAN_POINT('Ctrl Pts',(-21.4159221143717,-65.1168660371111,
27.1093505606753));
#13602=CARTESIAN_POINT('Ctrl Pts',(-21.5790734477433,-65.3784453571158,
27.1300604949136));
#13603=CARTESIAN_POINT('Ctrl Pts',(-21.6625691491406,-65.6897072078986,
27.1507704291519));
#13604=CARTESIAN_POINT('Ctrl Pts',(-21.6634529485587,-66.0005281517982,
27.1714803633902));
#13605=CARTESIAN_POINT('Origin',(-20.,-66.,30.));
#13606=CARTESIAN_POINT('',(-21.667507987647,-66.0012330299472,27.8714803633902));
#13607=CARTESIAN_POINT('',(-21.668061697955,-65.9990409238289,27.6785196366098));
#13608=CARTESIAN_POINT('',(-21.666,-66.,30.));
#13609=CARTESIAN_POINT('Ctrl Pts',(-21.668061697955,-65.9990409238289,27.6785196366098));
#13610=CARTESIAN_POINT('Ctrl Pts',(-21.6684477978651,-65.9427845343911,
27.6747447016723));
#13611=CARTESIAN_POINT('Ctrl Pts',(-21.6658484802025,-65.8865642454305,
27.6709697667349));
#13612=CARTESIAN_POINT('Ctrl Pts',(-21.6601461398808,-65.8306604734177,
27.6671948317974));
#13613=CARTESIAN_POINT('Ctrl Pts',(-21.6041876602164,-65.2820628954279,
27.6301504591336));
#13614=CARTESIAN_POINT('Ctrl Pts',(-21.2494086074079,-64.7639458475939,
27.5931060864697));
#13615=CARTESIAN_POINT('Ctrl Pts',(-20.7581628574682,-64.5134098873652,
27.5560617138059));
#13616=CARTESIAN_POINT('Ctrl Pts',(-20.2669171075285,-64.2628739271364,
27.519017341142));
#13617=CARTESIAN_POINT('Ctrl Pts',(-19.6392046604576,-64.2799190545128,
27.4819729684782));
#13618=CARTESIAN_POINT('Ctrl Pts',(-19.1622790863643,-64.5567450839289,
27.4449285958143));
#13619=CARTESIAN_POINT('Ctrl Pts',(-18.6853535122711,-64.8335711133449,
27.4078842231505));
#13620=CARTESIAN_POINT('Ctrl Pts',(-18.3592148111555,-65.3701780448006,
27.3708398504866));
#13621=CARTESIAN_POINT('Ctrl Pts',(-18.3331104688645,-65.9210039858079,
27.3337954778227));
#13622=CARTESIAN_POINT('Ctrl Pts',(-18.3070061265735,-66.4718299268152,
27.2967511051589));
#13623=CARTESIAN_POINT('Ctrl Pts',(-18.580936143107,-67.0368748773742,27.259706732495));
#13624=CARTESIAN_POINT('Ctrl Pts',(-19.0295447562574,-67.3575631487953,
27.2226623598312));
#13625=CARTESIAN_POINT('Ctrl Pts',(-19.4781533694078,-67.6782514202164,
27.1856179871673));
#13626=CARTESIAN_POINT('Ctrl Pts',(-20.1014405791751,-67.7545830124997,
27.1485736145035));
#13627=CARTESIAN_POINT('Ctrl Pts',(-20.6141778837267,-67.5516270855043,
27.1115292418396));
#13628=CARTESIAN_POINT('Ctrl Pts',(-21.1269151882782,-67.3486711585089,
27.0744848691758));
#13629=CARTESIAN_POINT('Ctrl Pts',(-21.529102587614,-66.8664277122347,27.0374404965119));
#13630=CARTESIAN_POINT('Ctrl Pts',(-21.6366912297157,-66.3255808407892,
27.0003961238481));
#13631=CARTESIAN_POINT('Ctrl Pts',(-21.6578699890131,-66.2191154603979,
26.9931039614353));
#13632=CARTESIAN_POINT('Ctrl Pts',(-21.6676331392633,-66.1103792157407,
26.9858117990226));
#13633=CARTESIAN_POINT('Ctrl Pts',(-21.6666334680486,-66.0014645810993,
26.9785196366098));
#13634=CARTESIAN_POINT('Ctrl Pts',(-21.6634529485587,-66.0005281517982,
27.1714803633902));
#13635=CARTESIAN_POINT('Ctrl Pts',(-21.6641500230646,-66.2456803338898,
27.1878148018157));
#13636=CARTESIAN_POINT('Ctrl Pts',(-21.6134553249685,-66.4905582336354,
27.2041492402413));
#13637=CARTESIAN_POINT('Ctrl Pts',(-21.5099183448232,-66.7105685223684,
27.2204836786668));
#13638=CARTESIAN_POINT('Ctrl Pts',(-21.2751099983669,-67.2095231183808,
27.2575280513307));
#13639=CARTESIAN_POINT('Ctrl Pts',(-20.7685215622234,-67.580577834047,27.2945724239945));
#13640=CARTESIAN_POINT('Ctrl Pts',(-20.2219778753094,-67.6539307287216,
27.3316167966584));
#13641=CARTESIAN_POINT('Ctrl Pts',(-19.6754341883954,-67.7272836233961,
27.3686611693222));
#13642=CARTESIAN_POINT('Ctrl Pts',(-19.0889352507107,-67.5029346970789,
27.4057055419861));
#13643=CARTESIAN_POINT('Ctrl Pts',(-18.7308745178381,-67.0835504338329,
27.4427499146499));
#13644=CARTESIAN_POINT('Ctrl Pts',(-18.3728137849654,-66.6641661705869,
27.4797942873138));
#13645=CARTESIAN_POINT('Ctrl Pts',(-18.2431912569046,-66.049746570412,27.5168386599777));
#13646=CARTESIAN_POINT('Ctrl Pts',(-18.4013247536879,-65.5214621338897,
27.5538830326415));
#13647=CARTESIAN_POINT('Ctrl Pts',(-18.5594582504713,-64.9931776973674,
27.5909274053054));
#13648=CARTESIAN_POINT('Ctrl Pts',(-19.0053477720987,-64.5510284244976,
27.6279717779692));
#13649=CARTESIAN_POINT('Ctrl Pts',(-19.5349454983304,-64.3973505240179,
27.6650161506331));
#13650=CARTESIAN_POINT('Ctrl Pts',(-20.064543224562,-64.2436726235382,27.7020605232969));
#13651=CARTESIAN_POINT('Ctrl Pts',(-20.6778491553978,-64.3784660954486,
27.7391048959608));
#13652=CARTESIAN_POINT('Ctrl Pts',(-21.0942024272058,-64.7400467942635,
27.7761492686246));
#13653=CARTESIAN_POINT('Ctrl Pts',(-21.4513544078936,-65.0502143166643,
27.8079263002132));
#13654=CARTESIAN_POINT('Ctrl Pts',(-21.6635811543817,-65.5272604795206,
27.8397033318017));
#13655=CARTESIAN_POINT('Ctrl Pts',(-21.667507987647,-66.0012330299472,27.8714803633902));
#13656=CARTESIAN_POINT('Origin',(-20.,-66.,30.));
#13657=CARTESIAN_POINT('',(-21.6672880470512,-65.9986896255742,28.5714803633902));
#13658=CARTESIAN_POINT('',(-21.6637335962722,-65.999144500325,28.3785196366098));
#13659=CARTESIAN_POINT('',(-21.666,-66.,30.));
#13660=CARTESIAN_POINT('Ctrl Pts',(-21.6637335962722,-65.999144500325,28.3785196366098));
#13661=CARTESIAN_POINT('Ctrl Pts',(-21.6647696506054,-65.7764847271083,
28.3636776043221));
#13662=CARTESIAN_POINT('Ctrl Pts',(-21.6232171112865,-65.5541957879046,
28.3488355720345));
#13663=CARTESIAN_POINT('Ctrl Pts',(-21.5372474702476,-65.3506685773165,
28.3339935397468));
#13664=CARTESIAN_POINT('Ctrl Pts',(-21.3226750074813,-64.8426830339538,
28.2969491670829));
#13665=CARTESIAN_POINT('Ctrl Pts',(-20.8314033075768,-64.451574904792,28.2599047944191));
#13666=CARTESIAN_POINT('Ctrl Pts',(-20.2882479685347,-64.3563229666671,
28.2228604217552));
#13667=CARTESIAN_POINT('Ctrl Pts',(-19.7450926294927,-64.2610710285423,
28.1858160490913));
#13668=CARTESIAN_POINT('Ctrl Pts',(-19.1500536513131,-64.4616752814544,
28.1487716764275));
#13669=CARTESIAN_POINT('Ctrl Pts',(-18.7754325806809,-64.8663352714203,
28.1117273037637));
#13670=CARTESIAN_POINT('Ctrl Pts',(-18.4008115100487,-65.2709952613862,
28.0746829310998));
#13671=CARTESIAN_POINT('Ctrl Pts',(-18.2466083469639,-65.8797109884059,
28.037638558436));
#13672=CARTESIAN_POINT('Ctrl Pts',(-18.3833894935089,-66.4139221563812,
28.0005941857721));
#13673=CARTESIAN_POINT('Ctrl Pts',(-18.5201706400539,-66.9481333243564,
27.9635498131082));
#13674=CARTESIAN_POINT('Ctrl Pts',(-18.9479360962286,-67.4078399332872,
27.9265054404444));
#13675=CARTESIAN_POINT('Ctrl Pts',(-19.4709319710131,-67.5826711919994,
27.8894610677805));
#13676=CARTESIAN_POINT('Ctrl Pts',(-19.9939278457975,-67.7575024507116,
27.8524166951167));
#13677=CARTESIAN_POINT('Ctrl Pts',(-20.6121541391916,-67.6474583592052,
27.8153723224528));
#13678=CARTESIAN_POINT('Ctrl Pts',(-21.0426983326285,-67.3028972593792,
27.778327949789));
#13679=CARTESIAN_POINT('Ctrl Pts',(-21.429368755205,-66.9934479900496,27.7450585120626));
#13680=CARTESIAN_POINT('Ctrl Pts',(-21.6646589037003,-66.494842434616,27.7117890743362));
#13681=CARTESIAN_POINT('Ctrl Pts',(-21.668061697955,-65.9990409238289,27.6785196366098));
#13682=CARTESIAN_POINT('Ctrl Pts',(-21.667507987647,-66.0012330299472,27.8714803633902));
#13683=CARTESIAN_POINT('Ctrl Pts',(-21.668158897097,-66.0797984263558,27.8767477044656));
#13684=CARTESIAN_POINT('Ctrl Pts',(-21.6630865222461,-66.1582793716597,
27.8820150455409));
#13685=CARTESIAN_POINT('Ctrl Pts',(-21.6520022273457,-66.2359018296592,
27.8872823866162));
#13686=CARTESIAN_POINT('Ctrl Pts',(-21.5740481428971,-66.7818082405207,
27.9243267592801));
#13687=CARTESIAN_POINT('Ctrl Pts',(-21.1987393612196,-67.2852531365244,
27.9613711319439));
#13688=CARTESIAN_POINT('Ctrl Pts',(-20.6978245668292,-67.5158502255527,
27.9984155046077));
#13689=CARTESIAN_POINT('Ctrl Pts',(-20.1969097724387,-67.7464473145809,
28.0354598772716));
#13690=CARTESIAN_POINT('Ctrl Pts',(-19.5703889653353,-67.7041965966336,
28.0725042499355));
#13691=CARTESIAN_POINT('Ctrl Pts',(-19.1049703966511,-67.4084328317332,
28.1095486225993));
#13692=CARTESIAN_POINT('Ctrl Pts',(-18.6395518279668,-67.1126690668328,
28.1465929952632));
#13693=CARTESIAN_POINT('Ctrl Pts',(-18.3352354977017,-66.5633922549793,
28.183637367927));
#13694=CARTESIAN_POINT('Ctrl Pts',(-18.3312825474759,-66.0119622749373,
28.2206817405908));
#13695=CARTESIAN_POINT('Ctrl Pts',(-18.3273295972502,-65.4605322948953,
28.2577261132547));
#13696=CARTESIAN_POINT('Ctrl Pts',(-18.6237400270638,-64.9069491466648,
28.2947704859186));
#13697=CARTESIAN_POINT('Ctrl Pts',(-19.0848705909317,-64.6045433732873,
28.3318148585824));
#13698=CARTESIAN_POINT('Ctrl Pts',(-19.5460011547996,-64.3021375999098,
28.3688592312463));
#13699=CARTESIAN_POINT('Ctrl Pts',(-20.1718518527218,-64.2509092013851,
28.4059036039101));
#13700=CARTESIAN_POINT('Ctrl Pts',(-20.6760210887083,-64.4743013010429,
28.442947976574));
#13701=CARTESIAN_POINT('Ctrl Pts',(-21.1801903246949,-64.6976934007006,
28.4799923492378));
#13702=CARTESIAN_POINT('Ctrl Pts',(-21.5626780987458,-65.1957059985407,
28.5170367219017));
#13703=CARTESIAN_POINT('Ctrl Pts',(-21.6484504781688,-65.7404387289994,
28.5540810945655));
#13704=CARTESIAN_POINT('Ctrl Pts',(-21.6618792086344,-65.8257233982873,
28.5598808508404));
#13705=CARTESIAN_POINT('Ctrl Pts',(-21.6680349141495,-65.9121532615772,
28.5656806071153));
#13706=CARTESIAN_POINT('Ctrl Pts',(-21.6672880470512,-65.9986896255742,
28.5714803633902));
#13707=CARTESIAN_POINT('Origin',(-20.,-66.,30.));
#13708=CARTESIAN_POINT('',(-21.6633862072226,-65.9995968836612,29.2714803633902));
#13709=CARTESIAN_POINT('',(-21.6649409508278,-66.0014219187278,29.0785196366098));
#13710=CARTESIAN_POINT('',(-21.666,-66.,30.));
#13711=CARTESIAN_POINT('Ctrl Pts',(-21.6649409508278,-66.0014219187278,
29.0785196366098));
#13712=CARTESIAN_POINT('Ctrl Pts',(-21.6617887517993,-65.6134426418904,
29.0526105069719));
#13713=CARTESIAN_POINT('Ctrl Pts',(-21.5266091317759,-65.2234833383847,
29.026701377334));
#13714=CARTESIAN_POINT('Ctrl Pts',(-21.2788296086732,-64.9279198195793,
29.0007922476961));
#13715=CARTESIAN_POINT('Ctrl Pts',(-20.9245592367783,-64.5053288144204,
28.9637478750323));
#13716=CARTESIAN_POINT('Ctrl Pts',(-20.3401039506114,-64.2757085402715,
28.9267035023684));
#13717=CARTESIAN_POINT('Ctrl Pts',(-19.7929219910902,-64.3441377534661,
28.8896591297046));
#13718=CARTESIAN_POINT('Ctrl Pts',(-19.2457400315691,-64.4125669666608,
28.8526147570407));
#13719=CARTESIAN_POINT('Ctrl Pts',(-18.7358313986938,-64.7790456671989,
28.8155703843769));
#13720=CARTESIAN_POINT('Ctrl Pts',(-18.4965403177724,-65.2758659894837,
28.778526011713));
#13721=CARTESIAN_POINT('Ctrl Pts',(-18.2572492368509,-65.7726863117686,
28.7414816390492));
#13722=CARTESIAN_POINT('Ctrl Pts',(-18.2885757078835,-66.3998482558001,
28.7044372663853));
#13723=CARTESIAN_POINT('Ctrl Pts',(-18.576184121226,-66.8703501735627,28.6673928937214));
#13724=CARTESIAN_POINT('Ctrl Pts',(-18.8637925345685,-67.3408520913253,
28.6303485210576));
#13725=CARTESIAN_POINT('Ctrl Pts',(-19.4076828902209,-67.654693982819,28.5933041483937));
#13726=CARTESIAN_POINT('Ctrl Pts',(-19.9589602577799,-67.6682556221481,
28.5562597757299));
#13727=CARTESIAN_POINT('Ctrl Pts',(-20.5102376253389,-67.6818172614771,
28.519215403066));
#13728=CARTESIAN_POINT('Ctrl Pts',(-21.0689020048045,-67.3950986486416,
28.4821710304022));
#13729=CARTESIAN_POINT('Ctrl Pts',(-21.3792975817233,-66.9393078634422,
28.4451266577383));
#13730=CARTESIAN_POINT('Ctrl Pts',(-21.565331458246,-66.6661321710056,28.4229243173621));
#13731=CARTESIAN_POINT('Ctrl Pts',(-21.6621837525239,-66.3322234195205,
28.400721976986));
#13732=CARTESIAN_POINT('Ctrl Pts',(-21.6637335962722,-65.999144500325,28.3785196366098));
#13733=CARTESIAN_POINT('Ctrl Pts',(-21.6672880470512,-65.9986896255742,
28.5714803633902));
#13734=CARTESIAN_POINT('Ctrl Pts',(-21.6632645028067,-66.4648808530385,
28.6027249797792));
#13735=CARTESIAN_POINT('Ctrl Pts',(-21.4589128498261,-66.934162969427,28.6339695961681));
#13736=CARTESIAN_POINT('Ctrl Pts',(-21.1121531076304,-67.2441368484079,
28.6652142125571));
#13737=CARTESIAN_POINT('Ctrl Pts',(-20.7010263728738,-67.6116493742805,
28.7022585852209));
#13738=CARTESIAN_POINT('Ctrl Pts',(-20.0897159185654,-67.7552215629484,
28.7393029578848));
#13739=CARTESIAN_POINT('Ctrl Pts',(-19.557969439069,-67.6091519554042,28.7763473305487));
#13740=CARTESIAN_POINT('Ctrl Pts',(-19.0262229595727,-67.46308234786,28.8133917032125));
#13741=CARTESIAN_POINT('Ctrl Pts',(-18.5740404548885,-67.0273709441037,
28.8504360758764));
#13742=CARTESIAN_POINT('Ctrl Pts',(-18.4083495380249,-66.5014078572109,
28.8874804485402));
#13743=CARTESIAN_POINT('Ctrl Pts',(-18.2426586211614,-65.9754447703182,
28.9245248212041));
#13744=CARTESIAN_POINT('Ctrl Pts',(-18.3634592921185,-65.3592300002889,
28.9615691938679));
#13745=CARTESIAN_POINT('Ctrl Pts',(-18.7154707865322,-64.9347555528772,
28.9986135665318));
#13746=CARTESIAN_POINT('Ctrl Pts',(-19.0674822809459,-64.5102811054654,
29.0356579391956));
#13747=CARTESIAN_POINT('Ctrl Pts',(-19.6507045988162,-64.2775469806712,
29.0727023118595));
#13748=CARTESIAN_POINT('Ctrl Pts',(-20.1982437297823,-64.3430568941632,
29.1097466845233));
#13749=CARTESIAN_POINT('Ctrl Pts',(-20.7457828607485,-64.4085668076551,
29.1467910571872));
#13750=CARTESIAN_POINT('Ctrl Pts',(-21.2576388048104,-64.7723207594334,
29.183835429851));
#13751=CARTESIAN_POINT('Ctrl Pts',(-21.4995762087385,-65.2678577825561,
29.2208798025149));
#13752=CARTESIAN_POINT('Ctrl Pts',(-21.6097339057125,-65.4934831565009,
29.23774665614));
#13753=CARTESIAN_POINT('Ctrl Pts',(-21.6639343505905,-65.7464286935643,
29.2546135097651));
#13754=CARTESIAN_POINT('Ctrl Pts',(-21.6633862072226,-65.9995968836612,
29.2714803633902));
#13755=CARTESIAN_POINT('Origin',(-20.,-66.,30.));
#13756=CARTESIAN_POINT('',(-21.6658101117288,-66.0015225986475,29.9714803633902));
#13757=CARTESIAN_POINT('',(-21.6687601732843,-66.0000189542795,29.7785196366098));
#13758=CARTESIAN_POINT('',(-21.666,-66.,30.));
#13759=CARTESIAN_POINT('Ctrl Pts',(-21.6687600689797,-66.0000189535633,
29.7785196366098));
#13760=CARTESIAN_POINT('Ctrl Pts',(-21.6686675101817,-65.4495889757353,
29.7415434096217));
#13761=CARTESIAN_POINT('Ctrl Pts',(-21.3695595260236,-64.8990728100273,
29.7045671826336));
#13762=CARTESIAN_POINT('Ctrl Pts',(-20.9076739098537,-64.5996824807776,
29.6675909556455));
#13763=CARTESIAN_POINT('Ctrl Pts',(-20.4449370573627,-64.2997403873821,
29.6305465829816));
#13764=CARTESIAN_POINT('Ctrl Pts',(-19.8188220349343,-64.2518506127082,
29.5935022103178));
#13765=CARTESIAN_POINT('Ctrl Pts',(-19.3158513986555,-64.4779284601082,
29.5564578376539));
#13766=CARTESIAN_POINT('Ctrl Pts',(-18.8128807623766,-64.7040063075082,
29.5194134649901));
#13767=CARTESIAN_POINT('Ctrl Pts',(-18.4330545122472,-65.2040517769822,
29.4823690923262));
#13768=CARTESIAN_POINT('Ctrl Pts',(-18.3501886152343,-65.7492342208998,
29.4453247196624));
#13769=CARTESIAN_POINT('Ctrl Pts',(-18.2673227182214,-66.2944166648174,
29.4082803469985));
#13770=CARTESIAN_POINT('Ctrl Pts',(-18.4814171743249,-66.8847360831788,
29.3712359743347));
#13771=CARTESIAN_POINT('Ctrl Pts',(-18.894498147094,-67.2500506927688,29.3341916016708));
#13772=CARTESIAN_POINT('Ctrl Pts',(-19.3075791198632,-67.6153653023587,
29.297147229007));
#13773=CARTESIAN_POINT('Ctrl Pts',(-19.9196466092979,-67.7556751031773,
29.2601028563431));
#13774=CARTESIAN_POINT('Ctrl Pts',(-20.4506064868622,-67.6067715690999,
29.2230584836792));
#13775=CARTESIAN_POINT('Ctrl Pts',(-20.9815663644265,-67.4578680350225,
29.1860141110154));
#13776=CARTESIAN_POINT('Ctrl Pts',(-21.4314186301202,-67.0197511660492,
29.1489697383515));
#13777=CARTESIAN_POINT('Ctrl Pts',(-21.5943020341556,-66.4929118634782,
29.1119253656877));
#13778=CARTESIAN_POINT('Ctrl Pts',(-21.6432634865546,-66.3345481702125,
29.1007901226617));
#13779=CARTESIAN_POINT('Ctrl Pts',(-21.6662957050299,-66.1681679112409,
29.0896548796358));
#13780=CARTESIAN_POINT('Ctrl Pts',(-21.6649409508278,-66.0014219187278,
29.0785196366098));
#13781=CARTESIAN_POINT('Ctrl Pts',(-21.6633862072226,-65.9995968836612,
29.2714803633902));
#13782=CARTESIAN_POINT('Ctrl Pts',(-21.6627304729945,-66.3024575172582,
29.291657882429));
#13783=CARTESIAN_POINT('Ctrl Pts',(-21.5837245035949,-66.6056367877023,
29.3118354014677));
#13784=CARTESIAN_POINT('Ctrl Pts',(-21.4284375187128,-66.8627440451906,
29.3320129205065));
#13785=CARTESIAN_POINT('Ctrl Pts',(-21.1433425609645,-67.334773190235,29.3690572931703));
#13786=CARTESIAN_POINT('Ctrl Pts',(-20.6011337816736,-67.6515113858566,
29.4061016658341));
#13787=CARTESIAN_POINT('Ctrl Pts',(-20.0499365888083,-67.6680130003919,
29.443146038498));
#13788=CARTESIAN_POINT('Ctrl Pts',(-19.498739395943,-67.6845146149272,29.4801904111618));
#13789=CARTESIAN_POINT('Ctrl Pts',(-18.9385537895033,-67.4007796483764,
29.5172347838257));
#13790=CARTESIAN_POINT('Ctrl Pts',(-18.6257317273414,-66.9466508052827,
29.5542791564896));
#13791=CARTESIAN_POINT('Ctrl Pts',(-18.3129096651795,-66.4925219621889,
29.5913235291534));
#13792=CARTESIAN_POINT('Ctrl Pts',(-18.2474511472954,-65.8679992425523,
29.6283679018173));
#13793=CARTESIAN_POINT('Ctrl Pts',(-18.4593112796838,-65.358876533366,29.6654122744811));
#13794=CARTESIAN_POINT('Ctrl Pts',(-18.6711714120723,-64.8497538241797,
29.702456647145));
#13795=CARTESIAN_POINT('Ctrl Pts',(-19.1603501947334,-64.4560311254436,
29.7395010198088));
#13796=CARTESIAN_POINT('Ctrl Pts',(-19.7029897897767,-64.3578836924866,
29.7765453924727));
#13797=CARTESIAN_POINT('Ctrl Pts',(-20.2456293848201,-64.2597362595296,
29.8135897651365));
#13798=CARTESIAN_POINT('Ctrl Pts',(-20.8417297922457,-64.4571640923516,
29.8506341378004));
#13799=CARTESIAN_POINT('Ctrl Pts',(-21.2185037344739,-64.8598203293115,
29.8876785104643));
#13800=CARTESIAN_POINT('Ctrl Pts',(-21.5026166529591,-65.1634502405319,
29.9156124614396));
#13801=CARTESIAN_POINT('Ctrl Pts',(-21.6620166986301,-65.5837766199149,
29.9435464124149));
#13802=CARTESIAN_POINT('Ctrl Pts',(-21.6658101117288,-66.0015225986475,
29.9714803633902));
#13803=CARTESIAN_POINT('Origin',(-20.,-66.,30.));
#13804=CARTESIAN_POINT('',(-21.6685541439151,-65.9994693779326,30.6714803633902));
#13805=CARTESIAN_POINT('',(-21.6649962084657,-65.998566115082,30.4785196366098));
#13806=CARTESIAN_POINT('',(-21.666,-66.,30.));
#13807=CARTESIAN_POINT('Ctrl Pts',(-21.6649962084657,-65.998566115082,30.4785196366098));
#13808=CARTESIAN_POINT('Ctrl Pts',(-21.6663489160884,-65.8338748640736,
30.4675206849354));
#13809=CARTESIAN_POINT('Ctrl Pts',(-21.6438880711133,-65.6695444194489,
30.4565217332609));
#13810=CARTESIAN_POINT('Ctrl Pts',(-21.5961003017824,-65.5129426030537,
30.4455227815864));
#13811=CARTESIAN_POINT('Ctrl Pts',(-21.4351515142742,-64.985509060469,30.4084784089226));
#13812=CARTESIAN_POINT('Ctrl Pts',(-20.9869101831435,-64.5457441677195,
30.3714340362587));
#13813=CARTESIAN_POINT('Ctrl Pts',(-20.4565003628192,-64.3948929942162,
30.3343896635948));
#13814=CARTESIAN_POINT('Ctrl Pts',(-19.9260905424949,-64.2440418207129,
30.297345290931));
#13815=CARTESIAN_POINT('Ctrl Pts',(-19.313512232977,-64.3821043664557,30.2603009182671));
#13816=CARTESIAN_POINT('Ctrl Pts',(-18.8990933241246,-64.7459004934683,
30.2232565456033));
#13817=CARTESIAN_POINT('Ctrl Pts',(-18.4846744152722,-65.1096966204808,
30.1862121729394));
#13818=CARTESIAN_POINT('Ctrl Pts',(-18.2684149070852,-65.6992263287631,
30.1491678002756));
#13819=CARTESIAN_POINT('Ctrl Pts',(-18.3492794064557,-66.2447092219737,
30.1121234276117));
#13820=CARTESIAN_POINT('Ctrl Pts',(-18.4301439058262,-66.7901921151842,
30.0750790549479));
#13821=CARTESIAN_POINT('Ctrl Pts',(-18.8081324127541,-67.2916281933229,
30.038034682284));
#13822=CARTESIAN_POINT('Ctrl Pts',(-19.310269947728,-67.5195504388677,30.0009903096202));
#13823=CARTESIAN_POINT('Ctrl Pts',(-19.8124074827018,-67.7474726844124,
29.9639459369563));
#13824=CARTESIAN_POINT('Ctrl Pts',(-20.4386940457216,-67.7018810973633,
29.9269015642924));
#13825=CARTESIAN_POINT('Ctrl Pts',(-20.9025285803499,-67.4036392851875,
29.8898571916286));
#13826=CARTESIAN_POINT('Ctrl Pts',(-21.3672163705614,-67.1048488366504,
29.852744673289));
#13827=CARTESIAN_POINT('Ctrl Pts',(-21.6688529689417,-66.5524777713161,
29.8156321549494));
#13828=CARTESIAN_POINT('Ctrl Pts',(-21.6687600689797,-66.0000189535633,
29.7785196366098));
#13829=CARTESIAN_POINT('Ctrl Pts',(-21.6658101117288,-66.0015225986475,
29.9714803633902));
#13830=CARTESIAN_POINT('Ctrl Pts',(-21.667047301305,-66.1377669139721,29.9805907850787));
#13831=CARTESIAN_POINT('Ctrl Pts',(-21.651732877632,-66.2737367564617,29.9897012067673));
#13832=CARTESIAN_POINT('Ctrl Pts',(-21.6187951015409,-66.405294277785,29.9988116284558));
#13833=CARTESIAN_POINT('Ctrl Pts',(-21.4848650493489,-66.940227348201,30.0358560011196));
#13834=CARTESIAN_POINT('Ctrl Pts',(-21.0595574679341,-67.4022088479354,
30.0729003737835));
#13835=CARTESIAN_POINT('Ctrl Pts',(-20.5375014765234,-67.5798269510023,
30.1099447464474));
#13836=CARTESIAN_POINT('Ctrl Pts',(-20.0154454851128,-67.7574450540693,
30.1469891191112));
#13837=CARTESIAN_POINT('Ctrl Pts',(-19.3966410837063,-67.6506997604689,
30.1840334917751));
#13838=CARTESIAN_POINT('Ctrl Pts',(-18.9642653443397,-67.3084398172795,
30.2210778644389));
#13839=CARTESIAN_POINT('Ctrl Pts',(-18.531889604973,-66.9661798740901,30.2581222371028));
#13840=CARTESIAN_POINT('Ctrl Pts',(-18.2859425276461,-66.3884052813118,
30.2951666097666));
#13841=CARTESIAN_POINT('Ctrl Pts',(-18.3389743351351,-65.839517063093,30.3322109824305));
#13842=CARTESIAN_POINT('Ctrl Pts',(-18.392006142624,-65.2906288448743,30.3692553550943));
#13843=CARTESIAN_POINT('Ctrl Pts',(-18.7440168349289,-64.7706270012152,
30.4062997277582));
#13844=CARTESIAN_POINT('Ctrl Pts',(-19.2339193917479,-64.5174746093107,
30.443344100422));
#13845=CARTESIAN_POINT('Ctrl Pts',(-19.723821948567,-64.2643222174062,30.4803884730859));
#13846=CARTESIAN_POINT('Ctrl Pts',(-20.3516163699004,-64.2780192772562,
30.5174328457497));
#13847=CARTESIAN_POINT('Ctrl Pts',(-20.830011573672,-64.5522977447179,30.5544772184136));
#13848=CARTESIAN_POINT('Ctrl Pts',(-21.3084067774437,-64.8265762121797,
30.5915215910775));
#13849=CARTESIAN_POINT('Ctrl Pts',(-21.6374027636536,-65.3614360872531,
30.6285659637413));
#13850=CARTESIAN_POINT('Ctrl Pts',(-21.6664444944342,-65.9121149651648,
30.6656103364052));
#13851=CARTESIAN_POINT('Ctrl Pts',(-21.667978472302,-65.9412017030505,30.6675670120668));
#13852=CARTESIAN_POINT('Ctrl Pts',(-21.6686755990056,-65.9703325748355,
30.6695236877285));
#13853=CARTESIAN_POINT('Ctrl Pts',(-21.6685541439151,-65.9994693779326,
30.6714803633902));
#13854=CARTESIAN_POINT('Origin',(-20.,-66.,30.));
#13855=CARTESIAN_POINT('',(-21.6642459804044,-65.9988133681836,31.3714803633902));
#13856=CARTESIAN_POINT('',(-21.663702450327,-66.0008273570352,31.1785196366098));
#13857=CARTESIAN_POINT('',(-21.666,-66.,30.));
#13858=CARTESIAN_POINT('Ctrl Pts',(-21.663702450327,-66.0008273570352,31.1785196366098));
#13859=CARTESIAN_POINT('Ctrl Pts',(-21.6622144391999,-65.6697775666387,
31.1564535875851));
#13860=CARTESIAN_POINT('Ctrl Pts',(-21.5666298198028,-65.3379360420718,
31.1343875385604));
#13861=CARTESIAN_POINT('Ctrl Pts',(-21.3827355870193,-65.065760535162,31.1123214895357));
#13862=CARTESIAN_POINT('Ctrl Pts',(-21.0740148693979,-64.6088336563782,
31.0752771168719));
#13863=CARTESIAN_POINT('Ctrl Pts',(-20.5164065201483,-64.3200666557085,
31.038232744208));
#13864=CARTESIAN_POINT('Ctrl Pts',(-19.9650830935122,-64.3316049955387,
31.0011883715442));
#13865=CARTESIAN_POINT('Ctrl Pts',(-19.4137596668761,-64.3431433353688,
30.9641439988803));
#13866=CARTESIAN_POINT('Ctrl Pts',(-18.8687211628537,-64.6549870156988,
30.9270996262165));
#13867=CARTESIAN_POINT('Ctrl Pts',(-18.5793879271388,-65.1244302313857,
30.8900552535526));
#13868=CARTESIAN_POINT('Ctrl Pts',(-18.2900546914239,-65.5938734470727,
30.8530108808888));
#13869=CARTESIAN_POINT('Ctrl Pts',(-18.2564267240166,-66.2209161981167,
30.8159665082249));
#13870=CARTESIAN_POINT('Ctrl Pts',(-18.4938928445943,-66.7186113815589,
30.7789221355611));
#13871=CARTESIAN_POINT('Ctrl Pts',(-18.7313589651721,-67.2163065650011,
30.7418777628972));
#13872=CARTESIAN_POINT('Ctrl Pts',(-19.2399191737349,-67.5846541808414,
30.7048333902334));
#13873=CARTESIAN_POINT('Ctrl Pts',(-19.7868463104771,-67.655091111061,30.6677890175695));
#13874=CARTESIAN_POINT('Ctrl Pts',(-20.3337734472193,-67.7255280412805,
30.6307446449057));
#13875=CARTESIAN_POINT('Ctrl Pts',(-20.9190675121408,-67.4980542858792,
30.5937002722418));
#13876=CARTESIAN_POINT('Ctrl Pts',(-21.2748864226587,-67.0767663119687,
30.5566558995779));
#13877=CARTESIAN_POINT('Ctrl Pts',(-21.5250581128238,-66.7805641671022,
30.5306104785886));
#13878=CARTESIAN_POINT('Ctrl Pts',(-21.6617930086926,-66.3885535514064,
30.5045650575992));
#13879=CARTESIAN_POINT('Ctrl Pts',(-21.6649962084657,-65.998566115082,30.4785196366098));
#13880=CARTESIAN_POINT('Ctrl Pts',(-21.6685541439151,-65.9994693779326,
30.6714803633902));
#13881=CARTESIAN_POINT('Ctrl Pts',(-21.666376174669,-66.5219593024021,30.7065680603924));
#13882=CARTESIAN_POINT('Ctrl Pts',(-21.4009689693529,-67.0463565435816,
30.7416557573945));
#13883=CARTESIAN_POINT('Ctrl Pts',(-20.9776818232741,-67.3523680286141,
30.7767434543967));
#13884=CARTESIAN_POINT('Ctrl Pts',(-20.530789945982,-67.6754443334016,30.8137878270606));
#13885=CARTESIAN_POINT('Ctrl Pts',(-19.9079187160463,-67.7550990622266,
30.8508321997244));
#13886=CARTESIAN_POINT('Ctrl Pts',(-19.3941062662719,-67.5548806435889,
30.8878765723883));
#13887=CARTESIAN_POINT('Ctrl Pts',(-18.8802938164976,-67.3546622249512,
30.9249209450521));
#13888=CARTESIAN_POINT('Ctrl Pts',(-18.4755401468847,-66.8745706588508,
30.961965317716));
#13889=CARTESIAN_POINT('Ctrl Pts',(-18.3650685021226,-66.3343052940453,
30.9990096903798));
#13890=CARTESIAN_POINT('Ctrl Pts',(-18.2545968573606,-65.7940399292398,
31.0360540630437));
#13891=CARTESIAN_POINT('Ctrl Pts',(-18.4384072374494,-65.1936007657291,
31.0730984357075));
#13892=CARTESIAN_POINT('Ctrl Pts',(-18.8323843951074,-64.8077605812633,
31.1101428083714));
#13893=CARTESIAN_POINT('Ctrl Pts',(-19.2263615527654,-64.4219203967975,
31.1471871810353));
#13894=CARTESIAN_POINT('Ctrl Pts',(-19.8305054879926,-64.2506791913767,
31.1842315536991));
#13895=CARTESIAN_POINT('Ctrl Pts',(-20.3683480465923,-64.3724003105954,
31.221275926363));
#13896=CARTESIAN_POINT('Ctrl Pts',(-20.9061906051919,-64.4941214298141,
31.2583202990268));
#13897=CARTESIAN_POINT('Ctrl Pts',(-21.377731787164,-64.9088048736724,31.2953646716906));
#13898=CARTESIAN_POINT('Ctrl Pts',(-21.567185067798,-65.4266833373701,31.3324090443545));
#13899=CARTESIAN_POINT('Ctrl Pts',(-21.6337915817138,-65.6087550279923,
31.3454328173664));
#13900=CARTESIAN_POINT('Ctrl Pts',(-21.665531173842,-65.8035819366461,31.3584565903783));
#13901=CARTESIAN_POINT('Ctrl Pts',(-21.6642459804044,-65.9988133681836,
31.3714803633902));
#13902=CARTESIAN_POINT('Origin',(-20.,-66.,30.));
#13903=CARTESIAN_POINT('',(-21.664269144494,-66.0011975491416,32.0714803633902));
#13904=CARTESIAN_POINT('',(-21.6680158191842,-66.0009873428354,31.8785196366098));
#13905=CARTESIAN_POINT('',(-21.666,-66.,30.));
#13906=CARTESIAN_POINT('Ctrl Pts',(-21.6680158191842,-66.0009873428354,
31.8785196366098));
#13907=CARTESIAN_POINT('Ctrl Pts',(-21.6645484604468,-65.5071812065553,
31.8453864902349));
#13908=CARTESIAN_POINT('Ctrl Pts',(-21.4314257512534,-65.010531043531,31.81225334386));
#13909=CARTESIAN_POINT('Ctrl Pts',(-21.0474729911752,-64.7009382562677,
31.7791201974851));
#13910=CARTESIAN_POINT('Ctrl Pts',(-20.618196249126,-64.3547993639436,31.7420758248213));
#13911=CARTESIAN_POINT('Ctrl Pts',(-20.0003779851722,-64.2424871003486,
31.7050314521574));
#13912=CARTESIAN_POINT('Ctrl Pts',(-19.4767439954439,-64.4153977675876,
31.6679870794935));
#13913=CARTESIAN_POINT('Ctrl Pts',(-18.9531100057157,-64.5883084348267,
31.6309427068297));
#13914=CARTESIAN_POINT('Ctrl Pts',(-18.523660290213,-65.0464420328999,31.5938983341659));
#13915=CARTESIAN_POINT('Ctrl Pts',(-18.384919490238,-65.5801476113475,31.556853961502));
#13916=CARTESIAN_POINT('Ctrl Pts',(-18.246178690263,-66.1138531897951,31.5198095888381));
#13917=CARTESIAN_POINT('Ctrl Pts',(-18.3981468058157,-66.7231307486171,
31.4827652161743));
#13918=CARTESIAN_POINT('Ctrl Pts',(-18.7712802365157,-67.129162886431,31.4457208435104));
#13919=CARTESIAN_POINT('Ctrl Pts',(-19.1444136672158,-67.535195024245,31.4086764708466));
#13920=CARTESIAN_POINT('Ctrl Pts',(-19.7387124130632,-67.737981741051,31.3716320981827));
#13921=CARTESIAN_POINT('Ctrl Pts',(-20.2822136722728,-67.6447238444348,
31.3345877255189));
#13922=CARTESIAN_POINT('Ctrl Pts',(-20.8257149314825,-67.5514659478186,
31.297543352855));
#13923=CARTESIAN_POINT('Ctrl Pts',(-21.3184187040544,-67.1621634377803,
31.2604989801912));
#13924=CARTESIAN_POINT('Ctrl Pts',(-21.534854047344,-66.6549688043121,31.2234546075273));
#13925=CARTESIAN_POINT('Ctrl Pts',(-21.6223663571936,-66.4498924371922,
31.2084762838881));
#13926=CARTESIAN_POINT('Ctrl Pts',(-21.6647125048327,-66.2255422978791,
31.193497960249));
#13927=CARTESIAN_POINT('Ctrl Pts',(-21.663702450327,-66.0008273570352,31.1785196366098));
#13928=CARTESIAN_POINT('Ctrl Pts',(-21.6642459804044,-65.9988133681836,
31.3714803633902));
#13929=CARTESIAN_POINT('Ctrl Pts',(-21.661875613767,-66.3588915154422,31.3955009630422));
#13930=CARTESIAN_POINT('Ctrl Pts',(-21.5471653402657,-66.7203457219942,
31.4195215626941));
#13931=CARTESIAN_POINT('Ctrl Pts',(-21.3316726311519,-67.0056883393076,
31.4435421623461));
#13932=CARTESIAN_POINT('Ctrl Pts',(-20.9993415345756,-67.4457413940104,
31.4805865350099));
#13933=CARTESIAN_POINT('Ctrl Pts',(-20.427313962127,-67.704774019879,31.5176309076738));
#13934=CARTESIAN_POINT('Ctrl Pts',(-19.8773609883515,-67.6642477896035,
31.5546752803376));
#13935=CARTESIAN_POINT('Ctrl Pts',(-19.327408014576,-67.623721559328,31.5917196530015));
#13936=CARTESIAN_POINT('Ctrl Pts',(-18.7995296394736,-67.2836364729084,
31.6287640256653));
#13937=CARTESIAN_POINT('Ctrl Pts',(-18.5352933960363,-66.7996221586996,
31.6658083983292));
#13938=CARTESIAN_POINT('Ctrl Pts',(-18.271057152599,-66.3156078444908,31.7028527709931));
#13939=CARTESIAN_POINT('Ctrl Pts',(-18.2704630408269,-65.6876643024928,
31.7398971436569));
#13940=CARTESIAN_POINT('Ctrl Pts',(-18.5337829379588,-65.2031508553324,
31.7769415163207));
#13941=CARTESIAN_POINT('Ctrl Pts',(-18.7971028350908,-64.7186374081719,
31.8139858889846));
#13942=CARTESIAN_POINT('Ctrl Pts',(-19.3243367411268,-64.377554055849,31.8510302616485));
#13943=CARTESIAN_POINT('Ctrl Pts',(-19.8742120448026,-64.3359872528416,
31.8880746343123));
#13944=CARTESIAN_POINT('Ctrl Pts',(-20.4240873484785,-64.2944204498342,
31.9251190069762));
#13945=CARTESIAN_POINT('Ctrl Pts',(-20.9966040497942,-64.5523701961424,
31.96216337964));
#13946=CARTESIAN_POINT('Ctrl Pts',(-21.3297672392087,-64.9917936114538,
31.9992077523039));
#13947=CARTESIAN_POINT('Ctrl Pts',(-21.5464314888222,-65.2775615100873,
32.023298622666));
#13948=CARTESIAN_POINT('Ctrl Pts',(-21.6618678224006,-65.6400786537288,
32.0473894930281));
#13949=CARTESIAN_POINT('Ctrl Pts',(-21.664269144494,-66.0011975491416,32.0714803633902));
#13950=CARTESIAN_POINT('Origin',(-20.,-66.,30.));
#13951=CARTESIAN_POINT('',(-21.6685680182217,-66.0005124578236,32.7714803633902));
#13952=CARTESIAN_POINT('',(-21.666694799795,-65.9985455596449,32.5785196366098));
#13953=CARTESIAN_POINT('',(-21.666,-66.,30.));
#13954=CARTESIAN_POINT('Ctrl Pts',(-21.666694799795,-65.9985455596449,32.5785196366098));
#13955=CARTESIAN_POINT('Ctrl Pts',(-21.6676729868231,-65.8916766829262,
32.5713637655485));
#13956=CARTESIAN_POINT('Ctrl Pts',(-21.6582744615622,-65.7849791688801,
32.5642078944873));
#13957=CARTESIAN_POINT('Ctrl Pts',(-21.6378751056044,-65.6804280680173,
32.557052023426));
#13958=CARTESIAN_POINT('Ctrl Pts',(-21.5322721206239,-65.1391899839851,
32.5200076507622));
#13959=CARTESIAN_POINT('Ctrl Pts',(-21.1318572715651,-64.6554737443548,
32.4829632780983));
#13960=CARTESIAN_POINT('Ctrl Pts',(-20.6198682734443,-64.4506374198246,
32.4459189054345));
#13961=CARTESIAN_POINT('Ctrl Pts',(-20.1078792753236,-64.2458010952945,
32.4088745327706));
#13962=CARTESIAN_POINT('Ctrl Pts',(-19.4843161281408,-64.3198446858643,
32.3718301601067));
#13963=CARTESIAN_POINT('Ctrl Pts',(-19.0345335996503,-64.6388843873256,
32.3347857874429));
#13964=CARTESIAN_POINT('Ctrl Pts',(-18.5847510711598,-64.9579240887869,
32.2977414147791));
#13965=CARTESIAN_POINT('Ctrl Pts',(-18.3087491613615,-65.5219599011395,
32.2606970421152));
#13966=CARTESIAN_POINT('Ctrl Pts',(-18.3328317758437,-66.0728779365345,
32.2236526694514));
#13967=CARTESIAN_POINT('Ctrl Pts',(-18.3569143903258,-66.6237959719295,
32.1866082967875));
#13968=CARTESIAN_POINT('Ctrl Pts',(-18.6810815290885,-67.1615962303668,
32.1495639241236));
#13969=CARTESIAN_POINT('Ctrl Pts',(-19.1569879298867,-67.4401707297795,
32.1125195514598));
#13970=CARTESIAN_POINT('Ctrl Pts',(-19.6328943306849,-67.7187452291921,
32.0754751787959));
#13971=CARTESIAN_POINT('Ctrl Pts',(-20.2605399935188,-67.7380939695802,
32.0384308061321));
#13972=CARTESIAN_POINT('Ctrl Pts',(-20.7527019111292,-67.4893625865627,
32.0013864334682));
#13973=CARTESIAN_POINT('Ctrl Pts',(-21.2448638287396,-67.2406312035451,
31.9643420608044));
#13974=CARTESIAN_POINT('Ctrl Pts',(-21.6015420011265,-66.7238196971218,
31.9272976881405));
#13975=CARTESIAN_POINT('Ctrl Pts',(-21.6595134772477,-66.1754311833835,
31.8902533154767));
#13976=CARTESIAN_POINT('Ctrl Pts',(-21.6656342331172,-66.1175311187514,
31.8863420891877));
#13977=CARTESIAN_POINT('Ctrl Pts',(-21.6684251260605,-66.0592790462557,
31.8824308628988));
#13978=CARTESIAN_POINT('Ctrl Pts',(-21.6680158191842,-66.0009873428354,
31.8785196366098));
#13979=CARTESIAN_POINT('Ctrl Pts',(-21.664269144494,-66.0011975491416,32.0714803633902));
#13980=CARTESIAN_POINT('Ctrl Pts',(-21.6655603195657,-66.1953688004339,
32.084433865692));
#13981=CARTESIAN_POINT('Ctrl Pts',(-21.6341714670255,-66.3891357982996,
32.0973873679937));
#13982=CARTESIAN_POINT('Ctrl Pts',(-21.5682671171625,-66.5703501394802,
32.1103408702954));
#13983=CARTESIAN_POINT('Ctrl Pts',(-21.3797941281882,-67.0885861678804,
32.1473852429593));
#13984=CARTESIAN_POINT('Ctrl Pts',(-20.9090384727262,-67.504161140366,32.1844296156231));
#13985=CARTESIAN_POINT('Ctrl Pts',(-20.3714272030969,-67.6268997710916,
32.221473988287));
#13986=CARTESIAN_POINT('Ctrl Pts',(-19.8338159334676,-67.7496384018173,
32.2585183609508));
#13987=CARTESIAN_POINT('Ctrl Pts',(-19.229349049671,-67.579540690783,32.2955627336147));
#13988=CARTESIAN_POINT('Ctrl Pts',(-18.8346424935248,-67.1944466980488,
32.3326071062786));
#13989=CARTESIAN_POINT('Ctrl Pts',(-18.4399359373785,-66.8093527053147,
32.3696514789424));
#13990=CARTESIAN_POINT('Ctrl Pts',(-18.2549897088826,-66.2092624308807,
32.4066958516062));
#13991=CARTESIAN_POINT('Ctrl Pts',(-18.3644388419032,-65.6687889939883,
32.4437402242701));
#13992=CARTESIAN_POINT('Ctrl Pts',(-18.4738879749238,-65.1283155570959,
32.4807845969339));
#13993=CARTESIAN_POINT('Ctrl Pts',(-18.8777324694608,-64.6474589577452,
32.5178289695978));
#13994=CARTESIAN_POINT('Ctrl Pts',(-19.3911651372318,-64.4462686389668,
32.5548733422617));
#13995=CARTESIAN_POINT('Ctrl Pts',(-19.9045978050028,-64.2450783201884,
32.5919177149255));
#13996=CARTESIAN_POINT('Ctrl Pts',(-20.5276186460077,-64.3235542819823,
32.6289620875894));
#13997=CARTESIAN_POINT('Ctrl Pts',(-20.9751210624724,-64.6457843798355,
32.6660064602532));
#13998=CARTESIAN_POINT('Ctrl Pts',(-21.399835381487,-64.9516056034546,32.7011644279656));
#13999=CARTESIAN_POINT('Ctrl Pts',(-21.6664519287834,-65.4769877413138,
32.7363223956779));
#14000=CARTESIAN_POINT('Ctrl Pts',(-21.6685680182217,-66.0005124578236,
32.7714803633902));
#14001=CARTESIAN_POINT('Origin',(-20.,-66.,30.));
#14002=CARTESIAN_POINT('',(-21.665778632213,-65.9984780340856,33.4714803633902));
#14003=CARTESIAN_POINT('',(-21.6632991006019,-65.9999263102654,33.2785196366098));
#14004=CARTESIAN_POINT('',(-21.666,-66.,30.));
#14005=CARTESIAN_POINT('Ctrl Pts',(-21.6632991006019,-65.9999263102654,
33.2785196366098));
#14006=CARTESIAN_POINT('Ctrl Pts',(-21.6634070404292,-65.7263673499551,
33.2602966681983));
#14007=CARTESIAN_POINT('Ctrl Pts',(-21.5996813808277,-65.4528557432902,
33.2420736997869));
#14008=CARTESIAN_POINT('Ctrl Pts',(-21.4718465072752,-65.2135974693183,
33.2238507313754));
#14009=CARTESIAN_POINT('Ctrl Pts',(-21.2119787081117,-64.7272237642339,
33.1868063587115));
#14010=CARTESIAN_POINT('Ctrl Pts',(-20.687183619355,-64.3823997995165,33.1497619860477));
#14011=CARTESIAN_POINT('Ctrl Pts',(-20.1376178014656,-64.3369238075172,
33.1127176133838));
#14012=CARTESIAN_POINT('Ctrl Pts',(-19.5880519835761,-64.2914478155178,
33.07567324072));
#14013=CARTESIAN_POINT('Ctrl Pts',(-19.0137154365539,-64.5453197962364,
33.0386288680561));
#14014=CARTESIAN_POINT('Ctrl Pts',(-18.67743586716,-64.9823629351308,33.0015844953922));
#14015=CARTESIAN_POINT('Ctrl Pts',(-18.3411562977662,-65.4194060740252,
32.9645401227284));
#14016=CARTESIAN_POINT('Ctrl Pts',(-18.2429337060008,-66.0396203710956,
32.9274957500646));
#14017=CARTESIAN_POINT('Ctrl Pts',(-18.427716682852,-66.5591835583106,32.8904513774007));
#14018=CARTESIAN_POINT('Ctrl Pts',(-18.6124996597033,-67.0787467455257,
32.8534070047369));
#14019=CARTESIAN_POINT('Ctrl Pts',(-19.0802882051712,-67.4976588228855,
32.816362632073));
#14020=CARTESIAN_POINT('Ctrl Pts',(-19.6170130748635,-67.6242173796775,
32.7793182594091));
#14021=CARTESIAN_POINT('Ctrl Pts',(-20.1537379445558,-67.7507759364695,
32.7422738867453));
#14022=CARTESIAN_POINT('Ctrl Pts',(-20.7593991384724,-67.5849809726938,
32.7052295140814));
#14023=CARTESIAN_POINT('Ctrl Pts',(-21.1568341749797,-67.2027035265888,
32.6681851414176));
#14024=CARTESIAN_POINT('Ctrl Pts',(-21.4774965825568,-66.8942707137504,
32.638296639815));
#14025=CARTESIAN_POINT('Ctrl Pts',(-21.6626091274417,-66.4449133834543,
32.6084081382124));
#14026=CARTESIAN_POINT('Ctrl Pts',(-21.666694799795,-65.9985455596449,32.5785196366098));
#14027=CARTESIAN_POINT('Ctrl Pts',(-21.6685680182217,-66.0005124578236,
32.7714803633902));
#14028=CARTESIAN_POINT('Ctrl Pts',(-21.6686815572529,-66.0286022389381,
32.7733667683417));
#14029=CARTESIAN_POINT('Ctrl Pts',(-21.6680336333681,-66.0566866727747,
32.7752531732933));
#14030=CARTESIAN_POINT('Ctrl Pts',(-21.6666078109475,-66.0847315576818,
32.7771395782448));
#14031=CARTESIAN_POINT('Ctrl Pts',(-21.6386081510336,-66.6354644037626,
32.8141839509086));
#14032=CARTESIAN_POINT('Ctrl Pts',(-21.3106248392815,-67.1709458620117,
32.8512283235725));
#14033=CARTESIAN_POINT('Ctrl Pts',(-20.8327494937987,-67.4461290789448,
32.8882726962363));
#14034=CARTESIAN_POINT('Ctrl Pts',(-20.3548741483159,-67.7213122958779,
32.9253170689002));
#14035=CARTESIAN_POINT('Ctrl Pts',(-19.7271067691025,-67.7361972714949,
32.962361441564));
#14036=CARTESIAN_POINT('Ctrl Pts',(-19.2367260632258,-67.4839723480544,
32.9994058142279));
#14037=CARTESIAN_POINT('Ctrl Pts',(-18.7463453573491,-67.2317474246138,
33.0364501868918));
#14038=CARTESIAN_POINT('Ctrl Pts',(-18.3933513248091,-66.7124126021157,
33.0734945595556));
#14039=CARTESIAN_POINT('Ctrl Pts',(-18.3392809817557,-66.1636257156765,
33.1105389322195));
#14040=CARTESIAN_POINT('Ctrl Pts',(-18.2852106387023,-65.6148388292373,
33.1475833048833));
#14041=CARTESIAN_POINT('Ctrl Pts',(-18.5300639851355,-65.036599878857,33.1846276775472));
#14042=CARTESIAN_POINT('Ctrl Pts',(-18.9617913110511,-64.6935223879976,
33.221672050211));
#14043=CARTESIAN_POINT('Ctrl Pts',(-19.3935186369667,-64.3504448971382,
33.2587164228749));
#14044=CARTESIAN_POINT('Ctrl Pts',(-20.0121199423648,-64.2425288657996,
33.2957607955387));
#14045=CARTESIAN_POINT('Ctrl Pts',(-20.5345110959589,-64.4191587934175,
33.3328051682026));
#14046=CARTESIAN_POINT('Ctrl Pts',(-21.056902249553,-64.5957887210355,33.3698495408664));
#14047=CARTESIAN_POINT('Ctrl Pts',(-21.4830832513432,-65.05696460761,33.4068939135303));
#14048=CARTESIAN_POINT('Ctrl Pts',(-21.6180252877123,-65.5916432921331,
33.4439382861941));
#14049=CARTESIAN_POINT('Ctrl Pts',(-21.6514679198442,-65.7241525015422,
33.4531189785928));
#14050=CARTESIAN_POINT('Ctrl Pts',(-21.6670227959202,-65.8611762171652,
33.4622996709915));
#14051=CARTESIAN_POINT('Ctrl Pts',(-21.665778632213,-65.9984780340856,33.4714803633902));
#14052=CARTESIAN_POINT('Origin',(-20.,-66.,30.));
#14053=CARTESIAN_POINT('',(-21.6633939784266,-66.0004198226392,34.1714803633902));
#14054=CARTESIAN_POINT('',(-21.6664243436945,-66.0014929634474,33.9785196366098));
#14055=CARTESIAN_POINT('',(-21.666,-66.,30.));
#14056=CARTESIAN_POINT('Ctrl Pts',(-21.6664243436945,-66.0014929634474,
33.9785196366098));
#14057=CARTESIAN_POINT('Ctrl Pts',(-21.6623854969713,-65.56387976128,33.9492295708481));
#14058=CARTESIAN_POINT('Ctrl Pts',(-21.4853949308404,-65.1233755126288,
33.9199395050864));
#14059=CARTESIAN_POINT('Ctrl Pts',(-21.1760642722398,-64.8160937930611,
33.8906494393247));
#14060=CARTESIAN_POINT('Ctrl Pts',(-20.7848408353656,-64.4274617351793,
33.8536050666609));
#14061=CARTESIAN_POINT('Ctrl Pts',(-20.1819298910283,-64.2519287056668,
33.816560693997));
#14062=CARTESIAN_POINT('Ctrl Pts',(-19.6432353511812,-64.3698220749688,
33.7795163213332));
#14063=CARTESIAN_POINT('Ctrl Pts',(-19.1045408113341,-64.4877154442707,
33.7424719486693));
#14064=CARTESIAN_POINT('Ctrl Pts',(-18.6300626759773,-64.8990352123871,
33.7054275760055));
#14065=CARTESIAN_POINT('Ctrl Pts',(-18.4369314781643,-65.4155533578892,
33.6683832033416));
#14066=CARTESIAN_POINT('Ctrl Pts',(-18.2438002803514,-65.9320715033912,
33.6313388306778));
#14067=CARTESIAN_POINT('Ctrl Pts',(-18.3320160200823,-66.553788026279,33.5942944580139));
#14068=CARTESIAN_POINT('Ctrl Pts',(-18.6612094384485,-66.9961932108407,
33.5572500853501));
#14069=CARTESIAN_POINT('Ctrl Pts',(-18.9904028568147,-67.4385983954023,
33.5202057126862));
#14070=CARTESIAN_POINT('Ctrl Pts',(-19.5605739538163,-67.7016922416377,
33.4831613400223));
#14071=CARTESIAN_POINT('Ctrl Pts',(-20.1108012147773,-67.6650778276609,
33.4461169673585));
#14072=CARTESIAN_POINT('Ctrl Pts',(-20.6610284757384,-67.628463413684,33.4090725946946));
#14073=CARTESIAN_POINT('Ctrl Pts',(-21.191311900659,-67.2921407394949,33.3720282220308));
#14074=CARTESIAN_POINT('Ctrl Pts',(-21.458983358334,-66.8100176796745,33.334983849367));
#14075=CARTESIAN_POINT('Ctrl Pts',(-21.5949811455672,-66.5650619048632,
33.3161624451146));
#14076=CARTESIAN_POINT('Ctrl Pts',(-21.6631876160688,-66.2824688501306,
33.2973410408622));
#14077=CARTESIAN_POINT('Ctrl Pts',(-21.6632991006019,-65.9999263102654,
33.2785196366098));
#14078=CARTESIAN_POINT('Ctrl Pts',(-21.665778632213,-65.9984780340856,33.4714803633902));
#14079=CARTESIAN_POINT('Ctrl Pts',(-21.6620025575742,-66.4151932185574,
33.4993440436554));
#14080=CARTESIAN_POINT('Ctrl Pts',(-21.5034836506645,-66.8344701079231,
33.5272077239205));
#14081=CARTESIAN_POINT('Ctrl Pts',(-21.2206590512588,-67.1378719231945,
33.5550714041857));
#14082=CARTESIAN_POINT('Ctrl Pts',(-20.8446477074886,-67.5412403872612,
33.5921157768495));
#14083=CARTESIAN_POINT('Ctrl Pts',(-20.2489219490002,-67.7397958329229,
33.6291601495134));
#14084=CARTESIAN_POINT('Ctrl Pts',(-19.7060976064966,-67.642675382864,33.6662045221772));
#14085=CARTESIAN_POINT('Ctrl Pts',(-19.1632732639931,-67.5455549328051,
33.7032488948411));
#14086=CARTESIAN_POINT('Ctrl Pts',(-18.6733503374743,-67.1527585870256,
33.740293267505));
#14087=CARTESIAN_POINT('Ctrl Pts',(-18.4605272000038,-66.64403767922,33.7773376401688));
#14088=CARTESIAN_POINT('Ctrl Pts',(-18.2477040625333,-66.1353167714144,
33.8143820128327));
#14089=CARTESIAN_POINT('Ctrl Pts',(-18.3119807141111,-65.5106713015827,
33.8514263854965));
#14090=CARTESIAN_POINT('Ctrl Pts',(-18.6239428934263,-65.055951338178,33.8884707581604));
#14091=CARTESIAN_POINT('Ctrl Pts',(-18.9359050727415,-64.6012313747734,
33.9255151308242));
#14092=CARTESIAN_POINT('Ctrl Pts',(-19.4955527797942,-64.3164369177958,
33.9625595034881));
#14093=CARTESIAN_POINT('Ctrl Pts',(-20.0467802112671,-64.3318954984015,
33.9996038761519));
#14094=CARTESIAN_POINT('Ctrl Pts',(-20.59800764274,-64.3473540790071,34.0366482488158));
#14095=CARTESIAN_POINT('Ctrl Pts',(-21.1408147986332,-64.6630656971959,
34.0736926214796));
#14096=CARTESIAN_POINT('Ctrl Pts',(-21.4268024396972,-65.1345545373491,
34.1107369941435));
#14097=CARTESIAN_POINT('Ctrl Pts',(-21.5831181554361,-65.3922618817548,
34.1309847838924));
#14098=CARTESIAN_POINT('Ctrl Pts',(-21.6627085390352,-65.6965079757682,
34.1512325736413));
#14099=CARTESIAN_POINT('Ctrl Pts',(-21.6633939784266,-66.0004198226392,
34.1714803633902));
#14100=CARTESIAN_POINT('Origin',(-20.,-66.,30.));
#14101=CARTESIAN_POINT('',(-21.6673174954184,-66.0013023234915,34.8714803633902));
#14102=CARTESIAN_POINT('',(-21.668208945928,-65.9991411290017,34.6785196366098));
#14103=CARTESIAN_POINT('',(-21.666,-66.,30.));
#14104=CARTESIAN_POINT('Ctrl Pts',(-21.668208945928,-65.9991411290017,34.6785196366098));
#14105=CARTESIAN_POINT('Ctrl Pts',(-21.6685189954827,-65.9497833734107,
34.6752068461617));
#14106=CARTESIAN_POINT('Ctrl Pts',(-21.6665182740216,-65.9004511060839,
34.6718940557137));
#14107=CARTESIAN_POINT('Ctrl Pts',(-21.6621249449702,-65.851332844456,34.6685812652657));
#14108=CARTESIAN_POINT('Ctrl Pts',(-21.6129977450565,-65.302081324664,34.6315368926018));
#14109=CARTESIAN_POINT('Ctrl Pts',(-21.2646936610931,-64.7795895453484,
34.594492519938));
#14110=CARTESIAN_POINT('Ctrl Pts',(-20.7766036652056,-64.5229598163238,
34.5574481472741));
#14111=CARTESIAN_POINT('Ctrl Pts',(-20.2885136693181,-64.2663300872993,
34.5204037746103));
#14112=CARTESIAN_POINT('Ctrl Pts',(-19.6606377615066,-64.2755624085656,
34.4833594019464));
#14113=CARTESIAN_POINT('Ctrl Pts',(-19.1803042290292,-64.5464319940161,
34.4463150292825));
#14114=CARTESIAN_POINT('Ctrl Pts',(-18.6999706965518,-64.8173015794665,
34.4092706566187));
#14115=CARTESIAN_POINT('Ctrl Pts',(-18.3671795394086,-65.349808429101,34.3722262839548));
#14116=CARTESIAN_POINT('Ctrl Pts',(-18.3342225828221,-65.9002668758333,
34.335181911291));
#14117=CARTESIAN_POINT('Ctrl Pts',(-18.3012656262355,-66.4507253225656,
34.2981375386271));
#14118=CARTESIAN_POINT('Ctrl Pts',(-18.5681428702056,-67.0191353663957,
34.2610931659633));
#14119=CARTESIAN_POINT('Ctrl Pts',(-19.0127260145093,-67.3453814116786,
34.2240487932994));
#14120=CARTESIAN_POINT('Ctrl Pts',(-19.457309158813,-67.6716274569616,34.1870044206356));
#14121=CARTESIAN_POINT('Ctrl Pts',(-20.0795982034502,-67.7557095036974,
34.1499600479717));
#14122=CARTESIAN_POINT('Ctrl Pts',(-20.5948214457436,-67.5591499392339,
34.1129156753078));
#14123=CARTESIAN_POINT('Ctrl Pts',(-21.110044688037,-67.3625903747704,34.075871302644));
#14124=CARTESIAN_POINT('Ctrl Pts',(-21.5182021279864,-66.8853891991076,
34.0388269299801));
#14125=CARTESIAN_POINT('Ctrl Pts',(-21.6325128832557,-66.3459230681507,
34.0017825573163));
#14126=CARTESIAN_POINT('Ctrl Pts',(-21.6564409623358,-66.2329994135725,
33.9940282504141));
#14127=CARTESIAN_POINT('Ctrl Pts',(-21.6674935955452,-66.1173475027186,
33.986273943512));
#14128=CARTESIAN_POINT('Ctrl Pts',(-21.6664243436945,-66.0014929634474,
33.9785196366098));
#14129=CARTESIAN_POINT('Ctrl Pts',(-21.6633939784266,-66.0004198226392,
34.1714803633902));
#14130=CARTESIAN_POINT('Ctrl Pts',(-21.6639625856531,-66.2525303294208,
34.1882769463052));
#14131=CARTESIAN_POINT('Ctrl Pts',(-21.6102323157922,-66.5044108221688,
34.2050735292201));
#14132=CARTESIAN_POINT('Ctrl Pts',(-21.5009589145427,-66.7293033613947,
34.2218701121351));
#14133=CARTESIAN_POINT('Ctrl Pts',(-21.2599596220895,-67.2252972831696,
34.2589144847989));
#14134=CARTESIAN_POINT('Ctrl Pts',(-20.7487929109483,-67.5900190646018,
34.2959588574628));
#14135=CARTESIAN_POINT('Ctrl Pts',(-20.2013787183707,-67.6565649760457,
34.3330032301266));
#14136=CARTESIAN_POINT('Ctrl Pts',(-19.6539645257931,-67.7231108874895,
34.3700476027905));
#14137=CARTESIAN_POINT('Ctrl Pts',(-19.070302851779,-67.4914809289449,34.4070919754543));
#14138=CARTESIAN_POINT('Ctrl Pts',(-18.7174887835078,-67.0676732583278,
34.4441363481182));
#14139=CARTESIAN_POINT('Ctrl Pts',(-18.3646747152366,-66.6438655877108,
34.481180720782));
#14140=CARTESIAN_POINT('Ctrl Pts',(-18.2427082527083,-66.0278802050213,
34.5182250934459));
#14141=CARTESIAN_POINT('Ctrl Pts',(-18.4074036119675,-65.501604681277,34.5552694661097));
#14142=CARTESIAN_POINT('Ctrl Pts',(-18.5720989712267,-64.9753291575327,
34.5923138387736));
#14143=CARTESIAN_POINT('Ctrl Pts',(-19.0234561522734,-64.5387634927337,
34.6293582114374));
#14144=CARTESIAN_POINT('Ctrl Pts',(-19.5549253011755,-64.3916876550998,
34.6664025841013));
#14145=CARTESIAN_POINT('Ctrl Pts',(-20.0863944500777,-64.244611817466,34.7034469567651));
#14146=CARTESIAN_POINT('Ctrl Pts',(-20.6979755668353,-64.3870258069973,
34.740491329429));
#14147=CARTESIAN_POINT('Ctrl Pts',(-21.1097969476086,-64.7537603158085,
34.7775357020928));
#14148=CARTESIAN_POINT('Ctrl Pts',(-21.4579237781244,-65.0637736569165,
34.808850589192));
#14149=CARTESIAN_POINT('Ctrl Pts',(-21.6633042078259,-65.5340843001723,
34.8401654762911));
#14150=CARTESIAN_POINT('Ctrl Pts',(-21.6673174954184,-66.0013023234915,
34.8714803633902));
#14151=CARTESIAN_POINT('Origin',(-20.,-66.,30.));
#14152=CARTESIAN_POINT('',(-21.6674773009859,-65.998786811783,35.5714803633902));
#14153=CARTESIAN_POINT('',(-21.6638441630143,-65.999055839902,35.3785196366098));
#14154=CARTESIAN_POINT('',(-21.666,-66.,30.));
#14155=CARTESIAN_POINT('',(-18.7309291201477,-64.9206413469514,36.));
#14156=CARTESIAN_POINT('Ctrl Pts',(-21.6674773009859,-65.998786811783,35.5714803633902));
#14157=CARTESIAN_POINT('Ctrl Pts',(-21.6635425730949,-66.4716252930546,
35.6031871242686));
#14158=CARTESIAN_POINT('Ctrl Pts',(-21.4523796956911,-66.9474486915342,
35.634893885147));
#14159=CARTESIAN_POINT('Ctrl Pts',(-21.0965955086794,-67.2577323833415,
35.6666006460253));
#14160=CARTESIAN_POINT('Ctrl Pts',(-20.6809175382262,-67.6202501679528,
35.7036450186892));
#14161=CARTESIAN_POINT('Ctrl Pts',(-20.0678278060009,-67.7568020473594,
35.740689391353));
#14162=CARTESIAN_POINT('Ctrl Pts',(-19.5379530745693,-67.6038093166544,
35.7777337640169));
#14163=CARTESIAN_POINT('Ctrl Pts',(-19.0080783431377,-67.4508165859494,
35.8147781366807));
#14164=CARTESIAN_POINT('Ctrl Pts',(-18.5614186124997,-67.0082792451327,
35.8518225093446));
#14165=CARTESIAN_POINT('Ctrl Pts',(-18.4024070521432,-66.4812299699562,
35.8888668820084));
#14166=CARTESIAN_POINT('Ctrl Pts',(-18.2433954917868,-65.9541806947796,
35.9259112546723));
#14167=CARTESIAN_POINT('Ctrl Pts',(-18.372032101712,-65.3426194852432,35.9629556273362));
#14168=CARTESIAN_POINT('Ctrl Pts',(-18.7309291201477,-64.9206413469514,
36.));
#14169=CARTESIAN_POINT('',(-21.2714721999681,-64.9187950709037,36.));
#14170=CARTESIAN_POINT('Origin',(-20.,-66.,36.));
#14171=CARTESIAN_POINT('Ctrl Pts',(-21.2714736587042,-64.9187939493416,
36.));
#14172=CARTESIAN_POINT('Ctrl Pts',(-20.9206574088577,-64.5073240780818,
35.9636818543909));
#14173=CARTESIAN_POINT('Ctrl Pts',(-20.3507903997101,-64.2812824034869,
35.9273637087819));
#14174=CARTESIAN_POINT('Ctrl Pts',(-19.8134508486065,-64.3418046038641,
35.8910455631728));
#14175=CARTESIAN_POINT('Ctrl Pts',(-19.2653665165382,-64.4035370218501,
35.854001190509));
#14176=CARTESIAN_POINT('Ctrl Pts',(-18.7511235035973,-64.7634083085501,
35.8169568178451));
#14177=CARTESIAN_POINT('Ctrl Pts',(-18.5057149290944,-65.2571540728335,
35.7799124451812));
#14178=CARTESIAN_POINT('Ctrl Pts',(-18.2603063545915,-65.7508998371168,
35.7428680725174));
#14179=CARTESIAN_POINT('Ctrl Pts',(-18.2837322185265,-66.3785200789834,
35.7058236998535));
#14180=CARTESIAN_POINT('Ctrl Pts',(-18.565439975346,-66.8525938141442,35.6687793271897));
#14181=CARTESIAN_POINT('Ctrl Pts',(-18.8471477321655,-67.3266675493049,
35.6317349545258));
#14182=CARTESIAN_POINT('Ctrl Pts',(-19.3871373818695,-67.6471947777599,
35.594690581862));
#14183=CARTESIAN_POINT('Ctrl Pts',(-19.9382149975217,-67.6676009890549,
35.5576462091981));
#14184=CARTESIAN_POINT('Ctrl Pts',(-20.4892926131739,-67.68800720035,35.5206018365343));
#14185=CARTESIAN_POINT('Ctrl Pts',(-21.0514581947743,-67.4082923944853,
35.4835574638704));
#14186=CARTESIAN_POINT('Ctrl Pts',(-21.367495855437,-66.9564068860944,35.4465130912066));
#14187=CARTESIAN_POINT('Ctrl Pts',(-21.5608539895331,-66.6799343336008,
35.423848606341));
#14188=CARTESIAN_POINT('Ctrl Pts',(-21.6620806326978,-66.3390142228699,
35.4011841214754));
#14189=CARTESIAN_POINT('Ctrl Pts',(-21.6638441630143,-65.999055839902,35.3785196366098));
#14190=CARTESIAN_POINT('Origin',(-20.,-66.,37.5459252805377));
#14191=CARTESIAN_POINT('',(-22.0554079541519,-65.9981768930466,25.3540747194623));
#14192=CARTESIAN_POINT('',(-22.0529266054906,-66.0015060728813,25.2959252805377));
#14193=CARTESIAN_POINT('',(-22.05475,-65.9999999999998,37.5459252805377));
#14194=CARTESIAN_POINT('',(-18.1825721112405,-65.0413794120407,25.));
#14195=CARTESIAN_POINT('Ctrl Pts',(-22.0529266054906,-66.0015060728812,
25.2959252805377));
#14196=CARTESIAN_POINT('Ctrl Pts',(-22.0499364984145,-65.5475810030442,
25.2713722656862));
#14197=CARTESIAN_POINT('Ctrl Pts',(-21.6783088984842,-64.4040177540137,
25.2097748781708));
#14198=CARTESIAN_POINT('Ctrl Pts',(-19.7840052970778,-63.5820406376141,
25.1111331179915));
#14199=CARTESIAN_POINT('Ctrl Pts',(-18.5013225746365,-64.4370673526013,
25.0370443726639));
#14200=CARTESIAN_POINT('Ctrl Pts',(-18.1825721112405,-65.0413794120407,
25.));
#14201=CARTESIAN_POINT('',(-17.9429020987956,-66.0754554248319,25.));
#14202=CARTESIAN_POINT('Origin',(-20.,-66.,25.));
#14203=CARTESIAN_POINT('Ctrl Pts',(-22.0554079541519,-65.9981768930466,
25.3540747194623));
#14204=CARTESIAN_POINT('Ctrl Pts',(-22.0567025337672,-65.8578133551516,
25.3464567039117));
#14205=CARTESIAN_POINT('Ctrl Pts',(-21.9795742048134,-65.0363088793791,
25.3017943156971));
#14206=CARTESIAN_POINT('Ctrl Pts',(-20.8736249251117,-63.7340407352631,
25.2200875548188));
#14207=CARTESIAN_POINT('Ctrl Pts',(-18.5861500435499,-64.0348865828967,
25.109680663882));
#14208=CARTESIAN_POINT('Ctrl Pts',(-17.9193181381118,-65.408977698993,25.0363181456091));
#14209=CARTESIAN_POINT('Ctrl Pts',(-17.9428998377409,-66.0754556195432,
25.));
#14210=CARTESIAN_POINT('Origin',(-20.,-66.,37.5459252805377));
#14211=CARTESIAN_POINT('',(-22.0514168805361,-66.0000495912933,26.0540747194623));
#14212=CARTESIAN_POINT('',(-22.058013816727,-66.0004830916995,25.9959252805377));
#14213=CARTESIAN_POINT('',(-22.05475,-65.9999999999998,37.5459252805377));
#14214=CARTESIAN_POINT('Ctrl Pts',(-22.058013816727,-66.0004830916995,25.9959252805377));
#14215=CARTESIAN_POINT('Ctrl Pts',(-22.0559447889388,-65.3463924343595,
25.9603051683359));
#14216=CARTESIAN_POINT('Ctrl Pts',(-21.3649311801284,-64.0082840748463,
25.8876406834704));
#14217=CARTESIAN_POINT('Ctrl Pts',(-19.0858252946999,-63.7500130051076,
25.7779318259409));
#14218=CARTESIAN_POINT('Ctrl Pts',(-17.6139704758136,-65.5475930823177,
25.6667987079494));
#14219=CARTESIAN_POINT('Ctrl Pts',(-18.3256043860741,-67.7593785018947,
25.5556655899578));
#14220=CARTESIAN_POINT('Ctrl Pts',(-20.570308099232,-68.3606229135291,25.4445324719662));
#14221=CARTESIAN_POINT('Ctrl Pts',(-21.9115055060277,-67.1462798849558,
25.3579523688262));
#14222=CARTESIAN_POINT('Ctrl Pts',(-22.0544478238668,-66.2324406648902,
25.30841663835));
#14223=CARTESIAN_POINT('Ctrl Pts',(-22.0529266054906,-66.0015060728812,
25.2959252805377));
#14224=CARTESIAN_POINT('Ctrl Pts',(-22.0514168805361,-66.0000495912932,
26.0540747194623));
#14225=CARTESIAN_POINT('Ctrl Pts',(-22.0513428634009,-65.6540999925487,
26.0353896065614));
#14226=CARTESIAN_POINT('Ctrl Pts',(-21.8042540993797,-64.6221844734596,
25.9796601209967));
#14227=CARTESIAN_POINT('Ctrl Pts',(-20.1701400827706,-63.5773513899392,
25.8868862627681));
#14228=CARTESIAN_POINT('Ctrl Pts',(-18.0569488868988,-64.5430601781429,
25.7757531447766));
#14229=CARTESIAN_POINT('Ctrl Pts',(-17.7220730992874,-66.842211172105,25.664620026785));
#14230=CARTESIAN_POINT('Ctrl Pts',(-19.4721283107045,-68.3705502400566,
25.5534869087934));
#14231=CARTESIAN_POINT('Ctrl Pts',(-21.55207742503,-67.7732034363132,25.4499718063526));
#14232=CARTESIAN_POINT('Ctrl Pts',(-22.0504073392519,-66.540363708537,25.3835010765755));
#14233=CARTESIAN_POINT('Ctrl Pts',(-22.0554079541519,-65.9981768930466,
25.3540747194623));
#14234=CARTESIAN_POINT('Origin',(-20.,-66.,37.5459252805377));
#14235=CARTESIAN_POINT('',(-22.0555312835971,-66.0018063313406,26.7540747194623));
#14236=CARTESIAN_POINT('',(-22.0542237095723,-65.9981345160623,26.6959252805377));
#14237=CARTESIAN_POINT('',(-22.05475,-65.9999999999998,37.5459252805377));
#14238=CARTESIAN_POINT('Ctrl Pts',(-22.0542237095723,-65.9981345160623,
26.6959252805377));
#14239=CARTESIAN_POINT('Ctrl Pts',(-22.0558088267349,-65.8202139937513,
26.6862824436496));
#14240=CARTESIAN_POINT('Ctrl Pts',(-21.9531907694769,-64.9605855088004,
26.6395952340976));
#14241=CARTESIAN_POINT('Ctrl Pts',(-20.7492058643109,-63.6898348017937,
26.5558636518818));
#14242=CARTESIAN_POINT('Ctrl Pts',(-18.465507605261,-64.1175799233661,26.4447305338903));
#14243=CARTESIAN_POINT('Ctrl Pts',(-17.5862395732934,-66.2681888349264,
26.3335974158987));
#14244=CARTESIAN_POINT('Ctrl Pts',(-18.9161353225687,-68.1733430727544,
26.2224642979071));
#14245=CARTESIAN_POINT('Ctrl Pts',(-21.2380361875332,-68.089363595114,26.1113311799156));
#14246=CARTESIAN_POINT('Ctrl Pts',(-22.0457930405706,-66.7329547828402,
26.0358181741258));
#14247=CARTESIAN_POINT('Ctrl Pts',(-22.0580965462382,-66.0266367280669,
25.9973495409998));
#14248=CARTESIAN_POINT('Ctrl Pts',(-22.058013816727,-66.0004830916995,25.9959252805377));
#14249=CARTESIAN_POINT('Ctrl Pts',(-22.0555312835971,-66.0018063313406,
26.7540747194623));
#14250=CARTESIAN_POINT('Ctrl Pts',(-22.0505008655215,-65.4537399884148,
26.7243225092112));
#14251=CARTESIAN_POINT('Ctrl Pts',(-21.5431051312739,-64.2150554479046,
26.6575259262963));
#14252=CARTESIAN_POINT('Ctrl Pts',(-19.4513023285576,-63.6341803621276,
26.5536849707175));
#14253=CARTESIAN_POINT('Ctrl Pts',(-17.7147940941022,-65.1778050096466,
26.4425518527259));
#14254=CARTESIAN_POINT('Ctrl Pts',(-18.0697955898292,-67.4739347707333,
26.3314187347343));
#14255=CARTESIAN_POINT('Ctrl Pts',(-20.1913974492333,-68.4210616212703,
26.2202856167428));
#14256=CARTESIAN_POINT('Ctrl Pts',(-21.8105645272037,-67.3656512612381,
26.1278376116521));
#14257=CARTESIAN_POINT('Ctrl Pts',(-22.0514896068728,-66.3399661110351,
26.0724339792253));
#14258=CARTESIAN_POINT('Ctrl Pts',(-22.0514168805361,-66.0000495912932,
26.0540747194623));
#14259=CARTESIAN_POINT('Origin',(-20.,-66.,37.5459252805377));
#14260=CARTESIAN_POINT('',(-22.0572927814363,-65.9988171297943,27.4540747194623));
#14261=CARTESIAN_POINT('',(-22.051608611075,-66.0006513925013,27.3959252805377));
#14262=CARTESIAN_POINT('',(-22.05475,-65.9999999999998,37.5459252805377));
#14263=CARTESIAN_POINT('Ctrl Pts',(-22.051608611075,-66.0006513925013,27.3959252805377));
#14264=CARTESIAN_POINT('Ctrl Pts',(-22.0505185829512,-65.6173024522387,
27.3752153462994));
#14265=CARTESIAN_POINT('Ctrl Pts',(-21.7633388641963,-64.5467312818546,
27.3174610393972));
#14266=CARTESIAN_POINT('Ctrl Pts',(-20.0378654071592,-63.5716800778574,
27.2226623598312));
#14267=CARTESIAN_POINT('Ctrl Pts',(-17.9804255504411,-64.6511150930585,
27.1115292418396));
#14268=CARTESIAN_POINT('Ctrl Pts',(-17.7713797576864,-66.9651026482916,
27.0003961238481));
#14269=CARTESIAN_POINT('Ctrl Pts',(-19.602054852468,-68.3957903104112,26.8892630058565));
#14270=CARTESIAN_POINT('Ctrl Pts',(-21.6064981577545,-67.699876740124,26.787772724753));
#14271=CARTESIAN_POINT('Ctrl Pts',(-22.0497193665927,-66.5037217839924,
26.7233268163134));
#14272=CARTESIAN_POINT('Ctrl Pts',(-22.0542237095723,-65.9981345160623,
26.6959252805377));
#14273=CARTESIAN_POINT('Ctrl Pts',(-22.0572927814363,-65.9988171297943,
27.4540747194623));
#14274=CARTESIAN_POINT('Ctrl Pts',(-22.0577689751881,-65.9294336866987,
27.4502997845249));
#14275=CARTESIAN_POINT('Ctrl Pts',(-22.0231033120199,-65.1796547626522,
27.4094804769235));
#14276=CARTESIAN_POINT('Ctrl Pts',(-21.1033854005481,-63.836504637639,27.3316167966584));
#14277=CARTESIAN_POINT('Ctrl Pts',(-18.7808305074767,-63.8995721204905,
27.2204836786668));
#14278=CARTESIAN_POINT('Ctrl Pts',(-17.5741075252728,-65.8850338715259,
27.1093505606753));
#14279=CARTESIAN_POINT('Ctrl Pts',(-18.5876568076359,-67.9757171467262,
26.9982174426837));
#14280=CARTESIAN_POINT('Ctrl Pts',(-20.8938381898737,-68.2581463290383,
26.8870843246921));
#14281=CARTESIAN_POINT('Ctrl Pts',(-21.98355270846,-66.951522387647,26.8057034169517));
#14282=CARTESIAN_POINT('Ctrl Pts',(-22.0567642214294,-66.1361354703139,
26.7613668818751));
#14283=CARTESIAN_POINT('Ctrl Pts',(-22.0555312835971,-66.0018063313406,
26.7540747194623));
#14284=CARTESIAN_POINT('Origin',(-20.,-66.,37.5459252805377));
#14285=CARTESIAN_POINT('',(-22.0519547460626,-65.9989448751757,28.1540747194623));
#14286=CARTESIAN_POINT('',(-22.0566098665172,-66.0015207492701,28.0959252805377));
#14287=CARTESIAN_POINT('',(-22.05475,-65.9999999999998,37.5459252805377));
#14288=CARTESIAN_POINT('Ctrl Pts',(-22.0566098665172,-66.0015207492701,
28.0959252805377));
#14289=CARTESIAN_POINT('Ctrl Pts',(-22.0517667328726,-65.4169498621218,
28.0641482489492));
#14290=CARTESIAN_POINT('Ctrl Pts',(-21.4848825853714,-64.1426999769185,
27.9953268446968));
#14291=CARTESIAN_POINT('Ctrl Pts',(-19.3231871724393,-63.667598701565,27.8894610677806));
#14292=CARTESIAN_POINT('Ctrl Pts',(-17.6733825603793,-65.3035642809691,
27.778327949789));
#14293=CARTESIAN_POINT('Ctrl Pts',(-18.152989804436,-67.5769352415803,27.6671948317974));
#14294=CARTESIAN_POINT('Ctrl Pts',(-20.3230534758781,-68.4070330021147,
27.5560617138059));
#14295=CARTESIAN_POINT('Ctrl Pts',(-21.8481481825977,-67.2899652950944,
27.4656385300526));
#14296=CARTESIAN_POINT('Ctrl Pts',(-22.0524683432725,-66.3030082029172,
27.4122597189632));
#14297=CARTESIAN_POINT('Ctrl Pts',(-22.051608611075,-66.0006513925013,27.3959252805377));
#14298=CARTESIAN_POINT('Ctrl Pts',(-22.0519547460626,-65.9989448751757,
28.1540747194623));
#14299=CARTESIAN_POINT('Ctrl Pts',(-22.0532325567715,-65.7243289273863,
28.1392326871747));
#14300=CARTESIAN_POINT('Ctrl Pts',(-21.8740722613233,-64.7658952750654,
28.0873462822231));
#14301=CARTESIAN_POINT('Ctrl Pts',(-20.4194990521396,-63.6078896201836,
27.9984155046077));
#14302=CARTESIAN_POINT('Ctrl Pts',(-18.2178369745624,-64.3501313764944,
27.8872823866162));
#14303=CARTESIAN_POINT('Ctrl Pts',(-17.6472806432027,-66.6023978352466,
27.7761492686246));
#14304=CARTESIAN_POINT('Ctrl Pts',(-19.2300256691482,-68.3033260850074,
27.665016150633));
#14305=CARTESIAN_POINT('Ctrl Pts',(-21.439781925539,-67.909990145913,27.557657967579));
#14306=CARTESIAN_POINT('Ctrl Pts',(-22.053095967814,-66.6103106197642,27.4873441571887));
#14307=CARTESIAN_POINT('Ctrl Pts',(-22.0572927814363,-65.9988171297943,
27.4540747194623));
#14308=CARTESIAN_POINT('Origin',(-20.,-66.,37.5459252805377));
#14309=CARTESIAN_POINT('',(-22.0534438287596,-66.0017537139889,28.8540747194623));
#14310=CARTESIAN_POINT('',(-22.0563386042488,-65.9983838584325,28.7959252805377));
#14311=CARTESIAN_POINT('',(-22.05475,-65.9999999999998,37.5459252805377));
#14312=CARTESIAN_POINT('Ctrl Pts',(-22.0563386042488,-65.9983838584325,
28.7959252805377));
#14313=CARTESIAN_POINT('Ctrl Pts',(-22.0572597478083,-65.8916548104596,
28.7901255242628));
#14314=CARTESIAN_POINT('Ctrl Pts',(-22.001175176898,-65.1041931970662,28.747281395324));
#14315=CARTESIAN_POINT('Ctrl Pts',(-20.9838411260118,-63.7795883131318,
28.6673928937215));
#14316=CARTESIAN_POINT('Ctrl Pts',(-18.6681747606656,-63.9691349251399,
28.5562597757299));
#14317=CARTESIAN_POINT('Ctrl Pts',(-17.5714472744839,-66.0174091877327,
28.4451266577383));
#14318=CARTESIAN_POINT('Ctrl Pts',(-18.6974268296081,-68.0497498764889,
28.3339935397468));
#14319=CARTESIAN_POINT('Ctrl Pts',(-21.0155726190361,-68.2060788009229,
28.2228604217552));
#14320=CARTESIAN_POINT('Ctrl Pts',(-22.0071593704442,-66.8759492827429,
28.1435043353522));
#14321=CARTESIAN_POINT('Ctrl Pts',(-22.0574126613506,-66.0984188574757,
28.101192621613));
#14322=CARTESIAN_POINT('Ctrl Pts',(-22.0566098665172,-66.0015207492701,
28.0959252805377));
#14323=CARTESIAN_POINT('Ctrl Pts',(-22.0534438287596,-66.0017537139889,
28.8540747194623));
#14324=CARTESIAN_POINT('Ctrl Pts',(-22.0495560850897,-65.5232420578776,
28.8281655898244));
#14325=CARTESIAN_POINT('Ctrl Pts',(-21.644456045474,-64.3546300343245,28.7652120875227));
#14326=CARTESIAN_POINT('Ctrl Pts',(-19.6986309083236,-63.5901559812818,
28.6652142125571));
#14327=CARTESIAN_POINT('Ctrl Pts',(-17.8119536633046,-64.9461381720334,
28.5540810945656));
#14328=CARTESIAN_POINT('Ctrl Pts',(-17.9278625462951,-67.2666561873374,
28.4429479765739));
#14329=CARTESIAN_POINT('Ctrl Pts',(-19.9402731854491,-68.4278806048883,
28.3318148585824));
#14330=CARTESIAN_POINT('Ctrl Pts',(-21.7312864923139,-67.5086939343413,
28.2355237728785));
#14331=CARTESIAN_POINT('Ctrl Pts',(-22.0500432566018,-66.4097455409721,
28.1762770598385));
#14332=CARTESIAN_POINT('Ctrl Pts',(-22.0519547460626,-65.9989448751757,
28.1540747194623));
#14333=CARTESIAN_POINT('Origin',(-20.,-66.,37.5459252805377));
#14334=CARTESIAN_POINT('',(-22.05815424133,-66.0000233771342,29.5540747194623));
#14335=CARTESIAN_POINT('',(-22.0515262960928,-65.9995028191493,29.4959252805377));
#14336=CARTESIAN_POINT('',(-22.05475,-65.9999999999998,37.5459252805377));
#14337=CARTESIAN_POINT('Ctrl Pts',(-22.0515262960928,-65.9995028191493,
29.4959252805377));
#14338=CARTESIAN_POINT('Ctrl Pts',(-22.0522023450635,-65.6872595186681,
29.4790584269126));
#14339=CARTESIAN_POINT('Ctrl Pts',(-21.8385380384052,-64.6901194966521,
29.4251472006236));
#14340=CARTESIAN_POINT('Ctrl Pts',(-20.2885122041186,-63.5885829625528,
29.3341916016708));
#14341=CARTESIAN_POINT('Ctrl Pts',(-18.1305721243274,-64.4497062091094,
29.2230584836793));
#14342=CARTESIAN_POINT('Ctrl Pts',(-17.6836060163159,-66.729719352058,29.1119253656877));
#14343=CARTESIAN_POINT('Ctrl Pts',(-19.3566948545509,-68.3418646225293,
29.0007922476961));
#14344=CARTESIAN_POINT('Ctrl Pts',(-21.5005207642192,-67.8383663168731,
28.8954588859795));
#14345=CARTESIAN_POINT('Ctrl Pts',(-22.0513761927624,-66.5733577027495,
28.8271698969266));
#14346=CARTESIAN_POINT('Ctrl Pts',(-22.0563386042488,-65.9983838584325,
28.7959252805377));
#14347=CARTESIAN_POINT('Ctrl Pts',(-22.0581541126866,-66.0000233762508,
29.5540747194623));
#14348=CARTESIAN_POINT('Ctrl Pts',(-22.0580399559099,-65.3211542304274,
29.5170984924742));
#14349=CARTESIAN_POINT('Ctrl Pts',(-21.3195544042373,-63.961952016278,29.4430778928223));
#14350=CARTESIAN_POINT('Ctrl Pts',(-19.004330572597,-63.784867065997,29.3320129205064));
#14351=CARTESIAN_POINT('Ctrl Pts',(-17.5989620477711,-65.6350503104176,
29.2208798025149));
#14352=CARTESIAN_POINT('Ctrl Pts',(-18.391117960758,-67.8192498750237,29.1097466845233));
#14353=CARTESIAN_POINT('Ctrl Pts',(-20.6557860410391,-68.3384003490309,
28.9986135665318));
#14354=CARTESIAN_POINT('Ctrl Pts',(-21.9322057879489,-67.0952788496883,
28.9133895781781));
#14355=CARTESIAN_POINT('Ctrl Pts',(-22.0551147058285,-66.2074087728823,
28.8652099624883));
#14356=CARTESIAN_POINT('Ctrl Pts',(-22.0534438287596,-66.0017537139889,
28.8540747194623));
#14357=CARTESIAN_POINT('Origin',(-20.,-66.,37.5459252805377));
#14358=CARTESIAN_POINT('',(-22.0535119803991,-65.9982315275897,30.2540747194623));
#14359=CARTESIAN_POINT('',(-22.0545158025659,-66.0018778868973,30.1959252805377));
#14360=CARTESIAN_POINT('',(-22.05475,-65.9999999999998,37.5459252805377));
#14361=CARTESIAN_POINT('Ctrl Pts',(-22.0545158025659,-66.0018778868973,
30.1959252805377));
#14362=CARTESIAN_POINT('Ctrl Pts',(-22.0498372217949,-65.4866536673289,
30.1679913295624));
#14363=CARTESIAN_POINT('Ctrl Pts',(-21.5925294629705,-64.2807662177915,
30.1030130059232));
#14364=CARTESIAN_POINT('Ctrl Pts',(-19.5677488993405,-63.6101610082697,
30.0009903096201));
#14365=CARTESIAN_POINT('Ctrl Pts',(-17.7577727222585,-65.0669468100008,
29.8898571916286));
#14366=CARTESIAN_POINT('Ctrl Pts',(-17.9999712029712,-67.3776996158348,
29.7787240736371));
#14367=CARTESIAN_POINT('Ctrl Pts',(-20.072674759091,-68.4275275075284,29.6675909556455));
#14368=CARTESIAN_POINT('Ctrl Pts',(-21.7743809927857,-67.4334540389223,
29.573324691279));
#14369=CARTESIAN_POINT('Ctrl Pts',(-22.0507175506515,-66.3730339637372,
29.5161027995764));
#14370=CARTESIAN_POINT('Ctrl Pts',(-22.0515262960928,-65.9995028191493,
29.4959252805377));
#14371=CARTESIAN_POINT('Ctrl Pts',(-22.0535119803991,-65.9982315275897,
30.2540747194623));
#14372=CARTESIAN_POINT('Ctrl Pts',(-22.0551803333329,-65.7951106704412,
30.2430757677879));
#14373=CARTESIAN_POINT('Ctrl Pts',(-21.9341785310365,-64.9098242979182,
30.1950324434496));
#14374=CARTESIAN_POINT('Ctrl Pts',(-20.6643636396598,-63.6640221580101,
30.1099447464473));
#14375=CARTESIAN_POINT('Ctrl Pts',(-18.3978055097405,-64.1748577207922,
29.9988116284558));
#14376=CARTESIAN_POINT('Ctrl Pts',(-17.5976388390673,-66.3561353344053,
29.8876785104642));
#14377=CARTESIAN_POINT('Ctrl Pts',(-18.9962076588936,-68.2114638726205,
29.7765453924727));
#14378=CARTESIAN_POINT('Ctrl Pts',(-21.313486738182,-68.0427736322436,29.6654122744811));
#14379=CARTESIAN_POINT('Ctrl Pts',(-22.0575867329659,-66.6826457097529,
29.5912553834776));
#14380=CARTESIAN_POINT('Ctrl Pts',(-22.0581543230729,-66.0012745043528,
29.554142865138));
#14381=CARTESIAN_POINT('Ctrl Pts',(-22.0581541126866,-66.0000233762508,
29.5540747194623));
#14382=CARTESIAN_POINT('Origin',(-20.,-66.,37.5459252805377));
#14383=CARTESIAN_POINT('',(-22.0519163324186,-66.0010204152869,30.9540747194623));
#14384=CARTESIAN_POINT('',(-22.0579001363803,-65.9993455608086,30.8959252805377));
#14385=CARTESIAN_POINT('',(-22.05475,-65.9999999999998,37.5459252805377));
#14386=CARTESIAN_POINT('Ctrl Pts',(-22.0579001363803,-65.9993455608086,
30.8959252805377));
#14387=CARTESIAN_POINT('Ctrl Pts',(-22.058049932207,-65.9634098788375,30.893968604876));
#14388=CARTESIAN_POINT('Ctrl Pts',(-22.0409122080377,-65.2472748593686,
30.8549675565505));
#14389=CARTESIAN_POINT('Ctrl Pts',(-21.207949773882,-63.8930997260919,30.778922135561));
#14390=CARTESIAN_POINT('Ctrl Pts',(-18.8850915735795,-63.8424201935705,
30.6677890175695));
#14391=CARTESIAN_POINT('Ctrl Pts',(-17.582641447505,-65.766442621407,30.556655899578));
#14392=CARTESIAN_POINT('Ctrl Pts',(-18.4926530149794,-67.9042259548608,
30.4455227815864));
#14393=CARTESIAN_POINT('Ctrl Pts',(-20.7822478717438,-68.2991867448226,
30.3343896635948));
#14394=CARTESIAN_POINT('Ctrl Pts',(-21.9603524673483,-67.0194951717011,
30.2511904965786));
#14395=CARTESIAN_POINT('Ctrl Pts',(-22.0560416820867,-66.1699139054527,
30.2050357022262));
#14396=CARTESIAN_POINT('Ctrl Pts',(-22.0545158025659,-66.0018778868973,
30.1959252805377));
#14397=CARTESIAN_POINT('Ctrl Pts',(-22.0519163324186,-66.0010204152869,
30.9540747194623));
#14398=CARTESIAN_POINT('Ctrl Pts',(-22.0500811038091,-65.5927223619752,
30.9320086704376));
#14399=CARTESIAN_POINT('Ctrl Pts',(-21.7342815688762,-64.4963597903545,
30.8728982487491));
#14400=CARTESIAN_POINT('Ctrl Pts',(-19.9491839985917,-63.5719165463332,
30.7767434543967));
#14401=CARTESIAN_POINT('Ctrl Pts',(-17.9325251760105,-64.7257475226081,
30.6656103364052));
#14402=CARTESIAN_POINT('Ctrl Pts',(-17.8081006873606,-67.0458245202808,
30.5544772184136));
#14403=CARTESIAN_POINT('Ctrl Pts',(-19.6897887219546,-68.4087217537406,
30.443344100422));
#14404=CARTESIAN_POINT('Ctrl Pts',(-21.6410622563722,-67.6503619047499,
30.3432099341049));
#14405=CARTESIAN_POINT('Ctrl Pts',(-22.0495613353008,-66.4792199338248,
30.2801201404517));
#14406=CARTESIAN_POINT('Ctrl Pts',(-22.0535119803991,-65.9982315275897,
30.2540747194623));
#14407=CARTESIAN_POINT('Origin',(-20.,-66.,37.5459252805377));
#14408=CARTESIAN_POINT('',(-22.0572361971601,-66.0012177327075,31.6540747194623));
#14409=CARTESIAN_POINT('',(-22.0525866916182,-65.9985364755553,31.5959252805377));
#14410=CARTESIAN_POINT('',(-22.05475,-65.9999999999998,37.5459252805377));
#14411=CARTESIAN_POINT('Ctrl Pts',(-22.0525866916182,-65.9985364755553,
31.5959252805377));
#14412=CARTESIAN_POINT('Ctrl Pts',(-22.0541717763817,-65.7577490902302,
31.5829015075258));
#14413=CARTESIAN_POINT('Ctrl Pts',(-21.9036809516229,-64.8339923497498,
31.53283336185));
#14414=CARTESIAN_POINT('Ctrl Pts',(-20.5360719702046,-63.63128763604,31.4457208435104));
#14415=CARTESIAN_POINT('Ctrl Pts',(-18.3007212782933,-64.2648852353891,
31.3345877255189));
#14416=CARTESIAN_POINT('Ctrl Pts',(-17.6206173554466,-66.4865281607617,
31.2234546075273));
#14417=CARTESIAN_POINT('Ctrl Pts',(-19.1182180804836,-68.2628813638435,
31.1123214895358));
#14418=CARTESIAN_POINT('Ctrl Pts',(-21.3822834251028,-67.9733455779535,
31.0031450472058));
#14419=CARTESIAN_POINT('Ctrl Pts',(-22.0552139525217,-66.6437550279776,
30.9310129775398));
#14420=CARTESIAN_POINT('Ctrl Pts',(-22.0579001363803,-65.9993455608086,
30.8959252805377));
#14421=CARTESIAN_POINT('Ctrl Pts',(-22.0572361971601,-66.0012177327075,
31.6540747194623));
#14422=CARTESIAN_POINT('Ctrl Pts',(-22.0529597533631,-65.3921852245915,
31.6209415730874));
#14423=CARTESIAN_POINT('Ctrl Pts',(-21.4439785259947,-64.0947971370138,
31.5507640540487));
#14424=CARTESIAN_POINT('Ctrl Pts',(-19.2384841459624,-63.6938635929289,
31.4435421623461));
#14425=CARTESIAN_POINT('Ctrl Pts',(-17.6495073099557,-65.3889716553072,
31.3324090443545));
#14426=CARTESIAN_POINT('Ctrl Pts',(-18.2117938983683,-67.6433169085898,
31.221275926363));
#14427=CARTESIAN_POINT('Ctrl Pts',(-20.4107170941006,-68.3936338468077,
31.1101428083714));
#14428=CARTESIAN_POINT('Ctrl Pts',(-21.8717661429505,-67.239207813012,31.0210757394045));
#14429=CARTESIAN_POINT('Ctrl Pts',(-22.0531620764135,-66.2781710903763,
30.9690530431015));
#14430=CARTESIAN_POINT('Ctrl Pts',(-22.0519163324186,-66.0010204152869,
30.9540747194623));
#14431=CARTESIAN_POINT('Origin',(-20.,-66.,37.5459252805377));
#14432=CARTESIAN_POINT('',(-22.0556069266979,-65.9982061756783,32.3540747194623));
#14433=CARTESIAN_POINT('',(-22.0526152608938,-66.0014769892548,32.2959252805377));
#14434=CARTESIAN_POINT('',(-22.05475,-65.9999999999998,37.5459252805377));
#14435=CARTESIAN_POINT('Ctrl Pts',(-22.0526152608939,-66.0014769892548,
32.2959252805377));
#14436=CARTESIAN_POINT('Ctrl Pts',(-22.049653606289,-65.5560934056117,32.2718344101756));
#14437=CARTESIAN_POINT('Ctrl Pts',(-21.6883555136058,-64.4214701158507,
32.2106991671496));
#14438=CARTESIAN_POINT('Ctrl Pts',(-19.8169356466133,-63.578294224532,32.1125195514598));
#14439=CARTESIAN_POINT('Ctrl Pts',(-17.8661543709335,-64.8403128647219,
32.0013864334682));
#14440=CARTESIAN_POINT('Ctrl Pts',(-17.8683526023209,-67.163722815959,31.8902533154767));
#14441=CARTESIAN_POINT('Ctrl Pts',(-19.8215184328882,-68.4220478423468,
31.7791201974851));
#14442=CARTESIAN_POINT('Ctrl Pts',(-21.690001156166,-67.5759383023312,31.6810108525055));
#14443=CARTESIAN_POINT('Ctrl Pts',(-22.0496632157189,-66.4426364593967,
31.6199458801897));
#14444=CARTESIAN_POINT('Ctrl Pts',(-22.0525866916182,-65.9985364755553,
31.5959252805377));
#14445=CARTESIAN_POINT('Ctrl Pts',(-22.0556069266979,-65.9982061756783,
32.3540747194623));
#14446=CARTESIAN_POINT('Ctrl Pts',(-22.0568133671517,-65.8664001586089,
32.3469188484011));
#14447=CARTESIAN_POINT('Ctrl Pts',(-21.9852145475282,-65.0535687993885,
32.302718604676));
#14448=CARTESIAN_POINT('Ctrl Pts',(-20.9021196384422,-63.7451492994194,
32.221473988287));
#14449=CARTESIAN_POINT('Ctrl Pts',(-18.594917279486,-64.0191128067246,32.1103408702954));
#14450=CARTESIAN_POINT('Ctrl Pts',(-17.5737019298616,-66.106062240275,31.9992077523039));
#14451=CARTESIAN_POINT('Ctrl Pts',(-18.7731300721891,-68.0959393369569,
31.8880746343123));
#14452=CARTESIAN_POINT('Ctrl Pts',(-21.095437861579,-68.1675302570873,31.7769415163208));
#14453=CARTESIAN_POINT('Ctrl Pts',(-22.0216974673029,-66.8254194714185,
31.6989415447041));
#14454=CARTESIAN_POINT('Ctrl Pts',(-22.057741013069,-66.0731114167429,31.6579859457513));
#14455=CARTESIAN_POINT('Ctrl Pts',(-22.0572361971601,-66.0012177327075,
31.6540747194623));
#14456=CARTESIAN_POINT('Origin',(-20.,-66.,37.5459252805377));
#14457=CARTESIAN_POINT('',(-22.0514188637225,-65.9999091152567,33.0540747194623));
#14458=CARTESIAN_POINT('',(-22.0579172481639,-66.0006320364424,32.9959252805377));
#14459=CARTESIAN_POINT('',(-22.05475,-65.9999999999998,37.5459252805377));
#14460=CARTESIAN_POINT('Ctrl Pts',(-22.0579172481639,-66.0006320364424,
32.9959252805377));
#14461=CARTESIAN_POINT('Ctrl Pts',(-22.055307383354,-65.3549463154049,32.9607673128254));
#14462=CARTESIAN_POINT('Ctrl Pts',(-21.3800044998465,-64.0242259372538,
32.8885649724492));
#14463=CARTESIAN_POINT('Ctrl Pts',(-19.1139377351588,-63.7387912340402,
32.7793182594091));
#14464=CARTESIAN_POINT('Ctrl Pts',(-17.6197009851889,-65.5179750831086,
32.6681851414176));
#14465=CARTESIAN_POINT('Ctrl Pts',(-18.3040075812308,-67.7383271084264,
32.557052023426));
#14466=CARTESIAN_POINT('Ctrl Pts',(-20.5405531925411,-68.3676937442268,
32.4459189054345));
#14467=CARTESIAN_POINT('Ctrl Pts',(-21.9047825486759,-67.1633756004897,
32.358876657805));
#14468=CARTESIAN_POINT('Ctrl Pts',(-22.0542077230658,-66.2409568083382,
32.3088787828394));
#14469=CARTESIAN_POINT('Ctrl Pts',(-22.0526152608939,-66.0014769892548,
32.2959252805377));
#14470=CARTESIAN_POINT('Ctrl Pts',(-22.0514188637225,-65.9999091152567,
33.0540747194623));
#14471=CARTESIAN_POINT('Ctrl Pts',(-22.0515519905893,-65.6625169941898,
33.0358517510508));
#14472=CARTESIAN_POINT('Ctrl Pts',(-21.8131840852274,-64.6394379208522,
32.9805844099755));
#14473=CARTESIAN_POINT('Ctrl Pts',(-20.2002808122731,-63.5796572308245,
32.8882726962363));
#14474=CARTESIAN_POINT('Ctrl Pts',(-18.0752183512995,-64.5189911786904,
32.7771395782448));
#14475=CARTESIAN_POINT('Ctrl Pts',(-17.7117918139106,-66.8138026917249,
32.6660064602532));
#14476=CARTESIAN_POINT('Ctrl Pts',(-19.442623471414,-68.3637899503476,32.5548733422617));
#14477=CARTESIAN_POINT('Ctrl Pts',(-21.5392921623106,-67.789843471444,32.4508960953313));
#14478=CARTESIAN_POINT('Ctrl Pts',(-22.0505678899225,-66.5487309571744,
32.3839632210649));
#14479=CARTESIAN_POINT('Ctrl Pts',(-22.0556069266979,-65.9982061756783,
32.3540747194623));
#14480=CARTESIAN_POINT('Origin',(-20.,-66.,37.5459252805377));
#14481=CARTESIAN_POINT('',(-22.0552733614683,-66.0018413365206,33.7540747194623));
#14482=CARTESIAN_POINT('',(-22.0544769775149,-65.99812289348,33.6959252805377));
#14483=CARTESIAN_POINT('',(-22.05475,-65.9999999999998,37.5459252805377));
#14484=CARTESIAN_POINT('Ctrl Pts',(-22.0544769775149,-65.99812289348,33.6959252805377));
#14485=CARTESIAN_POINT('Ctrl Pts',(-22.0560114585337,-65.8287826123771,
33.686744588139));
#14486=CARTESIAN_POINT('Ctrl Pts',(-21.9594169044098,-64.9778761409694,
33.6405195230764));
#14487=CARTESIAN_POINT('Ctrl Pts',(-20.7778958486438,-63.6993371678323,
33.5572500853501));
#14488=CARTESIAN_POINT('Ctrl Pts',(-18.4890524532058,-64.0986297225616,
33.4461169673585));
#14489=CARTESIAN_POINT('Ctrl Pts',(-17.5830877228631,-66.2381311930787,
33.334983849367));
#14490=CARTESIAN_POINT('Ctrl Pts',(-18.8891762373197,-68.159685622601,33.2238507313753));
#14491=CARTESIAN_POINT('Ctrl Pts',(-21.2119343809668,-68.1046107660899,
33.1127176133838));
#14492=CARTESIAN_POINT('Ctrl Pts',(-22.0415655539315,-66.7501146853756,
33.0367424631046));
#14493=CARTESIAN_POINT('Ctrl Pts',(-22.0580572807716,-66.0352763808272,
32.9978116854892));
#14494=CARTESIAN_POINT('Ctrl Pts',(-22.0579172481639,-66.0006320364424,
32.9959252805377));
#14495=CARTESIAN_POINT('Ctrl Pts',(-22.0552733614683,-66.0018413365206,
33.7540747194623));
#14496=CARTESIAN_POINT('Ctrl Pts',(-22.0502920767718,-65.4621140092977,
33.7247846537006));
#14497=CARTESIAN_POINT('Ctrl Pts',(-21.5559212661831,-64.2316956472682,
33.6584502152751));
#14498=CARTESIAN_POINT('Ctrl Pts',(-19.4807858227571,-63.6275354235162,
33.5550714041857));
#14499=CARTESIAN_POINT('Ctrl Pts',(-17.7252024818967,-65.1494309100778,
33.4439382861942));
#14500=CARTESIAN_POINT('Ctrl Pts',(-18.0516033664323,-67.4498007037218,
33.3328051682026));
#14501=CARTESIAN_POINT('Ctrl Pts',(-20.1612535373157,-68.4232558307668,
33.221672050211));
#14502=CARTESIAN_POINT('Ctrl Pts',(-21.8015900775427,-67.3829020390902,
33.1287619006309));
#14503=CARTESIAN_POINT('Ctrl Pts',(-22.0512813650165,-66.3483810743131,
33.0728961237147));
#14504=CARTESIAN_POINT('Ctrl Pts',(-22.0514188637225,-65.9999091152567,
33.0540747194623));
#14505=CARTESIAN_POINT('Origin',(-20.,-66.,37.5459252805377));
#14506=CARTESIAN_POINT('',(-22.0574743887429,-65.9989407171765,34.4540747194623));
#14507=CARTESIAN_POINT('',(-22.0515358806555,-66.000517785455,34.3959252805377));
#14508=CARTESIAN_POINT('',(-22.05475,-65.9999999999998,37.5459252805377));
#14509=CARTESIAN_POINT('Ctrl Pts',(-22.0515358806555,-66.000517785455,34.3959252805377));
#14510=CARTESIAN_POINT('Ctrl Pts',(-22.050690498549,-65.6256901339794,34.3756774907888));
#14511=CARTESIAN_POINT('Ctrl Pts',(-21.7729353091241,-64.5639295587311,
34.318385328376));
#14512=CARTESIAN_POINT('Ctrl Pts',(-20.0680811526701,-63.5723393435572,
34.2240487932995));
#14513=CARTESIAN_POINT('Ctrl Pts',(-17.9973678404257,-64.6260873816269,
34.1129156753078));
#14514=CARTESIAN_POINT('Ctrl Pts',(-17.7595423005167,-66.9372943668669,
34.0017825573163));
#14515=CARTESIAN_POINT('Ctrl Pts',(-19.5722718322054,-68.3906526348572,
33.8906494393247));
#14516=CARTESIAN_POINT('Ctrl Pts',(-21.5943860795634,-67.7166817852802,
33.7886970137319));
#14517=CARTESIAN_POINT('Ctrl Pts',(-22.0498197810177,-66.5120757898144,
33.7237889608028));
#14518=CARTESIAN_POINT('Ctrl Pts',(-22.0544769775149,-65.99812289348,33.6959252805377));
#14519=CARTESIAN_POINT('Ctrl Pts',(-22.0574743887429,-65.9989407171765,
34.4540747194623));
#14520=CARTESIAN_POINT('Ctrl Pts',(-22.0578567862954,-65.9380656581726,
34.4507619290143));
#14521=CARTESIAN_POINT('Ctrl Pts',(-22.0277962110148,-65.1968548676797,
34.4104047659024));
#14522=CARTESIAN_POINT('Ctrl Pts',(-21.1302229793561,-63.8504031421106,
34.3330032301266));
#14523=CARTESIAN_POINT('Ctrl Pts',(-18.8070632766386,-63.8845630078765,
34.221870112135));
#14524=CARTESIAN_POINT('Ctrl Pts',(-17.5757260074789,-65.8548543331223,
34.1107369941435));
#14525=CARTESIAN_POINT('Ctrl Pts',(-18.5631798196893,-67.9579885544186,
33.9996038761519));
#14526=CARTESIAN_POINT('Ctrl Pts',(-20.8656679609891,-68.2690946508119,
33.8884707581604));
#14527=CARTESIAN_POINT('Ctrl Pts',(-21.977838232828,-66.968790137621,33.8066277059305));
#14528=CARTESIAN_POINT('Ctrl Pts',(-22.0565921161143,-66.1447297606308,
33.7618290263645));
#14529=CARTESIAN_POINT('Ctrl Pts',(-22.0552733614683,-66.0018413365206,
33.7540747194623));
#14530=CARTESIAN_POINT('Origin',(-20.,-66.,37.5459252805377));
#14531=CARTESIAN_POINT('',(-22.0520911128174,-65.9988355264336,35.1540747194623));
#14532=CARTESIAN_POINT('',(-22.0563749241962,-66.0016062120012,35.0959252805377));
#14533=CARTESIAN_POINT('',(-22.05475,-65.9999999999998,37.5459252805377));
#14534=CARTESIAN_POINT('Ctrl Pts',(-22.0563749241962,-66.0016062120012,
35.0959252805377));
#14535=CARTESIAN_POINT('Ctrl Pts',(-22.0514251626832,-65.4253659758576,
35.0646103934386));
#14536=CARTESIAN_POINT('Ctrl Pts',(-21.4984704660108,-64.1591280998276,
34.9962511336756));
#14537=CARTESIAN_POINT('Ctrl Pts',(-19.3522645237931,-63.6593583355034,
34.8908475012488));
#14538=CARTESIAN_POINT('Ctrl Pts',(-17.6822294077865,-65.2746643974708,
34.7797143832572));
#14539=CARTESIAN_POINT('Ctrl Pts',(-18.1335089795993,-67.5538288003781,
34.6685812652656));
#14540=CARTESIAN_POINT('Ctrl Pts',(-20.2930746903084,-68.4108665986726,
34.5574481472741));
#14541=CARTESIAN_POINT('Ctrl Pts',(-21.8398174471696,-67.3072525302986,
34.4665628190314));
#14542=CARTESIAN_POINT('Ctrl Pts',(-22.0522371685899,-66.3114565992663,
34.4127218634526));
#14543=CARTESIAN_POINT('Ctrl Pts',(-22.0515358806555,-66.000517785455,34.3959252805377));
#14544=CARTESIAN_POINT('Ctrl Pts',(-22.0520911128174,-65.9988355264336,
35.1540747194623));
#14545=CARTESIAN_POINT('Ctrl Pts',(-22.0534711048112,-65.7328124009057,
35.1396948316641));
#14546=CARTESIAN_POINT('Ctrl Pts',(-21.8818113373711,-64.7831882718686,
35.088270571202));
#14547=CARTESIAN_POINT('Ctrl Pts',(-20.4492273324997,-63.61330436034,34.9998019380759));
#14548=CARTESIAN_POINT('Ctrl Pts',(-18.2385100652431,-64.3280768123671,
34.8886688200844));
#14549=CARTESIAN_POINT('Ctrl Pts',(-17.6399645748577,-66.5730756011264,
34.7775357020929));
#14550=CARTESIAN_POINT('Ctrl Pts',(-19.2014229874425,-68.2935648037488,
34.6664025841013));
#14551=CARTESIAN_POINT('Ctrl Pts',(-21.4254342373654,-67.9261851342807,
34.5585822565578));
#14552=CARTESIAN_POINT('Ctrl Pts',(-22.0535807303049,-66.618784347459,34.4878063016781));
#14553=CARTESIAN_POINT('Ctrl Pts',(-22.0574743887429,-65.9989407171765,
34.4540747194623));
#14554=CARTESIAN_POINT('Origin',(-20.,-66.,37.5459252805377));
#14555=CARTESIAN_POINT('',(-22.0526726878338,-66.0023207051531,35.8540747194623));
#14556=CARTESIAN_POINT('',(-22.0565720193282,-65.9985037223956,35.7959252805377));
#14557=CARTESIAN_POINT('',(-22.05475,-65.9999999999998,37.5459252805377));
#14558=CARTESIAN_POINT('',(-20.5301702171886,-67.9851743256717,36.));
#14559=CARTESIAN_POINT('Ctrl Pts',(-20.5301702171885,-67.9851743256717,
36.));
#14560=CARTESIAN_POINT('Ctrl Pts',(-21.190259562418,-67.8088876857537,35.9629556273362));
#14561=CARTESIAN_POINT('Ctrl Pts',(-21.9249294223933,-67.1127898537559,
35.9143138671569));
#14562=CARTESIAN_POINT('Ctrl Pts',(-22.0542897540197,-66.2165895473215,
35.8656721069777));
#14563=CARTESIAN_POINT('Ctrl Pts',(-22.0526726878338,-66.0023207051531,
35.8540747194623));
#14564=CARTESIAN_POINT('',(-19.4686890762993,-67.9887317545258,36.));
#14565=CARTESIAN_POINT('Origin',(-20.,-66.,36.));
#14566=CARTESIAN_POINT('Ctrl Pts',(-19.4686883835207,-67.9887339150381,
36.));
#14567=CARTESIAN_POINT('Ctrl Pts',(-20.1132089071786,-68.1600296783296,
35.9636818543909));
#14568=CARTESIAN_POINT('Ctrl Pts',(-21.4929690160207,-67.8407342776925,
35.8956569479035));
#14569=CARTESIAN_POINT('Ctrl Pts',(-22.0517191488996,-66.5816759129075,
35.8276320414161));
#14570=CARTESIAN_POINT('Ctrl Pts',(-22.0565720193282,-65.9985037223956,
35.7959252805377));
#14571=CARTESIAN_POINT('Origin',(20.,-66.,30.));
#14572=CARTESIAN_POINT('',(18.3313536394157,-66.0003916926001,25.7714803633902));
#14573=CARTESIAN_POINT('',(18.3334666271624,-65.9985218536523,25.5785196366098));
#14574=CARTESIAN_POINT('',(18.334,-66.,30.));
#14575=CARTESIAN_POINT('',(19.2300979593295,-67.4774325188554,25.));
#14576=CARTESIAN_POINT('Ctrl Pts',(18.3334666271624,-65.9985218536523,25.5785196366098));
#14577=CARTESIAN_POINT('Ctrl Pts',(18.3324169745748,-65.8847145132893,25.5709016210591));
#14578=CARTESIAN_POINT('Ctrl Pts',(18.3430836686143,-65.7711020898156,25.5632836055085));
#14579=CARTESIAN_POINT('Ctrl Pts',(18.3661914671125,-65.6600764989809,25.5556655899578));
#14580=CARTESIAN_POINT('Ctrl Pts',(18.478558512482,-65.1201887375622,25.5186212172939));
#14581=CARTESIAN_POINT('Ctrl Pts',(18.8851100097676,-64.6414696565181,25.4815768446301));
#14582=CARTESIAN_POINT('Ctrl Pts',(19.3995346321509,-64.4430321483538,25.4445324719662));
#14583=CARTESIAN_POINT('Ctrl Pts',(19.9139592545342,-64.2445946401895,25.4074880993024));
#14584=CARTESIAN_POINT('Ctrl Pts',(20.5362570020153,-64.326438704905,25.3704437266385));
#14585=CARTESIAN_POINT('Ctrl Pts',(20.9821827720363,-64.6510268476224,25.3333993539747));
#14586=CARTESIAN_POINT('Ctrl Pts',(21.4281085420573,-64.9756149903398,25.2963549813108));
#14587=CARTESIAN_POINT('Ctrl Pts',(21.6976623346182,-65.5429472110592,25.259310608647));
#14588=CARTESIAN_POINT('Ctrl Pts',(21.6664135658646,-66.0935811418539,25.2222662359831));
#14589=CARTESIAN_POINT('Ctrl Pts',(21.635164797111,-66.6442150726486,25.1852218633193));
#14590=CARTESIAN_POINT('Ctrl Pts',(21.3031134670429,-67.1781507135186,25.1481774906554));
#14591=CARTESIAN_POINT('Ctrl Pts',(20.8246618488694,-67.4504550129278,25.1111331179916));
#14592=CARTESIAN_POINT('Ctrl Pts',(20.3462102306959,-67.722759312337,25.0740887453277));
#14593=CARTESIAN_POINT('Ctrl Pts',(19.7213583244171,-67.7334322702853,25.0370443726639));
#14594=CARTESIAN_POINT('Ctrl Pts',(19.2300979593295,-67.4774325188554,25.));
#14595=CARTESIAN_POINT('',(18.6629739733599,-65.0009969633526,25.));
#14596=CARTESIAN_POINT('Origin',(20.,-66.,25.));
#14597=CARTESIAN_POINT('',(18.3354783848229,-66.0012211146297,25.0714803633902));
#14598=CARTESIAN_POINT('Ctrl Pts',(18.6629725546621,-65.0009957901906,25.));
#14599=CARTESIAN_POINT('Ctrl Pts',(18.4510073215875,-65.2854499389498,25.0238267877967));
#14600=CARTESIAN_POINT('Ctrl Pts',(18.3378311125484,-65.6440627071064,25.0476535755935));
#14601=CARTESIAN_POINT('Ctrl Pts',(18.3354783848229,-66.0012211146297,25.0714803633902));
#14602=CARTESIAN_POINT('',(18.334,-66.,24.));
#14603=CARTESIAN_POINT('',(18.334,-66.,30.));
#14604=CARTESIAN_POINT('Origin',(20.,-66.,24.));
#14605=CARTESIAN_POINT('Ctrl Pts',(18.3354783848229,-66.0012211146297,25.0714803633902));
#14606=CARTESIAN_POINT('Ctrl Pts',(18.3342449510884,-66.1884638727438,25.0839717212025));
#14607=CARTESIAN_POINT('Ctrl Pts',(18.363470829549,-66.3753069066835,25.0964630790149));
#14608=CARTESIAN_POINT('Ctrl Pts',(18.4248900596206,-66.5508551769228,25.1089544368272));
#14609=CARTESIAN_POINT('Ctrl Pts',(18.607034937838,-67.0714611543465,25.1459988094911));
#14610=CARTESIAN_POINT('Ctrl Pts',(19.0723133986938,-67.4927321215424,25.1830431821549));
#14611=CARTESIAN_POINT('Ctrl Pts',(19.6082884916208,-67.6221190201672,25.2200875548188));
#14612=CARTESIAN_POINT('Ctrl Pts',(20.1442635845478,-67.751505918792,25.2571319274826));
#14613=CARTESIAN_POINT('Ctrl Pts',(20.7509353095461,-67.5890087488456,25.2941763001465));
#14614=CARTESIAN_POINT('Ctrl Pts',(21.1504371531331,-67.2088726584111,25.3312206728103));
#14615=CARTESIAN_POINT('Ctrl Pts',(21.54993899672,-66.8287365679766,25.3682650454742));
#14616=CARTESIAN_POINT('Ctrl Pts',(21.7422709588957,-66.230961557054,25.405309418138));
#14617=CARTESIAN_POINT('Ctrl Pts',(21.6395392404303,-65.6891597889306,25.4423537908019));
#14618=CARTESIAN_POINT('Ctrl Pts',(21.5368075219649,-65.1473580208071,25.4793981634657));
#14619=CARTESIAN_POINT('Ctrl Pts',(21.1390121228584,-64.6615294954828,25.5164425361296));
#14620=CARTESIAN_POINT('Ctrl Pts',(20.6281313212479,-64.453969540756,25.5534869087934));
#14621=CARTESIAN_POINT('Ctrl Pts',(20.1172505196373,-64.2464095860292,25.5905312814573));
#14622=CARTESIAN_POINT('Ctrl Pts',(19.4932843155229,-64.3171182018999,25.6275756541212));
#14623=CARTESIAN_POINT('Ctrl Pts',(19.0418023782432,-64.6337524622506,25.664620026785));
#14624=CARTESIAN_POINT('Ctrl Pts',(18.6076787555033,-64.9382129529964,25.7002401389867));
#14625=CARTESIAN_POINT('Ctrl Pts',(18.3330312172753,-65.4700522046137,25.7358602511885));
#14626=CARTESIAN_POINT('Ctrl Pts',(18.3313536394157,-66.0003916926001,25.7714803633902));
#14627=CARTESIAN_POINT('Origin',(20.,-66.,30.));
#14628=CARTESIAN_POINT('',(18.3344266756531,-65.9984874576763,26.4714803633902));
#14629=CARTESIAN_POINT('',(18.3367026517093,-66.000040209255,26.2785196366098));
#14630=CARTESIAN_POINT('',(18.334,-66.,30.));
#14631=CARTESIAN_POINT('Ctrl Pts',(18.3367026517093,-66.000040209255,26.2785196366098));
#14632=CARTESIAN_POINT('Ctrl Pts',(18.3367626645399,-65.7195428345507,26.2598345237089));
#14633=CARTESIAN_POINT('Ctrl Pts',(18.4039333309142,-65.4390183287806,26.241149410808));
#14634=CARTESIAN_POINT('Ctrl Pts',(18.5380532069523,-65.1953424610818,26.2224642979072));
#14635=CARTESIAN_POINT('Ctrl Pts',(18.8039540177177,-64.7122402341857,26.1854199252433));
#14636=CARTESIAN_POINT('Ctrl Pts',(19.3330018695053,-64.3739733253295,26.1483755525794));
#14637=CARTESIAN_POINT('Ctrl Pts',(19.8830898278916,-64.3353399906558,26.1113311799156));
#14638=CARTESIAN_POINT('Ctrl Pts',(20.433177786278,-64.296706655982,26.0742868072517));
#14639=CARTESIAN_POINT('Ctrl Pts',(21.0043058512631,-64.5577068954906,26.0372424345879));
#14640=CARTESIAN_POINT('Ctrl Pts',(21.3351230048638,-64.9989005442132,26.000198061924));
#14641=CARTESIAN_POINT('Ctrl Pts',(21.6659401584645,-65.4400941929357,25.9631536892602));
#14642=CARTESIAN_POINT('Ctrl Pts',(21.7564464006808,-66.0614812508722,25.9261093165963));
#14643=CARTESIAN_POINT('Ctrl Pts',(21.5652075003073,-66.578705400814,25.8890649439325));
#14644=CARTESIAN_POINT('Ctrl Pts',(21.3739685999339,-67.0959295507558,25.8520205712686));
#14645=CARTESIAN_POINT('Ctrl Pts',(20.9009845569708,-67.508990792703,25.8149761986048));
#14646=CARTESIAN_POINT('Ctrl Pts',(20.3627356556273,-67.6288589318993,25.7779318259409));
#14647=CARTESIAN_POINT('Ctrl Pts',(19.8244867542837,-67.7487270710955,25.7408874532771));
#14648=CARTESIAN_POINT('Ctrl Pts',(19.2209729945597,-67.575402107541,25.7038430806132));
#14649=CARTESIAN_POINT('Ctrl Pts',(18.8283074114245,-67.188211404867,25.6667987079494));
#14650=CARTESIAN_POINT('Ctrl Pts',(18.5163918127925,-66.88064480113,25.6373723508362));
#14651=CARTESIAN_POINT('Ctrl Pts',(18.3375211544446,-66.4381291788607,25.607945993723));
#14652=CARTESIAN_POINT('Ctrl Pts',(18.3334666271624,-65.9985218536523,25.5785196366098));
#14653=CARTESIAN_POINT('Ctrl Pts',(18.3313536394157,-66.0003916926001,25.7714803633902));
#14654=CARTESIAN_POINT('Ctrl Pts',(18.331286561923,-66.0215971722449,25.7729046238523));
#14655=CARTESIAN_POINT('Ctrl Pts',(18.3316559029049,-66.0428002541,25.7743288843144));
#14656=CARTESIAN_POINT('Ctrl Pts',(18.3324689176524,-66.0639863067127,25.7757531447766));
#14657=CARTESIAN_POINT('Ctrl Pts',(18.3536150647863,-66.6150259859933,25.8127975174404));
#14658=CARTESIAN_POINT('Ctrl Pts',(18.674905029499,-67.1545454397239,25.8498418901043));
#14659=CARTESIAN_POINT('Ctrl Pts',(19.1493178612708,-67.4356536527718,25.8868862627681));
#14660=CARTESIAN_POINT('Ctrl Pts',(19.6237306930425,-67.7167618658197,25.923930635432));
#14661=CARTESIAN_POINT('Ctrl Pts',(20.2512663918733,-67.7394588381849,25.9609750080958));
#14662=CARTESIAN_POINT('Ctrl Pts',(20.7447484303696,-67.4933561307171,25.9980193807597));
#14663=CARTESIAN_POINT('Ctrl Pts',(21.2382304688658,-67.2472534232492,26.0350637534235));
#14664=CARTESIAN_POINT('Ctrl Pts',(21.5976588470276,-66.7323510359483,26.0721081260874));
#14665=CARTESIAN_POINT('Ctrl Pts',(21.6585539923065,-66.1842793662227,26.1091524987512));
#14666=CARTESIAN_POINT('Ctrl Pts',(21.7194491375853,-65.636207696497,26.1461968714151));
#14667=CARTESIAN_POINT('Ctrl Pts',(21.4818110499811,-65.0549667443465,26.1832412440789));
#14668=CARTESIAN_POINT('Ctrl Pts',(21.0543866287213,-64.7065433408633,26.2202856167428));
#14669=CARTESIAN_POINT('Ctrl Pts',(20.6269622074615,-64.3581199373801,26.2573299894066));
#14670=CARTESIAN_POINT('Ctrl Pts',(20.0097514525462,-64.2425140825642,26.2943743620705));
#14671=CARTESIAN_POINT('Ctrl Pts',(19.4852026366556,-64.4126295250552,26.3314187347344));
#14672=CARTESIAN_POINT('Ctrl Pts',(18.960653820765,-64.5827449675462,26.3684631073982));
#14673=CARTESIAN_POINT('Ctrl Pts',(18.5287669438991,-65.0385817073442,26.4055074800621));
#14674=CARTESIAN_POINT('Ctrl Pts',(18.3871816973018,-65.5715397639926,26.4425518527259));
#14675=CARTESIAN_POINT('Ctrl Pts',(18.3503263440991,-65.7102714319599,26.452194689614));
#14676=CARTESIAN_POINT('Ctrl Pts',(18.3331414559104,-65.8542287411456,26.4618375265021));
#14677=CARTESIAN_POINT('Ctrl Pts',(18.3344266756531,-65.9984874576763,26.4714803633902));
#14678=CARTESIAN_POINT('Origin',(20.,-66.,30.));
#14679=CARTESIAN_POINT('',(18.3365470086803,-66.0005281518116,27.1714803633902));
#14680=CARTESIAN_POINT('',(18.3333666774615,-66.0014645809704,26.9785196366098));
#14681=CARTESIAN_POINT('',(18.334,-66.,30.));
#14682=CARTESIAN_POINT('Ctrl Pts',(18.3333666774615,-66.0014645809704,26.9785196366098));
#14683=CARTESIAN_POINT('Ctrl Pts',(18.3374453613588,-65.5570901083669,26.9487674263587));
#14684=CARTESIAN_POINT('Ctrl Pts',(18.5206885203257,-65.1097460475429,26.9190152161076));
#14685=CARTESIAN_POINT('Ctrl Pts',(18.8387597416989,-64.8015503031277,26.8892630058565));
#14686=CARTESIAN_POINT('Ctrl Pts',(19.2347891041815,-64.4178168623791,26.8522186331927));
#14687=CARTESIAN_POINT('Ctrl Pts',(19.8398377304009,-64.2498002251426,26.8151742605288));
#14688=CARTESIAN_POINT('Ctrl Pts',(20.3770233944236,-64.374388121695,26.7781298878649));
#14689=CARTESIAN_POINT('Ctrl Pts',(20.9142090584462,-64.4989760182474,26.7410855152011));
#14690=CARTESIAN_POINT('Ctrl Pts',(21.3835317602721,-64.9161684485887,26.7040411425372));
#14691=CARTESIAN_POINT('Ctrl Pts',(21.5702203295955,-65.435049925312,26.6669967698734));
#14692=CARTESIAN_POINT('Ctrl Pts',(21.7569088989189,-65.9539314020353,26.6299523972095));
#14693=CARTESIAN_POINT('Ctrl Pts',(21.6609633357398,-66.5745019251406,26.5929080245457));
#14694=CARTESIAN_POINT('Ctrl Pts',(21.3262899503724,-67.0127762524406,26.5558636518818));
#14695=CARTESIAN_POINT('Ctrl Pts',(20.9916165650051,-67.4510505797406,26.518819279218));
#14696=CARTESIAN_POINT('Ctrl Pts',(20.4182153574495,-67.7070287112352,26.4817749065541));
#14697=CARTESIAN_POINT('Ctrl Pts',(19.8684865381395,-67.6635699328358,26.4447305338903));
#14698=CARTESIAN_POINT('Ctrl Pts',(19.3187577188295,-67.6201111544364,26.4076861612264));
#14699=CARTESIAN_POINT('Ctrl Pts',(18.7927012877651,-67.2772154661431,26.3706417885626));
#14700=CARTESIAN_POINT('Ctrl Pts',(18.5310499571044,-66.7917988495284,26.3335974158987));
#14701=CARTESIAN_POINT('Ctrl Pts',(18.4013750725946,-66.5512254744963,26.3152381561357));
#14702=CARTESIAN_POINT('Ctrl Pts',(18.3366436854535,-66.2756459383905,26.2968788963728));
#14703=CARTESIAN_POINT('Ctrl Pts',(18.3367026517093,-66.000040209255,26.2785196366098));
#14704=CARTESIAN_POINT('Ctrl Pts',(18.3344266756531,-65.9984874576763,26.4714803633902));
#14705=CARTESIAN_POINT('Ctrl Pts',(18.3380788161142,-66.4084197657567,26.498881899166));
#14706=CARTESIAN_POINT('Ctrl Pts',(18.4908762665155,-66.8207859249028,26.5262834349417));
#14707=CARTESIAN_POINT('Ctrl Pts',(18.7652754263391,-67.1225936158832,26.5536849707175));
#14708=CARTESIAN_POINT('Ctrl Pts',(19.1362380183026,-67.5306100376265,26.5907293433813));
#14709=CARTESIAN_POINT('Ctrl Pts',(19.7294468185584,-67.7365635076143,26.6277737160452));
#14710=CARTESIAN_POINT('Ctrl Pts',(20.2734377447371,-67.6462056352892,26.664818088709));
#14711=CARTESIAN_POINT('Ctrl Pts',(20.8174286709158,-67.5558477629641,26.7018624613729));
#14712=CARTESIAN_POINT('Ctrl Pts',(21.3122017230173,-67.1691785483262,26.7389068340367));
#14713=CARTESIAN_POINT('Ctrl Pts',(21.5313390460231,-66.6631454483979,26.7759512067006));
#14714=CARTESIAN_POINT('Ctrl Pts',(21.7504763690289,-66.1571123484697,26.8129955793644));
#14715=CARTESIAN_POINT('Ctrl Pts',(21.693977962939,-65.5317153632511,26.8500399520283));
#14716=CARTESIAN_POINT('Ctrl Pts',(21.3876985948801,-65.0731484534342,26.8870843246922));
#14717=CARTESIAN_POINT('Ctrl Pts',(21.0814192268212,-64.6145815436172,26.924128697356));
#14718=CARTESIAN_POINT('Ctrl Pts',(20.5253588967934,-64.322844709202,26.9611730700199));
#14719=CARTESIAN_POINT('Ctrl Pts',(19.9739817626904,-64.3314424706716,26.9982174426837));
#14720=CARTESIAN_POINT('Ctrl Pts',(19.4226046285874,-64.3400402321411,27.0352618153476));
#14721=CARTESIAN_POINT('Ctrl Pts',(18.8759106904092,-64.6489725894954,27.0723061880114));
#14722=CARTESIAN_POINT('Ctrl Pts',(18.5840778492301,-65.1168660144091,27.1093505606753));
#14723=CARTESIAN_POINT('Ctrl Pts',(18.4209265116641,-65.3784453411378,27.1300604949136));
#14724=CARTESIAN_POINT('Ctrl Pts',(18.3374308081207,-65.689707199922,27.1507704291519));
#14725=CARTESIAN_POINT('Ctrl Pts',(18.3365470086803,-66.0005281518116,27.1714803633902));
#14726=CARTESIAN_POINT('Origin',(20.,-66.,30.));
#14727=CARTESIAN_POINT('',(18.3324919694882,-66.0012330299788,27.8714803633902));
#14728=CARTESIAN_POINT('',(18.3319384476764,-65.9990409239126,27.6785196366098));
#14729=CARTESIAN_POINT('',(18.334,-66.,30.));
#14730=CARTESIAN_POINT('Ctrl Pts',(18.3319384476764,-65.9990409239126,27.6785196366098));
#14731=CARTESIAN_POINT('Ctrl Pts',(18.3315523477999,-65.9427845393862,27.6747447016724));
#14732=CARTESIAN_POINT('Ctrl Pts',(18.3341516652356,-65.886564255334,27.6709697667349));
#14733=CARTESIAN_POINT('Ctrl Pts',(18.3398540050594,-65.8306604882018,27.6671948317974));
#14734=CARTESIAN_POINT('Ctrl Pts',(18.395812479838,-65.2820629581077,27.6301504591336));
#14735=CARTESIAN_POINT('Ctrl Pts',(18.7505915016711,-64.7639459555085,27.5931060864697));
#14736=CARTESIAN_POINT('Ctrl Pts',(19.241837208723,-64.5134100171528,27.5560617138058));
#14737=CARTESIAN_POINT('Ctrl Pts',(19.7330829157748,-64.262874078797,27.519017341142));
#14738=CARTESIAN_POINT('Ctrl Pts',(20.3607953080454,-64.2799192046846,27.4819729684782));
#14739=CARTESIAN_POINT('Ctrl Pts',(20.8377208404994,-64.5567452099326,27.4449285958143));
#14740=CARTESIAN_POINT('Ctrl Pts',(21.3146463729533,-64.8335712151806,27.4078842231505));
#14741=CARTESIAN_POINT('Ctrl Pts',(21.6407850455905,-65.370178099789,27.3708398504866));
#14742=CARTESIAN_POINT('Ctrl Pts',(21.6668893856045,-65.9210039927054,27.3337954778227));
#14743=CARTESIAN_POINT('Ctrl Pts',(21.6929937256185,-66.4718298856219,27.2967511051589));
#14744=CARTESIAN_POINT('Ctrl Pts',(21.4190637330094,-67.0368747868466,27.259706732495));
#14745=CARTESIAN_POINT('Ctrl Pts',(20.970455159021,-67.3575630302712,27.2226623598312));
#14746=CARTESIAN_POINT('Ctrl Pts',(20.5218465850326,-67.6782512736958,27.1856179871673));
#14747=CARTESIAN_POINT('Ctrl Pts',(19.898559429665,-67.7545828593205,27.1485736145035));
#14748=CARTESIAN_POINT('Ctrl Pts',(19.3858221698857,-67.5516269500416,27.1115292418396));
#14749=CARTESIAN_POINT('Ctrl Pts',(18.8730849101064,-67.3486710407626,27.0744848691758));
#14750=CARTESIAN_POINT('Ctrl Pts',(18.4708975459154,-66.8664276365802,27.0374404965119));
#14751=CARTESIAN_POINT('Ctrl Pts',(18.3633089131928,-66.3255808123586,27.0003961238481));
#14752=CARTESIAN_POINT('Ctrl Pts',(18.3421301557416,-66.2191154412634,26.9931039614353));
#14753=CARTESIAN_POINT('Ctrl Pts',(18.3323670063393,-66.1103792061011,26.9858117990226));
#14754=CARTESIAN_POINT('Ctrl Pts',(18.3333666774615,-66.0014645809704,26.9785196366098));
#14755=CARTESIAN_POINT('Ctrl Pts',(18.3365470086803,-66.0005281518116,27.1714803633902));
#14756=CARTESIAN_POINT('Ctrl Pts',(18.3358499341568,-66.2456803402052,27.1878148018157));
#14757=CARTESIAN_POINT('Ctrl Pts',(18.3865446335564,-66.4905582462458,27.2041492402413));
#14758=CARTESIAN_POINT('Ctrl Pts',(18.4900816163634,-66.7105685406344,27.2204836786668));
#14759=CARTESIAN_POINT('Ctrl Pts',(18.7248899688559,-67.209523149473,27.2575280513307));
#14760=CARTESIAN_POINT('Ctrl Pts',(19.231478418021,-67.5805778746772,27.2945724239945));
#14761=CARTESIAN_POINT('Ctrl Pts',(19.7780221189842,-67.6539307712373,27.3316167966584));
#14762=CARTESIAN_POINT('Ctrl Pts',(20.3245658199475,-67.7272836677973,27.3686611693222));
#14763=CARTESIAN_POINT('Ctrl Pts',(20.911064772709,-67.5029347357133,27.4057055419861));
#14764=CARTESIAN_POINT('Ctrl Pts',(21.2691255147861,-67.0835504616866,27.4427499146499));
#14765=CARTESIAN_POINT('Ctrl Pts',(21.6271862568631,-66.66416618766,27.4797942873138));
#14766=CARTESIAN_POINT('Ctrl Pts',(21.7568087882558,-66.0497465716907,27.5168386599777));
#14767=CARTESIAN_POINT('Ctrl Pts',(21.5986752874074,-65.5214621215884,27.5538830326415));
#14768=CARTESIAN_POINT('Ctrl Pts',(21.4405417865591,-64.993177671486,27.5909274053054));
#14769=CARTESIAN_POINT('Ctrl Pts',(20.9946522534698,-64.5510283872504,27.6279717779692));
#14770=CARTESIAN_POINT('Ctrl Pts',(20.4650545136244,-64.3973504828203,27.6650161506331));
#14771=CARTESIAN_POINT('Ctrl Pts',(19.935456773779,-64.2436725783903,27.7020605232969));
#14772=CARTESIAN_POINT('Ctrl Pts',(19.3221508271775,-64.3784660537657,27.7391048959608));
#14773=CARTESIAN_POINT('Ctrl Pts',(18.9057975446667,-64.7400467618753,27.7761492686246));
#14774=CARTESIAN_POINT('Ctrl Pts',(18.548645554798,-65.0502142922492,27.8079263002132));
#14775=CARTESIAN_POINT('Ctrl Pts',(18.3364188028544,-65.5272604673683,27.8397033318017));
#14776=CARTESIAN_POINT('Ctrl Pts',(18.3324919694882,-66.0012330299788,27.8714803633902));
#14777=CARTESIAN_POINT('Origin',(20.,-66.,30.));
#14778=CARTESIAN_POINT('',(18.3327119100896,-65.9986896255405,28.5714803633902));
#14779=CARTESIAN_POINT('',(18.3362665489809,-65.9991445003998,28.3785196366098));
#14780=CARTESIAN_POINT('',(18.334,-66.,30.));
#14781=CARTESIAN_POINT('Ctrl Pts',(18.3362665489809,-65.9991445003998,28.3785196366098));
#14782=CARTESIAN_POINT('Ctrl Pts',(18.3352304947382,-65.7764847466224,28.3636776043221));
#14783=CARTESIAN_POINT('Ctrl Pts',(18.3767830304293,-65.5541958268257,28.3488355720344));
#14784=CARTESIAN_POINT('Ctrl Pts',(18.4627526639626,-65.3506686340066,28.3339935397468));
#14785=CARTESIAN_POINT('Ctrl Pts',(18.6773251079956,-64.8426831349939,28.2969491670829));
#14786=CARTESIAN_POINT('Ctrl Pts',(19.1685967650093,-64.451575039978,28.2599047944191));
#14787=CARTESIAN_POINT('Ctrl Pts',(19.7117520566309,-64.3563231101692,28.2228604217552));
#14788=CARTESIAN_POINT('Ctrl Pts',(20.2549073482526,-64.2610711803603,28.1858160490914));
#14789=CARTESIAN_POINT('Ctrl Pts',(20.849946274482,-64.4616754157586,28.1487716764275));
#14790=CARTESIAN_POINT('Ctrl Pts',(21.2245673124077,-64.8663353703955,28.1117273037637));
#14791=CARTESIAN_POINT('Ctrl Pts',(21.5991883503334,-65.2709953250324,28.0746829310998));
#14792=CARTESIAN_POINT('Ctrl Pts',(21.7533914999553,-65.8797109989079,28.0376385584359));
#14793=CARTESIAN_POINT('Ctrl Pts',(21.6166103653521,-66.4139221202436,28.0005941857721));
#14794=CARTESIAN_POINT('Ctrl Pts',(21.4798292307489,-66.9481332415792,27.9635498131082));
#14795=CARTESIAN_POINT('Ctrl Pts',(21.0520638119205,-67.407839810375,27.9265054404444));
#14796=CARTESIAN_POINT('Ctrl Pts',(20.5290679827964,-67.5826710538235,27.8894610677805));
#14797=CARTESIAN_POINT('Ctrl Pts',(20.0060721536723,-67.757502297272,27.8524166951167));
#14798=CARTESIAN_POINT('Ctrl Pts',(19.3878459142524,-67.6474582153731,27.8153723224528));
#14799=CARTESIAN_POINT('Ctrl Pts',(18.9573017584045,-67.3028971456291,27.778327949789));
#14800=CARTESIAN_POINT('Ctrl Pts',(18.5706313695867,-66.9934479033162,27.7450585120626));
#14801=CARTESIAN_POINT('Ctrl Pts',(18.3353412416341,-66.4948423914134,27.7117890743362));
#14802=CARTESIAN_POINT('Ctrl Pts',(18.3319384476764,-65.9990409239126,27.6785196366098));
#14803=CARTESIAN_POINT('Ctrl Pts',(18.3324919694882,-66.0012330299788,27.8714803633902));
#14804=CARTESIAN_POINT('Ctrl Pts',(18.3318410600215,-66.079798428407,27.8767477044655));
#14805=CARTESIAN_POINT('Ctrl Pts',(18.3369134350028,-66.1582793757284,27.8820150455408));
#14806=CARTESIAN_POINT('Ctrl Pts',(18.3479977301881,-66.2359018357232,27.8872823866162));
#14807=CARTESIAN_POINT('Ctrl Pts',(18.4259518166406,-66.7818082606177,27.92432675928));
#14808=CARTESIAN_POINT('Ctrl Pts',(18.8012606079657,-67.285253169563,27.9613711319439));
#14809=CARTESIAN_POINT('Ctrl Pts',(19.3021754152326,-67.515850264519,27.9984155046078));
#14810=CARTESIAN_POINT('Ctrl Pts',(19.8030902224995,-67.746447359475,28.0354598772716));
#14811=CARTESIAN_POINT('Ctrl Pts',(20.4296110457082,-67.7041966404415,28.0725042499354));
#14812=CARTESIAN_POINT('Ctrl Pts',(20.8950296263565,-67.4084328679382,28.1095486225993));
#14813=CARTESIAN_POINT('Ctrl Pts',(21.3604482070047,-67.112669095435,28.1465929952631));
#14814=CARTESIAN_POINT('Ctrl Pts',(21.6647645450926,-66.5633922694618,28.183637367927));
#14815=CARTESIAN_POINT('Ctrl Pts',(21.66871749542,-66.0119622752448,28.2206817405909));
#14816=CARTESIAN_POINT('Ctrl Pts',(21.6726704457474,-65.4605322810278,28.2577261132547));
#14817=CARTESIAN_POINT('Ctrl Pts',(21.3762600083143,-64.906949118567,28.2947704859186));
#14818=CARTESIAN_POINT('Ctrl Pts',(20.9151294325926,-64.6045433374158,28.3318148585824));
#14819=CARTESIAN_POINT('Ctrl Pts',(20.4539988568709,-64.3021375562647,28.3688592312463));
#14820=CARTESIAN_POINT('Ctrl Pts',(19.8281481428606,-64.2509091564231,28.4059036039101));
#14821=CARTESIAN_POINT('Ctrl Pts',(19.3239788939139,-64.4743012618234,28.442947976574));
#14822=CARTESIAN_POINT('Ctrl Pts',(18.8198096449673,-64.6976933672236,28.4799923492378));
#14823=CARTESIAN_POINT('Ctrl Pts',(18.4373218610842,-65.1957059778656,28.5170367219017));
#14824=CARTESIAN_POINT('Ctrl Pts',(18.3515494794562,-65.7404387223271,28.5540810945655));
#14825=CARTESIAN_POINT('Ctrl Pts',(18.3381207486454,-65.8257233938074,28.5598808508404));
#14826=CARTESIAN_POINT('Ctrl Pts',(18.3319650429721,-65.912153259319,28.5656806071153));
#14827=CARTESIAN_POINT('Ctrl Pts',(18.3327119100896,-65.9986896255405,28.5714803633902));
#14828=CARTESIAN_POINT('Origin',(20.,-66.,30.));
#14829=CARTESIAN_POINT('',(18.3366137500186,-65.9995968836509,29.2714803633902));
#14830=CARTESIAN_POINT('',(18.3350591945307,-66.0014219186036,29.0785196366098));
#14831=CARTESIAN_POINT('',(18.334,-66.,30.));
#14832=CARTESIAN_POINT('Ctrl Pts',(18.3350591945307,-66.0014219186036,29.0785196366098));
#14833=CARTESIAN_POINT('Ctrl Pts',(18.338211393284,-65.613442675639,29.0526105069719));
#14834=CARTESIAN_POINT('Ctrl Pts',(18.4733910015055,-65.2234834061788,29.026701377334));
#14835=CARTESIAN_POINT('Ctrl Pts',(18.7211705029757,-64.9279199131777,29.0007922476961));
#14836=CARTESIAN_POINT('Ctrl Pts',(19.0754408439409,-64.5053289449133,28.9637478750323));
#14837=CARTESIAN_POINT('Ctrl Pts',(19.6598960790816,-64.2757086908116,28.9267035023684));
#14838=CARTESIAN_POINT('Ctrl Pts',(20.2070779908308,-64.344137898032,28.8896591297046));
#14839=CARTESIAN_POINT('Ctrl Pts',(20.7542599025799,-64.4125671052524,28.8526147570407));
#14840=CARTESIAN_POINT('Ctrl Pts',(21.2641684909374,-64.779045773795,28.8155703843769));
#14841=CARTESIAN_POINT('Ctrl Pts',(21.5034595509674,-65.2758660527047,28.778526011713));
#14842=CARTESIAN_POINT('Ctrl Pts',(21.7427506109974,-65.7726863316144,28.7414816390492));
#14843=CARTESIAN_POINT('Ctrl Pts',(21.7114241426998,-66.3998482208912,28.7044372663853));
#14844=CARTESIAN_POINT('Ctrl Pts',(21.423815754467,-66.8703500975764,28.6673928937214));
#14845=CARTESIAN_POINT('Ctrl Pts',(21.1362073662343,-67.3408519742616,28.6303485210576));
#14846=CARTESIAN_POINT('Ctrl Pts',(20.5923170580665,-67.6546938383551,28.5933041483937));
#14847=CARTESIAN_POINT('Ctrl Pts',(20.041039738637,-67.6682554765002,28.5562597757299));
#14848=CARTESIAN_POINT('Ctrl Pts',(19.4897624192075,-67.6818171146452,28.519215403066));
#14849=CARTESIAN_POINT('Ctrl Pts',(18.9310980885164,-67.3950985268418,28.4821710304022));
#14850=CARTESIAN_POINT('Ctrl Pts',(18.6207025386969,-66.9393077814354,28.4451266577383));
#14851=CARTESIAN_POINT('Ctrl Pts',(18.434668678416,-66.6661321128486,28.4229243173622));
#14852=CARTESIAN_POINT('Ctrl Pts',(18.3378163925938,-66.3322233905155,28.400721976986));
#14853=CARTESIAN_POINT('Ctrl Pts',(18.3362665489809,-65.9991445003998,28.3785196366098));
#14854=CARTESIAN_POINT('Ctrl Pts',(18.3327119100896,-65.9986896255405,28.5714803633902));
#14855=CARTESIAN_POINT('Ctrl Pts',(18.3367354544376,-66.4648808649886,28.6027249797792));
#14856=CARTESIAN_POINT('Ctrl Pts',(18.5410871126712,-66.9341629934405,28.6339695961681));
#14857=CARTESIAN_POINT('Ctrl Pts',(18.8878468637807,-67.2441368803895,28.6652142125571));
#14858=CARTESIAN_POINT('Ctrl Pts',(19.2989736091057,-67.6116494157094,28.702258585221));
#14859=CARTESIAN_POINT('Ctrl Pts',(19.9102840791284,-67.755221608068,28.7393029578848));
#14860=CARTESIAN_POINT('Ctrl Pts',(20.4420305722938,-67.609151996769,28.7763473305487));
#14861=CARTESIAN_POINT('Ctrl Pts',(20.9737770654591,-67.4630823854699,28.8133917032125));
#14862=CARTESIAN_POINT('Ctrl Pts',(21.4259595817671,-67.0273709705132,28.8504360758764));
#14863=CARTESIAN_POINT('Ctrl Pts',(21.5916505028899,-66.5014078701001,28.8874804485402));
#14864=CARTESIAN_POINT('Ctrl Pts',(21.7573414240127,-65.9754447696869,28.9245248212041));
#14865=CARTESIAN_POINT('Ctrl Pts',(21.6365407499503,-65.3592299838174,28.9615691938679));
#14866=CARTESIAN_POINT('Ctrl Pts',(21.2845292464878,-64.9347555254941,28.9986135665318));
#14867=CARTESIAN_POINT('Ctrl Pts',(20.9325177430254,-64.5102810671709,29.0356579391956));
#14868=CARTESIAN_POINT('Ctrl Pts',(20.3492954101628,-64.277546936394,29.0727023118595));
#14869=CARTESIAN_POINT('Ctrl Pts',(19.8017562651217,-64.3430568515699,29.1097466845233));
#14870=CARTESIAN_POINT('Ctrl Pts',(19.2542171200805,-64.4085667667459,29.1467910571872));
#14871=CARTESIAN_POINT('Ctrl Pts',(18.7423611628609,-64.7723207278747,29.183835429851));
#14872=CARTESIAN_POINT('Ctrl Pts',(18.5004237527135,-65.2678577637357,29.2208798025149));
#14873=CARTESIAN_POINT('Ctrl Pts',(18.3902660529079,-65.4934831434804,29.23774665614));
#14874=CARTESIAN_POINT('Ctrl Pts',(18.3360656066366,-65.746428687046,29.2546135097651));
#14875=CARTESIAN_POINT('Ctrl Pts',(18.3366137500186,-65.9995968836509,29.2714803633902));
#14876=CARTESIAN_POINT('Origin',(20.,-66.,30.));
#14877=CARTESIAN_POINT('',(18.33418984545,-66.0015225986866,29.9714803633902));
#14878=CARTESIAN_POINT('',(18.3312399724094,-66.0000189542779,29.7785196366098));
#14879=CARTESIAN_POINT('',(18.334,-66.,30.));
#14880=CARTESIAN_POINT('Ctrl Pts',(18.3312400767123,-66.0000189535616,29.7785196366098));
#14881=CARTESIAN_POINT('Ctrl Pts',(18.3313326355021,-65.4495890237892,29.7415434096217));
#14882=CARTESIAN_POINT('Ctrl Pts',(18.6304405935465,-64.8990729061442,29.7045671826336));
#14883=CARTESIAN_POINT('Ctrl Pts',(19.0923261693912,-64.599682603033,29.6675909556455));
#14884=CARTESIAN_POINT('Ctrl Pts',(19.5550629814828,-64.2997405358241,29.6305465829816));
#14885=CARTESIAN_POINT('Ctrl Pts',(20.1811779492479,-64.2518507653313,29.5935022103178));
#14886=CARTESIAN_POINT('Ctrl Pts',(20.6841485416147,-64.4779285929935,29.5564578376539));
#14887=CARTESIAN_POINT('Ctrl Pts',(21.1871191339814,-64.7040064206556,29.5194134649901));
#14888=CARTESIAN_POINT('Ctrl Pts',(21.5669453509498,-65.2040518464729,29.4823690923262));
#14889=CARTESIAN_POINT('Ctrl Pts',(21.6498112407281,-65.7492342427931,29.4453247196624));
#14890=CARTESIAN_POINT('Ctrl Pts',(21.7326771305064,-66.2944166391133,29.4082803469985));
#14891=CARTESIAN_POINT('Ctrl Pts',(21.5185826930945,-66.8847360059365,29.3712359743346));
#14892=CARTESIAN_POINT('Ctrl Pts',(21.1055017563896,-67.2500505836325,29.3341916016708));
#14893=CARTESIAN_POINT('Ctrl Pts',(20.6924208196846,-67.6153651613285,29.2971472290069));
#14894=CARTESIAN_POINT('Ctrl Pts',(20.0803533836867,-67.7556749498972,29.2601028563431));
#14895=CARTESIAN_POINT('Ctrl Pts',(19.5493935524781,-67.6067714288199,29.2230584836792));
#14896=CARTESIAN_POINT('Ctrl Pts',(19.0184337212696,-67.4578679077427,29.1860141110154));
#14897=CARTESIAN_POINT('Ctrl Pts',(18.5685814948505,-67.0197510770193,29.1489697383515));
#14898=CARTESIAN_POINT('Ctrl Pts',(18.4056981050357,-66.4929118204442,29.1119253656877));
#14899=CARTESIAN_POINT('Ctrl Pts',(18.3567366569113,-66.3345481410045,29.1007901226617));
#14900=CARTESIAN_POINT('Ctrl Pts',(18.3337044404468,-66.1681678965589,29.0896548796358));
#14901=CARTESIAN_POINT('Ctrl Pts',(18.3350591945307,-66.0014219186036,29.0785196366098));
#14902=CARTESIAN_POINT('Ctrl Pts',(18.3366137500186,-65.9995968836509,29.2714803633902));
#14903=CARTESIAN_POINT('Ctrl Pts',(18.3372694842635,-66.3024575250332,29.2916578824289));
#14904=CARTESIAN_POINT('Ctrl Pts',(18.416275455694,-66.6056368032707,29.3118354014677));
#14905=CARTESIAN_POINT('Ctrl Pts',(18.5715624445679,-66.8627440673682,29.3320129205064));
#14906=CARTESIAN_POINT('Ctrl Pts',(18.8566574096448,-67.3347732245466,29.3690572931703));
#14907=CARTESIAN_POINT('Ctrl Pts',(19.3988662028737,-67.6515114283102,29.4061016658342));
#14908=CARTESIAN_POINT('Ctrl Pts',(19.9500634099081,-67.6680130432697,29.443146038498));
#14909=CARTESIAN_POINT('Ctrl Pts',(20.5012606169424,-67.6845146582292,29.4801904111619));
#14910=CARTESIAN_POINT('Ctrl Pts',(21.0614462377821,-67.4007796843847,29.5172347838257));
#14911=CARTESIAN_POINT('Ctrl Pts',(21.3742683079854,-66.9466508296172,29.5542791564896));
#14912=CARTESIAN_POINT('Ctrl Pts',(21.6870903781887,-66.4925219748497,29.5913235291534));
#14913=CARTESIAN_POINT('Ctrl Pts',(21.7525488977555,-65.8679992391592,29.6283679018173));
#14914=CARTESIAN_POINT('Ctrl Pts',(21.540688759921,-65.3588765168854,29.6654122744811));
#14915=CARTESIAN_POINT('Ctrl Pts',(21.3288286220865,-64.8497537946116,29.702456647145));
#14916=CARTESIAN_POINT('Ctrl Pts',(20.8396498268506,-64.4560310857545,29.7395010198088));
#14917=CARTESIAN_POINT('Ctrl Pts',(20.2970102178582,-64.3578836502745,29.7765453924727));
#14918=CARTESIAN_POINT('Ctrl Pts',(19.7543706088658,-64.2597362147945,29.8135897651365));
#14919=CARTESIAN_POINT('Ctrl Pts',(19.1582701861169,-64.4571640526916,29.8506341378004));
#14920=CARTESIAN_POINT('Ctrl Pts',(18.7814962342033,-64.8598203000021,29.8876785104643));
#14921=CARTESIAN_POINT('Ctrl Pts',(18.4973833084148,-65.1634502190276,29.9156124614396));
#14922=CARTESIAN_POINT('Ctrl Pts',(18.3379832586462,-65.5837766092154,29.9435464124149));
#14923=CARTESIAN_POINT('Ctrl Pts',(18.33418984545,-66.0015225986866,29.9714803633902));
#14924=CARTESIAN_POINT('Origin',(20.,-66.,30.));
#14925=CARTESIAN_POINT('',(18.3314458131932,-65.999469377919,30.6714803633902));
#14926=CARTESIAN_POINT('',(18.3350039368976,-65.9985661152072,30.4785196366098));
#14927=CARTESIAN_POINT('',(18.334,-66.,30.));
#14928=CARTESIAN_POINT('Ctrl Pts',(18.3350039368976,-65.9985661152072,30.4785196366098));
#14929=CARTESIAN_POINT('Ctrl Pts',(18.333651229393,-65.8338748785772,30.4675206849353));
#14930=CARTESIAN_POINT('Ctrl Pts',(18.3561120724071,-65.6695444482994,30.4565217332609));
#14931=CARTESIAN_POINT('Ctrl Pts',(18.4038998375659,-65.5129426455764,30.4455227815864));
#14932=CARTESIAN_POINT('Ctrl Pts',(18.5648486110225,-64.9855091490396,30.4084784089225));
#14933=CARTESIAN_POINT('Ctrl Pts',(19.0130899030193,-64.5457442946841,30.3714340362587));
#14934=CARTESIAN_POINT('Ctrl Pts',(19.5434996770359,-64.3948931343509,30.3343896635948));
#14935=CARTESIAN_POINT('Ctrl Pts',(20.0739094510525,-64.2440419740177,30.297345290931));
#14936=CARTESIAN_POINT('Ctrl Pts',(20.6864877070889,-64.3821045077068,30.2603009182671));
#14937=CARTESIAN_POINT('Ctrl Pts',(21.1009065797602,-64.745900602958,30.2232565456033));
#14938=CARTESIAN_POINT('Ctrl Pts',(21.5153254524316,-65.1096966982092,30.1862121729394));
#14939=CARTESIAN_POINT('Ctrl Pts',(21.7315849417379,-65.6992263550224,30.1491678002755));
#14940=CARTESIAN_POINT('Ctrl Pts',(21.6507204494273,-66.2447092006093,30.1121234276117));
#14941=CARTESIAN_POINT('Ctrl Pts',(21.5698559571167,-66.7901920461962,30.0750790549479));
#14942=CARTESIAN_POINT('Ctrl Pts',(21.1918674831892,-67.2916280805568,30.038034682284));
#14943=CARTESIAN_POINT('Ctrl Pts',(20.6897299920547,-67.5195503062027,30.0009903096202));
#14944=CARTESIAN_POINT('Ctrl Pts',(20.1875925009203,-67.7474725318485,29.9639459369563));
#14945=CARTESIAN_POINT('Ctrl Pts',(19.5613059925788,-67.7018809487796,29.9269015642924));
#14946=CARTESIAN_POINT('Ctrl Pts',(19.0974714984457,-67.403639162642,29.8898571916286));
#14947=CARTESIAN_POINT('Ctrl Pts',(18.6327837488041,-67.104848740191,29.852744673289));
#14948=CARTESIAN_POINT('Ctrl Pts',(18.3311471767583,-66.5524777230817,29.8156321549494));
#14949=CARTESIAN_POINT('Ctrl Pts',(18.3312400767123,-66.0000189535616,29.7785196366098));
#14950=CARTESIAN_POINT('Ctrl Pts',(18.33418984545,-66.0015225986866,29.9714803633902));
#14951=CARTESIAN_POINT('Ctrl Pts',(18.332952655842,-66.1377669175135,29.9805907850787));
#14952=CARTESIAN_POINT('Ctrl Pts',(18.3482670799087,-66.2737367634984,29.9897012067673));
#14953=CARTESIAN_POINT('Ctrl Pts',(18.3812048568464,-66.4052942882035,29.9988116284558));
#14954=CARTESIAN_POINT('Ctrl Pts',(18.5151349124813,-66.9402273723704,30.0358560011197));
#14955=CARTESIAN_POINT('Ctrl Pts',(18.940442504829,-67.4022088839804,30.0729003737835));
#14956=CARTESIAN_POINT('Ctrl Pts',(19.4624985096596,-67.5798269916133,30.1099447464474));
#14957=CARTESIAN_POINT('Ctrl Pts',(19.9845545144902,-67.7574450992461,30.1469891191112));
#14958=CARTESIAN_POINT('Ctrl Pts',(20.6033589318036,-67.6506998029017,30.1840334917751));
#14959=CARTESIAN_POINT('Ctrl Pts',(21.0357346822848,-67.3084398509142,30.2210778644389));
#14960=CARTESIAN_POINT('Ctrl Pts',(21.4681104327661,-66.9661798989267,30.2581222371028));
#14961=CARTESIAN_POINT('Ctrl Pts',(21.7140575164153,-66.3884052912962,30.2951666097666));
#14962=CARTESIAN_POINT('Ctrl Pts',(21.6610257075631,-65.8395170589677,30.3322109824305));
#14963=CARTESIAN_POINT('Ctrl Pts',(21.6079938987109,-65.2906288266393,30.3692553550943));
#14964=CARTESIAN_POINT('Ctrl Pts',(21.2559831973573,-64.770626969613,30.4062997277582));
#14965=CARTESIAN_POINT('Ctrl Pts',(20.7660806279449,-64.517474571201,30.443344100422));
#14966=CARTESIAN_POINT('Ctrl Pts',(20.2761780585324,-64.264322172789,30.4803884730859));
#14967=CARTESIAN_POINT('Ctrl Pts',(19.648383621061,-64.2780192329911,30.5174328457497));
#14968=CARTESIAN_POINT('Ctrl Pts',(19.1699884049918,-64.5522977075035,30.5544772184136));
#14969=CARTESIAN_POINT('Ctrl Pts',(18.6915931889226,-64.8265761820158,30.5915215910775));
#14970=CARTESIAN_POINT('Ctrl Pts',(18.3625971942555,-65.3614360708382,30.6285659637413));
#14971=CARTESIAN_POINT('Ctrl Pts',(18.3335554627283,-65.9121149629056,30.6656103364052));
#14972=CARTESIAN_POINT('Ctrl Pts',(18.3320214848211,-65.941201701539,30.6675670120669));
#14973=CARTESIAN_POINT('Ctrl Pts',(18.3313243580995,-65.9703325740729,30.6695236877285));
#14974=CARTESIAN_POINT('Ctrl Pts',(18.3314458131932,-65.999469377919,30.6714803633902));
#14975=CARTESIAN_POINT('Origin',(20.,-66.,30.));
#14976=CARTESIAN_POINT('',(18.3357539768147,-65.9988133681531,31.3714803633902));
#14977=CARTESIAN_POINT('',(18.3362976949234,-66.000827356963,31.1785196366098));
#14978=CARTESIAN_POINT('',(18.334,-66.,30.));
#14979=CARTESIAN_POINT('Ctrl Pts',(18.3362976949234,-66.000827356963,31.1785196366098));
#14980=CARTESIAN_POINT('Ctrl Pts',(18.3377857059205,-65.6697775954689,31.1564535875851));
#14981=CARTESIAN_POINT('Ctrl Pts',(18.4333703169726,-65.3379360998736,31.1343875385604));
#14982=CARTESIAN_POINT('Ctrl Pts',(18.6172645337012,-65.0657606167262,31.1123214895358));
#14983=CARTESIAN_POINT('Ctrl Pts',(18.9259852243695,-64.6088337778346,31.0752771168719));
#14984=CARTESIAN_POINT('Ctrl Pts',(19.4835935249369,-64.3200668023759,31.0382327442081));
#14985=CARTESIAN_POINT('Ctrl Pts',(20.0349169034394,-64.3316051411987,31.0011883715442));
#14986=CARTESIAN_POINT('Ctrl Pts',(20.5862402819419,-64.3431434800215,30.9641439988803));
#14987=CARTESIAN_POINT('Ctrl Pts',(21.1312787383795,-64.6549871331258,30.9270996262165));
#14988=CARTESIAN_POINT('Ctrl Pts',(21.420611948834,-65.1244303078278,30.8900552535526));
#14989=CARTESIAN_POINT('Ctrl Pts',(21.7099451592885,-65.5938734825299,30.8530108808888));
#14990=CARTESIAN_POINT('Ctrl Pts',(21.7435731237599,-66.2209161788296,30.8159665082249));
#14991=CARTESIAN_POINT('Ctrl Pts',(21.5061070239143,-66.7186113188203,30.7789221355611));
#14992=CARTESIAN_POINT('Ctrl Pts',(21.2686409240686,-67.2163064588109,30.7418777628972));
#14993=CARTESIAN_POINT('Ctrl Pts',(20.7600807599058,-67.5846540424924,30.7048333902334));
#14994=CARTESIAN_POINT('Ctrl Pts',(20.2131536709134,-67.6550909665624,30.6677890175695));
#14995=CARTESIAN_POINT('Ctrl Pts',(19.6662265819209,-67.7255278906324,30.6307446449057));
#14996=CARTESIAN_POINT('Ctrl Pts',(19.0809325680987,-67.4980541550909,30.5937002722418));
#14997=CARTESIAN_POINT('Ctrl Pts',(18.7251136886458,-67.0767662179611,30.556655899578));
#14998=CARTESIAN_POINT('Ctrl Pts',(18.4749420203221,-66.7805640989547,30.5306104785886));
#14999=CARTESIAN_POINT('Ctrl Pts',(18.3382071363911,-66.3885535174836,30.5045650575992));
#15000=CARTESIAN_POINT('Ctrl Pts',(18.3350039368976,-65.9985661152072,30.4785196366098));
#15001=CARTESIAN_POINT('Ctrl Pts',(18.3314458131932,-65.999469377919,30.6714803633902));
#15002=CARTESIAN_POINT('Ctrl Pts',(18.3336237824952,-66.5219593158195,30.7065680603924));
#15003=CARTESIAN_POINT('Ctrl Pts',(18.599030994634,-67.0463565704791,30.7416557573945));
#15004=CARTESIAN_POINT('Ctrl Pts',(19.0223181515937,-67.352368063378,30.7767434543967));
#15005=CARTESIAN_POINT('Ctrl Pts',(19.4692100403736,-67.6754443764704,30.8137878270606));
#15006=CARTESIAN_POINT('Ctrl Pts',(20.0920812863208,-67.755099107343,30.8508321997244));
#15007=CARTESIAN_POINT('Ctrl Pts',(20.6058937493031,-67.5548806835585,30.8878765723883));
#15008=CARTESIAN_POINT('Ctrl Pts',(21.1197062122855,-67.354662259774,30.9249209450521));
#15009=CARTESIAN_POINT('Ctrl Pts',(21.524459892303,-66.8745706813325,30.961965317716));
#15010=CARTESIAN_POINT('Ctrl Pts',(21.6349315399048,-66.334305302639,30.9990096903798));
#15011=CARTESIAN_POINT('Ctrl Pts',(21.7454031875066,-65.7940399239454,31.0360540630437));
#15012=CARTESIAN_POINT('Ctrl Pts',(21.5615928026928,-65.1936007449999,31.0730984357075));
#15013=CARTESIAN_POINT('Ctrl Pts',(21.1676156349072,-64.8077605506157,31.1101428083714));
#15014=CARTESIAN_POINT('Ctrl Pts',(20.7736384671217,-64.4219203562316,31.1471871810353));
#15015=CARTESIAN_POINT('Ctrl Pts',(20.1694945163644,-64.2506791464088,31.1842315536991));
#15016=CARTESIAN_POINT('Ctrl Pts',(19.631651943939,-64.3724002687565,31.221275926363));
#15017=CARTESIAN_POINT('Ctrl Pts',(19.0938093715137,-64.4941213911041,31.2583202990268));
#15018=CARTESIAN_POINT('Ctrl Pts',(18.6222681774202,-64.9088048456222,31.2953646716907));
#15019=CARTESIAN_POINT('Ctrl Pts',(18.432814891916,-65.4266833226324,31.3324090443545));
#15020=CARTESIAN_POINT('Ctrl Pts',(18.366208376288,-65.608755017935,31.3454328173664));
#15021=CARTESIAN_POINT('Ctrl Pts',(18.334468783344,-65.803581931597,31.3584565903783));
#15022=CARTESIAN_POINT('Ctrl Pts',(18.3357539768147,-65.9988133681531,31.3714803633902));
#15023=CARTESIAN_POINT('Origin',(20.,-66.,30.));
#15024=CARTESIAN_POINT('',(18.3357308127244,-66.0011975491724,32.0714803633902));
#15025=CARTESIAN_POINT('',(18.3319843264428,-66.0009873427492,31.8785196366098));
#15026=CARTESIAN_POINT('',(18.334,-66.,30.));
#15027=CARTESIAN_POINT('Ctrl Pts',(18.3319843264428,-66.0009873427492,31.8785196366098));
#15028=CARTESIAN_POINT('Ctrl Pts',(18.3354516848774,-65.5071812495811,31.8453864902349));
#15029=CARTESIAN_POINT('Ctrl Pts',(18.5685743737179,-65.010531129917,31.81225334386));
#15030=CARTESIAN_POINT('Ctrl Pts',(18.952527100275,-64.7009383696829,31.7791201974851));
#15031=CARTESIAN_POINT('Ctrl Pts',(19.381803804846,-64.3547995075786,31.7420758248213));
#15032=CARTESIAN_POINT('Ctrl Pts',(19.9996220148609,-64.2424872537891,31.7050314521574));
#15033=CARTESIAN_POINT('Ctrl Pts',(20.523255958873,-64.4153979059321,31.6679870794935));
#15034=CARTESIAN_POINT('Ctrl Pts',(21.0468899028851,-64.5883085580752,31.6309427068297));
#15035=CARTESIAN_POINT('Ctrl Pts',(21.4763395808944,-65.0464421161508,31.5938983341658));
#15036=CARTESIAN_POINT('Ctrl Pts',(21.6150803687566,-65.5801476480029,31.556853961502));
#15037=CARTESIAN_POINT('Ctrl Pts',(21.7538211566187,-66.1138531798551,31.5198095888381));
#15038=CARTESIAN_POINT('Ctrl Pts',(21.6018530543337,-66.7231306854838,31.4827652161743));
#15039=CARTESIAN_POINT('Ctrl Pts',(21.2287196562103,-67.129162787849,31.4457208435104));
#15040=CARTESIAN_POINT('Ctrl Pts',(20.8555862580868,-67.5351948902141,31.4086764708466));
#15041=CARTESIAN_POINT('Ctrl Pts',(20.2612875641249,-67.7379815893157,31.3716320981827));
#15042=CARTESIAN_POINT('Ctrl Pts',(19.7177863523659,-67.6447237008414,31.3345877255189));
#15043=CARTESIAN_POINT('Ctrl Pts',(19.1742851406069,-67.5514658123671,31.297543352855));
#15044=CARTESIAN_POINT('Ctrl Pts',(18.6815814110507,-67.162163336317,31.2604989801912));
#15045=CARTESIAN_POINT('Ctrl Pts',(18.4651460866572,-66.6549687471297,31.2234546075273));
#15046=CARTESIAN_POINT('Ctrl Pts',(18.3776337844479,-66.4498923979142,31.2084762838881));
#15047=CARTESIAN_POINT('Ctrl Pts',(18.3352876405059,-66.225542278188,31.193497960249));
#15048=CARTESIAN_POINT('Ctrl Pts',(18.3362976949234,-66.000827356963,31.1785196366098));
#15049=CARTESIAN_POINT('Ctrl Pts',(18.3357539768147,-65.9988133681531,31.3714803633902));
#15050=CARTESIAN_POINT('Ctrl Pts',(18.338124343513,-66.3588915246679,31.3955009630422));
#15051=CARTESIAN_POINT('Ctrl Pts',(18.452834619963,-66.7203457405113,31.4195215626941));
#15052=CARTESIAN_POINT('Ctrl Pts',(18.6683273346162,-67.0056883651597,31.4435421623461));
#15053=CARTESIAN_POINT('Ctrl Pts',(19.0006584397354,-67.4457414311745,31.4805865350099));
#15054=CARTESIAN_POINT('Ctrl Pts',(19.5726860268885,-67.7047740637018,31.5176309076738));
#15055=CARTESIAN_POINT('Ctrl Pts',(20.122639014801,-67.6642478323845,31.5546752803376));
#15056=CARTESIAN_POINT('Ctrl Pts',(20.6725920027136,-67.6237216010672,31.5917196530015));
#15057=CARTESIAN_POINT('Ctrl Pts',(21.2004703913856,-67.2836365059054,31.6287640256653));
#15058=CARTESIAN_POINT('Ctrl Pts',(21.4647066416153,-66.7996221792546,31.6658083983292));
#15059=CARTESIAN_POINT('Ctrl Pts',(21.728942891845,-66.3156078526038,31.702852770993));
#15060=CARTESIAN_POINT('Ctrl Pts',(21.7295370036324,-65.6876642944639,31.7398971436569));
#15061=CARTESIAN_POINT('Ctrl Pts',(21.4662170997316,-65.2031508348486,31.7769415163208));
#15062=CARTESIAN_POINT('Ctrl Pts',(21.2028971958308,-64.7186373752333,31.8139858889846));
#15063=CARTESIAN_POINT('Ctrl Pts',(20.6756632762418,-64.3775540141426,31.8510302616484));
#15064=CARTESIAN_POINT('Ctrl Pts',(20.1257879584309,-64.3359872100667,31.8880746343123));
#15065=CARTESIAN_POINT('Ctrl Pts',(19.57591264062,-64.2944204059907,31.9251190069761));
#15066=CARTESIAN_POINT('Ctrl Pts',(19.0033959245872,-64.5523701589297,31.96216337964));
#15067=CARTESIAN_POINT('Ctrl Pts',(18.6702327266084,-64.9917935855369,31.9992077523039));
#15068=CARTESIAN_POINT('Ctrl Pts',(18.4535684714254,-65.2775614915163,32.023298622666));
#15069=CARTESIAN_POINT('Ctrl Pts',(18.3381321348796,-65.6400786444767,32.0473894930281));
#15070=CARTESIAN_POINT('Ctrl Pts',(18.3357308127244,-66.0011975491724,32.0714803633902));
#15071=CARTESIAN_POINT('Origin',(20.,-66.,30.));
#15072=CARTESIAN_POINT('',(18.3314319388862,-66.0005124578368,32.7714803633902));
#15073=CARTESIAN_POINT('',(18.3333053457166,-65.9985455597719,32.5785196366098));
#15074=CARTESIAN_POINT('',(18.334,-66.,30.));
#15075=CARTESIAN_POINT('Ctrl Pts',(18.3333053457166,-65.9985455597719,32.5785196366098));
#15076=CARTESIAN_POINT('Ctrl Pts',(18.3323271587739,-65.8916766923834,32.5713637655485));
#15077=CARTESIAN_POINT('Ctrl Pts',(18.3417256832142,-65.7849791876526,32.5642078944873));
#15078=CARTESIAN_POINT('Ctrl Pts',(18.3621250373911,-65.6804280959176,32.557052023426));
#15079=CARTESIAN_POINT('Ctrl Pts',(18.4677280131519,-65.1391900591385,32.5200076507622));
#15080=CARTESIAN_POINT('Ctrl Pts',(18.8681428272523,-64.6554738617393,32.4829632780983));
#15081=CARTESIAN_POINT('Ctrl Pts',(19.3801317806736,-64.4506375550925,32.4459189054345));
#15082=CARTESIAN_POINT('Ctrl Pts',(19.892120734095,-64.2458012484457,32.4088745327706));
#15083=CARTESIAN_POINT('Ctrl Pts',(20.5156838268372,-64.3198448325512,32.3718301601068));
#15084=CARTESIAN_POINT('Ctrl Pts',(20.9654663160592,-64.6388845061585,32.3347857874429));
#15085=CARTESIAN_POINT('Ctrl Pts',(21.4152488052812,-64.9579241797659,32.297741414779));
#15086=CARTESIAN_POINT('Ctrl Pts',(21.691250690983,-65.5219599428751,32.2606970421152));
#15087=CARTESIAN_POINT('Ctrl Pts',(21.6671680786034,-66.0728779301719,32.2236526694513));
#15088=CARTESIAN_POINT('Ctrl Pts',(21.6430854662238,-66.6237959174687,32.1866082967875));
#15089=CARTESIAN_POINT('Ctrl Pts',(21.3189183557627,-67.1615961289531,32.1495639241236));
#15090=CARTESIAN_POINT('Ctrl Pts',(20.8430119965137,-67.4401706040447,32.1125195514598));
#15091=CARTESIAN_POINT('Ctrl Pts',(20.3671056372647,-67.7187450791363,32.0754751787959));
#15092=CARTESIAN_POINT('Ctrl Pts',(19.7394600292277,-67.7380938178351,32.0384308061321));
#15093=CARTESIAN_POINT('Ctrl Pts',(19.2472981545858,-67.4893624565331,32.0013864334682));
#15094=CARTESIAN_POINT('Ctrl Pts',(18.7551362799438,-67.2406310952312,31.9643420608044));
#15095=CARTESIAN_POINT('Ctrl Pts',(18.3984581386968,-66.7238196339284,31.9272976881405));
#15096=CARTESIAN_POINT('Ctrl Pts',(18.3404866676369,-66.1754311680674,31.8902533154767));
#15097=CARTESIAN_POINT('Ctrl Pts',(18.3343659123018,-66.1175311084903,31.8863420891877));
#15098=CARTESIAN_POINT('Ctrl Pts',(18.3315750196022,-66.0592790410803,31.8824308628988));
#15099=CARTESIAN_POINT('Ctrl Pts',(18.3319843264428,-66.0009873427492,31.8785196366098));
#15100=CARTESIAN_POINT('Ctrl Pts',(18.3357308127244,-66.0011975491724,32.0714803633902));
#15101=CARTESIAN_POINT('Ctrl Pts',(18.3344396376196,-66.195368805456,32.0844338656919));
#15102=CARTESIAN_POINT('Ctrl Pts',(18.3658284909666,-66.3891358083027,32.0973873679937));
#15103=CARTESIAN_POINT('Ctrl Pts',(18.4317328425237,-66.5703501541415,32.1103408702954));
#15104=CARTESIAN_POINT('Ctrl Pts',(18.6202058363429,-67.0885861958634,32.1473852429593));
#15105=CARTESIAN_POINT('Ctrl Pts',(19.0909615039061,-67.5041611790318,32.1844296156231));
#15106=CARTESIAN_POINT('Ctrl Pts',(19.6285727873552,-67.6268998129126,32.221473988287));
#15107=CARTESIAN_POINT('Ctrl Pts',(20.1661840708043,-67.7496384467933,32.2585183609508));
#15108=CARTESIAN_POINT('Ctrl Pts',(20.7706509701393,-67.5795407313865,32.2955627336147));
#15109=CARTESIAN_POINT('Ctrl Pts',(21.1653575364318,-67.1944467287532,32.3326071062785));
#15110=CARTESIAN_POINT('Ctrl Pts',(21.5600641027243,-66.8093527261198,32.3696514789424));
#15111=CARTESIAN_POINT('Ctrl Pts',(21.7450103359744,-66.20926243626,32.4066958516063));
#15112=CARTESIAN_POINT('Ctrl Pts',(21.6355612001404,-65.6687889854742,32.4437402242701));
#15113=CARTESIAN_POINT('Ctrl Pts',(21.5261120643063,-65.1283155346885,32.480784596934));
#15114=CARTESIAN_POINT('Ctrl Pts',(21.1222675593881,-64.6474589229769,32.5178289695978));
#15115=CARTESIAN_POINT('Ctrl Pts',(20.6088348784189,-64.4462685990267,32.5548733422617));
#15116=CARTESIAN_POINT('Ctrl Pts',(20.0954021974497,-64.2450782750765,32.5919177149255));
#15117=CARTESIAN_POINT('Ctrl Pts',(19.4723813404294,-64.3235542388877,32.6289620875894));
#15118=CARTESIAN_POINT('Ctrl Pts',(19.0248789124613,-64.6457843450241,32.6660064602532));
#15119=CARTESIAN_POINT('Ctrl Pts',(18.600164582529,-64.9516055765046,32.7011644279656));
#15120=CARTESIAN_POINT('Ctrl Pts',(18.3335480283789,-65.4769877278693,32.7363223956779));
#15121=CARTESIAN_POINT('Ctrl Pts',(18.3314319388862,-66.0005124578368,32.7714803633902));
#15122=CARTESIAN_POINT('Origin',(20.,-66.,30.));
#15123=CARTESIAN_POINT('',(18.3342213249666,-65.9984780340466,33.4714803633902));
#15124=CARTESIAN_POINT('',(18.3367010446132,-65.9999263102719,33.2785196366098));
#15125=CARTESIAN_POINT('',(18.334,-66.,30.));
#15126=CARTESIAN_POINT('Ctrl Pts',(18.3367010446132,-65.9999263102719,33.2785196366098));
#15127=CARTESIAN_POINT('Ctrl Pts',(18.3365931047954,-65.7263673738448,33.2602966681983));
#15128=CARTESIAN_POINT('Ctrl Pts',(18.4003187588333,-65.4528557910589,33.2420736997868));
#15129=CARTESIAN_POINT('Ctrl Pts',(18.5281536212252,-65.2135975379756,33.2238507313754));
#15130=CARTESIAN_POINT('Ctrl Pts',(18.7880213977008,-64.7272238753543,33.1868063587115));
#15131=CARTESIAN_POINT('Ctrl Pts',(19.3128164406399,-64.3823999407418,33.1497619860477));
#15132=CARTESIAN_POINT('Ctrl Pts',(19.8623822105493,-64.3369239527128,33.1127176133838));
#15133=CARTESIAN_POINT('Ctrl Pts',(20.4119479804586,-64.2914479646837,33.07567324072));
#15134=CARTESIAN_POINT('Ctrl Pts',(20.9862844773381,-64.545319923238,33.0386288680561));
#15135=CARTESIAN_POINT('Ctrl Pts',(21.3225640173729,-64.9823630239762,33.0015844953923));
#15136=CARTESIAN_POINT('Ctrl Pts',(21.6588435574077,-65.4194061247144,32.9645401227284));
#15137=CARTESIAN_POINT('Ctrl Pts',(21.7570661405977,-66.0396203676365,32.9274957500645));
#15138=CARTESIAN_POINT('Ctrl Pts',(21.572283179879,-66.5591835094909,32.8904513774007));
#15139=CARTESIAN_POINT('Ctrl Pts',(21.3875002191603,-67.0787466513452,32.8534070047368));
#15140=CARTESIAN_POINT('Ctrl Pts',(20.9197117145329,-67.4976586921317,32.816362632073));
#15141=CARTESIAN_POINT('Ctrl Pts',(20.3829868916996,-67.6242172378744,32.7793182594091));
#15142=CARTESIAN_POINT('Ctrl Pts',(19.8462620688664,-67.7507757836172,32.7422738867453));
#15143=CARTESIAN_POINT('Ctrl Pts',(19.2406009278272,-67.5849808343162,32.7052295140814));
#15144=CARTESIAN_POINT('Ctrl Pts',(18.8431659260182,-67.2027034215861,32.6681851414176));
#15145=CARTESIAN_POINT('Ctrl Pts',(18.5225035464367,-66.8942706356756,32.638296639815));
#15146=CARTESIAN_POINT('Ctrl Pts',(18.3373910177132,-66.4449133446109,32.6084081382124));
#15147=CARTESIAN_POINT('Ctrl Pts',(18.3333053457166,-65.9985455597719,32.5785196366098));
#15148=CARTESIAN_POINT('Ctrl Pts',(18.3314319388862,-66.0005124578368,32.7714803633902));
#15149=CARTESIAN_POINT('Ctrl Pts',(18.3313183998521,-66.0286022396733,32.7733667683417));
#15150=CARTESIAN_POINT('Ctrl Pts',(18.3319663237535,-66.0566866742318,32.7752531732933));
#15151=CARTESIAN_POINT('Ctrl Pts',(18.3333921462108,-66.0847315598599,32.7771395782448));
#15152=CARTESIAN_POINT('Ctrl Pts',(18.3613918068445,-66.6354644200977,32.8141839509086));
#15153=CARTESIAN_POINT('Ctrl Pts',(18.6893751270277,-67.1709458921119,32.8512283235725));
#15154=CARTESIAN_POINT('Ctrl Pts',(19.1672504847947,-67.4461291161188,32.8882726962364));
#15155=CARTESIAN_POINT('Ctrl Pts',(19.6451258425617,-67.7213123401258,32.9253170689002));
#15156=CARTESIAN_POINT('Ctrl Pts',(20.2728932379124,-67.7361973161255,32.962361441564));
#15157=CARTESIAN_POINT('Ctrl Pts',(20.7632739563948,-67.4839723862013,32.9994058142279));
#15158=CARTESIAN_POINT('Ctrl Pts',(21.2536546748772,-67.231747456277,33.0364501868917));
#15159=CARTESIAN_POINT('Ctrl Pts',(21.6066487164913,-66.7124126204288,33.0734945595556));
#15160=CARTESIAN_POINT('Ctrl Pts',(21.6607190609346,-66.1636257198826,33.1105389322195));
#15161=CARTESIAN_POINT('Ctrl Pts',(21.7147894053779,-65.6148388193364,33.1475833048833));
#15162=CARTESIAN_POINT('Ctrl Pts',(21.4699360526505,-65.0365998540921,33.1846276775472));
#15163=CARTESIAN_POINT('Ctrl Pts',(21.038208715637,-64.6935223544135,33.221672050211));
#15164=CARTESIAN_POINT('Ctrl Pts',(20.6064813786234,-64.3504448547349,33.2587164228749));
#15165=CARTESIAN_POINT('Ctrl Pts',(19.9878800573237,-64.2425288206219,33.2957607955387));
#15166=CARTESIAN_POINT('Ctrl Pts',(19.4654888903011,-64.4191587527804,33.3328051682026));
#15167=CARTESIAN_POINT('Ctrl Pts',(18.9430977232784,-64.5957886849389,33.3698495408664));
#15168=CARTESIAN_POINT('Ctrl Pts',(18.5169167105327,-65.0569645833689,33.4068939135303));
#15169=CARTESIAN_POINT('Ctrl Pts',(18.3819746706949,-65.5916432816362,33.4439382861941));
#15170=CARTESIAN_POINT('Ctrl Pts',(18.3485320377033,-65.7241524944515,33.4531189785928));
#15171=CARTESIAN_POINT('Ctrl Pts',(18.3329771612274,-65.8611762135967,33.4622996709915));
#15172=CARTESIAN_POINT('Ctrl Pts',(18.3342213249666,-65.9984780340466,33.4714803633902));
#15173=CARTESIAN_POINT('Origin',(20.,-66.,30.));
#15174=CARTESIAN_POINT('',(18.3366059788164,-66.0004198226349,34.1714803633902));
#15175=CARTESIAN_POINT('',(18.3335758017906,-66.001492963312,33.9785196366098));
#15176=CARTESIAN_POINT('',(18.334,-66.,30.));
#15177=CARTESIAN_POINT('Ctrl Pts',(18.3335758017906,-66.001492963312,33.9785196366098));
#15178=CARTESIAN_POINT('Ctrl Pts',(18.3376146481614,-65.563879799351,33.9492295708481));
#15179=CARTESIAN_POINT('Ctrl Pts',(18.5146051988431,-65.1233755891636,33.9199395050864));
#15180=CARTESIAN_POINT('Ctrl Pts',(18.8239358304384,-64.8160938964247,33.8906494393248));
#15181=CARTESIAN_POINT('Ctrl Pts',(19.2151592331577,-64.4274618724746,33.8536050666609));
#15182=CARTESIAN_POINT('Ctrl Pts',(19.8180701248551,-64.2519288582829,33.816560693997));
#15183=CARTESIAN_POINT('Ctrl Pts',(20.3567646176707,-64.3698222172911,33.7795163213332));
#15184=CARTESIAN_POINT('Ctrl Pts',(20.8954591104862,-64.4877155762994,33.7424719486693));
#15185=CARTESIAN_POINT('Ctrl Pts',(21.3699372044197,-64.8990353085074,33.7054275760055));
#15186=CARTESIAN_POINT('Ctrl Pts',(21.5630683853716,-65.4155534089152,33.6683832033416));
#15187=CARTESIAN_POINT('Ctrl Pts',(21.7561995663234,-65.9320715093229,33.6313388306778));
#15188=CARTESIAN_POINT('Ctrl Pts',(21.6679838342935,-66.5537879779303,33.5942944580139));
#15189=CARTESIAN_POINT('Ctrl Pts',(21.3387904446675,-66.9961931238673,33.55725008535));
#15190=CARTESIAN_POINT('Ctrl Pts',(21.0095970550415,-67.4385982698042,33.5202057126862));
#15191=CARTESIAN_POINT('Ctrl Pts',(20.4394260078194,-67.7016920930707,33.4831613400223));
#15192=CARTESIAN_POINT('Ctrl Pts',(19.8891987948963,-67.6650776822906,33.4461169673585));
#15193=CARTESIAN_POINT('Ctrl Pts',(19.3389715819732,-67.6284632715105,33.4090725946946));
#15194=CARTESIAN_POINT('Ctrl Pts',(18.8086882033491,-67.2921406266838,33.3720282220308));
#15195=CARTESIAN_POINT('Ctrl Pts',(18.5410167690432,-66.8100176089554,33.3349838493669));
#15196=CARTESIAN_POINT('Ctrl Pts',(18.4050189936833,-66.56506185553,33.3161624451146));
#15197=CARTESIAN_POINT('Ctrl Pts',(18.3368125291365,-66.2824688254694,33.2973410408622));
#15198=CARTESIAN_POINT('Ctrl Pts',(18.3367010446132,-65.9999263102719,33.2785196366098));
#15199=CARTESIAN_POINT('Ctrl Pts',(18.3342213249666,-65.9984780340466,33.4714803633902));
#15200=CARTESIAN_POINT('Ctrl Pts',(18.3379973997026,-66.41519322923,33.4993440436554));
#15201=CARTESIAN_POINT('Ctrl Pts',(18.4965163106871,-66.8344701293732,33.5272077239205));
#15202=CARTESIAN_POINT('Ctrl Pts',(18.779340917363,-67.1378719524441,33.5550714041857));
#15203=CARTESIAN_POINT('Ctrl Pts',(19.155352270799,-67.5412404268801,33.5921157768495));
#15204=CARTESIAN_POINT('Ctrl Pts',(19.7510780446009,-67.7397958776474,33.6291601495134));
#15205=CARTESIAN_POINT('Ctrl Pts',(20.2939024010583,-67.6426754250913,33.6662045221772));
#15206=CARTESIAN_POINT('Ctrl Pts',(20.8367267575157,-67.5455549725352,33.7032488948411));
#15207=CARTESIAN_POINT('Ctrl Pts',(21.3266496966286,-67.1527586166557,33.740293267505));
#15208=CARTESIAN_POINT('Ctrl Pts',(21.5394728395698,-66.6440376957742,33.7773376401688));
#15209=CARTESIAN_POINT('Ctrl Pts',(21.752295982511,-66.1353167748926,33.8143820128327));
#15210=CARTESIAN_POINT('Ctrl Pts',(21.6880193292805,-65.5106712890091,33.8514263854965));
#15211=CARTESIAN_POINT('Ctrl Pts',(21.3760571419463,-65.0559513139131,33.8884707581604));
#15212=CARTESIAN_POINT('Ctrl Pts',(21.0640949546121,-64.6012313388172,33.9255151308242));
#15213=CARTESIAN_POINT('Ctrl Pts',(20.5044472331742,-64.316436874509,33.9625595034881));
#15214=CARTESIAN_POINT('Ctrl Pts',(19.9532197875309,-64.3318954555163,33.9996038761519));
#15215=CARTESIAN_POINT('Ctrl Pts',(19.4019923418877,-64.3473540365236,34.0366482488158));
#15216=CARTESIAN_POINT('Ctrl Pts',(18.859185172039,-64.6630656628465,34.0736926214796));
#15217=CARTESIAN_POINT('Ctrl Pts',(18.5731975236246,-65.1345545151115,34.1107369941435));
#15218=CARTESIAN_POINT('Ctrl Pts',(18.416881803868,-65.3922618661374,34.1309847838924));
#15219=CARTESIAN_POINT('Ctrl Pts',(18.3372914182245,-65.6965079679593,34.1512325736413));
#15220=CARTESIAN_POINT('Ctrl Pts',(18.3366059788164,-66.0004198226349,34.1714803633902));
#15221=CARTESIAN_POINT('Origin',(20.,-66.,30.));
#15222=CARTESIAN_POINT('',(18.332682461926,-66.0013023226252,34.8714803633902));
#15223=CARTESIAN_POINT('',(18.3317911996431,-65.9991411289371,34.6785196366098));
#15224=CARTESIAN_POINT('',(18.334,-66.,30.));
#15225=CARTESIAN_POINT('Ctrl Pts',(18.3317911996431,-65.9991411289371,34.6785196366098));
#15226=CARTESIAN_POINT('Ctrl Pts',(18.331481150105,-65.9497833776327,34.6752068461618));
#15227=CARTESIAN_POINT('Ctrl Pts',(18.3334818713826,-65.9004511145936,34.6718940557137));
#15228=CARTESIAN_POINT('Ctrl Pts',(18.3378752000437,-65.851332857239,34.6685812652657));
#15229=CARTESIAN_POINT('Ctrl Pts',(18.3870023955927,-65.3020813852329,34.6315368926018));
#15230=CARTESIAN_POINT('Ctrl Pts',(18.7353064493333,-64.7795896519118,34.5944925199379));
#15231=CARTESIAN_POINT('Ctrl Pts',(19.2233964026499,-64.5229599453814,34.5574481472741));
#15232=CARTESIAN_POINT('Ctrl Pts',(19.7114863559666,-64.2663302388509,34.5204037746102));
#15233=CARTESIAN_POINT('Ctrl Pts',(20.3393622088594,-64.275562559111,34.4833594019464));
#15234=CARTESIAN_POINT('Ctrl Pts',(20.8196956993778,-64.5464321208658,34.4463150292825));
#15235=CARTESIAN_POINT('Ctrl Pts',(21.3000291898962,-64.8173016826206,34.4092706566187));
#15236=CARTESIAN_POINT('Ctrl Pts',(21.6328203180401,-65.3498084858701,34.3722262839548));
#15237=CARTESIAN_POINT('Ctrl Pts',(21.6657772717621,-65.9002668845694,34.335181911291));
#15238=CARTESIAN_POINT('Ctrl Pts',(21.698734225484,-66.4507252832687,34.2981375386271));
#15239=CARTESIAN_POINT('Ctrl Pts',(21.4318570047839,-67.0191352774177,34.2610931659632));
#15240=CARTESIAN_POINT('Ctrl Pts',(20.9872738992879,-67.3453812942044,34.2240487932994));
#15241=CARTESIAN_POINT('Ctrl Pts',(20.5426907937918,-67.671627310991,34.1870044206355));
#15242=CARTESIAN_POINT('Ctrl Pts',(19.9204018034998,-67.7557093504152,34.1499600479717));
#15243=CARTESIAN_POINT('Ctrl Pts',(19.405178606192,-67.5591498031194,34.1129156753078));
#15244=CARTESIAN_POINT('Ctrl Pts',(18.8899554088842,-67.3625902558236,34.075871302644));
#15245=CARTESIAN_POINT('Ctrl Pts',(18.4817980045605,-66.8853891218078,34.0388269299801));
#15246=CARTESIAN_POINT('Ctrl Pts',(18.3674872592693,-66.3459230379456,34.0017825573163));
#15247=CARTESIAN_POINT('Ctrl Pts',(18.3435591822778,-66.2329993932254,33.9940282504141));
#15248=CARTESIAN_POINT('Ctrl Pts',(18.3325065500332,-66.1173474924684,33.986273943512));
#15249=CARTESIAN_POINT('Ctrl Pts',(18.3335758017906,-66.001492963312,33.9785196366098));
#15250=CARTESIAN_POINT('Ctrl Pts',(18.3366059788164,-66.0004198226349,34.1714803633902));
#15251=CARTESIAN_POINT('Ctrl Pts',(18.336037371576,-66.2525303358908,34.1882769463051));
#15252=CARTESIAN_POINT('Ctrl Pts',(18.3897676428184,-66.5044108351101,34.2050735292201));
#15253=CARTESIAN_POINT('Ctrl Pts',(18.4990410468759,-66.729303380124,34.2218701121351));
#15254=CARTESIAN_POINT('Ctrl Pts',(18.7400403455219,-67.2252973146641,34.2589144847989));
#15255=CARTESIAN_POINT('Ctrl Pts',(19.2512070697942,-67.5900191055372,34.2959588574628));
#15256=CARTESIAN_POINT('Ctrl Pts',(19.7986212764483,-67.6565650186632,34.3330032301266));
#15257=CARTESIAN_POINT('Ctrl Pts',(20.3460354831024,-67.7231109317891,34.3700476027905));
#15258=CARTESIAN_POINT('Ctrl Pts',(20.9296971721382,-67.491480967168,34.4070919754543));
#15259=CARTESIAN_POINT('Ctrl Pts',(21.2825112494692,-67.0676732857095,34.4441363481182));
#15260=CARTESIAN_POINT('Ctrl Pts',(21.6353253268003,-66.643865604251,34.481180720782));
#15261=CARTESIAN_POINT('Ctrl Pts',(21.7572917924265,-66.0278802059553,34.5182250934459));
#15262=CARTESIAN_POINT('Ctrl Pts',(21.5925964289533,-65.5016046685849,34.5552694661097));
#15263=CARTESIAN_POINT('Ctrl Pts',(21.4279010654802,-64.9753291312145,34.5923138387736));
#15264=CARTESIAN_POINT('Ctrl Pts',(20.9765438729076,-64.5387634547694,34.6293582114374));
#15265=CARTESIAN_POINT('Ctrl Pts',(20.4450747103033,-64.3916876135341,34.6664025841013));
#15266=CARTESIAN_POINT('Ctrl Pts',(19.9136055476989,-64.2446117722988,34.7034469567651));
#15267=CARTESIAN_POINT('Ctrl Pts',(19.3020244150628,-64.3870257662733,34.740491329429));
#15268=CARTESIAN_POINT('Ctrl Pts',(18.8902030237858,-64.7537602841853,34.7775357020928));
#15269=CARTESIAN_POINT('Ctrl Pts',(18.5420761843907,-65.0637736329866,34.808850589192));
#15270=CARTESIAN_POINT('Ctrl Pts',(18.3366957496508,-65.5340842872638,34.8401654762911));
#15271=CARTESIAN_POINT('Ctrl Pts',(18.332682461926,-66.0013023226252,34.8714803633902));
#15272=CARTESIAN_POINT('Origin',(20.,-66.,30.));
#15273=CARTESIAN_POINT('',(18.3325226604529,-65.9987867968397,35.5714803633902));
#15274=CARTESIAN_POINT('',(18.3361559831984,-65.999055845664,35.3785196366098));
#15275=CARTESIAN_POINT('',(18.334,-66.,30.));
#15276=CARTESIAN_POINT('',(21.2690708798524,-64.9206413469515,36.));
#15277=CARTESIAN_POINT('Ctrl Pts',(18.3325226604529,-65.9987867968397,35.5714803633902));
#15278=CARTESIAN_POINT('Ctrl Pts',(18.3364573709904,-66.4716253136251,35.6031871242686));
#15279=CARTESIAN_POINT('Ctrl Pts',(18.5476202216759,-66.9474487737269,35.634893885147));
#15280=CARTESIAN_POINT('Ctrl Pts',(18.9034044398461,-67.2577324547277,35.6666006460253));
#15281=CARTESIAN_POINT('Ctrl Pts',(19.3190824467032,-67.6202502267133,35.7036450186892));
#15282=CARTESIAN_POINT('Ctrl Pts',(19.9321722943361,-67.7568019946271,35.740689391353));
#15283=CARTESIAN_POINT('Ctrl Pts',(20.4620469760753,-67.6038093106228,35.7777337640169));
#15284=CARTESIAN_POINT('Ctrl Pts',(20.9919216578146,-67.4508166266185,35.8147781366807));
#15285=CARTESIAN_POINT('Ctrl Pts',(21.4385811736603,-67.0082794906961,35.8518225093446));
#15286=CARTESIAN_POINT('Ctrl Pts',(21.5975927337787,-66.4812302053523,35.8888668820085));
#15287=CARTESIAN_POINT('Ctrl Pts',(21.756604293897,-65.9541809200085,35.9259112546723));
#15288=CARTESIAN_POINT('Ctrl Pts',(21.627967898288,-65.3426194852432,35.9629556273362));
#15289=CARTESIAN_POINT('Ctrl Pts',(21.2690708798524,-64.9206413469514,36.));
#15290=CARTESIAN_POINT('',(18.7285279290194,-64.9187949404949,36.));
#15291=CARTESIAN_POINT('Origin',(20.,-66.,36.));
#15292=CARTESIAN_POINT('Ctrl Pts',(18.7285264739144,-64.9187938215856,36.));
#15293=CARTESIAN_POINT('Ctrl Pts',(19.0793427655227,-64.5073237570503,35.9636818543909));
#15294=CARTESIAN_POINT('Ctrl Pts',(19.6492096702252,-64.2812825989047,35.9273637087819));
#15295=CARTESIAN_POINT('Ctrl Pts',(20.1865491454986,-64.341804902964,35.8910455631728));
#15296=CARTESIAN_POINT('Ctrl Pts',(20.7346334002206,-64.4035374267052,35.8540011905089));
#15297=CARTESIAN_POINT('Ctrl Pts',(21.2488763655857,-64.7634083897207,35.8169568178451));
#15298=CARTESIAN_POINT('Ctrl Pts',(21.4942849262207,-65.2571540480588,35.7799124451812));
#15299=CARTESIAN_POINT('Ctrl Pts',(21.7396934868558,-65.7508997063968,35.7428680725174));
#15300=CARTESIAN_POINT('Ctrl Pts',(21.7162676427607,-66.3785200600576,35.7058236998535));
#15301=CARTESIAN_POINT('Ctrl Pts',(21.434559910799,-66.8525937901543,35.6687793271897));
#15302=CARTESIAN_POINT('Ctrl Pts',(21.1528521788373,-67.326667520251,35.6317349545258));
#15303=CARTESIAN_POINT('Ctrl Pts',(20.6128625590089,-67.6471946267836,35.594690581862));
#15304=CARTESIAN_POINT('Ctrl Pts',(20.0617849892622,-67.6676008155073,35.5576462091981));
#15305=CARTESIAN_POINT('Ctrl Pts',(19.5107074195156,-67.6880070042309,35.5206018365343));
#15306=CARTESIAN_POINT('Ctrl Pts',(18.9485418998507,-67.4082922751456,35.4835574638704));
#15307=CARTESIAN_POINT('Ctrl Pts',(18.6325042689313,-66.956406817939,35.4465130912066));
#15308=CARTESIAN_POINT('Ctrl Pts',(18.4391461530328,-66.679934296761,35.423848606341));
#15309=CARTESIAN_POINT('Ctrl Pts',(18.3379195160153,-66.3390142077648,35.4011841214754));
#15310=CARTESIAN_POINT('Ctrl Pts',(18.3361559831984,-65.999055845664,35.3785196366098));
#15311=CARTESIAN_POINT('Origin',(20.,-66.,37.5459252805377));
#15312=CARTESIAN_POINT('',(17.9445921681644,-65.9981769380503,25.3540747194623));
#15313=CARTESIAN_POINT('',(17.9470733560714,-66.0015060535927,25.2959252805377));
#15314=CARTESIAN_POINT('',(17.94525,-65.9999999999999,37.5459252805377));
#15315=CARTESIAN_POINT('',(21.8174278887595,-65.0413794120408,25.));
#15316=CARTESIAN_POINT('Ctrl Pts',(17.9470733560714,-66.0015060535927,25.2959252805377));
#15317=CARTESIAN_POINT('Ctrl Pts',(17.9500635199578,-65.5475809519615,25.2713722656862));
#15318=CARTESIAN_POINT('Ctrl Pts',(18.3216912761193,-64.4040176334961,25.2097748781708));
#15319=CARTESIAN_POINT('Ctrl Pts',(20.2159939907177,-63.5820409220313,25.1111331179916));
#15320=CARTESIAN_POINT('Ctrl Pts',(21.4986774253636,-64.4370673526013,25.0370443726639));
#15321=CARTESIAN_POINT('Ctrl Pts',(21.8174278887595,-65.0413794120408,25.));
#15322=CARTESIAN_POINT('',(22.0570978924847,-66.0754551987761,25.));
#15323=CARTESIAN_POINT('Origin',(20.,-66.,25.));
#15324=CARTESIAN_POINT('Ctrl Pts',(17.9445921681644,-65.9981769380503,25.3540747194623));
#15325=CARTESIAN_POINT('Ctrl Pts',(17.943297586139,-65.8578134130738,25.3464567039117));
#15326=CARTESIAN_POINT('Ctrl Pts',(18.0204259142703,-65.0363089952078,25.3017943156971));
#15327=CARTESIAN_POINT('Ctrl Pts',(19.1263754391461,-63.7340406632385,25.2200875548188));
#15328=CARTESIAN_POINT('Ctrl Pts',(21.4138493882471,-64.0348872703216,25.109680663882));
#15329=CARTESIAN_POINT('Ctrl Pts',(22.0806819706411,-65.4089772617309,25.0363181456091));
#15330=CARTESIAN_POINT('Ctrl Pts',(22.0571001480269,-66.0754553928761,25.));
#15331=CARTESIAN_POINT('Origin',(20.,-66.,37.5459252805377));
#15332=CARTESIAN_POINT('',(17.9485832974788,-66.0000495918166,26.0540747194623));
#15333=CARTESIAN_POINT('',(17.9419861288051,-66.0004830914585,25.9959252805377));
#15334=CARTESIAN_POINT('',(17.94525,-65.9999999999999,37.5459252805377));
#15335=CARTESIAN_POINT('Ctrl Pts',(17.9419861288051,-66.0004830914585,25.9959252805377));
#15336=CARTESIAN_POINT('Ctrl Pts',(17.9440551582811,-65.3463924174249,25.9603051683359));
#15337=CARTESIAN_POINT('Ctrl Pts',(18.6350687960196,-64.0082840246707,25.8876406834704));
#15338=CARTESIAN_POINT('Ctrl Pts',(20.9141747077605,-63.7500129462385,25.7779318259409));
#15339=CARTESIAN_POINT('Ctrl Pts',(22.3860296230922,-65.5475930706263,25.6667987079494));
#15340=CARTESIAN_POINT('Ctrl Pts',(21.6743955907743,-67.7593785514666,25.5556655899578));
#15341=CARTESIAN_POINT('Ctrl Pts',(19.429692000846,-68.3606229571339,25.4445324719662));
#15342=CARTESIAN_POINT('Ctrl Pts',(18.0884943176257,-67.1462799502129,25.3579523688262));
#15343=CARTESIAN_POINT('Ctrl Pts',(17.9455521087929,-66.2324406617768,25.30841663835));
#15344=CARTESIAN_POINT('Ctrl Pts',(17.9470733560714,-66.0015060535927,25.2959252805377));
#15345=CARTESIAN_POINT('Ctrl Pts',(17.9485832974788,-66.0000495918166,26.0540747194623));
#15346=CARTESIAN_POINT('Ctrl Pts',(17.9486573139036,-65.6541000235851,26.0353896065614));
#15347=CARTESIAN_POINT('Ctrl Pts',(18.1957460549727,-64.6221845951523,25.9796601209967));
#15348=CARTESIAN_POINT('Ctrl Pts',(19.829859942873,-63.5773515961876,25.8868862627681));
#15349=CARTESIAN_POINT('Ctrl Pts',(21.9430509240163,-64.5430603155101,25.7757531447765));
#15350=CARTESIAN_POINT('Ctrl Pts',(22.2779267364902,-66.8422110789462,25.664620026785));
#15351=CARTESIAN_POINT('Ctrl Pts',(20.5278715823273,-68.3705500709468,25.5534869087934));
#15352=CARTESIAN_POINT('Ctrl Pts',(18.4479228041263,-67.7732032161842,25.4499718063526));
#15353=CARTESIAN_POINT('Ctrl Pts',(17.949592792374,-66.5403637036397,25.3835010765755));
#15354=CARTESIAN_POINT('Ctrl Pts',(17.9445921681644,-65.9981769380503,25.3540747194623));
#15355=CARTESIAN_POINT('Origin',(20.,-66.,37.5459252805377));
#15356=CARTESIAN_POINT('',(17.9444688958667,-66.0018063311818,26.7540747194623));
#15357=CARTESIAN_POINT('',(17.9457762375739,-65.9981345160027,26.6959252805377));
#15358=CARTESIAN_POINT('',(17.94525,-65.9999999999999,37.5459252805377));
#15359=CARTESIAN_POINT('Ctrl Pts',(17.9457762375739,-65.9981345160027,26.6959252805377));
#15360=CARTESIAN_POINT('Ctrl Pts',(17.9441911203672,-65.8202139891171,26.6862824436496));
#15361=CARTESIAN_POINT('Ctrl Pts',(18.0468091802697,-64.9605854820692,26.6395952340976));
#15362=CARTESIAN_POINT('Ctrl Pts',(19.2507941167209,-63.6898347424764,26.5558636518818));
#15363=CARTESIAN_POINT('Ctrl Pts',(21.5344924336398,-64.1175798748589,26.4447305338903));
#15364=CARTESIAN_POINT('Ctrl Pts',(22.4137604897707,-66.2681888420218,26.3335974158987));
#15365=CARTESIAN_POINT('Ctrl Pts',(21.0838647034058,-68.1733431282881,26.2224642979072));
#15366=CARTESIAN_POINT('Ctrl Pts',(18.7619637841276,-68.0893636493551,26.1113311799156));
#15367=CARTESIAN_POINT('Ctrl Pts',(17.9542069036107,-66.7329548013126,26.0358181741258));
#15368=CARTESIAN_POINT('Ctrl Pts',(17.9419033992264,-66.0266367284935,25.9973495409998));
#15369=CARTESIAN_POINT('Ctrl Pts',(17.9419861288051,-66.0004830914585,25.9959252805377));
#15370=CARTESIAN_POINT('Ctrl Pts',(17.9444688958667,-66.0018063311818,26.7540747194623));
#15371=CARTESIAN_POINT('Ctrl Pts',(17.9494993134766,-65.4537400361145,26.7243225092112));
#15372=CARTESIAN_POINT('Ctrl Pts',(18.4568950033307,-64.2150556037813,26.6575259262963));
#15373=CARTESIAN_POINT('Ctrl Pts',(20.5486976238089,-63.6341805685774,26.5536849707175));
#15374=CARTESIAN_POINT('Ctrl Pts',(22.2852057058799,-65.1778050816215,26.4425518527259));
#15375=CARTESIAN_POINT('Ctrl Pts',(21.9302042425984,-67.4739346416768,26.3314187347344));
#15376=CARTESIAN_POINT('Ctrl Pts',(19.8086025657231,-68.4210614106236,26.2202856167428));
#15377=CARTESIAN_POINT('Ctrl Pts',(18.1894356332652,-67.3656511409621,26.1278376116521));
#15378=CARTESIAN_POINT('Ctrl Pts',(17.9485105718401,-66.3399660815773,26.0724339792253));
#15379=CARTESIAN_POINT('Ctrl Pts',(17.9485832974788,-66.0000495918166,26.0540747194623));
#15380=CARTESIAN_POINT('Origin',(20.,-66.,37.5459252805377));
#15381=CARTESIAN_POINT('',(17.9427073981771,-65.9988171298974,27.4540747194623));
#15382=CARTESIAN_POINT('',(17.948391336186,-66.000651392518,27.3959252805377));
#15383=CARTESIAN_POINT('',(17.94525,-65.9999999999999,37.5459252805377));
#15384=CARTESIAN_POINT('Ctrl Pts',(17.948391336186,-66.000651392518,27.3959252805377));
#15385=CARTESIAN_POINT('Ctrl Pts',(17.9494813643374,-65.6173024424008,27.3752153462994));
#15386=CARTESIAN_POINT('Ctrl Pts',(18.2366610904736,-64.5467312444963,27.3174610393972));
#15387=CARTESIAN_POINT('Ctrl Pts',(19.9621345918737,-63.5716800154371,27.2226623598312));
#15388=CARTESIAN_POINT('Ctrl Pts',(22.0195745014619,-64.6511150583807,27.1115292418397));
#15389=CARTESIAN_POINT('Ctrl Pts',(22.2286202996251,-66.9651026731069,27.000396123848));
#15390=CARTESIAN_POINT('Ctrl Pts',(20.3979451577182,-68.3957903719854,26.8892630058565));
#15391=CARTESIAN_POINT('Ctrl Pts',(18.3935018010201,-67.6998767838394,26.787772724753));
#15392=CARTESIAN_POINT('Ctrl Pts',(17.9502805806786,-66.5037217969321,26.7233268163134));
#15393=CARTESIAN_POINT('Ctrl Pts',(17.9457762375739,-65.9981345160027,26.6959252805377));
#15394=CARTESIAN_POINT('Ctrl Pts',(17.9427073981771,-65.9988171298974,27.4540747194623));
#15395=CARTESIAN_POINT('Ctrl Pts',(17.9422312044669,-65.9294336928593,27.4502997845249));
#15396=CARTESIAN_POINT('Ctrl Pts',(17.9768968646083,-65.1796548342728,27.4094804769236));
#15397=CARTESIAN_POINT('Ctrl Pts',(18.8966146957805,-63.836504826525,27.3316167966584));
#15398=CARTESIAN_POINT('Ctrl Pts',(21.219169386089,-63.8995723038675,27.2204836786668));
#15399=CARTESIAN_POINT('Ctrl Pts',(22.4258922629222,-65.8850338815669,27.1093505606752));
#15400=CARTESIAN_POINT('Ctrl Pts',(21.41234306908,-67.9757169742283,26.9982174426837));
#15401=CARTESIAN_POINT('Ctrl Pts',(19.1061618881228,-68.2581461319033,26.8870843246921));
#15402=CARTESIAN_POINT('Ctrl Pts',(18.0164474647602,-66.9515223045583,26.8057034169517));
#15403=CARTESIAN_POINT('Ctrl Pts',(17.9432359581487,-66.1361354584251,26.7613668818751));
#15404=CARTESIAN_POINT('Ctrl Pts',(17.9444688958667,-66.0018063311818,26.7540747194623));
#15405=CARTESIAN_POINT('Origin',(20.,-66.,37.5459252805377));
#15406=CARTESIAN_POINT('',(17.9480454330843,-65.9989448752678,28.1540747194623));
#15407=CARTESIAN_POINT('',(17.9433900806158,-66.0015207493092,28.0959252805377));
#15408=CARTESIAN_POINT('',(17.94525,-65.9999999999999,37.5459252805377));
#15409=CARTESIAN_POINT('Ctrl Pts',(17.9433900806158,-66.0015207493092,28.0959252805377));
#15410=CARTESIAN_POINT('Ctrl Pts',(17.9482332143848,-65.416949847134,28.0641482489491));
#15411=CARTESIAN_POINT('Ctrl Pts',(18.5151173764583,-64.1426999291749,27.9953268446968));
#15412=CARTESIAN_POINT('Ctrl Pts',(20.676812844959,-63.6675986416085,27.8894610677805));
#15413=CARTESIAN_POINT('Ctrl Pts',(22.3266174994283,-65.3035642630666,27.778327949789));
#15414=CARTESIAN_POINT('Ctrl Pts',(21.8470102430435,-67.576935282117,27.6671948317974));
#15415=CARTESIAN_POINT('Ctrl Pts',(19.6769465158166,-68.4070330639894,27.5560617138059));
#15416=CARTESIAN_POINT('Ctrl Pts',(18.1518517698952,-67.2899653282545,27.4656385300526));
#15417=CARTESIAN_POINT('Ctrl Pts',(17.9475316039668,-66.3030082107063,27.4122597189632));
#15418=CARTESIAN_POINT('Ctrl Pts',(17.948391336186,-66.000651392518,27.3959252805377));
#15419=CARTESIAN_POINT('Ctrl Pts',(17.9480454330843,-65.9989448752678,28.1540747194623));
#15420=CARTESIAN_POINT('Ctrl Pts',(17.946767622487,-65.7243289514539,28.1392326871746));
#15421=CARTESIAN_POINT('Ctrl Pts',(18.1259279022936,-64.7658953828094,28.0873462822231));
#15422=CARTESIAN_POINT('Ctrl Pts',(19.580500984485,-63.6078898290281,27.9984155046077));
#15423=CARTESIAN_POINT('Ctrl Pts',(21.7821628698452,-64.3501315205369,27.8872823866162));
#15424=CARTESIAN_POINT('Ctrl Pts',(22.3527191513918,-66.6023977826542,27.7761492686246));
#15425=CARTESIAN_POINT('Ctrl Pts',(20.7699742636292,-68.3033258839143,27.6650161506331));
#15426=CARTESIAN_POINT('Ctrl Pts',(18.560218200161,-67.9099899791605,27.5576579675789));
#15427=CARTESIAN_POINT('Ctrl Pts',(17.9469042114332,-66.6103105664805,27.4873441571887));
#15428=CARTESIAN_POINT('Ctrl Pts',(17.9427073981771,-65.9988171298974,27.4540747194623));
#15429=CARTESIAN_POINT('Origin',(20.,-66.,37.5459252805377));
#15430=CARTESIAN_POINT('',(17.9465563505173,-66.0017537138358,28.8540747194623));
#15431=CARTESIAN_POINT('',(17.9436613428911,-65.998383858391,28.7959252805377));
#15432=CARTESIAN_POINT('',(17.94525,-65.9999999999999,37.5459252805377));
#15433=CARTESIAN_POINT('Ctrl Pts',(17.9436613428911,-65.998383858391,28.7959252805377));
#15434=CARTESIAN_POINT('Ctrl Pts',(17.9427401993079,-65.8916548076745,28.7901255242628));
#15435=CARTESIAN_POINT('Ctrl Pts',(17.99882477166,-65.1041931740386,28.747281395324));
#15436=CARTESIAN_POINT('Ctrl Pts',(19.0161588486977,-63.7795882560541,28.6673928937214));
#15437=CARTESIAN_POINT('Ctrl Pts',(21.3318252735703,-63.9691348729347,28.5562597757299));
#15438=CARTESIAN_POINT('Ctrl Pts',(22.4285527879442,-66.0174091881803,28.4451266577383));
#15439=CARTESIAN_POINT('Ctrl Pts',(21.3025732038757,-68.0497499291796,28.3339935397468));
#15440=CARTESIAN_POINT('Ctrl Pts',(18.9844273548577,-68.2060788576321,28.2228604217552));
#15441=CARTESIAN_POINT('Ctrl Pts',(17.9928405779599,-66.8759493052599,28.1435043353522));
#15442=CARTESIAN_POINT('Ctrl Pts',(17.9425872857618,-66.0984188600057,28.101192621613));
#15443=CARTESIAN_POINT('Ctrl Pts',(17.9433900806158,-66.0015207493092,28.0959252805377));
#15444=CARTESIAN_POINT('Ctrl Pts',(17.9465563505173,-66.0017537138358,28.8540747194623));
#15445=CARTESIAN_POINT('Ctrl Pts',(17.9504440938478,-65.5232420995012,28.8281655898244));
#15446=CARTESIAN_POINT('Ctrl Pts',(18.355544098096,-64.3546301779743,28.7652120875227));
#15447=CARTESIAN_POINT('Ctrl Pts',(20.3013690653653,-63.5901561916745,28.6652142125571));
#15448=CARTESIAN_POINT('Ctrl Pts',(22.188046145667,-64.9461382640413,28.5540810945655));
#15449=CARTESIAN_POINT('Ctrl Pts',(22.0721372727958,-67.2666560767515,28.442947976574));
#15450=CARTESIAN_POINT('Ctrl Pts',(20.0597268093363,-68.4278803929209,28.3318148585824));
#15451=CARTESIAN_POINT('Ctrl Pts',(18.2687136588368,-67.5086938026241,28.2355237728786));
#15452=CARTESIAN_POINT('Ctrl Pts',(17.9499569223782,-66.4097455051991,28.1762770598385));
#15453=CARTESIAN_POINT('Ctrl Pts',(17.9480454330843,-65.9989448752678,28.1540747194623));
#15454=CARTESIAN_POINT('Origin',(20.,-66.,37.5459252805377));
#15455=CARTESIAN_POINT('',(17.9418459383603,-66.0000233771323,29.5540747194623));
#15456=CARTESIAN_POINT('',(17.9484736511709,-65.9995028191367,29.4959252805377));
#15457=CARTESIAN_POINT('',(17.94525,-65.9999999999999,37.5459252805377));
#15458=CARTESIAN_POINT('Ctrl Pts',(17.9484736511709,-65.9995028191366,29.4959252805377));
#15459=CARTESIAN_POINT('Ctrl Pts',(17.9477976021827,-65.6872595106289,29.4790584269126));
#15460=CARTESIAN_POINT('Ctrl Pts',(18.1614619143335,-64.6901194629804,29.4251472006236));
#15461=CARTESIAN_POINT('Ctrl Pts',(19.7114877884649,-63.5885829005652,29.3341916016708));
#15462=CARTESIAN_POINT('Ctrl Pts',(21.869427923728,-64.4497061692577,29.2230584836792));
#15463=CARTESIAN_POINT('Ctrl Pts',(22.3163940432292,-66.7297193708161,29.1119253656877));
#15464=CARTESIAN_POINT('Ctrl Pts',(20.6433051619858,-68.3418646827291,29.0007922476961));
#15465=CARTESIAN_POINT('Ctrl Pts',(18.4994791972086,-67.8383663641301,28.8954588859795));
#15466=CARTESIAN_POINT('Ctrl Pts',(17.9486237545051,-66.5733577174882,28.8271698969266));
#15467=CARTESIAN_POINT('Ctrl Pts',(17.9436613428911,-65.998383858391,28.7959252805377));
#15468=CARTESIAN_POINT('Ctrl Pts',(17.9418460670015,-66.0000233762489,29.5540747194623));
#15469=CARTESIAN_POINT('Ctrl Pts',(17.9419602237683,-65.3211542896944,29.5170984924742));
#15470=CARTESIAN_POINT('Ctrl Pts',(18.6804457109671,-63.9619521942107,29.4430778928223));
#15471=CARTESIAN_POINT('Ctrl Pts',(20.9956693404756,-63.7848672593903,29.3320129205065));
#15472=CARTESIAN_POINT('Ctrl Pts',(22.4010377426051,-65.6350503422798,29.2208798025149));
#15473=CARTESIAN_POINT('Ctrl Pts',(21.6088818987778,-67.8192497161933,29.1097466845234));
#15474=CARTESIAN_POINT('Ctrl Pts',(19.3442140162146,-68.3384001448757,28.9986135665318));
#15475=CARTESIAN_POINT('Ctrl Pts',(18.0677943807432,-67.0952787540644,28.9133895781781));
#15476=CARTESIAN_POINT('Ctrl Pts',(17.9448854735943,-66.2074087547744,28.8652099624883));
#15477=CARTESIAN_POINT('Ctrl Pts',(17.9465563505173,-66.0017537138358,28.8540747194623));
#15478=CARTESIAN_POINT('Origin',(20.,-66.,37.5459252805377));
#15479=CARTESIAN_POINT('',(17.9464881988838,-65.9982315277441,30.2540747194623));
#15480=CARTESIAN_POINT('',(17.9454841446209,-66.0018778869456,30.1959252805377));
#15481=CARTESIAN_POINT('',(17.94525,-65.9999999999999,37.5459252805377));
#15482=CARTESIAN_POINT('Ctrl Pts',(17.9454841446209,-66.0018778869456,30.1959252805377));
#15483=CARTESIAN_POINT('Ctrl Pts',(17.9501627255122,-65.4866536541329,30.1679913295624));
#15484=CARTESIAN_POINT('Ctrl Pts',(18.4074704960921,-64.280766173597,30.1030130059232));
#15485=CARTESIAN_POINT('Ctrl Pts',(20.432251111771,-63.6101609468367,30.0009903096202));
#15486=CARTESIAN_POINT('Ctrl Pts',(22.24222733538,-65.0669467860159,29.8898571916286));
#15487=CARTESIAN_POINT('Ctrl Pts',(22.0000288484413,-67.3776996512498,29.7787240736371));
#15488=CARTESIAN_POINT('Ctrl Pts',(19.9273252390408,-68.4275275699302,29.6675909556455));
#15489=CARTESIAN_POINT('Ctrl Pts',(18.2256189616023,-67.4334540757706,29.573324691279));
#15490=CARTESIAN_POINT('Ctrl Pts',(17.9492823966329,-66.3730339733265,29.5161027995764));
#15491=CARTESIAN_POINT('Ctrl Pts',(17.9484736511709,-65.9995028191366,29.4959252805377));
#15492=CARTESIAN_POINT('Ctrl Pts',(17.9464881988838,-65.9982315277441,30.2540747194623));
#15493=CARTESIAN_POINT('Ctrl Pts',(17.9448198460957,-65.7951106883291,30.2430757677879));
#15494=CARTESIAN_POINT('Ctrl Pts',(18.0658216378279,-64.9098243930965,30.1950324434495));
#15495=CARTESIAN_POINT('Ctrl Pts',(19.3356364183429,-63.6640223619538,30.1099447464474));
#15496=CARTESIAN_POINT('Ctrl Pts',(21.6021943503792,-64.1748578801372,29.9988116284558));
#15497=CARTESIAN_POINT('Ctrl Pts',(22.4023609511933,-66.3561353033128,29.8876785104642));
#15498=CARTESIAN_POINT('Ctrl Pts',(21.0037922534698,-68.2114636795477,29.7765453924727));
#15499=CARTESIAN_POINT('Ctrl Pts',(18.6865133764925,-68.0427734538981,29.6654122744811));
#15500=CARTESIAN_POINT('Ctrl Pts',(17.9424134466727,-66.6826456501542,29.5912553834777));
#15501=CARTESIAN_POINT('Ctrl Pts',(17.9418458566153,-66.0012745042416,29.5541428651381));
#15502=CARTESIAN_POINT('Ctrl Pts',(17.9418460670015,-66.0000233762489,29.5540747194623));
#15503=CARTESIAN_POINT('Origin',(20.,-66.,37.5459252805377));
#15504=CARTESIAN_POINT('',(17.9480838467249,-66.0010204151978,30.9540747194623));
#15505=CARTESIAN_POINT('',(17.9420998107195,-65.9993455607918,30.8959252805377));
#15506=CARTESIAN_POINT('',(17.94525,-65.9999999999999,37.5459252805377));
#15507=CARTESIAN_POINT('Ctrl Pts',(17.9420998107195,-65.9993455607918,30.8959252805377));
#15508=CARTESIAN_POINT('Ctrl Pts',(17.9419500148889,-65.963409877897,30.893968604876));
#15509=CARTESIAN_POINT('Ctrl Pts',(17.9590877394987,-65.2472748400191,30.8549675565505));
#15510=CARTESIAN_POINT('Ctrl Pts',(18.7920501950665,-63.8930996719321,30.7789221355611));
#15511=CARTESIAN_POINT('Ctrl Pts',(21.1149084550803,-63.8424201381079,30.6677890175695));
#15512=CARTESIAN_POINT('Ctrl Pts',(22.4173586146354,-65.7664426154033,30.556655899578));
#15513=CARTESIAN_POINT('Ctrl Pts',(21.5073470237683,-67.9042260038106,30.4455227815864));
#15514=CARTESIAN_POINT('Ctrl Pts',(19.2177521081477,-68.2991868039253,30.3343896635948));
#15515=CARTESIAN_POINT('Ctrl Pts',(18.0396474822591,-67.0194951979082,30.2511904965786));
#15516=CARTESIAN_POINT('Ctrl Pts',(17.9439582650609,-66.1699139098205,30.2050357022262));
#15517=CARTESIAN_POINT('Ctrl Pts',(17.9454841446209,-66.0018778869456,30.1959252805377));
#15518=CARTESIAN_POINT('Ctrl Pts',(17.948083846725,-66.0010204151978,30.9540747194623));
#15519=CARTESIAN_POINT('Ctrl Pts',(17.9499190751742,-65.5927223975328,30.9320086704377));
#15520=CARTESIAN_POINT('Ctrl Pts',(18.2657185825361,-64.4963599216305,30.8728982487491));
#15521=CARTESIAN_POINT('Ctrl Pts',(20.0508159969719,-63.5719167583182,30.7767434543967));
#15522=CARTESIAN_POINT('Ctrl Pts',(22.0674746434876,-64.7257476338574,30.6656103364051));
#15523=CARTESIAN_POINT('Ctrl Pts',(22.1918991212745,-67.0458244289748,30.5544772184136));
#15524=CARTESIAN_POINT('Ctrl Pts',(20.3102112509622,-68.4087215434459,30.443344100422));
#15525=CARTESIAN_POINT('Ctrl Pts',(18.3589378869015,-67.6503617606642,30.343209934105));
#15526=CARTESIAN_POINT('Ctrl Pts',(17.9504388436372,-66.4792198919863,30.2801201404517));
#15527=CARTESIAN_POINT('Ctrl Pts',(17.9464881988838,-65.9982315277441,30.2540747194623));
#15528=CARTESIAN_POINT('Origin',(20.,-66.,37.5459252805377));
#15529=CARTESIAN_POINT('',(17.942763982448,-66.0012177326012,31.6540747194623));
#15530=CARTESIAN_POINT('',(17.9474132556182,-65.9985364755177,31.5959252805377));
#15531=CARTESIAN_POINT('',(17.94525,-65.9999999999999,37.5459252805377));
#15532=CARTESIAN_POINT('Ctrl Pts',(17.9474132556182,-65.9985364755177,31.5959252805377));
#15533=CARTESIAN_POINT('Ctrl Pts',(17.945828170814,-65.7577490840029,31.5829015075258));
#15534=CARTESIAN_POINT('Ctrl Pts',(18.0963189994412,-64.8339923197765,31.53283336185));
#15535=CARTESIAN_POINT('Ctrl Pts',(19.4639280160152,-63.6312875751501,31.4457208435104));
#15536=CARTESIAN_POINT('Ctrl Pts',(21.6992787653883,-64.2648851907865,31.3345877255189));
#15537=CARTESIAN_POINT('Ctrl Pts',(22.3793827057175,-66.4865281732684,31.2234546075273));
#15538=CARTESIAN_POINT('Ctrl Pts',(20.8817819421834,-68.2628814220129,31.1123214895357));
#15539=CARTESIAN_POINT('Ctrl Pts',(18.6177165393643,-67.9733456286802,31.0031450472059));
#15540=CARTESIAN_POINT('Ctrl Pts',(17.9447859946471,-66.643755044526,30.9310129775399));
#15541=CARTESIAN_POINT('Ctrl Pts',(17.9420998107195,-65.9993455607918,30.8959252805377));
#15542=CARTESIAN_POINT('Ctrl Pts',(17.942763982448,-66.0012177326012,31.6540747194623));
#15543=CARTESIAN_POINT('Ctrl Pts',(17.9470404258716,-65.392185277657,31.6209415730874));
#15544=CARTESIAN_POINT('Ctrl Pts',(18.5560216000726,-64.0947973033485,31.5507640540487));
#15545=CARTESIAN_POINT('Ctrl Pts',(20.7615157875532,-63.6938637942672,31.4435421623461));
#15546=CARTESIAN_POINT('Ctrl Pts',(22.3504924848334,-65.3889717086535,31.3324090443545));
#15547=CARTESIAN_POINT('Ctrl Pts',(21.7882059455114,-67.6433167651191,31.221275926363));
#15548=CARTESIAN_POINT('Ctrl Pts',(19.5892829417572,-68.3936336378304,31.1101428083714));
#15549=CARTESIAN_POINT('Ctrl Pts',(18.128234020465,-67.2392077048223,31.0210757394045));
#15550=CARTESIAN_POINT('Ctrl Pts',(17.9468381028388,-66.2781710660904,30.9690530431015));
#15551=CARTESIAN_POINT('Ctrl Pts',(17.948083846725,-66.0010204151978,30.9540747194623));
#15552=CARTESIAN_POINT('Origin',(20.,-66.,37.5459252805377));
#15553=CARTESIAN_POINT('',(17.9443932527679,-65.998206175835,32.3540747194623));
#15554=CARTESIAN_POINT('',(17.9473846863418,-66.0014769892929,32.2959252805377));
#15555=CARTESIAN_POINT('',(17.94525,-65.9999999999999,37.5459252805377));
#15556=CARTESIAN_POINT('Ctrl Pts',(17.9473846863418,-66.001476989293,32.2959252805377));
#15557=CARTESIAN_POINT('Ctrl Pts',(17.9503463410227,-65.5560933942008,32.2718344101756));
#15558=CARTESIAN_POINT('Ctrl Pts',(18.3116444429935,-64.4214700752732,32.2106991671496));
#15559=CARTESIAN_POINT('Ctrl Pts',(20.1830643580926,-63.5782941622798,32.1125195514598));
#15560=CARTESIAN_POINT('Ctrl Pts',(22.1338456839189,-64.8403128349112,32.0013864334682));
#15561=CARTESIAN_POINT('Ctrl Pts',(22.131647452475,-67.1637228458735,31.8902533154766));
#15562=CARTESIAN_POINT('Ctrl Pts',(20.1784815716998,-68.4220479046079,31.7791201974851));
#15563=CARTESIAN_POINT('Ctrl Pts',(18.309998800391,-67.5759383428421,31.6810108525054));
#15564=CARTESIAN_POINT('Ctrl Pts',(17.9503367315926,-66.442636470775,31.6199458801896));
#15565=CARTESIAN_POINT('Ctrl Pts',(17.9474132556182,-65.9985364755177,31.5959252805377));
#15566=CARTESIAN_POINT('Ctrl Pts',(17.9443932527679,-65.998206175835,32.3540747194623));
#15567=CARTESIAN_POINT('Ctrl Pts',(17.9431868124194,-65.8664001702729,32.3469188484011));
#15568=CARTESIAN_POINT('Ctrl Pts',(18.0147856257919,-65.0535688820171,32.302718604676));
#15569=CARTESIAN_POINT('Ctrl Pts',(19.0978804403178,-63.7451494962803,32.221473988287));
#15570=CARTESIAN_POINT('Ctrl Pts',(21.4050825978426,-64.0191129796669,32.1103408702954));
#15571=CARTESIAN_POINT('Ctrl Pts',(22.4262978583092,-66.1060622310153,31.9992077523039));
#15572=CARTESIAN_POINT('Ctrl Pts',(21.2268698206984,-68.0959391539699,31.8880746343123));
#15573=CARTESIAN_POINT('Ctrl Pts',(18.9045622340586,-68.16753006785,31.7769415163208));
#15574=CARTESIAN_POINT('Ctrl Pts',(17.9783027092024,-66.8254193993548,31.6989415447041));
#15575=CARTESIAN_POINT('Ctrl Pts',(17.9422591665831,-66.0731114103599,31.6579859457513));
#15576=CARTESIAN_POINT('Ctrl Pts',(17.942763982448,-66.0012177326012,31.6540747194623));
#15577=CARTESIAN_POINT('Origin',(20.,-66.,37.5459252805377));
#15578=CARTESIAN_POINT('',(17.9485813153775,-65.9999091152646,33.0540747194623));
#15579=CARTESIAN_POINT('',(17.9420826989354,-66.0006320364587,32.9959252805377));
#15580=CARTESIAN_POINT('',(17.94525,-65.9999999999999,37.5459252805377));
#15581=CARTESIAN_POINT('Ctrl Pts',(17.9420826989354,-66.0006320364586,32.9959252805377));
#15582=CARTESIAN_POINT('Ctrl Pts',(17.9446925638124,-65.3549462988232,32.9607673128254));
#15583=CARTESIAN_POINT('Ctrl Pts',(18.6199954646792,-64.0242258864647,32.8885649724491));
#15584=CARTESIAN_POINT('Ctrl Pts',(20.8860622876183,-63.7387911759138,32.7793182594092));
#15585=CARTESIAN_POINT('Ctrl Pts',(22.3802990759988,-65.5179750707177,32.6681851414176));
#15586=CARTESIAN_POINT('Ctrl Pts',(21.6959924623663,-67.7383271531118,32.5570520234261));
#15587=CARTESIAN_POINT('Ctrl Pts',(19.4594467935634,-68.3676938050906,32.4459189054344));
#15588=CARTESIAN_POINT('Ctrl Pts',(18.09521740236,-67.1633756303953,32.358876657805));
#15589=CARTESIAN_POINT('Ctrl Pts',(17.945792224129,-66.2409568145323,32.3088787828394));
#15590=CARTESIAN_POINT('Ctrl Pts',(17.9473846863418,-66.001476989293,32.2959252805377));
#15591=CARTESIAN_POINT('Ctrl Pts',(17.9485813153775,-65.9999091152646,33.0540747194623));
#15592=CARTESIAN_POINT('Ctrl Pts',(17.9484481885224,-65.6625170236538,33.0358517510509));
#15593=CARTESIAN_POINT('Ctrl Pts',(18.1868160730737,-64.6394380396369,32.9805844099755));
#15594=CARTESIAN_POINT('Ctrl Pts',(19.7997192052125,-63.5796574421335,32.8882726962363));
#15595=CARTESIAN_POINT('Ctrl Pts',(21.9247814806566,-64.5189913079908,32.7771395782448));
#15596=CARTESIAN_POINT('Ctrl Pts',(22.2882079863162,-66.8138026206755,32.6660064602532));
#15597=CARTESIAN_POINT('Ctrl Pts',(20.5573764799239,-68.3637897439758,32.5548733422617));
#15598=CARTESIAN_POINT('Ctrl Pts',(18.4607079720781,-67.7898433151808,32.4508960953314));
#15599=CARTESIAN_POINT('Ctrl Pts',(17.9494322891033,-66.5487309092672,32.3839632210649));
#15600=CARTESIAN_POINT('Ctrl Pts',(17.9443932527679,-65.998206175835,32.3540747194623));
#15601=CARTESIAN_POINT('Origin',(20.,-66.,37.5459252805377));
#15602=CARTESIAN_POINT('',(17.9447268179648,-66.0018413363536,33.7540747194623));
#15603=CARTESIAN_POINT('',(17.9455229696729,-65.9981228934317,33.6959252805377));
#15604=CARTESIAN_POINT('',(17.94525,-65.9999999999999,37.5459252805377));
#15605=CARTESIAN_POINT('Ctrl Pts',(17.9455229696729,-65.9981228934317,33.6959252805377));
#15606=CARTESIAN_POINT('Ctrl Pts',(17.9439884886147,-65.8287826079759,33.686744588139));
#15607=CARTESIAN_POINT('Ctrl Pts',(18.0405830452216,-64.9778761146953,33.6405195230764));
#15608=CARTESIAN_POINT('Ctrl Pts',(19.2221041313598,-63.699337108691,33.55725008535));
#15609=CARTESIAN_POINT('Ctrl Pts',(21.5109475856345,-64.0986296736855,33.4461169673585));
#15610=CARTESIAN_POINT('Ctrl Pts',(22.4169123392658,-66.2381311992,33.3349838493669));
#15611=CARTESIAN_POINT('Ctrl Pts',(21.110823791235,-68.1596856781178,33.2238507313754));
#15612=CARTESIAN_POINT('Ctrl Pts',(18.7880655878792,-68.1046108201909,33.1127176133838));
#15613=CARTESIAN_POINT('Ctrl Pts',(17.9584343935882,-66.7501147046579,33.0367424631046));
#15614=CARTESIAN_POINT('Ctrl Pts',(17.9419426663241,-66.035276381734,32.9978116854892));
#15615=CARTESIAN_POINT('Ctrl Pts',(17.9420826989354,-66.0006320364586,32.9959252805377));
#15616=CARTESIAN_POINT('Ctrl Pts',(17.9447268179648,-66.0018413363536,33.7540747194623));
#15617=CARTESIAN_POINT('Ctrl Pts',(17.9497081022268,-65.4621140562523,33.7247846537006));
#15618=CARTESIAN_POINT('Ctrl Pts',(18.4440788696627,-64.23169580166,33.6584502152751));
#15619=CARTESIAN_POINT('Ctrl Pts',(20.5192141319096,-63.6275356306401,33.5550714041857));
#15620=CARTESIAN_POINT('Ctrl Pts',(22.2747973195027,-65.14943098434,33.4439382861942));
#15621=CARTESIAN_POINT('Ctrl Pts',(21.9483964634611,-67.4498005771448,33.3328051682026));
#15622=CARTESIAN_POINT('Ctrl Pts',(19.838746476763,-68.4232556192041,33.221672050211));
#15623=CARTESIAN_POINT('Ctrl Pts',(18.1984100797459,-67.382901918355,33.1287619006309));
#15624=CARTESIAN_POINT('Ctrl Pts',(17.9487188140715,-66.3483810438974,33.0728961237147));
#15625=CARTESIAN_POINT('Ctrl Pts',(17.9485813153775,-65.9999091152646,33.0540747194623));
#15626=CARTESIAN_POINT('Origin',(20.,-66.,37.5459252805377));
#15627=CARTESIAN_POINT('',(17.9425257907963,-65.9989407170969,34.4540747194623));
#15628=CARTESIAN_POINT('',(17.9484640666104,-66.0005177854496,34.3959252805377));
#15629=CARTESIAN_POINT('',(17.94525,-65.9999999999999,37.5459252805377));
#15630=CARTESIAN_POINT('Ctrl Pts',(17.9484640666104,-66.0005177854496,34.3959252805377));
#15631=CARTESIAN_POINT('Ctrl Pts',(17.9493094487375,-65.6256901243484,34.3756774907888));
#15632=CARTESIAN_POINT('Ctrl Pts',(18.2270646452969,-64.5639295218498,34.318385328376));
#15633=CARTESIAN_POINT('Ctrl Pts',(19.9319188455824,-63.5723392811283,34.2240487932994));
#15634=CARTESIAN_POINT('Ctrl Pts',(22.0026322110525,-64.6260873463218,34.1129156753078));
#15635=CARTESIAN_POINT('Ctrl Pts',(22.2404577570769,-66.9372943909543,34.0017825573163));
#15636=CARTESIAN_POINT('Ctrl Pts',(20.4277281787894,-68.3906526963146,33.8906494393247));
#15637=CARTESIAN_POINT('Ctrl Pts',(18.4056138794515,-67.7166818294076,33.7886970137319));
#15638=CARTESIAN_POINT('Ctrl Pts',(17.9501801662898,-66.5120758029774,33.7237889608029));
#15639=CARTESIAN_POINT('Ctrl Pts',(17.9455229696729,-65.9981228934317,33.6959252805377));
#15640=CARTESIAN_POINT('Ctrl Pts',(17.9425257907963,-65.9989407170969,34.4540747194623));
#15641=CARTESIAN_POINT('Ctrl Pts',(17.9421433932643,-65.9380656633799,34.4507619290143));
#15642=CARTESIAN_POINT('Ctrl Pts',(17.9722039657874,-65.1968549373091,34.4104047659024));
#15643=CARTESIAN_POINT('Ctrl Pts',(18.8697771195624,-63.8504033302666,34.3330032301266));
#15644=CARTESIAN_POINT('Ctrl Pts',(21.1929366190789,-63.8845631923098,34.2218701121351));
#15645=CARTESIAN_POINT('Ctrl Pts',(22.4242737809404,-65.8548543459294,34.1107369941435));
#15646=CARTESIAN_POINT('Ctrl Pts',(21.4368200548297,-67.9579883834045,33.9996038761519));
#15647=CARTESIAN_POINT('Ctrl Pts',(19.134332114609,-68.2690944527448,33.8884707581604));
#15648=CARTESIAN_POINT('Ctrl Pts',(18.0221619398455,-66.9687900530357,33.8066277059305));
#15649=CARTESIAN_POINT('Ctrl Pts',(17.9434080634338,-66.1447297479887,33.7618290263645));
#15650=CARTESIAN_POINT('Ctrl Pts',(17.9447268179648,-66.0018413363536,33.7540747194623));
#15651=CARTESIAN_POINT('Origin',(20.,-66.,37.5459252805377));
#15652=CARTESIAN_POINT('',(17.9479090675131,-65.9988355335402,35.1540747194623));
#15653=CARTESIAN_POINT('',(17.9436250231948,-66.0016062109329,35.0959252805377));
#15654=CARTESIAN_POINT('',(17.94525,-65.9999999999999,37.5459252805377));
#15655=CARTESIAN_POINT('Ctrl Pts',(17.9436250231948,-66.0016062109329,35.0959252805377));
#15656=CARTESIAN_POINT('Ctrl Pts',(17.9485747848709,-65.4253659599372,35.0646103934386));
#15657=CARTESIAN_POINT('Ctrl Pts',(18.5015294951086,-64.1591280542333,34.9962511336756));
#15658=CARTESIAN_POINT('Ctrl Pts',(20.6477354930483,-63.6593582743169,34.8908475012487));
#15659=CARTESIAN_POINT('Ctrl Pts',(22.317770651701,-65.2746643793748,34.7797143832572));
#15660=CARTESIAN_POINT('Ctrl Pts',(21.8664910684258,-67.5538288400258,34.6685812652657));
#15661=CARTESIAN_POINT('Ctrl Pts',(19.7069253021358,-68.4108666608038,34.5574481472741));
#15662=CARTESIAN_POINT('Ctrl Pts',(18.160182505541,-67.3072525638627,34.4665628190314));
#15663=CARTESIAN_POINT('Ctrl Pts',(17.947762778659,-66.3114566072458,34.4127218634526));
#15664=CARTESIAN_POINT('Ctrl Pts',(17.9484640666104,-66.0005177854496,34.3959252805377));
#15665=CARTESIAN_POINT('Ctrl Pts',(17.9479090675131,-65.9988355335402,35.1540747194623));
#15666=CARTESIAN_POINT('Ctrl Pts',(17.9465290735626,-65.732812424341,35.1396948316641));
#15667=CARTESIAN_POINT('Ctrl Pts',(18.1181888186522,-64.7831883521569,35.088270571202));
#15668=CARTESIAN_POINT('Ctrl Pts',(19.5507727141961,-63.6133045893429,34.9998019380759));
#15669=CARTESIAN_POINT('Ctrl Pts',(21.761489776565,-64.3280769471683,34.8886688200845));
#15670=CARTESIAN_POINT('Ctrl Pts',(22.3600352216356,-66.5730755571057,34.7775357020928));
#15671=CARTESIAN_POINT('Ctrl Pts',(20.7985769413999,-68.2935646002867,34.6664025841013));
#15672=CARTESIAN_POINT('Ctrl Pts',(18.5745658878196,-67.9261849676859,34.5585822565578));
#15673=CARTESIAN_POINT('Ctrl Pts',(17.9464194490253,-66.6187842935463,34.4878063016781));
#15674=CARTESIAN_POINT('Ctrl Pts',(17.9425257907963,-65.9989407170969,34.4540747194623));
#15675=CARTESIAN_POINT('Origin',(20.,-66.,37.5459252805377));
#15676=CARTESIAN_POINT('',(17.9473272127329,-66.0023217579764,35.8540747194623));
#15677=CARTESIAN_POINT('',(17.9434279331127,-65.9985037039655,35.7959252805377));
#15678=CARTESIAN_POINT('',(17.94525,-65.9999999999999,37.5459252805377));
#15679=CARTESIAN_POINT('',(19.4698297828114,-67.9851743256717,36.));
#15680=CARTESIAN_POINT('Ctrl Pts',(19.4698297828114,-67.9851743256717,36.));
#15681=CARTESIAN_POINT('Ctrl Pts',(18.8097404375819,-67.8088876857537,35.9629556273362));
#15682=CARTESIAN_POINT('Ctrl Pts',(18.0750703124531,-67.1127915443424,35.9143138671569));
#15683=CARTESIAN_POINT('Ctrl Pts',(17.9457101070604,-66.2165907677818,35.8656721069777));
#15684=CARTESIAN_POINT('Ctrl Pts',(17.9473272127329,-66.0023217579764,35.8540747194623));
#15685=CARTESIAN_POINT('',(20.5313109889995,-67.9887317423832,36.));
#15686=CARTESIAN_POINT('Origin',(20.,-66.,36.));
#15687=CARTESIAN_POINT('Ctrl Pts',(20.5313116823135,-67.9887339044341,36.));
#15688=CARTESIAN_POINT('Ctrl Pts',(19.886791211028,-68.1600296186371,35.9636818543909));
#15689=CARTESIAN_POINT('Ctrl Pts',(18.5070308443187,-67.8407344661192,35.8956569479035));
#15690=CARTESIAN_POINT('Ctrl Pts',(17.9482807821384,-66.581675938278,35.8276320414161));
#15691=CARTESIAN_POINT('Ctrl Pts',(17.9434279331127,-65.9985037039655,35.7959252805377));
#15692=CARTESIAN_POINT('Origin',(-20.,66.,30.));
#15693=CARTESIAN_POINT('',(-21.6686462681531,65.9996083069911,25.7714803633902));
#15694=CARTESIAN_POINT('',(-21.6665334416367,66.0014781716809,25.5785196366098));
#15695=CARTESIAN_POINT('',(-21.666,66.,30.));
#15696=CARTESIAN_POINT('',(-20.7699020406705,64.5225674811446,25.));
#15697=CARTESIAN_POINT('Ctrl Pts',(-21.6665334416367,66.0014781716809,25.5785196366098));
#15698=CARTESIAN_POINT('Ctrl Pts',(-21.6675830928675,66.1152855193122,25.5709016210591));
#15699=CARTESIAN_POINT('Ctrl Pts',(-21.6569163987491,66.2288979483422,25.5632836055085));
#15700=CARTESIAN_POINT('Ctrl Pts',(-21.6338086023805,66.3399235421032,25.5556655899578));
#15701=CARTESIAN_POINT('Ctrl Pts',(-21.5214415673665,66.8798113177522,25.518621217294));
#15702=CARTESIAN_POINT('Ctrl Pts',(-21.1148901326579,67.3585303508392,25.4815768446301));
#15703=CARTESIAN_POINT('Ctrl Pts',(-20.6004654535252,67.5569679067401,25.4445324719662));
#15704=CARTESIAN_POINT('Ctrl Pts',(-20.0860407743925,67.7554054626409,25.4074880993024));
#15705=CARTESIAN_POINT('Ctrl Pts',(-19.4637428508357,67.6735615413556,25.3704437266385));
#15706=CARTESIAN_POINT('Ctrl Pts',(-19.0178170908,67.3489733082452,25.3333993539747));
#15707=CARTESIAN_POINT('Ctrl Pts',(-18.5718913307643,67.0243850751348,25.2963549813108));
#15708=CARTESIAN_POINT('Ctrl Pts',(-18.3023377342496,66.4570525301995,25.259310608647));
#15709=CARTESIAN_POINT('Ctrl Pts',(-18.3335864217295,65.9064187381511,25.2222662359831));
#15710=CARTESIAN_POINT('Ctrl Pts',(-18.3648351092095,65.3557849461027,25.1852218633193));
#15711=CARTESIAN_POINT('Ctrl Pts',(-18.696886080684,64.8218499069412,25.1481774906554));
#15712=CARTESIAN_POINT('Ctrl Pts',(-19.1753377222773,64.5495456028442,25.1111331179916));
#15713=CARTESIAN_POINT('Ctrl Pts',(-19.6537893638706,64.2772412987472,25.0740887453277));
#15714=CARTESIAN_POINT('Ctrl Pts',(-20.2786416755828,64.2665677297147,25.0370443726639));
#15715=CARTESIAN_POINT('Ctrl Pts',(-20.7699020406704,64.5225674811445,25.));
#15716=CARTESIAN_POINT('',(-21.3370260870439,66.9990029413793,25.));
#15717=CARTESIAN_POINT('Origin',(-20.,66.,25.));
#15718=CARTESIAN_POINT('',(-21.6645215499604,65.9987788526261,25.0714803633902));
#15719=CARTESIAN_POINT('Ctrl Pts',(-21.3370275036536,66.9990041127265,25.));
#15720=CARTESIAN_POINT('Ctrl Pts',(-21.5489928091346,66.714549930132,25.0238267877968));
#15721=CARTESIAN_POINT('Ctrl Pts',(-21.6621689158337,66.3559372077737,25.0476535755935));
#15722=CARTESIAN_POINT('Ctrl Pts',(-21.6645215499604,65.9987788526261,25.0714803633902));
#15723=CARTESIAN_POINT('',(-21.666,66.,24.));
#15724=CARTESIAN_POINT('',(-21.666,66.,30.));
#15725=CARTESIAN_POINT('Origin',(-20.,66.,24.));
#15726=CARTESIAN_POINT('Ctrl Pts',(-21.6645215499604,65.9987788526261,25.0714803633902));
#15727=CARTESIAN_POINT('Ctrl Pts',(-21.6657549346251,65.8115361219705,25.0839717212025));
#15728=CARTESIAN_POINT('Ctrl Pts',(-21.6365290094972,65.624693117297,25.0964630790149));
#15729=CARTESIAN_POINT('Ctrl Pts',(-21.5751097615993,65.4491448676051,25.1089544368272));
#15730=CARTESIAN_POINT('Ctrl Pts',(-21.3929648305163,64.9285389511166,25.145998809491));
#15731=CARTESIAN_POINT('Ctrl Pts',(-20.927686570446,64.5072679681757,25.1830431821549));
#15732=CARTESIAN_POINT('Ctrl Pts',(-20.3917115430329,64.3778810633712,25.2200875548188));
#15733=CARTESIAN_POINT('Ctrl Pts',(-19.8557365156198,64.2484941585667,25.2571319274826));
#15734=CARTESIAN_POINT('Ctrl Pts',(-19.2490647208639,64.4109913318987,25.2941763001465));
#15735=CARTESIAN_POINT('Ctrl Pts',(-18.8495628769352,64.7911274066971,25.3312206728103));
#15736=CARTESIAN_POINT('Ctrl Pts',(-18.4500610330064,65.1712634814956,25.3682650454742));
#15737=CARTESIAN_POINT('Ctrl Pts',(-18.2577291399049,65.7690384577606,25.405309418138));
#15738=CARTESIAN_POINT('Ctrl Pts',(-18.3604608656205,66.3108401952129,25.4423537908019));
#15739=CARTESIAN_POINT('Ctrl Pts',(-18.4631925913361,66.8526419326652,25.4793981634657));
#15740=CARTESIAN_POINT('Ctrl Pts',(-18.8609879358689,67.3384704313048,25.5164425361296));
#15741=CARTESIAN_POINT('Ctrl Pts',(-19.3718687026598,67.5460303751797,25.5534869087934));
#15742=CARTESIAN_POINT('Ctrl Pts',(-19.8827494694507,67.7535903190547,25.5905312814573));
#15743=CARTESIAN_POINT('Ctrl Pts',(-20.5067156584998,67.682881708165,25.6275756541211));
#15744=CARTESIAN_POINT('Ctrl Pts',(-20.9581975756331,67.3662474649163,25.664620026785));
#15745=CARTESIAN_POINT('Ctrl Pts',(-21.3923211790011,67.0617869906151,25.7002401389867));
#15746=CARTESIAN_POINT('Ctrl Pts',(-21.6669686931593,66.5299477666492,25.7358602511885));
#15747=CARTESIAN_POINT('Ctrl Pts',(-21.6686462681531,65.9996083069911,25.7714803633902));
#15748=CARTESIAN_POINT('Origin',(-20.,66.,30.));
#15749=CARTESIAN_POINT('',(-21.6655732346566,66.0015125422222,26.4714803633902));
#15750=CARTESIAN_POINT('',(-21.6632974484405,65.9999597910396,26.2785196366098));
#15751=CARTESIAN_POINT('',(-21.666,66.,30.));
#15752=CARTESIAN_POINT('Ctrl Pts',(-21.6632974484405,65.9999597910396,26.2785196366098));
#15753=CARTESIAN_POINT('Ctrl Pts',(-21.66323743521,66.2804571829106,26.2598345237089));
#15754=CARTESIAN_POINT('Ctrl Pts',(-21.5960667645061,66.5609817057811,26.241149410808));
#15755=CARTESIAN_POINT('Ctrl Pts',(-21.4619468807006,66.8046575880589,26.2224642979072));
#15756=CARTESIAN_POINT('Ctrl Pts',(-21.196046054536,67.2877598438589,26.1854199252433));
#15757=CARTESIAN_POINT('Ctrl Pts',(-20.666998173837,67.6260267717087,26.1483755525794));
#15758=CARTESIAN_POINT('Ctrl Pts',(-20.116910180859,67.6646601094217,26.1113311799156));
#15759=CARTESIAN_POINT('Ctrl Pts',(-19.566822187881,67.7032934471347,26.0742868072517));
#15760=CARTESIAN_POINT('Ctrl Pts',(-18.995694082624,67.4422931947108,26.0372424345879));
#15761=CARTESIAN_POINT('Ctrl Pts',(-18.6648769112216,67.0010995179133,26.000198061924));
#15762=CARTESIAN_POINT('Ctrl Pts',(-18.3340597398192,66.5599058411157,25.9631536892602));
#15763=CARTESIAN_POINT('Ctrl Pts',(-18.2435535022714,65.9385187399443,25.9261093165963));
#15764=CARTESIAN_POINT('Ctrl Pts',(-18.4347924103425,65.4212945612671,25.8890649439325));
#15765=CARTESIAN_POINT('Ctrl Pts',(-18.6260313184137,64.9040703825899,25.8520205712686));
#15766=CARTESIAN_POINT('Ctrl Pts',(-19.0990153721038,64.4910091264068,25.8149761986048));
#15767=CARTESIAN_POINT('Ctrl Pts',(-19.6372643126555,64.3711409749501,25.7779318259409));
#15768=CARTESIAN_POINT('Ctrl Pts',(-20.1755132532071,64.2512728234933,25.7408874532771));
#15769=CARTESIAN_POINT('Ctrl Pts',(-20.7790270806202,64.424597776763,25.7038430806132));
#15770=CARTESIAN_POINT('Ctrl Pts',(-21.1716926766671,64.8117885125033,25.6667987079494));
#15771=CARTESIAN_POINT('Ctrl Pts',(-21.4836082855555,65.1193551425066,25.6373723508362));
#15772=CARTESIAN_POINT('Ctrl Pts',(-21.6624789195953,65.5618708183968,25.607945993723));
#15773=CARTESIAN_POINT('Ctrl Pts',(-21.6665334416367,66.0014781716809,25.5785196366098));
#15774=CARTESIAN_POINT('Ctrl Pts',(-21.6686462681531,65.9996083069911,25.7714803633902));
#15775=CARTESIAN_POINT('Ctrl Pts',(-21.6687133455312,65.978402828479,25.7729046238523));
#15776=CARTESIAN_POINT('Ctrl Pts',(-21.6683440044686,65.9571997477577,25.7743288843144));
#15777=CARTESIAN_POINT('Ctrl Pts',(-21.667530989676,65.9360136962792,25.7757531447766));
#15778=CARTESIAN_POINT('Ctrl Pts',(-21.6463848413682,65.3849740464984,25.8127975174404));
#15779=CARTESIAN_POINT('Ctrl Pts',(-21.3250948995353,64.8454546225443,25.8498418901043));
#15780=CARTESIAN_POINT('Ctrl Pts',(-20.8506820945636,64.5643464247502,25.8868862627681));
#15781=CARTESIAN_POINT('Ctrl Pts',(-20.3762692895919,64.283238226956,25.923930635432));
#15782=CARTESIAN_POINT('Ctrl Pts',(-19.7487336214815,64.2605412553218,25.9609750080958));
#15783=CARTESIAN_POINT('Ctrl Pts',(-19.2552516088359,64.5066439494556,25.9980193807597));
#15784=CARTESIAN_POINT('Ctrl Pts',(-18.7617695961903,64.7527466435894,26.0350637534235));
#15785=CARTESIAN_POINT('Ctrl Pts',(-18.4023412390094,65.2676490034913,26.0721081260874));
#15786=CARTESIAN_POINT('Ctrl Pts',(-18.3414460973868,65.8157206437916,26.1091524987512));
#15787=CARTESIAN_POINT('Ctrl Pts',(-18.2805509557642,66.3637922840919,26.1461968714151));
#15788=CARTESIAN_POINT('Ctrl Pts',(-18.5181890296997,66.9450332047907,26.1832412440789));
#15789=CARTESIAN_POINT('Ctrl Pts',(-18.9456134277585,67.2934565894908,26.2202856167428));
#15790=CARTESIAN_POINT('Ctrl Pts',(-19.3730378258172,67.6418799741908,26.2573299894066));
#15791=CARTESIAN_POINT('Ctrl Pts',(-19.9902485479992,67.7574858228921,26.2943743620705));
#15792=CARTESIAN_POINT('Ctrl Pts',(-20.5147973357793,67.5873703895759,26.3314187347344));
#15793=CARTESIAN_POINT('Ctrl Pts',(-21.0393461235593,67.4172549562597,26.3684631073982));
#15794=CARTESIAN_POINT('Ctrl Pts',(-21.4712329769374,66.9614182409261,26.4055074800621));
#15795=CARTESIAN_POINT('Ctrl Pts',(-21.6128182158583,66.4284602129379,26.4425518527259));
#15796=CARTESIAN_POINT('Ctrl Pts',(-21.6496735670628,66.2897285524311,26.452194689614));
#15797=CARTESIAN_POINT('Ctrl Pts',(-21.6668584543246,66.14577125099,26.4618375265021));
#15798=CARTESIAN_POINT('Ctrl Pts',(-21.6655732346566,66.0015125422222,26.4714803633902));
#15799=CARTESIAN_POINT('Origin',(-20.,66.,30.));
#15800=CARTESIAN_POINT('',(-21.6634529018243,65.9994718482165,27.1714803633902));
#15801=CARTESIAN_POINT('',(-21.6666334235039,65.9985354189402,26.9785196366098));
#15802=CARTESIAN_POINT('',(-21.666,66.,30.));
#15803=CARTESIAN_POINT('Ctrl Pts',(-21.6666334235039,65.9985354189402,26.9785196366098));
#15804=CARTESIAN_POINT('Ctrl Pts',(-21.6625547393445,66.4429099184687,26.9487674263587));
#15805=CARTESIAN_POINT('Ctrl Pts',(-21.4793115692531,66.8902540064005,26.9190152161076));
#15806=CARTESIAN_POINT('Ctrl Pts',(-21.1612403286263,67.1984497694804,26.8892630058565));
#15807=CARTESIAN_POINT('Ctrl Pts',(-20.7652109421709,67.5821832334683,26.8522186331926));
#15808=CARTESIAN_POINT('Ctrl Pts',(-20.1601622793762,67.7501998808548,26.8151742605288));
#15809=CARTESIAN_POINT('Ctrl Pts',(-19.6229765827774,67.6256119767683,26.7781298878649));
#15810=CARTESIAN_POINT('Ctrl Pts',(-19.0857908861786,67.5010240726819,26.7410855152011));
#15811=CARTESIAN_POINT('Ctrl Pts',(-18.6164681557757,67.0838316171223,26.7040411425373));
#15812=CARTESIAN_POINT('Ctrl Pts',(-18.4297795752062,66.56495010894,26.6669967698734));
#15813=CARTESIAN_POINT('Ctrl Pts',(-18.2430909946367,66.0460686007576,26.6299523972095));
#15814=CARTESIAN_POINT('Ctrl Pts',(-18.3390365639006,65.4254980399525,26.5929080245457));
#15815=CARTESIAN_POINT('Ctrl Pts',(-18.6737099694251,64.9872236861523,26.5558636518818));
#15816=CARTESIAN_POINT('Ctrl Pts',(-19.0083833749495,64.5489493323522,26.518819279218));
#15817=CARTESIAN_POINT('Ctrl Pts',(-19.5817846167346,64.2929711855571,26.4817749065541));
#15818=CARTESIAN_POINT('Ctrl Pts',(-20.1315134695615,64.3364299664923,26.4447305338903));
#15819=CARTESIAN_POINT('Ctrl Pts',(-20.6812423223883,64.3798887474276,26.4076861612264));
#15820=CARTESIAN_POINT('Ctrl Pts',(-21.2072987862569,64.7227844560932,26.3706417885626));
#15821=CARTESIAN_POINT('Ctrl Pts',(-21.4689501323761,65.208201102301,26.3335974158987));
#15822=CARTESIAN_POINT('Ctrl Pts',(-21.5986250245473,65.4487744919996,26.3152381561357));
#15823=CARTESIAN_POINT('Ctrl Pts',(-21.6633564150892,65.7243540450368,26.2968788963728));
#15824=CARTESIAN_POINT('Ctrl Pts',(-21.6632974484405,65.9999597910396,26.2785196366098));
#15825=CARTESIAN_POINT('Ctrl Pts',(-21.6655732346566,66.0015125422222,26.4714803633902));
#15826=CARTESIAN_POINT('Ctrl Pts',(-21.6619210944078,65.591580256201,26.4988818991659));
#15827=CARTESIAN_POINT('Ctrl Pts',(-21.5091236523064,65.1792141192603,26.5262834349417));
#15828=CARTESIAN_POINT('Ctrl Pts',(-21.2347245072689,64.8774064445228,26.5536849707175));
#15829=CARTESIAN_POINT('Ctrl Pts',(-20.8637619352948,64.4693900447385,26.5907293433813));
#15830=CARTESIAN_POINT('Ctrl Pts',(-20.270553166883,64.2634365858125,26.6277737160452));
#15831=CARTESIAN_POINT('Ctrl Pts',(-19.7265622699546,64.353794453272,26.664818088709));
#15832=CARTESIAN_POINT('Ctrl Pts',(-19.1825713730262,64.4441523207316,26.7018624613729));
#15833=CARTESIAN_POINT('Ctrl Pts',(-18.6877983475811,64.8308215145768,26.7389068340367));
#15834=CARTESIAN_POINT('Ctrl Pts',(-18.4686610363739,65.3368545872826,26.7759512067006));
#15835=CARTESIAN_POINT('Ctrl Pts',(-18.2495237251666,65.8428876599883,26.8129955793645));
#15836=CARTESIAN_POINT('Ctrl Pts',(-18.3060221281972,66.4682846115547,26.8500399520283));
#15837=CARTESIAN_POINT('Ctrl Pts',(-18.6123014797734,66.9268514966992,26.8870843246922));
#15838=CARTESIAN_POINT('Ctrl Pts',(-18.9185808313496,67.3854183818437,26.924128697356));
#15839=CARTESIAN_POINT('Ctrl Pts',(-19.4746411314715,67.6771552005663,26.9611730700198));
#15840=CARTESIAN_POINT('Ctrl Pts',(-20.0260182359126,67.6685574395601,26.9982174426837));
#15841=CARTESIAN_POINT('Ctrl Pts',(-20.5773953403537,67.6599596785538,27.0352618153475));
#15842=CARTESIAN_POINT('Ctrl Pts',(-21.1240892491141,67.3510273378186,27.0723061880114));
#15843=CARTESIAN_POINT('Ctrl Pts',(-21.4159220745912,66.8831339380774,27.1093505606753));
#15844=CARTESIAN_POINT('Ctrl Pts',(-21.5790734033788,66.6215546254215,27.1300604949136));
#15845=CARTESIAN_POINT('Ctrl Pts',(-21.6625691024306,66.3102927833835,27.1507704291519));
#15846=CARTESIAN_POINT('Ctrl Pts',(-21.6634529018243,65.9994718482165,27.1714803633902));
#15847=CARTESIAN_POINT('Origin',(-20.,66.,30.));
#15848=CARTESIAN_POINT('',(-21.667507940799,65.9987669700874,27.8714803633902));
#15849=CARTESIAN_POINT('',(-21.6680616533731,66.0009590761454,27.6785196366098));
#15850=CARTESIAN_POINT('',(-21.666,66.,30.));
#15851=CARTESIAN_POINT('Ctrl Pts',(-21.6680616533731,66.0009590761454,27.6785196366098));
#15852=CARTESIAN_POINT('Ctrl Pts',(-21.668447753273,66.0572154640797,27.6747447016723));
#15853=CARTESIAN_POINT('Ctrl Pts',(-21.6658484356799,66.1134357515378,27.6709697667349));
#15854=CARTESIAN_POINT('Ctrl Pts',(-21.6601460955106,66.1693395220565,27.6671948317974));
#15855=CARTESIAN_POINT('Ctrl Pts',(-21.6041876173419,66.7179370853841,27.6301504591336));
#15856=CARTESIAN_POINT('Ctrl Pts',(-21.2494085740158,67.2360541193704,27.5931060864697));
#15857=CARTESIAN_POINT('Ctrl Pts',(-20.7581628372053,67.4865900729032,27.5560617138058));
#15858=CARTESIAN_POINT('Ctrl Pts',(-20.2669171003947,67.737126026436,27.519017341142));
#15859=CARTESIAN_POINT('Ctrl Pts',(-19.6392046700997,67.7200808995153,27.4819729684782));
#15860=CARTESIAN_POINT('Ctrl Pts',(-19.1622791087534,67.4432548774978,27.4449285958143));
#15861=CARTESIAN_POINT('Ctrl Pts',(-18.6853535474071,67.1664288554803,27.4078842231505));
#15862=CARTESIAN_POINT('Ctrl Pts',(-18.3592148550096,66.629821938366,27.3708398504866));
#15863=CARTESIAN_POINT('Ctrl Pts',(-18.3331105134156,66.0789960120806,27.3337954778227));
#15864=CARTESIAN_POINT('Ctrl Pts',(-18.3070061718216,65.5281700857952,27.2967511051589));
#15865=CARTESIAN_POINT('Ctrl Pts',(-18.5809361810313,64.9631251503388,27.259706732495));
#15866=CARTESIAN_POINT('Ctrl Pts',(-19.0295447821931,64.6424368874882,27.2226623598312));
#15867=CARTESIAN_POINT('Ctrl Pts',(-19.4781533833549,64.3217486246376,27.1856179871673));
#15868=CARTESIAN_POINT('Ctrl Pts',(-20.1014405764689,64.2454170343927,27.1485736145035));
#15869=CARTESIAN_POINT('Ctrl Pts',(-20.6141778673144,64.4483729559646,27.1115292418396));
#15870=CARTESIAN_POINT('Ctrl Pts',(-21.12691515816,64.6513288775365,27.0744848691758));
#15871=CARTESIAN_POINT('Ctrl Pts',(-21.529102546737,65.1335723109252,27.0374404965119));
#15872=CARTESIAN_POINT('Ctrl Pts',(-21.6366911859674,65.6744191679142,27.0003961238481));
#15873=CARTESIAN_POINT('Ctrl Pts',(-21.6578699446997,65.7808845454597,26.9931039614353));
#15874=CARTESIAN_POINT('Ctrl Pts',(-21.6676330946903,65.8896207872102,26.9858117990226));
#15875=CARTESIAN_POINT('Ctrl Pts',(-21.6666334235039,65.9985354189402,26.9785196366098));
#15876=CARTESIAN_POINT('Ctrl Pts',(-21.6634529018243,65.9994718482165,27.1714803633902));
#15877=CARTESIAN_POINT('Ctrl Pts',(-21.6641499763108,65.7543196730124,27.1878148018157));
#15878=CARTESIAN_POINT('Ctrl Pts',(-21.6134552796394,65.5094417801467,27.2041492402413));
#15879=CARTESIAN_POINT('Ctrl Pts',(-21.5099183024031,65.2894314975948,27.2204836786668));
#15880=CARTESIAN_POINT('Ctrl Pts',(-21.275109962544,64.7904769156004,27.2575280513307));
#15881=CARTESIAN_POINT('Ctrl Pts',(-20.7685215406322,64.4194222103586,27.2945724239945));
#15882=CARTESIAN_POINT('Ctrl Pts',(-20.2219778690728,64.3460693177449,27.3316167966584));
#15883=CARTESIAN_POINT('Ctrl Pts',(-19.6754341975135,64.2727164251311,27.3686611693223));
#15884=CARTESIAN_POINT('Ctrl Pts',(-19.0889352763067,64.4970653451454,27.4057055419861));
#15885=CARTESIAN_POINT('Ctrl Pts',(-18.7308745534937,64.916449596609,27.4427499146499));
#15886=CARTESIAN_POINT('Ctrl Pts',(-18.3728138306807,65.3358338480726,27.4797942873138));
#15887=CARTESIAN_POINT('Ctrl Pts',(-18.2431913062614,65.9502534309856,27.5168386599777));
#15888=CARTESIAN_POINT('Ctrl Pts',(-18.401324798602,66.478537852666,27.5538830326415));
#15889=CARTESIAN_POINT('Ctrl Pts',(-18.5594582909426,67.0068222743464,27.5909274053054));
#15890=CARTESIAN_POINT('Ctrl Pts',(-19.005347800043,67.4489715347942,27.6279717779692));
#15891=CARTESIAN_POINT('Ctrl Pts',(-19.5349455113959,67.6026494309563,27.6650161506331));
#15892=CARTESIAN_POINT('Ctrl Pts',(-20.0645432227487,67.7563273271185,27.7020605232969));
#15893=CARTESIAN_POINT('Ctrl Pts',(-20.6778491363538,67.621533858995,27.7391048959608));
#15894=CARTESIAN_POINT('Ctrl Pts',(-21.0942023964646,67.2599531703386,27.7761492686246));
#15895=CARTESIAN_POINT('Ctrl Pts',(-21.4513543671184,66.9497856566518,27.8079263002132));
#15896=CARTESIAN_POINT('Ctrl Pts',(-21.6635811076441,66.472739507198,27.8397033318017));
#15897=CARTESIAN_POINT('Ctrl Pts',(-21.667507940799,65.9987669700874,27.8714803633902));
#15898=CARTESIAN_POINT('Origin',(-20.,66.,30.));
#15899=CARTESIAN_POINT('',(-21.6672880002095,66.001310374389,28.5714803633902));
#15900=CARTESIAN_POINT('',(-21.6637335518062,66.000855499652,28.3785196366098));
#15901=CARTESIAN_POINT('',(-21.666,66.,30.));
#15902=CARTESIAN_POINT('Ctrl Pts',(-21.6637335518062,66.000855499652,28.3785196366098));
#15903=CARTESIAN_POINT('Ctrl Pts',(-21.6647696061116,66.2235152669179,28.3636776043221));
#15904=CARTESIAN_POINT('Ctrl Pts',(-21.6232170679033,66.4458042001806,28.3488355720345));
#15905=CARTESIAN_POINT('Ctrl Pts',(-21.5372474291621,66.6493314053291,28.3339935397468));
#15906=CARTESIAN_POINT('Ctrl Pts',(-21.3226749721306,67.157316935115,28.2969491670829));
#15907=CARTESIAN_POINT('Ctrl Pts',(-20.8314032853562,67.5484250538238,28.2599047944191));
#15908=CARTESIAN_POINT('Ctrl Pts',(-20.2882479608308,67.6436769894029,28.2228604217552));
#15909=CARTESIAN_POINT('Ctrl Pts',(-19.7450926363055,67.738928924982,28.1858160490914));
#15910=CARTESIAN_POINT('Ctrl Pts',(-19.1500536740293,67.5383246774313,28.1487716764275));
#15911=CARTESIAN_POINT('Ctrl Pts',(-18.7754326134094,67.1336646982806,28.1117273037637));
#15912=CARTESIAN_POINT('Ctrl Pts',(-18.4008115527896,66.7290047191299,28.0746829310998));
#15913=CARTESIAN_POINT('Ctrl Pts',(-18.2466083938262,66.1202890083791,28.0376385584359));
#15914=CARTESIAN_POINT('Ctrl Pts',(-18.3833895367155,65.5860778546815,28.0005941857721));
#15915=CARTESIAN_POINT('Ctrl Pts',(-18.5201706796048,65.051866700984,27.9635498131083));
#15916=CARTESIAN_POINT('Ctrl Pts',(-18.9479361243467,64.5921601043397,27.9265054404444));
#15917=CARTESIAN_POINT('Ctrl Pts',(-19.4709319851533,64.4173288503001,27.8894610677805));
#15918=CARTESIAN_POINT('Ctrl Pts',(-19.9939278459598,64.2424975962605,27.8524166951167));
#15919=CARTESIAN_POINT('Ctrl Pts',(-20.6121541228309,64.3525416848257,27.8153723224528));
#15920=CARTESIAN_POINT('Ctrl Pts',(-21.0426983047608,64.6971027754428,27.778327949789));
#15921=CARTESIAN_POINT('Ctrl Pts',(-21.4293687170027,65.0065520365018,27.7450585120626));
#15922=CARTESIAN_POINT('Ctrl Pts',(-21.6646588592093,65.5051575786095,27.7117890743362));
#15923=CARTESIAN_POINT('Ctrl Pts',(-21.6680616533731,66.0009590761454,27.6785196366098));
#15924=CARTESIAN_POINT('Ctrl Pts',(-21.667507940799,65.9987669700874,27.8714803633902));
#15925=CARTESIAN_POINT('Ctrl Pts',(-21.6681588502308,65.9202015758861,27.8767477044655));
#15926=CARTESIAN_POINT('Ctrl Pts',(-21.6630864755223,65.8417206327871,27.8820150455409));
#15927=CARTESIAN_POINT('Ctrl Pts',(-21.6520021809334,65.7640981769684,27.8872823866162));
#15928=CARTESIAN_POINT('Ctrl Pts',(-21.5740480986749,65.2181917814439,27.92432675928));
#15929=CARTESIAN_POINT('Ctrl Pts',(-21.1987393275416,64.7147468995842,27.9613711319439));
#15930=CARTESIAN_POINT('Ctrl Pts',(-20.6978245472241,64.4841498170345,27.9984155046077));
#15931=CARTESIAN_POINT('Ctrl Pts',(-20.1969097669067,64.2535527344848,28.0354598772716));
#15932=CARTESIAN_POINT('Ctrl Pts',(-19.5703889774051,64.2958034512451,28.0725042499354));
#15933=CARTESIAN_POINT('Ctrl Pts',(-19.1049704217966,64.5915672078361,28.1095486225993));
#15934=CARTESIAN_POINT('Ctrl Pts',(-18.6395518661881,64.8873309644271,28.1465929952632));
#15935=CARTESIAN_POINT('Ctrl Pts',(-18.3352355444726,65.4366077608489,28.183637367927));
#15936=CARTESIAN_POINT('Ctrl Pts',(-18.3312825943579,65.9880377253988,28.2206817405909));
#15937=CARTESIAN_POINT('Ctrl Pts',(-18.3273296442431,66.5394676899486,28.2577261132547));
#15938=CARTESIAN_POINT('Ctrl Pts',(-18.6237400657292,67.0930508226264,28.2947704859186));
#15939=CARTESIAN_POINT('Ctrl Pts',(-19.0848706166418,67.395456587508,28.3318148585824));
#15940=CARTESIAN_POINT('Ctrl Pts',(-19.5460011675545,67.6978623523895,28.3688592312463));
#15941=CARTESIAN_POINT('Ctrl Pts',(-20.1718518478936,67.7490907494749,28.4059036039101));
#15942=CARTESIAN_POINT('Ctrl Pts',(-20.6760210697158,67.5256986560933,28.442947976574));
#15943=CARTESIAN_POINT('Ctrl Pts',(-21.1801902915379,67.3023065627116,28.4799923492378));
#15944=CARTESIAN_POINT('Ctrl Pts',(-21.562678054843,66.804293978863,28.5170367219017));
#15945=CARTESIAN_POINT('Ctrl Pts',(-21.6484504318563,66.2595612637084,28.5540810945655));
#15946=CARTESIAN_POINT('Ctrl Pts',(-21.6618791619446,66.1742765968166,28.5598808508404));
#15947=CARTESIAN_POINT('Ctrl Pts',(-21.6680348672868,66.0878467359549,28.5656806071153));
#15948=CARTESIAN_POINT('Ctrl Pts',(-21.6672880002095,66.001310374389,28.5714803633902));
#15949=CARTESIAN_POINT('Origin',(-20.,66.,30.));
#15950=CARTESIAN_POINT('',(-21.6633861604904,66.0004031163274,29.2714803633902));
#15951=CARTESIAN_POINT('',(-21.6649409063295,65.9985780813102,29.0785196366098));
#15952=CARTESIAN_POINT('',(-21.666,66.,30.));
#15953=CARTESIAN_POINT('Ctrl Pts',(-21.6649409063295,65.9985780813102,29.0785196366098));
#15954=CARTESIAN_POINT('Ctrl Pts',(-21.6617887073852,66.3865573477782,29.0526105069719));
#15955=CARTESIAN_POINT('Ctrl Pts',(-21.5266090909747,66.7765166408617,29.026701377334));
#15956=CARTESIAN_POINT('Ctrl Pts',(-21.2788295744943,67.0720801517677,29.0007922476961));
#15957=CARTESIAN_POINT('Ctrl Pts',(-20.9245592120679,67.4946711456321,28.9637478750323));
#15958=CARTESIAN_POINT('Ctrl Pts',(-20.3401039415215,67.7242914136439,28.9267035023684));
#15959=CARTESIAN_POINT('Ctrl Pts',(-19.7929219966247,67.6558622022781,28.8896591297046));
#15960=CARTESIAN_POINT('Ctrl Pts',(-19.2457400517279,67.5874329909124,28.8526147570407));
#15961=CARTESIAN_POINT('Ctrl Pts',(-18.7358314324807,67.2209543001691,28.8155703843769));
#15962=CARTESIAN_POINT('Ctrl Pts',(-18.4965403579548,66.7241339911626,28.778526011713));
#15963=CARTESIAN_POINT('Ctrl Pts',(-18.2572492834288,66.2273136821561,28.7414816390492));
#15964=CARTESIAN_POINT('Ctrl Pts',(-18.2885757536241,65.6001517548864,28.7044372663853));
#15965=CARTESIAN_POINT('Ctrl Pts',(-18.5761841592798,65.1296498496988,28.6673928937215));
#15966=CARTESIAN_POINT('Ctrl Pts',(-18.8637925649355,64.6591479445111,28.6303485210576));
#15967=CARTESIAN_POINT('Ctrl Pts',(-19.4076829060515,64.3453060614055,28.5933041483937));
#15968=CARTESIAN_POINT('Ctrl Pts',(-19.9589602588768,64.3317444224388,28.5562597757299));
#15969=CARTESIAN_POINT('Ctrl Pts',(-20.510237611702,64.3181827834722,28.519215403066));
#15970=CARTESIAN_POINT('Ctrl Pts',(-21.0689019762364,64.6049013886446,28.4821710304022));
#15971=CARTESIAN_POINT('Ctrl Pts',(-21.3792975448593,65.0606921616624,28.4451266577383));
#15972=CARTESIAN_POINT('Ctrl Pts',(-21.56533141641,65.3338678467978,28.4229243173622));
#15973=CARTESIAN_POINT('Ctrl Pts',(-21.6621837080993,65.6677765893587,28.400721976986));
#15974=CARTESIAN_POINT('Ctrl Pts',(-21.6637335518062,66.000855499652,28.3785196366098));
#15975=CARTESIAN_POINT('Ctrl Pts',(-21.6672880002095,66.001310374389,28.5714803633902));
#15976=CARTESIAN_POINT('Ctrl Pts',(-21.663264456078,65.5351191600222,28.6027249797792));
#15977=CARTESIAN_POINT('Ctrl Pts',(-21.4589128088386,65.065837056818,28.6339695961681));
#15978=CARTESIAN_POINT('Ctrl Pts',(-21.112153076385,64.7558631865457,28.6652142125571));
#15979=CARTESIAN_POINT('Ctrl Pts',(-20.7010263531788,64.3883506709982,28.7022585852209));
#15980=CARTESIAN_POINT('Ctrl Pts',(-20.0897159160448,64.2447784863638,28.7393029578848));
#15981=CARTESIAN_POINT('Ctrl Pts',(-19.5579694514877,64.3908480898042,28.7763473305487));
#15982=CARTESIAN_POINT('Ctrl Pts',(-19.0262229869306,64.5369176932446,28.8133917032125));
#15983=CARTESIAN_POINT('Ctrl Pts',(-18.5740404949502,64.9726290847598,28.8504360758764));
#15984=CARTESIAN_POINT('Ctrl Pts',(-18.4083495827417,65.4985921568759,28.8874804485402));
#15985=CARTESIAN_POINT('Ctrl Pts',(-18.2426586705331,66.0245552289919,28.9245248212041));
#15986=CARTESIAN_POINT('Ctrl Pts',(-18.3634593380964,66.6407699817089,28.9615691938679));
#15987=CARTESIAN_POINT('Ctrl Pts',(-18.7154708226205,67.0652444171952,28.9986135665318));
#15988=CARTESIAN_POINT('Ctrl Pts',(-19.0674823071445,67.4897188526815,29.0356579391956));
#15989=CARTESIAN_POINT('Ctrl Pts',(-19.6507046086295,67.7224529709372,29.0727023118595));
#15990=CARTESIAN_POINT('Ctrl Pts',(-20.1982437242128,67.6569430592857,29.1097466845233));
#15991=CARTESIAN_POINT('Ctrl Pts',(-20.745782839796,67.5914331476342,29.1467910571872));
#15992=CARTESIAN_POINT('Ctrl Pts',(-21.2576387694775,67.2276792060755,29.183835429851));
#15993=CARTESIAN_POINT('Ctrl Pts',(-21.4995761666085,66.7321421968747,29.2208798025149));
#15994=CARTESIAN_POINT('Ctrl Pts',(-21.6097338604876,66.5065168292688,29.23774665614));
#15995=CARTESIAN_POINT('Ctrl Pts',(-21.663934303843,66.2535712993117,29.2546135097651));
#15996=CARTESIAN_POINT('Ctrl Pts',(-21.6633861604904,66.0004031163274,29.2714803633902));
#15997=CARTESIAN_POINT('Origin',(-20.,66.,30.));
#15998=CARTESIAN_POINT('',(-21.6658100649286,65.9984774013953,29.9714803633902));
#15999=CARTESIAN_POINT('',(-21.6687601286834,65.999981045721,29.7785196366098));
#16000=CARTESIAN_POINT('',(-21.666,66.,30.));
#16001=CARTESIAN_POINT('Ctrl Pts',(-21.6687600243793,65.9999810464372,29.7785196366098));
#16002=CARTESIAN_POINT('Ctrl Pts',(-21.6686674655839,66.550411009554,29.7415434096217));
#16003=CARTESIAN_POINT('Ctrl Pts',(-21.3695594894198,67.1009271605486,29.7045671826336));
#16004=CARTESIAN_POINT('Ctrl Pts',(-20.9076738855946,67.4003174817966,29.6675909556455));
#16005=CARTESIAN_POINT('Ctrl Pts',(-20.444937045471,67.7002595671756,29.6305465829816));
#16006=CARTESIAN_POINT('Ctrl Pts',(-19.8188220397766,67.7481493405696,29.5935022103178));
#16007=CARTESIAN_POINT('Ctrl Pts',(-19.3158514169405,67.5220714992119,29.5564578376539));
#16008=CARTESIAN_POINT('Ctrl Pts',(-18.8128807941043,67.2959936578542,29.5194134649901));
#16009=CARTESIAN_POINT('Ctrl Pts',(-18.4330545541264,66.7959482017448,29.4823690923262));
#16010=CARTESIAN_POINT('Ctrl Pts',(-18.3501886593282,66.250765772398,29.4453247196624));
#16011=CARTESIAN_POINT('Ctrl Pts',(-18.26732276453,65.7055833430513,29.4082803469985));
#16012=CARTESIAN_POINT('Ctrl Pts',(-18.4814172149115,65.1152639404671,29.3712359743347));
#16013=CARTESIAN_POINT('Ctrl Pts',(-18.8944981766404,64.7499493406408,29.3341916016708));
#16014=CARTESIAN_POINT('Ctrl Pts',(-19.3075791383693,64.3846347408145,29.297147229007));
#16015=CARTESIAN_POINT('Ctrl Pts',(-19.9196466114455,64.244324943746,29.2601028563431));
#16016=CARTESIAN_POINT('Ctrl Pts',(-20.450606474819,64.3932284738437,29.2230584836793));
#16017=CARTESIAN_POINT('Ctrl Pts',(-20.9815663381925,64.5421320039414,29.1860141110154));
#16018=CARTESIAN_POINT('Ctrl Pts',(-21.4314185918632,64.9802488612052,29.1489697383515));
#16019=CARTESIAN_POINT('Ctrl Pts',(-21.5943019915453,65.5070881496957,29.1119253656877));
#16020=CARTESIAN_POINT('Ctrl Pts',(-21.6432634426356,65.6654518387288,29.1007901226617));
#16021=CARTESIAN_POINT('Ctrl Pts',(-21.6662956604954,65.8318320932536,29.0896548796358));
#16022=CARTESIAN_POINT('Ctrl Pts',(-21.6649409063295,65.9985780813102,29.0785196366098));
#16023=CARTESIAN_POINT('Ctrl Pts',(-21.6633861604904,66.0004031163274,29.2714803633902));
#16024=CARTESIAN_POINT('Ctrl Pts',(-21.6627304262808,65.6975424912392,29.291657882429));
#16025=CARTESIAN_POINT('Ctrl Pts',(-21.5837244591008,65.3943632293128,29.3118354014677));
#16026=CARTESIAN_POINT('Ctrl Pts',(-21.4284374785815,65.1372559790479,29.3320129205065));
#16027=CARTESIAN_POINT('Ctrl Pts',(-21.1433425288428,64.6652268472649,29.3690572931703));
#16028=CARTESIAN_POINT('Ctrl Pts',(-20.601133764785,64.3484886605419,29.4061016658341));
#16029=CARTESIAN_POINT('Ctrl Pts',(-20.0499365874053,64.3319870464702,29.443146038498));
#16030=CARTESIAN_POINT('Ctrl Pts',(-19.4987394100257,64.3154854323984,29.4801904111618));
#16031=CARTESIAN_POINT('Ctrl Pts',(-18.9385538193242,64.599220390978,29.5172347838257));
#16032=CARTESIAN_POINT('Ctrl Pts',(-18.6257317659509,65.0533492213131,29.5542791564896));
#16033=CARTESIAN_POINT('Ctrl Pts',(-18.3129097125776,65.5074780516483,29.5913235291534));
#16034=CARTESIAN_POINT('Ctrl Pts',(-18.2474511965325,66.1320007537391,29.6283679018173));
#16035=CARTESIAN_POINT('Ctrl Pts',(-18.4593113229688,66.6411234486219,29.6654122744811));
#16036=CARTESIAN_POINT('Ctrl Pts',(-18.6711714494052,67.1502461435046,29.702456647145));
#16037=CARTESIAN_POINT('Ctrl Pts',(-19.160350218323,67.5439688311792,29.7395010198088));
#16038=CARTESIAN_POINT('Ctrl Pts',(-19.7029897981211,67.6421162613788,29.7765453924727));
#16039=CARTESIAN_POINT('Ctrl Pts',(-20.2456293779192,67.7402636915784,29.8135897651365));
#16040=CARTESIAN_POINT('Ctrl Pts',(-20.8417297685976,67.542835864303,29.8506341378004));
#16041=CARTESIAN_POINT('Ctrl Pts',(-21.2185037002406,67.1401796386557,29.8876785104642));
#16042=CARTESIAN_POINT('Ctrl Pts',(-21.5026166107437,66.8365497359656,29.9156124614396));
#16043=CARTESIAN_POINT('Ctrl Pts',(-21.6620166519365,66.4162233683915,29.9435464124149));
#16044=CARTESIAN_POINT('Ctrl Pts',(-21.6658100649286,65.9984774013953,29.9714803633902));
#16045=CARTESIAN_POINT('Origin',(-20.,66.,30.));
#16046=CARTESIAN_POINT('',(-21.6685540970378,66.0005306220524,30.6714803633902));
#16047=CARTESIAN_POINT('',(-21.6649961639659,66.0014338848797,30.4785196366098));
#16048=CARTESIAN_POINT('',(-21.666,66.,30.));
#16049=CARTESIAN_POINT('Ctrl Pts',(-21.6649961639659,66.0014338848797,30.4785196366098));
#16050=CARTESIAN_POINT('Ctrl Pts',(-21.6663488715524,66.1661251314864,30.4675206849354));
#16051=CARTESIAN_POINT('Ctrl Pts',(-21.6438880271777,66.3304555717191,30.4565217332609));
#16052=CARTESIAN_POINT('Ctrl Pts',(-21.596100259124,66.4870573839289,30.4455227815864));
#16053=CARTESIAN_POINT('Ctrl Pts',(-21.4351514759174,67.0144909124171,30.4084784089226));
#16054=CARTESIAN_POINT('Ctrl Pts',(-20.9869101567667,67.4542557934131,30.3714340362587));
#16055=CARTESIAN_POINT('Ctrl Pts',(-20.4565003506185,67.6051069628847,30.3343896635948));
#16056=CARTESIAN_POINT('Ctrl Pts',(-19.9260905444702,67.7559581323562,30.297345290931));
#16057=CARTESIAN_POINT('Ctrl Pts',(-19.3135122513245,67.6178955903034,30.2603009182671));
#16058=CARTESIAN_POINT('Ctrl Pts',(-18.8990933535481,67.2540994730139,30.2232565456033));
#16059=CARTESIAN_POINT('Ctrl Pts',(-18.4846744557717,66.8903033557244,30.1862121729394));
#16060=CARTESIAN_POINT('Ctrl Pts',(-18.2684149533647,66.3007736631982,30.1491678002756));
#16061=CARTESIAN_POINT('Ctrl Pts',(-18.3492794505739,65.7552907845666,30.1121234276117));
#16062=CARTESIAN_POINT('Ctrl Pts',(-18.4301439477832,65.209807905935,30.0750790549479));
#16063=CARTESIAN_POINT('Ctrl Pts',(-18.8081324446088,64.7083718411979,30.038034682284));
#16064=CARTESIAN_POINT('Ctrl Pts',(-19.3102699661622,64.4804496017448,30.0009903096202));
#16065=CARTESIAN_POINT('Ctrl Pts',(-19.8124074877155,64.2525273622916,29.9639459369563));
#16066=CARTESIAN_POINT('Ctrl Pts',(-20.4386940339967,64.2981189481223,29.9269015642924));
#16067=CARTESIAN_POINT('Ctrl Pts',(-20.9025285562284,64.5963607523271,29.8898571916286));
#16068=CARTESIAN_POINT('Ctrl Pts',(-21.3672163340203,64.8951511928785,29.852744673289));
#16069=CARTESIAN_POINT('Ctrl Pts',(-21.6688529243389,65.4475222434498,29.8156321549494));
#16070=CARTESIAN_POINT('Ctrl Pts',(-21.6687600243793,65.9999810464372,29.7785196366098));
#16071=CARTESIAN_POINT('Ctrl Pts',(-21.6658100649286,65.9984774013953,29.9714803633902));
#16072=CARTESIAN_POINT('Ctrl Pts',(-21.66704725447,65.8622330898984,29.9805907850787));
#16073=CARTESIAN_POINT('Ctrl Pts',(-21.6517328312273,65.7262632512288,29.9897012067673));
#16074=CARTESIAN_POINT('Ctrl Pts',(-21.6187950560616,65.5947057336016,29.9988116284558));
#16075=CARTESIAN_POINT('Ctrl Pts',(-21.4848650076323,65.0597726782143,30.0358560011197));
#16076=CARTESIAN_POINT('Ctrl Pts',(-21.0595574381662,64.5977911914591,30.0729003737835));
#16077=CARTESIAN_POINT('Ctrl Pts',(-20.5375014614225,64.4201730933822,30.1099447464474));
#16078=CARTESIAN_POINT('Ctrl Pts',(-20.0154454846788,64.2425549953053,30.1469891191112));
#16079=CARTESIAN_POINT('Ctrl Pts',(-19.3966411006575,64.3493002859068,30.1840334917751));
#16080=CARTESIAN_POINT('Ctrl Pts',(-18.9642653734382,64.6915602194806,30.2210778644389));
#16081=CARTESIAN_POINT('Ctrl Pts',(-18.531889646219,65.0338201530543,30.2581222371028));
#16082=CARTESIAN_POINT('Ctrl Pts',(-18.2859425758018,65.6115947296003,30.2951666097666));
#16083=CARTESIAN_POINT('Ctrl Pts',(-18.3389743818009,66.1604829323982,30.3322109824305));
#16084=CARTESIAN_POINT('Ctrl Pts',(-18.3920061877999,66.7093711351962,30.3692553550943));
#16085=CARTESIAN_POINT('Ctrl Pts',(-18.7440168702152,67.229372964246,30.4062997277582));
#16086=CARTESIAN_POINT('Ctrl Pts',(-19.2339194132707,67.4825253490384,30.443344100422));
#16087=CARTESIAN_POINT('Ctrl Pts',(-19.7238219563261,67.7356777338307,30.4803884730859));
#16088=CARTESIAN_POINT('Ctrl Pts',(-20.3516163600219,67.7219806743655,30.5174328457498));
#16089=CARTESIAN_POINT('Ctrl Pts',(-20.8300115503532,67.4477022146095,30.5544772184136));
#16090=CARTESIAN_POINT('Ctrl Pts',(-21.3084067406845,67.1734237548535,30.5915215910775));
#16091=CARTESIAN_POINT('Ctrl Pts',(-21.6374027176515,66.6385638948067,30.6285659637413));
#16092=CARTESIAN_POINT('Ctrl Pts',(-21.6664444476162,66.087885032366,30.6656103364051));
#16093=CARTESIAN_POINT('Ctrl Pts',(-21.6679784254409,66.0587982952976,30.6675670120668));
#16094=CARTESIAN_POINT('Ctrl Pts',(-21.6686755521249,66.0296674243309,30.6695236877285));
#16095=CARTESIAN_POINT('Ctrl Pts',(-21.6685540970378,66.0005306220524,30.6714803633902));
#16096=CARTESIAN_POINT('Origin',(-20.,66.,30.));
#16097=CARTESIAN_POINT('',(-21.6642459336481,66.0011866317831,31.3714803633902));
#16098=CARTESIAN_POINT('',(-21.6637024058618,65.9991726429868,31.1785196366098));
#16099=CARTESIAN_POINT('',(-21.666,66.,30.));
#16100=CARTESIAN_POINT('Ctrl Pts',(-21.6637024058618,65.9991726429868,31.1785196366098));
#16101=CARTESIAN_POINT('Ctrl Pts',(-21.6622143947745,66.3302224245355,31.1564535875851));
#16102=CARTESIAN_POINT('Ctrl Pts',(-21.566629777932,66.6620639402334,31.1343875385604));
#16103=CARTESIAN_POINT('Ctrl Pts',(-21.3827355500634,66.9342394398688,31.1123214895358));
#16104=CARTESIAN_POINT('Ctrl Pts',(-21.0740148406931,67.3911663064406,31.0752771168719));
#16105=CARTESIAN_POINT('Ctrl Pts',(-20.5164065063464,67.6799332993925,31.038232744208));
#16106=CARTESIAN_POINT('Ctrl Pts',(-19.9650830944454,67.6683949598707,31.0011883715442));
#16107=CARTESIAN_POINT('Ctrl Pts',(-19.4137596825443,67.6568566203489,30.9641439988803));
#16108=CARTESIAN_POINT('Ctrl Pts',(-18.868721193089,67.3450129483535,30.9270996262165));
#16109=CARTESIAN_POINT('Ctrl Pts',(-18.579387965107,66.8755697452132,30.8900552535526));
#16110=CARTESIAN_POINT('Ctrl Pts',(-18.290054737125,66.4061265420728,30.8530108808888));
#16111=CARTESIAN_POINT('Ctrl Pts',(-18.2564267706164,65.7790838077876,30.8159665082249));
#16112=CARTESIAN_POINT('Ctrl Pts',(-18.4938928848475,65.2813886376472,30.7789221355611));
#16113=CARTESIAN_POINT('Ctrl Pts',(-18.7313589990786,64.7836934675067,30.7418777628972));
#16114=CARTESIAN_POINT('Ctrl Pts',(-19.2399191940493,64.4153458615111,30.7048333902334));
#16115=CARTESIAN_POINT('Ctrl Pts',(-19.786846316174,64.3449089331741,30.6677890175695));
#16116=CARTESIAN_POINT('Ctrl Pts',(-20.3337734382987,64.2744720048371,30.6307446449057));
#16117=CARTESIAN_POINT('Ctrl Pts',(-20.9190674875773,64.5019457541587,30.5937002722418));
#16118=CARTESIAN_POINT('Ctrl Pts',(-21.2748863885853,64.9232337168097,30.556655899578));
#16119=CARTESIAN_POINT('Ctrl Pts',(-21.5250580720641,65.2194358537596,30.5306104785886));
#16120=CARTESIAN_POINT('Ctrl Pts',(-21.6617929642784,65.6114464589783,30.5045650575992));
#16121=CARTESIAN_POINT('Ctrl Pts',(-21.6649961639659,66.0014338848797,30.4785196366098));
#16122=CARTESIAN_POINT('Ctrl Pts',(-21.6685540970378,66.0005306220524,30.6714803633902));
#16123=CARTESIAN_POINT('Ctrl Pts',(-21.6663761278529,65.4780407122621,30.7065680603924));
#16124=CARTESIAN_POINT('Ctrl Pts',(-21.4009689299932,64.9536434858154,30.7416557573946));
#16125=CARTESIAN_POINT('Ctrl Pts',(-20.9776817958066,64.6476320093801,30.7767434543967));
#16126=CARTESIAN_POINT('Ctrl Pts',(-20.5307899310697,64.3245557136693,30.8137878270606));
#16127=CARTESIAN_POINT('Ctrl Pts',(-19.9079187186333,64.2449009870822,30.8508321997244));
#16128=CARTESIAN_POINT('Ctrl Pts',(-19.3941062832943,64.4451194000948,30.8878765723883));
#16129=CARTESIAN_POINT('Ctrl Pts',(-18.8802938479553,64.6453378131074,30.9249209450521));
#16130=CARTESIAN_POINT('Ctrl Pts',(-18.4755401897137,65.1254293657198,30.961965317716));
#16131=CARTESIAN_POINT('Ctrl Pts',(-18.3650685480553,65.6656947153468,30.9990096903798));
#16132=CARTESIAN_POINT('Ctrl Pts',(-18.2545969063969,66.2059600649738,31.0360540630437));
#16133=CARTESIAN_POINT('Ctrl Pts',(-18.4384072813217,66.8063992116154,31.0730984357075));
#16134=CARTESIAN_POINT('Ctrl Pts',(-18.8323844279111,67.1922393852412,31.1101428083714));
#16135=CARTESIAN_POINT('Ctrl Pts',(-19.2263615745004,67.5780795588669,31.1471871810352));
#16136=CARTESIAN_POINT('Ctrl Pts',(-19.8305054927545,67.7493207594768,31.1842315536991));
#16137=CARTESIAN_POINT('Ctrl Pts',(-20.3683480362437,67.6275996436778,31.2212759263629));
#16138=CARTESIAN_POINT('Ctrl Pts',(-20.9061905797328,67.5058785278788,31.2583202990268));
#16139=CARTESIAN_POINT('Ctrl Pts',(-21.3777317484572,67.091195095671,31.2953646716907));
#16140=CARTESIAN_POINT('Ctrl Pts',(-21.5671850237686,66.5733166465229,31.3324090443545));
#16141=CARTESIAN_POINT('Ctrl Pts',(-21.6337915358132,66.3912449610159,31.3454328173664));
#16142=CARTESIAN_POINT('Ctrl Pts',(-21.6655311270496,66.1964180578357,31.3584565903783));
#16143=CARTESIAN_POINT('Ctrl Pts',(-21.6642459336481,66.0011866317831,31.3714803633902));
#16144=CARTESIAN_POINT('Origin',(-20.,66.,30.));
#16145=CARTESIAN_POINT('',(-21.6642690977371,65.998802450892,32.0714803633902));
#16146=CARTESIAN_POINT('',(-21.6680157746037,65.999012657191,31.8785196366098));
#16147=CARTESIAN_POINT('',(-21.666,66.,30.));
#16148=CARTESIAN_POINT('Ctrl Pts',(-21.6680157746037,65.999012657191,31.8785196366098));
#16149=CARTESIAN_POINT('Ctrl Pts',(-21.664548415959,66.4928187802733,31.8453864902349));
#16150=CARTESIAN_POINT('Ctrl Pts',(-21.4314257129962,66.9894689300238,31.81225334386));
#16151=CARTESIAN_POINT('Ctrl Pts',(-21.0474729631797,67.2990617090127,31.7791201974851));
#16152=CARTESIAN_POINT('Ctrl Pts',(-20.6181962326036,67.6452005920857,31.7420758248213));
#16153=CARTESIAN_POINT('Ctrl Pts',(-20.000377985162,67.757512852679,31.7050314521574));
#16154=CARTESIAN_POINT('Ctrl Pts',(-19.4767440094288,67.5846021900613,31.6679870794935));
#16155=CARTESIAN_POINT('Ctrl Pts',(-18.9531100336955,67.4116915274435,31.6309427068297));
#16156=CARTESIAN_POINT('Ctrl Pts',(-18.5236603296707,66.9535579416147,31.5938983341658));
#16157=CARTESIAN_POINT('Ctrl Pts',(-18.3849195334037,66.4198523774313,31.556853961502));
#16158=CARTESIAN_POINT('Ctrl Pts',(-18.2461787371368,65.8861468132478,31.5198095888381));
#16159=CARTESIAN_POINT('Ctrl Pts',(-18.3981468486279,65.2768692707098,31.4827652161743));
#16160=CARTESIAN_POINT('Ctrl Pts',(-18.7712802693553,64.8708371437477,31.4457208435104));
#16161=CARTESIAN_POINT('Ctrl Pts',(-19.1444136900827,64.4648050167856,31.4086764708466));
#16162=CARTESIAN_POINT('Ctrl Pts',(-19.7387124200466,64.2620183053994,31.3716320981827));
#16163=CARTESIAN_POINT('Ctrl Pts',(-20.2822136647303,64.3552761995232,31.3345877255189));
#16164=CARTESIAN_POINT('Ctrl Pts',(-20.825714909414,64.4485340936469,31.297543352855));
#16165=CARTESIAN_POINT('Ctrl Pts',(-21.3184186688175,64.8378365932804,31.2604989801912));
#16166=CARTESIAN_POINT('Ctrl Pts',(-21.5348540063224,65.345031213193,31.2234546075273));
#16167=CARTESIAN_POINT('Ctrl Pts',(-21.6223663138332,65.5501075748318,31.2084762838881));
#16168=CARTESIAN_POINT('Ctrl Pts',(-21.6647124603405,65.7744577081488,31.193497960249));
#16169=CARTESIAN_POINT('Ctrl Pts',(-21.6637024058618,65.9991726429868,31.1785196366098));
#16170=CARTESIAN_POINT('Ctrl Pts',(-21.6642459336481,66.0011866317831,31.3714803633902));
#16171=CARTESIAN_POINT('Ctrl Pts',(-21.6618755670773,65.6411084946407,31.3955009630422));
#16172=CARTESIAN_POINT('Ctrl Pts',(-21.5471652967987,65.2796542982436,31.4195215626941));
#16173=CARTESIAN_POINT('Ctrl Pts',(-21.3316725937391,64.9943116889468,31.4435421623461));
#16174=CARTESIAN_POINT('Ctrl Pts',(-20.9993415064995,64.5542586466071,31.4805865350099));
#16175=CARTESIAN_POINT('Ctrl Pts',(-20.4273139501218,64.2952260280159,31.5176309076738));
#16176=CARTESIAN_POINT('Ctrl Pts',(-19.877360991797,64.3357522571528,31.5546752803376));
#16177=CARTESIAN_POINT('Ctrl Pts',(-19.3274080334722,64.3762784862898,31.5917196530015));
#16178=CARTESIAN_POINT('Ctrl Pts',(-18.7995296732003,64.7163635631548,31.6287640256653));
#16179=CARTESIAN_POINT('Ctrl Pts',(-18.5352934371866,65.2003778637654,31.6658083983292));
#16180=CARTESIAN_POINT('Ctrl Pts',(-18.2710572011729,65.6843921643761,31.7028527709931));
#16181=CARTESIAN_POINT('Ctrl Pts',(-18.2704630894175,66.3123356887323,31.7398971436569));
#16182=CARTESIAN_POINT('Ctrl Pts',(-18.5337829791516,66.7968491222805,31.7769415163208));
#16183=CARTESIAN_POINT('Ctrl Pts',(-18.7971028688856,67.2813625558288,31.8139858889846));
#16184=CARTESIAN_POINT('Ctrl Pts',(-19.3243367601092,67.622445898569,31.8510302616485));
#16185=CARTESIAN_POINT('Ctrl Pts',(-19.8742120483366,67.6640127004086,31.8880746343123));
#16186=CARTESIAN_POINT('Ctrl Pts',(-20.4240873365639,67.7055795022482,31.9251190069762));
#16187=CARTESIAN_POINT('Ctrl Pts',(-20.996604021795,67.4476297631871,31.96216337964));
#16188=CARTESIAN_POINT('Ctrl Pts',(-21.3297672018495,67.0082063602211,31.9992077523039));
#16189=CARTESIAN_POINT('Ctrl Pts',(-21.5464314453758,66.7224384696162,32.023298622666));
#16190=CARTESIAN_POINT('Ctrl Pts',(-21.6618677757111,66.3599213361594,32.0473894930281));
#16191=CARTESIAN_POINT('Ctrl Pts',(-21.6642690977371,65.998802450892,32.0714803633902));
#16192=CARTESIAN_POINT('Origin',(-20.,66.,30.));
#16193=CARTESIAN_POINT('',(-21.668567971344,65.9994875421907,32.7714803633902));
#16194=CARTESIAN_POINT('',(-21.6666947552498,66.0014544403163,32.5785196366098));
#16195=CARTESIAN_POINT('',(-21.666,66.,30.));
#16196=CARTESIAN_POINT('Ctrl Pts',(-21.6666947552498,66.0014544403163,32.5785196366098));
#16197=CARTESIAN_POINT('Ctrl Pts',(-21.6676729422518,66.1083233141787,32.5713637655485));
#16198=CARTESIAN_POINT('Ctrl Pts',(-21.6582744172421,66.2150208253731,32.5642078944873));
#16199=CARTESIAN_POINT('Ctrl Pts',(-21.6378750618295,66.3195719234416,32.557052023426));
#16200=CARTESIAN_POINT('Ctrl Pts',(-21.5322720796714,66.8608099930084,32.5200076507622));
#16201=CARTESIAN_POINT('Ctrl Pts',(-21.1318572413143,67.3445262197104,32.4829632780983));
#16202=CARTESIAN_POINT('Ctrl Pts',(-20.6198682568773,67.549362538766,32.4459189054344));
#16203=CARTESIAN_POINT('Ctrl Pts',(-20.1078792724403,67.7541988578216,32.4088745327706));
#16204=CARTESIAN_POINT('Ctrl Pts',(-19.4843161419233,67.6801552692307,32.3718301601068));
#16205=CARTESIAN_POINT('Ctrl Pts',(-19.034533625454,67.3611155762963,32.3347857874429));
#16206=CARTESIAN_POINT('Ctrl Pts',(-18.5847511089847,67.0420758833619,32.2977414147791));
#16207=CARTESIAN_POINT('Ctrl Pts',(-18.308749206563,66.4780400860841,32.2606970421152));
#16208=CARTESIAN_POINT('Ctrl Pts',(-18.3328318204015,65.9271220654133,32.2236526694513));
#16209=CARTESIAN_POINT('Ctrl Pts',(-18.35691443424,65.3762040447425,32.1866082967875));
#16210=CARTESIAN_POINT('Ctrl Pts',(-18.6810815643387,64.8384038006788,32.1495639241236));
#16211=CARTESIAN_POINT('Ctrl Pts',(-19.1569879524176,64.5598293087115,32.1125195514598));
#16212=CARTESIAN_POINT('Ctrl Pts',(-19.6328943404965,64.2812548167441,32.0754751787959));
#16213=CARTESIAN_POINT('Ctrl Pts',(-20.2605399865555,64.2619060768732,32.0384308061321));
#16214=CARTESIAN_POINT('Ctrl Pts',(-20.752701891012,64.510637453243,32.0013864334682));
#16215=CARTESIAN_POINT('Ctrl Pts',(-21.2448637954686,64.7593688296128,31.9643420608044));
#16216=CARTESIAN_POINT('Ctrl Pts',(-21.6015419583227,65.2761803222235,31.9272976881405));
#16217=CARTESIAN_POINT('Ctrl Pts',(-21.6595134328945,65.8245688213051,31.8902533154767));
#16218=CARTESIAN_POINT('Ctrl Pts',(-21.6656341886004,65.8824688843898,31.8863420891877));
#16219=CARTESIAN_POINT('Ctrl Pts',(-21.6684250814691,65.9407209553286,31.8824308628987));
#16220=CARTESIAN_POINT('Ctrl Pts',(-21.6680157746037,65.999012657191,31.8785196366098));
#16221=CARTESIAN_POINT('Ctrl Pts',(-21.6642690977371,65.998802450892,32.0714803633902));
#16222=CARTESIAN_POINT('Ctrl Pts',(-21.6655602727724,65.8046312050549,32.0844338656919));
#16223=CARTESIAN_POINT('Ctrl Pts',(-21.6341714211142,65.610864212633,32.0973873679937));
#16224=CARTESIAN_POINT('Ctrl Pts',(-21.5682670731027,65.4296498765436,32.1103408702954));
#16225=CARTESIAN_POINT('Ctrl Pts',(-21.3797940894235,64.911413862703,32.1473852429593));
#16226=CARTESIAN_POINT('Ctrl Pts',(-20.9090384471872,64.4958389018927,32.1844296156231));
#16227=CARTESIAN_POINT('Ctrl Pts',(-20.3714271926618,64.3731002746154,32.221473988287));
#16228=CARTESIAN_POINT('Ctrl Pts',(-19.8338159381365,64.250361647338,32.2585183609508));
#16229=CARTESIAN_POINT('Ctrl Pts',(-19.2293490713221,64.4204593535935,32.2955627336147));
#16230=CARTESIAN_POINT('Ctrl Pts',(-18.834642526265,64.8055533355086,32.3326071062785));
#16231=CARTESIAN_POINT('Ctrl Pts',(-18.4399359812079,65.1906473174238,32.3696514789424));
#16232=CARTESIAN_POINT('Ctrl Pts',(-18.254989757908,65.7907375749985,32.4066958516063));
#16233=CARTESIAN_POINT('Ctrl Pts',(-18.3644388878536,66.3312109967065,32.4437402242701));
#16234=CARTESIAN_POINT('Ctrl Pts',(-18.4738880177993,66.8716844184144,32.480784596934));
#16235=CARTESIAN_POINT('Ctrl Pts',(-18.8777325009904,67.3525410042557,32.5178289695978));
#16236=CARTESIAN_POINT('Ctrl Pts',(-19.3911651543367,67.5537313173818,32.5548733422616));
#16237=CARTESIAN_POINT('Ctrl Pts',(-19.904597807683,67.7549216305078,32.5919177149255));
#16238=CARTESIAN_POINT('Ctrl Pts',(-20.5276186311845,67.6764456709187,32.6289620875894));
#16239=CARTESIAN_POINT('Ctrl Pts',(-20.9751210350767,67.3542155821184,32.6660064602532));
#16240=CARTESIAN_POINT('Ctrl Pts',(-21.3998353421592,67.0483943670912,32.7011644279656));
#16241=CARTESIAN_POINT('Ctrl Pts',(-21.6664518819652,66.5230122439924,32.7363223956779));
#16242=CARTESIAN_POINT('Ctrl Pts',(-21.668567971344,65.9994875421907,32.7714803633902));
#16243=CARTESIAN_POINT('Origin',(-20.,66.,30.));
#16244=CARTESIAN_POINT('',(-21.6657785854137,66.0015219658715,33.4714803633902));
#16245=CARTESIAN_POINT('',(-21.6632990561475,66.0000736897326,33.2785196366098));
#16246=CARTESIAN_POINT('',(-21.666,66.,30.));
#16247=CARTESIAN_POINT('Ctrl Pts',(-21.6632990561475,66.0000736897326,33.2785196366098));
#16248=CARTESIAN_POINT('Ctrl Pts',(-21.6634069959719,66.2736326427316,33.2602966681983));
#16249=CARTESIAN_POINT('Ctrl Pts',(-21.5996813380736,66.5471442420865,33.2420736997869));
#16250=CARTESIAN_POINT('Ctrl Pts',(-21.4718464679376,66.7864025096638,33.2238507313754));
#16251=CARTESIAN_POINT('Ctrl Pts',(-21.2119786757195,67.2727762017491,33.1868063587115));
#16252=CARTESIAN_POINT('Ctrl Pts',(-20.6871836009889,67.6176001572505,33.1497619860477));
#16253=CARTESIAN_POINT('Ctrl Pts',(-20.1376177977875,67.6630761480344,33.1127176133838));
#16254=CARTESIAN_POINT('Ctrl Pts',(-19.5880519945861,67.7085521388184,33.07567324072));
#16255=CARTESIAN_POINT('Ctrl Pts',(-19.0137154629139,67.4546801648849,33.0386288680561));
#16256=CARTESIAN_POINT('Ctrl Pts',(-18.6774359025077,67.0176370376711,33.0015844953923));
#16257=CARTESIAN_POINT('Ctrl Pts',(-18.3411563421015,66.5805939104574,32.9645401227284));
#16258=CARTESIAN_POINT('Ctrl Pts',(-18.2429337529613,65.9603796299633,32.9274957500645));
#16259=CARTESIAN_POINT('Ctrl Pts',(-18.4277167248739,65.4408164566345,32.8904513774007));
#16260=CARTESIAN_POINT('Ctrl Pts',(-18.6124996967865,64.9212532833056,32.8534070047368));
#16261=CARTESIAN_POINT('Ctrl Pts',(-19.080288229752,64.5023412171419,32.816362632073));
#16262=CARTESIAN_POINT('Ctrl Pts',(-19.6170130850995,64.3757826637324,32.7793182594092));
#16263=CARTESIAN_POINT('Ctrl Pts',(-20.1537379404469,64.2492241103229,32.7422738867453));
#16264=CARTESIAN_POINT('Ctrl Pts',(-20.7593991181762,64.4150190696675,32.7052295140814));
#16265=CARTESIAN_POINT('Ctrl Pts',(-21.1568341440614,64.7972965055555,32.6681851414176));
#16266=CARTESIAN_POINT('Ctrl Pts',(-21.4774965430683,65.1057293101505,32.638296639815));
#16267=CARTESIAN_POINT('Ctrl Pts',(-21.6626090830058,65.5550866284368,32.6084081382124));
#16268=CARTESIAN_POINT('Ctrl Pts',(-21.6666947552498,66.0014544403163,32.5785196366098));
#16269=CARTESIAN_POINT('Ctrl Pts',(-21.668567971344,65.9994875421907,32.7714803633902));
#16270=CARTESIAN_POINT('Ctrl Pts',(-21.668681510372,65.9713977618654,32.7733667683417));
#16271=CARTESIAN_POINT('Ctrl Pts',(-21.6680335865054,65.9433133288179,32.7752531732932));
#16272=CARTESIAN_POINT('Ctrl Pts',(-21.6666077641248,65.9152684446987,32.7771395782448));
#16273=CARTESIAN_POINT('Ctrl Pts',(-21.6386081049976,65.3645356140905,32.8141839509086));
#16274=CARTESIAN_POINT('Ctrl Pts',(-21.31062480246,64.8290541708855,32.8512283235725));
#16275=CARTESIAN_POINT('Ctrl Pts',(-20.8327494704029,64.5538709616836,32.8882726962364));
#16276=CARTESIAN_POINT('Ctrl Pts',(-20.3548741383459,64.2786877524817,32.9253170689002));
#16277=CARTESIAN_POINT('Ctrl Pts',(-19.7271067767693,64.2638027772828,32.962361441564));
#16278=CARTESIAN_POINT('Ctrl Pts',(-19.2367260846697,64.5160276936372,32.9994058142279));
#16279=CARTESIAN_POINT('Ctrl Pts',(-18.74634539257,64.7682526099916,33.0364501868917));
#16280=CARTESIAN_POINT('Ctrl Pts',(-18.3933513699472,65.2875874178992,33.0734945595556));
#16281=CARTESIAN_POINT('Ctrl Pts',(-18.3392810284129,65.8363742889205,33.1105389322195));
#16282=CARTESIAN_POINT('Ctrl Pts',(-18.2852106868786,66.3851611599418,33.1475833048833));
#16283=CARTESIAN_POINT('Ctrl Pts',(-18.5300640264328,66.9634000940767,33.1846276775472));
#16284=CARTESIAN_POINT('Ctrl Pts',(-18.9617913402192,67.3064775752974,33.221672050211));
#16285=CARTESIAN_POINT('Ctrl Pts',(-19.3935186540056,67.6495550565182,33.2587164228749));
#16286=CARTESIAN_POINT('Ctrl Pts',(-20.0121199420242,67.7574710848249,33.2957607955387));
#16287=CARTESIAN_POINT('Ctrl Pts',(-20.534511080942,67.5808411621693,33.3328051682026));
#16288=CARTESIAN_POINT('Ctrl Pts',(-21.0569022198598,67.4042112395138,33.3698495408664));
#16289=CARTESIAN_POINT('Ctrl Pts',(-21.4830832096766,66.9430353658961,33.4068939135303));
#16290=CARTESIAN_POINT('Ctrl Pts',(-21.6180252422545,66.4083566963944,33.4439382861941));
#16291=CARTESIAN_POINT('Ctrl Pts',(-21.6514678734469,66.2758474907081,33.4531189785928));
#16292=CARTESIAN_POINT('Ctrl Pts',(-21.6670227490859,66.1388237789346,33.4622996709915));
#16293=CARTESIAN_POINT('Ctrl Pts',(-21.6657785854137,66.0015219658715,33.4714803633902));
#16294=CARTESIAN_POINT('Origin',(-20.,66.,30.));
#16295=CARTESIAN_POINT('',(-21.6633939316965,65.999580177356,34.1714803633902));
#16296=CARTESIAN_POINT('',(-21.6664242991574,65.998507036594,33.9785196366098));
#16297=CARTESIAN_POINT('',(-21.666,66.,30.));
#16298=CARTESIAN_POINT('Ctrl Pts',(-21.6664242991574,65.998507036594,33.9785196366098));
#16299=CARTESIAN_POINT('Ctrl Pts',(-21.6623854525421,66.4361202270654,33.9492295708481));
#16300=CARTESIAN_POINT('Ctrl Pts',(-21.4853948911407,66.8766244639417,33.9199395050864));
#16301=CARTESIAN_POINT('Ctrl Pts',(-21.1760642408071,67.1839061752964,33.8906494393247));
#16302=CARTESIAN_POINT('Ctrl Pts',(-20.7848408143887,67.5725382227907,33.8536050666609));
#16303=CARTESIAN_POINT('Ctrl Pts',(-20.1819298861659,67.7480712476131,33.816560693997));
#16304=CARTESIAN_POINT('Ctrl Pts',(-19.6432353607165,67.6301778814624,33.7795163213332));
#16305=CARTESIAN_POINT('Ctrl Pts',(-19.1045408352671,67.5122845153116,33.7424719486693));
#16306=CARTESIAN_POINT('Ctrl Pts',(-18.6300627125911,67.1009647581878,33.7054275760055));
#16307=CARTESIAN_POINT('Ctrl Pts',(-18.4369315199398,66.5844466264903,33.6683832033416));
#16308=CARTESIAN_POINT('Ctrl Pts',(-18.2438003272885,66.0679284947929,33.6313388306778));
#16309=CARTESIAN_POINT('Ctrl Pts',(-18.3320160646619,65.4462119885219,33.5942944580139));
#16310=CARTESIAN_POINT('Ctrl Pts',(-18.66120947423,65.0038068157843,33.5572500853501));
#16311=CARTESIAN_POINT('Ctrl Pts',(-18.990402883798,64.5614016430468,33.5202057126862));
#16312=CARTESIAN_POINT('Ctrl Pts',(-19.5605739655607,64.2983078038427,33.4831613400223));
#16313=CARTESIAN_POINT('Ctrl Pts',(-20.110801211816,64.3349222168409,33.4461169673585));
#16314=CARTESIAN_POINT('Ctrl Pts',(-20.6610284580713,64.3715366298392,33.4090725946946));
#16315=CARTESIAN_POINT('Ctrl Pts',(-21.1913118688192,64.7078592950398,33.3720282220308));
#16316=CARTESIAN_POINT('Ctrl Pts',(-21.4589833193403,65.1899823419746,33.3349838493669));
#16317=CARTESIAN_POINT('Ctrl Pts',(-21.5949811029387,65.4349381102391,33.3161624451146));
#16318=CARTESIAN_POINT('Ctrl Pts',(-21.6631875716174,65.7175311574189,33.2973410408622));
#16319=CARTESIAN_POINT('Ctrl Pts',(-21.6632990561475,66.0000736897326,33.2785196366098));
#16320=CARTESIAN_POINT('Ctrl Pts',(-21.6657785854137,66.0015219658715,33.4714803633902));
#16321=CARTESIAN_POINT('Ctrl Pts',(-21.662002510881,65.584806793107,33.4993440436554));
#16322=CARTESIAN_POINT('Ctrl Pts',(-21.5034836084249,65.1655299155204,33.5272077239205));
#16323=CARTESIAN_POINT('Ctrl Pts',(-21.220659016965,64.8621281087732,33.5550714041857));
#16324=CARTESIAN_POINT('Ctrl Pts',(-20.8446476837586,64.4587596560393,33.5921157768495));
#16325=CARTESIAN_POINT('Ctrl Pts',(-20.2489219420067,64.2602042159574,33.6291601495134));
#16326=CARTESIAN_POINT('Ctrl Pts',(-19.7060976147537,64.357324663287,33.6662045221773));
#16327=CARTESIAN_POINT('Ctrl Pts',(-19.1632732875006,64.4544451106166,33.7032488948411));
#16328=CARTESIAN_POINT('Ctrl Pts',(-18.6733503747463,64.8472414453578,33.7402932675049));
#16329=CARTESIAN_POINT('Ctrl Pts',(-18.4605272432548,65.3559623388724,33.7773376401688));
#16330=CARTESIAN_POINT('Ctrl Pts',(-18.2477041117633,65.8646832323871,33.8143820128327));
#16331=CARTESIAN_POINT('Ctrl Pts',(-18.3119807615347,66.4893286846752,33.8514263854965));
#16332=CARTESIAN_POINT('Ctrl Pts',(-18.6239429320858,66.9440486353022,33.8884707581604));
#16333=CARTESIAN_POINT('Ctrl Pts',(-18.9359051026368,67.3987685859291,33.9255151308242));
#16334=CARTESIAN_POINT('Ctrl Pts',(-19.4955527939675,67.6835630348949,33.9625595034881));
#16335=CARTESIAN_POINT('Ctrl Pts',(-20.0467802099533,67.6681044547283,33.9996038761519));
#16336=CARTESIAN_POINT('Ctrl Pts',(-20.5980076259392,67.6526458745618,34.0366482488158));
#16337=CARTESIAN_POINT('Ctrl Pts',(-21.1408147665801,67.3369342652628,34.0736926214796));
#16338=CARTESIAN_POINT('Ctrl Pts',(-21.4268023996106,66.865445438347,34.1107369941435));
#16339=CARTESIAN_POINT('Ctrl Pts',(-21.5831181109586,66.6077381011766,34.1309847838924));
#16340=CARTESIAN_POINT('Ctrl Pts',(-21.6627084923234,66.3034920156973,34.1512325736413));
#16341=CARTESIAN_POINT('Ctrl Pts',(-21.6633939316965,65.999580177356,34.1714803633902));
#16342=CARTESIAN_POINT('Origin',(-20.,66.,30.));
#16343=CARTESIAN_POINT('',(-21.6673174487995,65.9986976755605,34.8714803633902));
#16344=CARTESIAN_POINT('',(-21.6682089013646,66.0008588710179,34.6785196366098));
#16345=CARTESIAN_POINT('',(-21.666,66.,30.));
#16346=CARTESIAN_POINT('Ctrl Pts',(-21.6682089013646,66.0008588710179,34.6785196366098));
#16347=CARTESIAN_POINT('Ctrl Pts',(-21.6685189509142,66.0502166252967,34.6752068461617));
#16348=CARTESIAN_POINT('Ctrl Pts',(-21.6665182295093,66.0995488913109,34.6718940557137));
#16349=CARTESIAN_POINT('Ctrl Pts',(-21.6621249005774,66.1486671516306,34.6685812652656));
#16350=CARTESIAN_POINT('Ctrl Pts',(-21.6129977019998,66.697918656794,34.6315368926018));
#16351=CARTESIAN_POINT('Ctrl Pts',(-21.2646936272885,67.2204104220295,34.5944925199379));
#16352=CARTESIAN_POINT('Ctrl Pts',(-20.7766036444332,67.4770401441681,34.5574481472741));
#16353=CARTESIAN_POINT('Ctrl Pts',(-20.2885136615778,67.7336698663066,34.5204037746102));
#16354=CARTESIAN_POINT('Ctrl Pts',(-19.6606377705784,67.7244375453482,34.4833594019464));
#16355=CARTESIAN_POINT('Ctrl Pts',(-19.1803042509458,67.4535679671517,34.4463150292825));
#16356=CARTESIAN_POINT('Ctrl Pts',(-18.6999707313132,67.1826983889551,34.4092706566187));
#16357=CARTESIAN_POINT('Ctrl Pts',(-18.3671795830475,66.6501915535204,34.3722262839548));
#16358=CARTESIAN_POINT('Ctrl Pts',(-18.3342226273379,66.0997331214924,34.335181911291));
#16359=CARTESIAN_POINT('Ctrl Pts',(-18.3012656716283,65.5492746894643,34.2981375386271));
#16360=CARTESIAN_POINT('Ctrl Pts',(-18.5681429084748,64.9808646608429,34.2610931659633));
#16361=CARTESIAN_POINT('Ctrl Pts',(-19.0127260408984,64.6546186242835,34.2240487932994));
#16362=CARTESIAN_POINT('Ctrl Pts',(-19.4573091733219,64.3283725877241,34.1870044206356));
#16363=CARTESIAN_POINT('Ctrl Pts',(-20.0795982013227,64.2442905432266,34.1499600479717));
#16364=CARTESIAN_POINT('Ctrl Pts',(-20.5948214298447,64.4408501024346,34.1129156753078));
#16365=CARTESIAN_POINT('Ctrl Pts',(-21.1100446583667,64.6374096616425,34.075871302644));
#16366=CARTESIAN_POINT('Ctrl Pts',(-21.5182020874101,65.114610824556,34.0388269299802));
#16367=CARTESIAN_POINT('Ctrl Pts',(-21.6325128396248,65.6540769410959,34.0017825573163));
#16368=CARTESIAN_POINT('Ctrl Pts',(-21.6564409180656,65.7670005926563,33.9940282504141));
#16369=CARTESIAN_POINT('Ctrl Pts',(-21.6674935509796,65.8826525004193,33.986273943512));
#16370=CARTESIAN_POINT('Ctrl Pts',(-21.6664242991574,65.998507036594,33.9785196366098));
#16371=CARTESIAN_POINT('Ctrl Pts',(-21.6633939316965,65.999580177356,34.1714803633902));
#16372=CARTESIAN_POINT('Ctrl Pts',(-21.6639625389079,65.7474696776501,34.1882769463052));
#16373=CARTESIAN_POINT('Ctrl Pts',(-21.6102322705569,65.495589191975,34.2050735292201));
#16374=CARTESIAN_POINT('Ctrl Pts',(-21.5009588723762,65.270696659075,34.2218701121351));
#16375=CARTESIAN_POINT('Ctrl Pts',(-21.2599595866913,64.7747027512516,34.2589144847989));
#16376=CARTESIAN_POINT('Ctrl Pts',(-20.7487928899015,64.4099809801376,34.2959588574628));
#16377=CARTESIAN_POINT('Ctrl Pts',(-20.2013787127083,64.3434350705321,34.3330032301266));
#16378=CARTESIAN_POINT('Ctrl Pts',(-19.6539645355152,64.2768891609266,34.3700476027905));
#16379=CARTESIAN_POINT('Ctrl Pts',(-19.0703028779187,64.5085191128297,34.4070919754543));
#16380=CARTESIAN_POINT('Ctrl Pts',(-18.7174888195492,64.932326771598,34.4441363481182));
#16381=CARTESIAN_POINT('Ctrl Pts',(-18.3646747611796,65.3561344303663,34.481180720782));
#16382=CARTESIAN_POINT('Ctrl Pts',(-18.242708302037,65.9721197959998,34.5182250934459));
#16383=CARTESIAN_POINT('Ctrl Pts',(-18.4074036566907,66.4983953048516,34.5552694661097));
#16384=CARTESIAN_POINT('Ctrl Pts',(-18.5720990113444,67.0246708137035,34.5923138387736));
#16385=CARTESIAN_POINT('Ctrl Pts',(-19.0234561797943,67.4612364657736,34.6293582114375));
#16386=CARTESIAN_POINT('Ctrl Pts',(-19.554925313721,67.6083122994716,34.6664025841013));
#16387=CARTESIAN_POINT('Ctrl Pts',(-20.0863944476476,67.7553881331697,34.7034469567652));
#16388=CARTESIAN_POINT('Ctrl Pts',(-20.697975547051,67.6129741484956,34.740491329429));
#16389=CARTESIAN_POINT('Ctrl Pts',(-21.1097969163446,67.2462396496305,34.7775357020928));
#16390=CARTESIAN_POINT('Ctrl Pts',(-21.4579237371563,66.9362263169302,34.808850589192));
#16391=CARTESIAN_POINT('Ctrl Pts',(-21.6633041613515,66.4659156857186,34.8401654762911));
#16392=CARTESIAN_POINT('Ctrl Pts',(-21.6673174487995,65.9986976755605,34.8714803633902));
#16393=CARTESIAN_POINT('Origin',(-20.,66.,30.));
#16394=CARTESIAN_POINT('',(-21.6674772588494,66.0012131718681,35.5714803633902));
#16395=CARTESIAN_POINT('',(-21.6638441182547,66.0009441583361,35.3785196366098));
#16396=CARTESIAN_POINT('',(-21.666,66.,30.));
#16397=CARTESIAN_POINT('',(-18.7309291201476,67.0793586530486,36.));
#16398=CARTESIAN_POINT('Ctrl Pts',(-21.6674772588494,66.0012131718681,35.5714803633902));
#16399=CARTESIAN_POINT('Ctrl Pts',(-21.6635425119738,65.5283747294322,35.6031871242686));
#16400=CARTESIAN_POINT('Ctrl Pts',(-21.4523796053324,65.0525513983493,35.6348938851469));
#16401=CARTESIAN_POINT('Ctrl Pts',(-21.0965954523948,64.7422676947146,35.6666006460253));
#16402=CARTESIAN_POINT('Ctrl Pts',(-20.6809175217517,64.379749896285,35.7036450186892));
#16403=CARTESIAN_POINT('Ctrl Pts',(-20.0678279157583,64.2431978949171,35.740689391353));
#16404=CARTESIAN_POINT('Ctrl Pts',(-19.5379531300011,64.3961906766735,35.7777337640169));
#16405=CARTESIAN_POINT('Ctrl Pts',(-19.0080783442439,64.5491834584299,35.8147781366807));
#16406=CARTESIAN_POINT('Ctrl Pts',(-18.5614183787227,64.9917210233105,35.8518225093446));
#16407=CARTESIAN_POINT('Ctrl Pts',(-18.4024068180897,65.5187702873923,35.8888668820084));
#16408=CARTESIAN_POINT('Ctrl Pts',(-18.2433952574568,66.045819551474,35.9259112546723));
#16409=CARTESIAN_POINT('Ctrl Pts',(-18.372032101712,66.6573805147568,35.9629556273362));
#16410=CARTESIAN_POINT('Ctrl Pts',(-18.7309291201477,67.0793586530486,36.));
#16411=CARTESIAN_POINT('',(-21.2714721605028,67.0812049688959,36.));
#16412=CARTESIAN_POINT('Origin',(-20.,66.,36.));
#16413=CARTESIAN_POINT('Ctrl Pts',(-21.271473618129,67.0812060896471,36.));
#16414=CARTESIAN_POINT('Ctrl Pts',(-20.9206573555038,67.4926760200616,35.9636818543909));
#16415=CARTESIAN_POINT('Ctrl Pts',(-20.350790378308,67.7187175367081,35.9273637087819));
#16416=CARTESIAN_POINT('Ctrl Pts',(-19.8134508504095,67.6581953046217,35.8910455631728));
#16417=CARTESIAN_POINT('Ctrl Pts',(-19.2653665420103,67.5964628542926,35.854001190509));
#16418=CARTESIAN_POINT('Ctrl Pts',(-18.7511235436386,67.2365916665876,35.8169568178451));
#16419=CARTESIAN_POINT('Ctrl Pts',(-18.5057149733845,66.7428459347189,35.7799124451812));
#16420=CARTESIAN_POINT('Ctrl Pts',(-18.2603064031304,66.2491002028503,35.7428680725174));
#16421=CARTESIAN_POINT('Ctrl Pts',(-18.2837322609937,65.6214799268181,35.7058236998535));
#16422=CARTESIAN_POINT('Ctrl Pts',(-18.5654400102027,65.147406193219,35.6687793271897));
#16423=CARTESIAN_POINT('Ctrl Pts',(-18.8471477594117,64.6733324596199,35.6317349545258));
#16424=CARTESIAN_POINT('Ctrl Pts',(-19.3871373999664,64.352805268454,35.594690581862));
#16425=CARTESIAN_POINT('Ctrl Pts',(-19.9382150015654,64.3323990640615,35.5576462091981));
#16426=CARTESIAN_POINT('Ctrl Pts',(-20.4892926031645,64.3119928596691,35.5206018365343));
#16427=CARTESIAN_POINT('Ctrl Pts',(-21.051458165808,64.5917076420502,35.4835574638704));
#16428=CARTESIAN_POINT('Ctrl Pts',(-21.3674958173659,65.0435931347764,35.4465130912065));
#16429=CARTESIAN_POINT('Ctrl Pts',(-21.5608539458915,65.3200656776861,35.423848606341));
#16430=CARTESIAN_POINT('Ctrl Pts',(-21.6620805871735,65.6609857817599,35.4011841214754));
#16431=CARTESIAN_POINT('Ctrl Pts',(-21.6638441182547,66.0009441583361,35.3785196366098));
#16432=CARTESIAN_POINT('Origin',(-20.,66.,37.5459252805377));
#16433=CARTESIAN_POINT('',(-22.0554079166885,66.0018230931942,25.3540747194623));
#16434=CARTESIAN_POINT('',(-22.0529265634941,65.9984939060226,25.2959252805377));
#16435=CARTESIAN_POINT('',(-22.05475,66.0000000000002,37.5459252805377));
#16436=CARTESIAN_POINT('',(-18.1825721112405,66.9586205879593,25.));
#16437=CARTESIAN_POINT('Ctrl Pts',(-22.0529265634941,65.9984939060226,25.2959252805377));
#16438=CARTESIAN_POINT('Ctrl Pts',(-22.0499365185657,66.4524189410876,25.2713722656861));
#16439=CARTESIAN_POINT('Ctrl Pts',(-21.6783090895603,67.5959821141663,25.2097748781708));
#16440=CARTESIAN_POINT('Ctrl Pts',(-19.7840045183826,68.4179596733709,25.1111331179915));
#16441=CARTESIAN_POINT('Ctrl Pts',(-18.5013225746364,67.5629326473987,25.0370443726639));
#16442=CARTESIAN_POINT('Ctrl Pts',(-18.1825721112405,66.9586205879592,25.));
#16443=CARTESIAN_POINT('',(-17.9429021015473,65.924544644241,25.));
#16444=CARTESIAN_POINT('Origin',(-20.,66.,25.));
#16445=CARTESIAN_POINT('Ctrl Pts',(-22.0554079166885,66.0018230931942,25.3540747194623));
#16446=CARTESIAN_POINT('Ctrl Pts',(-22.0567024970405,66.1421866271351,25.3464567039117));
#16447=CARTESIAN_POINT('Ctrl Pts',(-21.9795741683388,66.9636910851773,25.3017943156971));
#16448=CARTESIAN_POINT('Ctrl Pts',(-20.8736248136923,68.2659592866881,25.2200875548188));
#16449=CARTESIAN_POINT('Ctrl Pts',(-18.5861502173631,67.9651132068328,25.109680663882));
#16450=CARTESIAN_POINT('Ctrl Pts',(-17.9193181049043,66.5910224347197,25.0363181456091));
#16451=CARTESIAN_POINT('Ctrl Pts',(-17.9428998421776,65.9245444497166,25.));
#16452=CARTESIAN_POINT('Origin',(-20.,66.,37.5459252805377));
#16453=CARTESIAN_POINT('',(-22.0514168260403,65.9999504085468,26.0540747194623));
#16454=CARTESIAN_POINT('',(-22.0580137571954,65.9995169080372,25.9959252805377));
#16455=CARTESIAN_POINT('',(-22.05475,66.0000000000002,37.5459252805377));
#16456=CARTESIAN_POINT('Ctrl Pts',(-22.0580137571954,65.9995169080372,25.9959252805377));
#16457=CARTESIAN_POINT('Ctrl Pts',(-22.055944731254,66.6536075471323,25.9603051683359));
#16458=CARTESIAN_POINT('Ctrl Pts',(-21.3649311540752,67.9917158703155,25.8876406834703));
#16459=CARTESIAN_POINT('Ctrl Pts',(-19.0858252973621,68.2499869305541,25.777931825941));
#16460=CARTESIAN_POINT('Ctrl Pts',(-17.6139705839552,66.4524069049006,25.6667987079493));
#16461=CARTESIAN_POINT('Ctrl Pts',(-18.3256043606965,64.2406215522943,25.5556655899578));
#16462=CARTESIAN_POINT('Ctrl Pts',(-20.5703082087302,63.6393771341005,25.4445324719662));
#16463=CARTESIAN_POINT('Ctrl Pts',(-21.9115053131723,64.8537201864073,25.3579523688262));
#16464=CARTESIAN_POINT('Ctrl Pts',(-22.0544477502527,65.767559331704,25.30841663835));
#16465=CARTESIAN_POINT('Ctrl Pts',(-22.0529265634941,65.9984939060226,25.2959252805377));
#16466=CARTESIAN_POINT('Ctrl Pts',(-22.0514168260403,65.9999504085468,26.0540747194623));
#16467=CARTESIAN_POINT('Ctrl Pts',(-22.0513428091222,66.3458999979507,26.0353896065614));
#16468=CARTESIAN_POINT('Ctrl Pts',(-21.8042540521266,67.3778154892877,25.9796601209967));
#16469=CARTESIAN_POINT('Ctrl Pts',(-20.1701400749251,68.4226485469194,25.8868862627681));
#16470=CARTESIAN_POINT('Ctrl Pts',(-18.0569489447748,67.4569397798106,25.7757531447766));
#16471=CARTESIAN_POINT('Ctrl Pts',(-17.7220731495743,65.1577888564038,25.664620026785));
#16472=CARTESIAN_POINT('Ctrl Pts',(-19.4721283434274,63.6294498117299,25.5534869087935));
#16473=CARTESIAN_POINT('Ctrl Pts',(-21.5520773549122,64.2267966310467,25.4499718063526));
#16474=CARTESIAN_POINT('Ctrl Pts',(-22.0504072989427,65.4596362929778,25.3835010765755));
#16475=CARTESIAN_POINT('Ctrl Pts',(-22.0554079166885,66.0018230931942,25.3540747194623));
#16476=CARTESIAN_POINT('Origin',(-20.,66.,37.5459252805377));
#16477=CARTESIAN_POINT('',(-22.0555312286582,65.9981936687081,26.7540747194623));
#16478=CARTESIAN_POINT('',(-22.0542236518071,66.0018654838724,26.6959252805377));
#16479=CARTESIAN_POINT('',(-22.05475,66.0000000000002,37.5459252805377));
#16480=CARTESIAN_POINT('Ctrl Pts',(-22.0542236518071,66.0018654838723,26.6959252805377));
#16481=CARTESIAN_POINT('Ctrl Pts',(-22.0558087689216,66.1797860011837,26.6862824436496));
#16482=CARTESIAN_POINT('Ctrl Pts',(-21.9531907145538,67.0394144619844,26.6395952340976));
#16483=CARTESIAN_POINT('Ctrl Pts',(-20.7492058435804,68.3101651333771,26.5558636518819));
#16484=CARTESIAN_POINT('Ctrl Pts',(-18.4655076477758,67.8824200236192,26.4447305338902));
#16485=CARTESIAN_POINT('Ctrl Pts',(-17.5862396422193,65.7318111728283,26.3335974158987));
#16486=CARTESIAN_POINT('Ctrl Pts',(-18.9161353509539,63.8266569879394,26.2224642979071));
#16487=CARTESIAN_POINT('Ctrl Pts',(-21.2380361565659,63.9106364641676,26.1113311799156));
#16488=CARTESIAN_POINT('Ctrl Pts',(-22.0457929795606,65.2670452373488,26.0358181741258));
#16489=CARTESIAN_POINT('Ctrl Pts',(-22.0580964866329,65.9733632723993,25.9973495409998));
#16490=CARTESIAN_POINT('Ctrl Pts',(-22.0580137571954,65.9995169080372,25.9959252805377));
#16491=CARTESIAN_POINT('Ctrl Pts',(-22.0555312286582,65.9981936687081,26.7540747194623));
#16492=CARTESIAN_POINT('Ctrl Pts',(-22.0505008107251,66.546259996983,26.7243225092112));
#16493=CARTESIAN_POINT('Ctrl Pts',(-21.5431050900676,67.7849445043772,26.6575259262963));
#16494=CARTESIAN_POINT('Ctrl Pts',(-19.4513023431397,68.3658195746722,26.5536849707175));
#16495=CARTESIAN_POINT('Ctrl Pts',(-17.714794155333,66.8221949683201,26.4425518527259));
#16496=CARTESIAN_POINT('Ctrl Pts',(-18.0697956411282,64.5260652687741,26.3314187347344));
#16497=CARTESIAN_POINT('Ctrl Pts',(-20.1913974446539,63.5789384432151,26.2202856167427));
#16498=CARTESIAN_POINT('Ctrl Pts',(-21.8105644780809,64.6343487755811,26.1278376116522));
#16499=CARTESIAN_POINT('Ctrl Pts',(-22.0514895521636,65.6600338979829,26.0724339792253));
#16500=CARTESIAN_POINT('Ctrl Pts',(-22.0514168260403,65.9999504085468,26.0540747194623));
#16501=CARTESIAN_POINT('Origin',(-20.,66.,37.5459252805377));
#16502=CARTESIAN_POINT('',(-22.0572927264517,66.0011828701741,27.4540747194623));
#16503=CARTESIAN_POINT('',(-22.0516085534354,65.9993486075168,27.3959252805377));
#16504=CARTESIAN_POINT('',(-22.05475,66.0000000000002,37.5459252805377));
#16505=CARTESIAN_POINT('Ctrl Pts',(-22.0516085534354,65.9993486075168,27.3959252805377));
#16506=CARTESIAN_POINT('Ctrl Pts',(-22.0505185253417,66.3826975370093,27.3752153462994));
#16507=CARTESIAN_POINT('Ctrl Pts',(-21.7633388146539,67.4532686773158,27.3174610393972));
#16508=CARTESIAN_POINT('Ctrl Pts',(-20.0378654061023,68.4283198539221,27.2226623598312));
#16509=CARTESIAN_POINT('Ctrl Pts',(-17.980425607167,67.3488848690413,27.1115292418396));
#16510=CARTESIAN_POINT('Ctrl Pts',(-17.7713798203235,65.0348973788296,27.0003961238481));
#16511=CARTESIAN_POINT('Ctrl Pts',(-19.6020548636007,63.6042097568846,26.8892630058565));
#16512=CARTESIAN_POINT('Ctrl Pts',(-21.6064981126984,64.3001233076535,26.787772724753));
#16513=CARTESIAN_POINT('Ctrl Pts',(-22.0497193089643,65.4962782301495,26.7233268163134));
#16514=CARTESIAN_POINT('Ctrl Pts',(-22.0542236518071,66.0018654838723,26.6959252805377));
#16515=CARTESIAN_POINT('Ctrl Pts',(-22.0572927264517,66.0011828701741,27.4540747194623));
#16516=CARTESIAN_POINT('Ctrl Pts',(-22.0577689201907,66.0705663114154,27.4502997845249));
#16517=CARTESIAN_POINT('Ctrl Pts',(-22.0231032579491,66.8203452154228,27.4094804769236));
#16518=CARTESIAN_POINT('Ctrl Pts',(-21.1033853710592,68.1634953045376,27.3316167966584));
#16519=CARTESIAN_POINT('Ctrl Pts',(-18.7808305400592,68.1004278233727,27.2204836786668));
#16520=CARTESIAN_POINT('Ctrl Pts',(-17.5741075901122,66.1149661254002,27.1093505606753));
#16521=CARTESIAN_POINT('Ctrl Pts',(-18.5876568453766,64.0242829060802,26.9982174426837));
#16522=CARTESIAN_POINT('Ctrl Pts',(-20.8938381659967,63.7418537313102,26.8870843246922));
#16523=CARTESIAN_POINT('Ctrl Pts',(-21.9835526554325,65.0484776377887,26.8057034169517));
#16524=CARTESIAN_POINT('Ctrl Pts',(-22.0567641664555,65.8638645333256,26.7613668818751));
#16525=CARTESIAN_POINT('Ctrl Pts',(-22.0555312286582,65.9981936687081,26.7540747194623));
#16526=CARTESIAN_POINT('Origin',(-20.,66.,37.5459252805377));
#16527=CARTESIAN_POINT('',(-22.0519546912208,66.0010551247961,28.1540747194623));
#16528=CARTESIAN_POINT('',(-22.0566098087376,65.9984792507726,28.0959252805377));
#16529=CARTESIAN_POINT('',(-22.05475,66.0000000000002,37.5459252805377));
#16530=CARTESIAN_POINT('Ctrl Pts',(-22.0566098087376,65.9984792507726,28.0959252805377));
#16531=CARTESIAN_POINT('Ctrl Pts',(-22.0517666752291,66.5830501214977,28.0641482489491));
#16532=CARTESIAN_POINT('Ctrl Pts',(-21.4848825436541,67.8572999709014,27.9953268446968));
#16533=CARTESIAN_POINT('Ctrl Pts',(-19.3231871914542,68.3324012329073,27.8894610677805));
#16534=CARTESIAN_POINT('Ctrl Pts',(-17.6733826257443,66.6964356994646,27.778327949789));
#16535=CARTESIAN_POINT('Ctrl Pts',(-18.1529898563275,64.4230648027232,27.6671948317974));
#16536=CARTESIAN_POINT('Ctrl Pts',(-20.3230534668011,63.5929670655095,27.5560617138059));
#16537=CARTESIAN_POINT('Ctrl Pts',(-21.8481481306761,64.7100347411471,27.4656385300526));
#16538=CARTESIAN_POINT('Ctrl Pts',(-22.0524682856091,65.6969918055957,27.4122597189632));
#16539=CARTESIAN_POINT('Ctrl Pts',(-22.0516085534354,65.9993486075168,27.3959252805377));
#16540=CARTESIAN_POINT('Ctrl Pts',(-22.0519546912208,66.0010551247961,28.1540747194623));
#16541=CARTESIAN_POINT('Ctrl Pts',(-22.0532325018955,66.2756710652459,28.1392326871747));
#16542=CARTESIAN_POINT('Ctrl Pts',(-21.8740722112356,67.2341046919512,28.0873462822231));
#16543=CARTESIAN_POINT('Ctrl Pts',(-20.4194990409278,68.3921103158831,27.9984155046077));
#16544=CARTESIAN_POINT('Ctrl Pts',(-18.2178370221936,67.6498685794103,27.8872823866162));
#16545=CARTESIAN_POINT('Ctrl Pts',(-17.647280706083,65.3976021808533,27.7761492686246));
#16546=CARTESIAN_POINT('Ctrl Pts',(-19.2300256897269,63.6966739765529,27.6650161506331));
#16547=CARTESIAN_POINT('Ctrl Pts',(-21.4397818870587,64.0900099051345,27.557657967579));
#16548=CARTESIAN_POINT('Ctrl Pts',(-22.0530959129415,65.3896893965474,27.4873441571887));
#16549=CARTESIAN_POINT('Ctrl Pts',(-22.0572927264517,66.0011828701741,27.4540747194623));
#16550=CARTESIAN_POINT('Origin',(-20.,66.,37.5459252805377));
#16551=CARTESIAN_POINT('',(-22.0534437738779,65.998246286058,28.8540747194623));
#16552=CARTESIAN_POINT('',(-22.0563385464768,66.0016161415221,28.7959252805377));
#16553=CARTESIAN_POINT('',(-22.05475,66.0000000000002,37.5459252805377));
#16554=CARTESIAN_POINT('Ctrl Pts',(-22.0563385464768,66.0016161415221,28.7959252805377));
#16555=CARTESIAN_POINT('Ctrl Pts',(-22.0572596900105,66.1083451864965,28.7901255242628));
#16556=CARTESIAN_POINT('Ctrl Pts',(-22.0011751206758,66.8958067777666,28.747281395324));
#16557=CARTESIAN_POINT('Ctrl Pts',(-20.9838410983712,68.2204116244866,28.6673928937214));
#16558=CARTESIAN_POINT('Ctrl Pts',(-18.6681747980826,68.0308650178038,28.5562597757299));
#16559=CARTESIAN_POINT('Ctrl Pts',(-17.5714473427131,65.9825908127564,28.4451266577384));
#16560=CARTESIAN_POINT('Ctrl Pts',(-18.6974268662034,63.9502501810978,28.3339935397467));
#16561=CARTESIAN_POINT('Ctrl Pts',(-21.015572590504,63.7939212610561,28.2228604217552));
#16562=CARTESIAN_POINT('Ctrl Pts',(-22.007159314054,65.1240507418666,28.1435043353522));
#16563=CARTESIAN_POINT('Ctrl Pts',(-22.0574126035484,65.9015811452894,28.101192621613));
#16564=CARTESIAN_POINT('Ctrl Pts',(-22.0566098087376,65.9984792507726,28.0959252805377));
#16565=CARTESIAN_POINT('Ctrl Pts',(-22.0534437738779,65.998246286058,28.8540747194623));
#16566=CARTESIAN_POINT('Ctrl Pts',(-22.0495560303119,66.4767579293803,28.8281655898244));
#16567=CARTESIAN_POINT('Ctrl Pts',(-21.6444560015232,67.6453699217003,28.7652120875227));
#16568=CARTESIAN_POINT('Ctrl Pts',(-19.6986309163782,68.4098439543111,28.665214212557));
#16569=CARTESIAN_POINT('Ctrl Pts',(-17.8119537217837,67.0538617998004,28.5540810945656));
#16570=CARTESIAN_POINT('Ctrl Pts',(-17.9278626016764,64.733343846516,28.442947976574));
#16571=CARTESIAN_POINT('Ctrl Pts',(-19.9402731870454,63.5721194600009,28.3318148585824));
#16572=CARTESIAN_POINT('Ctrl Pts',(-21.7312864460425,64.4913061059809,28.2355237728785));
#16573=CARTESIAN_POINT('Ctrl Pts',(-22.050043201811,65.590254469979,28.1762770598385));
#16574=CARTESIAN_POINT('Ctrl Pts',(-22.0519546912208,66.0010551247961,28.1540747194623));
#16575=CARTESIAN_POINT('Origin',(-20.,66.,37.5459252805377));
#16576=CARTESIAN_POINT('',(-22.0581541863218,65.9999766228665,29.5540747194623));
#16577=CARTESIAN_POINT('',(-22.051526238456,66.0004971808368,29.4959252805377));
#16578=CARTESIAN_POINT('',(-22.05475,66.0000000000002,37.5459252805377));
#16579=CARTESIAN_POINT('Ctrl Pts',(-22.051526238456,66.0004971808368,29.4959252805377));
#16580=CARTESIAN_POINT('Ctrl Pts',(-22.0522022874077,66.3127404725456,29.4790584269126));
#16581=CARTESIAN_POINT('Ctrl Pts',(-21.8385379867522,67.3098804665473,29.4251472006236));
#16582=CARTESIAN_POINT('Ctrl Pts',(-20.288512196013,68.4114169696994,29.3341916016708));
#16583=CARTESIAN_POINT('Ctrl Pts',(-18.1305721768482,67.5502937473358,29.2230584836793));
#16584=CARTESIAN_POINT('Ctrl Pts',(-17.683606081394,65.270280668443,29.1119253656876));
#16585=CARTESIAN_POINT('Ctrl Pts',(-19.3566948726244,63.6581354432645,29.0007922476961));
#16586=CARTESIAN_POINT('Ctrl Pts',(-21.5005207220627,64.1616337347749,28.8954588859794));
#16587=CARTESIAN_POINT('Ctrl Pts',(-22.0513761351298,65.4266423133588,28.8271698969266));
#16588=CARTESIAN_POINT('Ctrl Pts',(-22.0563385464768,66.0016161415221,28.7959252805377));
#16589=CARTESIAN_POINT('Ctrl Pts',(-22.0581540576791,65.9999766237499,29.5540747194623));
#16590=CARTESIAN_POINT('Ctrl Pts',(-22.0580399009054,66.6788457514294,29.5170984924742));
#16591=CARTESIAN_POINT('Ctrl Pts',(-21.31955436897,68.0380479292517,29.4430778928222));
#16592=CARTESIAN_POINT('Ctrl Pts',(-19.0043305992079,68.2151328748,29.3320129205065));
#16593=CARTESIAN_POINT('Ctrl Pts',(-17.5989621119428,66.3649496798285,29.2208798025149));
#16594=CARTESIAN_POINT('Ctrl Pts',(-18.391118003758,64.1807501735986,29.1097466845233));
#16595=CARTESIAN_POINT('Ctrl Pts',(-20.6557860235121,63.6615997134667,28.9986135665318));
#16596=CARTESIAN_POINT('Ctrl Pts',(-21.9322057363075,64.9047211795848,28.9133895781781));
#16597=CARTESIAN_POINT('Ctrl Pts',(-22.0551146509022,65.792591232661,28.8652099624883));
#16598=CARTESIAN_POINT('Ctrl Pts',(-22.0534437738779,65.998246286058,28.8540747194623));
#16599=CARTESIAN_POINT('Origin',(-20.,66.,37.5459252805377));
#16600=CARTESIAN_POINT('',(-22.0535119255156,66.0017684723631,30.2540747194623));
#16601=CARTESIAN_POINT('',(-22.0545157448452,65.9981221131555,30.1959252805377));
#16602=CARTESIAN_POINT('',(-22.05475,66.0000000000002,37.5459252805377));
#16603=CARTESIAN_POINT('Ctrl Pts',(-22.0545157448452,65.9981221131555,30.1959252805377));
#16604=CARTESIAN_POINT('Ctrl Pts',(-22.0498371642056,66.5133463182488,30.1679913295624));
#16605=CARTESIAN_POINT('Ctrl Pts',(-21.592529418229,67.7192337339074,30.1030130059232));
#16606=CARTESIAN_POINT('Ctrl Pts',(-19.5677489114844,68.3898389245888,30.0009903096202));
#16607=CARTESIAN_POINT('Ctrl Pts',(-17.7577727852529,66.9330531637854,29.8898571916286));
#16608=CARTESIAN_POINT('Ctrl Pts',(-17.9999712591612,64.6223004228711,29.7787240736371));
#16609=CARTESIAN_POINT('Ctrl Pts',(-20.0726747570493,63.5724725606719,29.6675909556455));
#16610=CARTESIAN_POINT('Ctrl Pts',(-21.7743809429352,64.56654600135,29.573324691279));
#16611=CARTESIAN_POINT('Ctrl Pts',(-22.0507174930375,65.626966046743,29.5161027995764));
#16612=CARTESIAN_POINT('Ctrl Pts',(-22.051526238456,66.0004971808368,29.4959252805377));
#16613=CARTESIAN_POINT('Ctrl Pts',(-22.0535119255156,66.0017684723631,30.2540747194623));
#16614=CARTESIAN_POINT('Ctrl Pts',(-22.0551802784048,66.2048893240828,30.2430757677879));
#16615=CARTESIAN_POINT('Ctrl Pts',(-21.9341784793424,67.090175672945,30.1950324434496));
#16616=CARTESIAN_POINT('Ctrl Pts',(-20.6643636219036,68.335977779557,30.1099447464473));
#16617=CARTESIAN_POINT('Ctrl Pts',(-18.3978055525618,67.8251422304279,29.9988116284558));
#16618=CARTESIAN_POINT('Ctrl Pts',(-17.5976389032744,65.643864675113,29.8876785104642));
#16619=CARTESIAN_POINT('Ctrl Pts',(-18.9962076857216,63.7885361864844,29.7765453924727));
#16620=CARTESIAN_POINT('Ctrl Pts',(-21.3134867030769,63.9572264223528,29.6654122744811));
#16621=CARTESIAN_POINT('Ctrl Pts',(-22.0575866779735,65.317354308492,29.5912553834777));
#16622=CARTESIAN_POINT('Ctrl Pts',(-22.0581542680654,65.9987254956813,29.5541428651381));
#16623=CARTESIAN_POINT('Ctrl Pts',(-22.0581540576791,65.9999766237499,29.5540747194623));
#16624=CARTESIAN_POINT('Origin',(-20.,66.,37.5459252805377));
#16625=CARTESIAN_POINT('',(-22.0519162775778,65.9989795847404,30.9540747194623));
#16626=CARTESIAN_POINT('',(-22.0579000785645,66.000654439173,30.8959252805377));
#16627=CARTESIAN_POINT('',(-22.05475,66.0000000000002,37.5459252805377));
#16628=CARTESIAN_POINT('Ctrl Pts',(-22.0579000785645,66.000654439173,30.8959252805377));
#16629=CARTESIAN_POINT('Ctrl Pts',(-22.058049874387,66.0365901201345,30.893968604876));
#16630=CARTESIAN_POINT('Ctrl Pts',(-22.0409121506992,66.7527251194839,30.8549675565505));
#16631=CARTESIAN_POINT('Ctrl Pts',(-21.2079497399452,68.1069002147157,30.778922135561));
#16632=CARTESIAN_POINT('Ctrl Pts',(-18.8850916049024,68.1575797458132,30.6677890175695));
#16633=CARTESIAN_POINT('Ctrl Pts',(-17.5826415154197,66.2335573720312,30.5566558995779));
#16634=CARTESIAN_POINT('Ctrl Pts',(-18.4926530573277,64.0957740986377,30.4455227815864));
#16635=CARTESIAN_POINT('Ctrl Pts',(-20.7822478497669,63.7008133197721,30.3343896635948));
#16636=CARTESIAN_POINT('Ctrl Pts',(-21.960352412273,64.9805048569412,30.2511904965786));
#16637=CARTESIAN_POINT('Ctrl Pts',(-22.0560416243231,65.830086099321,30.2050357022262));
#16638=CARTESIAN_POINT('Ctrl Pts',(-22.0545157448452,65.9981221131555,30.1959252805377));
#16639=CARTESIAN_POINT('Ctrl Pts',(-22.0519162775778,65.9989795847404,30.9540747194623));
#16640=CARTESIAN_POINT('Ctrl Pts',(-22.0500810490173,66.4072776271396,30.9320086704376));
#16641=CARTESIAN_POINT('Ctrl Pts',(-21.7342815225247,67.5036401694582,30.872898248749));
#16642=CARTESIAN_POINT('Ctrl Pts',(-19.9491839999498,68.4280833887723,30.7767434543968));
#16643=CARTESIAN_POINT('Ctrl Pts',(-17.9325252312672,67.2742524433354,30.6656103364051));
#16644=CARTESIAN_POINT('Ctrl Pts',(-17.8081007459427,64.9541755076705,30.5544772184136));
#16645=CARTESIAN_POINT('Ctrl Pts',(-19.6897887302455,63.5912783106364,30.4433441004221));
#16646=CARTESIAN_POINT('Ctrl Pts',(-21.6410622125122,64.3496381393588,30.3432099341049));
#16647=CARTESIAN_POINT('Ctrl Pts',(-22.0495612805229,65.5207800789832,30.2801201404517));
#16648=CARTESIAN_POINT('Ctrl Pts',(-22.0535119255156,66.0017684723631,30.2540747194623));
#16649=CARTESIAN_POINT('Origin',(-20.,66.,37.5459252805377));
#16650=CARTESIAN_POINT('',(-22.057236142177,65.998782267325,31.6540747194623));
#16651=CARTESIAN_POINT('',(-22.0525866339517,66.0014635244036,31.5959252805377));
#16652=CARTESIAN_POINT('',(-22.05475,66.0000000000002,37.5459252805377));
#16653=CARTESIAN_POINT('Ctrl Pts',(-22.0525866339517,66.0014635244036,31.5959252805377));
#16654=CARTESIAN_POINT('Ctrl Pts',(-22.0541717186706,66.2422509029639,31.5829015075258));
#16655=CARTESIAN_POINT('Ctrl Pts',(-21.9036808981398,67.1660076174918,31.5328333618501));
#16656=CARTESIAN_POINT('Ctrl Pts',(-20.5360719551439,68.3687122974119,31.4457208435104));
#16657=CARTESIAN_POINT('Ctrl Pts',(-18.3007213260338,67.7351147158636,31.3345877255189));
#16658=CARTESIAN_POINT('Ctrl Pts',(-17.6206174222944,65.513471852907,31.2234546075273));
#16659=CARTESIAN_POINT('Ctrl Pts',(-19.1182181052569,63.7371186997313,31.1123214895358));
#16660=CARTESIAN_POINT('Ctrl Pts',(-21.3822833862681,64.0266544774867,31.0031450472059));
#16661=CARTESIAN_POINT('Ctrl Pts',(-22.0552138947814,65.3562449901084,30.9310129775399));
#16662=CARTESIAN_POINT('Ctrl Pts',(-22.0579000785645,66.000654439173,30.8959252805377));
#16663=CARTESIAN_POINT('Ctrl Pts',(-22.057236142177,65.998782267325,31.6540747194623));
#16664=CARTESIAN_POINT('Ctrl Pts',(-22.0529596984944,66.6078147591637,31.6209415730874));
#16665=CARTESIAN_POINT('Ctrl Pts',(-21.443978487402,67.9052028120665,31.5507640540487));
#16666=CARTESIAN_POINT('Ctrl Pts',(-19.2384841663151,68.3061363454358,31.4435421623461));
#16667=CARTESIAN_POINT('Ctrl Pts',(-17.6495073727765,66.611028328362,31.3324090443545));
#16668=CARTESIAN_POINT('Ctrl Pts',(-18.2117939461611,64.3566831353306,31.221275926363));
#16669=CARTESIAN_POINT('Ctrl Pts',(-20.4107170831235,63.6063662171661,31.1101428083713));
#16670=CARTESIAN_POINT('Ctrl Pts',(-21.8717660929245,64.7607922201078,31.0210757394046));
#16671=CARTESIAN_POINT('Ctrl Pts',(-22.0531620215394,65.7218289170582,30.9690530431015));
#16672=CARTESIAN_POINT('Ctrl Pts',(-22.0519162775778,65.9989795847404,30.9540747194623));
#16673=CARTESIAN_POINT('Origin',(-20.,66.,37.5459252805377));
#16674=CARTESIAN_POINT('',(-22.0556068717584,66.0017938242738,32.3540747194623));
#16675=CARTESIAN_POINT('',(-22.0526152032265,65.9985230107867,32.2959252805377));
#16676=CARTESIAN_POINT('',(-22.05475,66.0000000000002,37.5459252805377));
#16677=CARTESIAN_POINT('Ctrl Pts',(-22.0526152032265,65.9985230107867,32.2959252805377));
#16678=CARTESIAN_POINT('Ctrl Pts',(-22.0496535487049,66.4439065819169,32.2718344101756));
#16679=CARTESIAN_POINT('Ctrl Pts',(-21.6883554661722,67.5785298398012,32.2106991671496));
#16680=CARTESIAN_POINT('Ctrl Pts',(-19.8169356517564,68.4217057074312,32.1125195514598));
#16681=CARTESIAN_POINT('Ctrl Pts',(-17.866154430883,67.1596871026972,32.0013864334682));
#16682=CARTESIAN_POINT('Ctrl Pts',(-17.8683526622086,64.8362772167352,31.8902533154766));
#16683=CARTESIAN_POINT('Ctrl Pts',(-19.8215184379026,63.5779522256995,31.7791201974851));
#16684=CARTESIAN_POINT('Ctrl Pts',(-21.6900011086861,64.4240617419441,31.6810108525054));
#16685=CARTESIAN_POINT('Ctrl Pts',(-22.0496631581345,65.557363553039,31.6199458801896));
#16686=CARTESIAN_POINT('Ctrl Pts',(-22.0525866339517,66.0014635244036,31.5959252805377));
#16687=CARTESIAN_POINT('Ctrl Pts',(-22.0556068717584,66.0017938242738,32.3540747194623));
#16688=CARTESIAN_POINT('Ctrl Pts',(-22.05681331218,66.1335998378205,32.3469188484011));
#16689=CARTESIAN_POINT('Ctrl Pts',(-21.98521449447,66.9464311753166,32.302718604676));
#16690=CARTESIAN_POINT('Ctrl Pts',(-20.9021196143316,68.2548506403159,32.221473988287));
#16691=CARTESIAN_POINT('Ctrl Pts',(-18.5949173170392,67.9808871403329,32.1103408702954));
#16692=CARTESIAN_POINT('Ctrl Pts',(-17.5737019947084,65.8939377625597,31.9992077523039));
#16693=CARTESIAN_POINT('Ctrl Pts',(-18.7731301049792,63.9040607190605,31.8880746343123));
#16694=CARTESIAN_POINT('Ctrl Pts',(-21.0954378323017,63.8324698008436,31.7769415163208));
#16695=CARTESIAN_POINT('Ctrl Pts',(-22.0216974132697,65.1745805506422,31.6989415447041));
#16696=CARTESIAN_POINT('Ctrl Pts',(-22.0577409580724,65.9268885852111,31.6579859457513));
#16697=CARTESIAN_POINT('Ctrl Pts',(-22.057236142177,65.998782267325,31.6540747194623));
#16698=CARTESIAN_POINT('Origin',(-20.,66.,37.5459252805377));
#16699=CARTESIAN_POINT('',(-22.051418808895,66.0000908847409,33.0540747194623));
#16700=CARTESIAN_POINT('',(-22.0579171903476,65.9993679635754,32.9959252805377));
#16701=CARTESIAN_POINT('',(-22.05475,66.0000000000002,37.5459252805377));
#16702=CARTESIAN_POINT('Ctrl Pts',(-22.0579171903476,65.9993679635754,32.9959252805377));
#16703=CARTESIAN_POINT('Ctrl Pts',(-22.055307325611,66.6450536664726,32.9607673128253));
#16704=CARTESIAN_POINT('Ctrl Pts',(-21.3800044610758,67.9757740072377,32.8885649724492));
#16705=CARTESIAN_POINT('Ctrl Pts',(-19.1139377600523,68.2612087024321,32.7793182594091));
#16706=CARTESIAN_POINT('Ctrl Pts',(-17.6197010520624,66.4820249033491,32.6681851414176));
#16707=CARTESIAN_POINT('Ctrl Pts',(-18.304007628879,64.2616729404111,32.557052023426));
#16708=CARTESIAN_POINT('Ctrl Pts',(-20.5405531773546,63.6323063222924,32.4459189054345));
#16709=CARTESIAN_POINT('Ctrl Pts',(-21.9047824951618,64.8366244321949,32.358876657805));
#16710=CARTESIAN_POINT('Ctrl Pts',(-22.0542076653537,65.7590431984314,32.3088787828394));
#16711=CARTESIAN_POINT('Ctrl Pts',(-22.0526152032265,65.9985230107867,32.2959252805377));
#16712=CARTESIAN_POINT('Ctrl Pts',(-22.051418808895,66.0000908847409,33.0540747194623));
#16713=CARTESIAN_POINT('Ctrl Pts',(-22.0515519357582,66.3374829967905,33.0358517510508));
#16714=CARTESIAN_POINT('Ctrl Pts',(-21.813184036767,67.3605620427844,32.9805844099755));
#16715=CARTESIAN_POINT('Ctrl Pts',(-20.2002808069203,68.4203427044879,32.8882726962364));
#16716=CARTESIAN_POINT('Ctrl Pts',(-18.0752184027424,67.4810087817272,32.7771395782448));
#16717=CARTESIAN_POINT('Ctrl Pts',(-17.7117918750668,65.1861973300252,32.6660064602532));
#16718=CARTESIAN_POINT('Ctrl Pts',(-19.4426234863108,63.6362101128286,32.5548733422617));
#16719=CARTESIAN_POINT('Ctrl Pts',(-21.5392921211705,64.2101565763925,32.4508960953313));
#16720=CARTESIAN_POINT('Ctrl Pts',(-22.0505678351178,65.4512690574914,32.3839632210649));
#16721=CARTESIAN_POINT('Ctrl Pts',(-22.0556068717584,66.0017938242738,32.3540747194623));
#16722=CARTESIAN_POINT('Origin',(-20.,66.,37.5459252805377));
#16723=CARTESIAN_POINT('',(-22.0552733065389,65.9981586635305,33.7540747194623));
#16724=CARTESIAN_POINT('',(-22.0544769197952,66.0018771064673,33.6959252805377));
#16725=CARTESIAN_POINT('',(-22.05475,66.0000000000002,37.5459252805377));
#16726=CARTESIAN_POINT('Ctrl Pts',(-22.0544769197952,66.0018771064673,33.6959252805377));
#16727=CARTESIAN_POINT('Ctrl Pts',(-22.0560114007709,66.1712173828127,33.686744588139));
#16728=CARTESIAN_POINT('Ctrl Pts',(-21.9594168493607,67.0221238303151,33.6405195230764));
#16729=CARTESIAN_POINT('Ctrl Pts',(-20.7778958267891,68.3006627675311,33.5572500853501));
#16730=CARTESIAN_POINT('Ctrl Pts',(-18.4890524956552,67.9013702240204,33.4461169673585));
#16731=CARTESIAN_POINT('Ctrl Pts',(-17.5830877907652,65.7618688136113,33.334983849367));
#16732=CARTESIAN_POINT('Ctrl Pts',(-18.8891762685279,63.8403144380744,33.2238507313753));
#16733=CARTESIAN_POINT('Ctrl Pts',(-21.2119343469181,63.8953892930382,33.1127176133839));
#16734=CARTESIAN_POINT('Ctrl Pts',(-22.0415654965746,65.2498853356985,33.0367424631046));
#16735=CARTESIAN_POINT('Ctrl Pts',(-22.0580572229514,65.9647236201639,32.9978116854892));
#16736=CARTESIAN_POINT('Ctrl Pts',(-22.0579171903476,65.9993679635754,32.9959252805377));
#16737=CARTESIAN_POINT('Ctrl Pts',(-22.0552733065389,65.9981586635305,33.7540747194623));
#16738=CARTESIAN_POINT('Ctrl Pts',(-22.0502920219753,66.5378859763281,33.7247846537006));
#16739=CARTESIAN_POINT('Ctrl Pts',(-21.5559212245969,67.7683043054681,33.6584502152751));
#16740=CARTESIAN_POINT('Ctrl Pts',(-19.4807858366348,68.3724645130774,33.5550714041857));
#16741=CARTESIAN_POINT('Ctrl Pts',(-17.7252025426939,66.8505690671885,33.4439382861941));
#16742=CARTESIAN_POINT('Ctrl Pts',(-18.0516034185067,64.550199335027,33.3328051682026));
#16743=CARTESIAN_POINT('Ctrl Pts',(-20.1612535330058,63.5767442339982,33.221672050211));
#16744=CARTESIAN_POINT('Ctrl Pts',(-21.8015900293923,64.6170979978703,33.1287619006309));
#16745=CARTESIAN_POINT('Ctrl Pts',(-22.0512813101927,65.651618934998,33.0728961237147));
#16746=CARTESIAN_POINT('Ctrl Pts',(-22.051418808895,66.0000908847409,33.0540747194623));
#16747=CARTESIAN_POINT('Origin',(-20.,66.,37.5459252805377));
#16748=CARTESIAN_POINT('',(-22.0574743337809,66.0010592828478,34.4540747194623));
#16749=CARTESIAN_POINT('',(-22.0515358230213,65.9994822145391,34.3959252805377));
#16750=CARTESIAN_POINT('',(-22.05475,66.0000000000002,37.5459252805377));
#16751=CARTESIAN_POINT('Ctrl Pts',(-22.0515358230213,65.9994822145391,34.3959252805377));
#16752=CARTESIAN_POINT('Ctrl Pts',(-22.0506904409372,66.3743098554946,34.3756774907888));
#16753=CARTESIAN_POINT('Ctrl Pts',(-21.7729352593099,67.4360704009606,34.318385328376));
#16754=CARTESIAN_POINT('Ctrl Pts',(-20.0680811507602,68.427660588213,34.2240487932995));
#16755=CARTESIAN_POINT('Ctrl Pts',(-17.9973678966875,67.3739125797871,34.1129156753078));
#16756=CARTESIAN_POINT('Ctrl Pts',(-17.7595423634621,65.0627056594589,34.0017825573163));
#16757=CARTESIAN_POINT('Ctrl Pts',(-19.572271844222,63.6093474323109,33.8906494393247));
#16758=CARTESIAN_POINT('Ctrl Pts',(-21.5943860347699,64.2833182629478,33.7886970137319));
#16759=CARTESIAN_POINT('Ctrl Pts',(-22.0498197234289,65.4879242245718,33.7237889608028));
#16760=CARTESIAN_POINT('Ctrl Pts',(-22.0544769197952,66.0018771064673,33.6959252805377));
#16761=CARTESIAN_POINT('Ctrl Pts',(-22.0574743337809,66.0010592828478,34.4540747194623));
#16762=CARTESIAN_POINT('Ctrl Pts',(-22.0578567313271,66.0619343402333,34.4507619290143));
#16763=CARTESIAN_POINT('Ctrl Pts',(-22.0277961568906,66.8031451110045,34.4104047659024));
#16764=CARTESIAN_POINT('Ctrl Pts',(-21.1302229490745,68.1495968002898,34.3330032301266));
#16765=CARTESIAN_POINT('Ctrl Pts',(-18.8070633085623,68.1154369356633,34.2218701121351));
#16766=CARTESIAN_POINT('Ctrl Pts',(-17.5757260722497,66.1451456629571,34.1107369941435));
#16767=CARTESIAN_POINT('Ctrl Pts',(-18.5631798581025,64.0420114979335,33.999603876152));
#16768=CARTESIAN_POINT('Ctrl Pts',(-20.8656679378464,63.730905409822,33.8884707581604));
#16769=CARTESIAN_POINT('Ctrl Pts',(-21.9778381799678,65.0312098882729,33.8066277059305));
#16770=CARTESIAN_POINT('Ctrl Pts',(-22.0565920611496,65.8552702432393,33.7618290263645));
#16771=CARTESIAN_POINT('Ctrl Pts',(-22.0552733065389,65.9981586635305,33.7540747194623));
#16772=CARTESIAN_POINT('Origin',(-20.,66.,37.5459252805377));
#16773=CARTESIAN_POINT('',(-22.0520910576133,66.0011644713934,35.1540747194623));
#16774=CARTESIAN_POINT('',(-22.0563748666992,65.9983937868295,35.0959252805377));
#16775=CARTESIAN_POINT('',(-22.05475,66.0000000000002,37.5459252805377));
#16776=CARTESIAN_POINT('Ctrl Pts',(-22.0563748666992,65.9983937868295,35.0959252805377));
#16777=CARTESIAN_POINT('Ctrl Pts',(-22.0514251053644,66.5746340067409,35.0646103934386));
#16778=CARTESIAN_POINT('Ctrl Pts',(-21.4984704235166,67.840871850344,34.9962511336756));
#16779=CARTESIAN_POINT('Ctrl Pts',(-19.3522645421998,68.3406415976227,34.8908475012488));
#16780=CARTESIAN_POINT('Ctrl Pts',(-17.6822294728015,66.7253355827527,34.7797143832572));
#16781=CARTESIAN_POINT('Ctrl Pts',(-18.1335090320871,64.4461712429531,34.6685812652656));
#16782=CARTESIAN_POINT('Ctrl Pts',(-20.2930746820505,63.5891334692323,34.5574481472741));
#16783=CARTESIAN_POINT('Ctrl Pts',(-21.8398173954859,64.6927475063844,34.4665628190315));
#16784=CARTESIAN_POINT('Ctrl Pts',(-22.0522371109369,65.6885434094548,34.4127218634526));
#16785=CARTESIAN_POINT('Ctrl Pts',(-22.0515358230213,65.9994822145391,34.3959252805377));
#16786=CARTESIAN_POINT('Ctrl Pts',(-22.0520910576133,66.0011644713934,35.1540747194623));
#16787=CARTESIAN_POINT('Ctrl Pts',(-22.0534710502056,66.2671875919197,35.1396948316641));
#16788=CARTESIAN_POINT('Ctrl Pts',(-21.8818112896055,67.2168117035418,35.088270571202));
#16789=CARTESIAN_POINT('Ctrl Pts',(-20.4492273182073,68.3866955695652,34.999801938076));
#16790=CARTESIAN_POINT('Ctrl Pts',(-18.2385101136685,67.6719231463612,34.8886688200844));
#16791=CARTESIAN_POINT('Ctrl Pts',(-17.6399646371577,65.4269244123525,34.7775357020929));
#16792=CARTESIAN_POINT('Ctrl Pts',(-19.2014230092252,63.706435258535,34.6664025841013));
#16793=CARTESIAN_POINT('Ctrl Pts',(-21.4254341990431,64.0738149167194,34.5585822565578));
#16794=CARTESIAN_POINT('Ctrl Pts',(-22.053580675407,65.3812156690452,34.4878063016781));
#16795=CARTESIAN_POINT('Ctrl Pts',(-22.0574743337809,66.0010592828478,34.4540747194623));
#16796=CARTESIAN_POINT('Origin',(-20.,66.,37.5459252805377));
#16797=CARTESIAN_POINT('',(-22.0526727182563,65.9976789726186,35.8540747194623));
#16798=CARTESIAN_POINT('',(-22.0565719673595,66.0014962574405,35.7959252805377));
#16799=CARTESIAN_POINT('',(-22.05475,66.0000000000002,37.5459252805377));
#16800=CARTESIAN_POINT('',(-20.5301702171886,64.0148256743283,36.));
#16801=CARTESIAN_POINT('Ctrl Pts',(-20.5301702171886,64.0148256743283,36.));
#16802=CARTESIAN_POINT('Ctrl Pts',(-21.1902595624181,64.1911123142463,35.9629556273362));
#16803=CARTESIAN_POINT('Ctrl Pts',(-21.9249295035175,64.8872096289435,35.9143138671569));
#16804=CARTESIAN_POINT('Ctrl Pts',(-22.0542897965232,65.7834100791695,35.8656721069777));
#16805=CARTESIAN_POINT('Ctrl Pts',(-22.0526727182563,65.9976789726186,35.8540747194623));
#16806=CARTESIAN_POINT('',(-19.4686891477661,64.0112682321016,36.));
#16807=CARTESIAN_POINT('Origin',(-20.,66.,36.));
#16808=CARTESIAN_POINT('Ctrl Pts',(-19.4686884555735,64.0112660732732,36.));
#16809=CARTESIAN_POINT('Ctrl Pts',(-20.1132090364839,63.839970256324,35.9636818543909));
#16810=CARTESIAN_POINT('Ctrl Pts',(-21.4929688632731,64.1592659283774,35.8956569479034));
#16811=CARTESIAN_POINT('Ctrl Pts',(-22.0517190735163,65.4183241148264,35.8276320414161));
#16812=CARTESIAN_POINT('Ctrl Pts',(-22.0565719673595,66.0014962574405,35.7959252805377));
#16813=CARTESIAN_POINT('Origin',(20.,66.,30.));
#16814=CARTESIAN_POINT('',(18.3313535993656,65.999608307577,25.7714803633902));
#16815=CARTESIAN_POINT('',(18.3334665914316,66.0014781595158,25.5785196366098));
#16816=CARTESIAN_POINT('',(18.334,66.,30.));
#16817=CARTESIAN_POINT('',(19.2300979593296,64.5225674811446,25.));
#16818=CARTESIAN_POINT('Ctrl Pts',(18.3334665914316,66.0014781595158,25.5785196366098));
#16819=CARTESIAN_POINT('Ctrl Pts',(18.3324169395493,66.1152855036548,25.5709016210591));
#16820=CARTESIAN_POINT('Ctrl Pts',(18.3430836336298,66.2288979300146,25.5632836055085));
#16821=CARTESIAN_POINT('Ctrl Pts',(18.3661914310208,66.3399235223684,25.5556655899578));
#16822=CARTESIAN_POINT('Ctrl Pts',(18.4785584710069,66.8798112911743,25.518621217294));
#16823=CARTESIAN_POINT('Ctrl Pts',(18.8851099357623,67.3585303472824,25.4815768446301));
#16824=CARTESIAN_POINT('Ctrl Pts',(19.3995345876311,67.5569678802536,25.4445324719663));
#16825=CARTESIAN_POINT('Ctrl Pts',(19.9139592394999,67.7554054132248,25.4074880993024));
#16826=CARTESIAN_POINT('Ctrl Pts',(20.536257078482,67.6735614230591,25.3704437266385));
#16827=CARTESIAN_POINT('Ctrl Pts',(20.9821828433076,67.3489732333682,25.3333993539747));
#16828=CARTESIAN_POINT('Ctrl Pts',(21.4281086081331,67.0243850436773,25.2963549813108));
#16829=CARTESIAN_POINT('Ctrl Pts',(21.697662298802,66.4570526544611,25.259310608647));
#16830=CARTESIAN_POINT('Ctrl Pts',(21.6664135722727,65.9064187957527,25.2222662359831));
#16831=CARTESIAN_POINT('Ctrl Pts',(21.6351648457434,65.3557849370443,25.1852218633193));
#16832=CARTESIAN_POINT('Ctrl Pts',(21.3031137020159,64.8218496088437,25.1481774906554));
#16833=CARTESIAN_POINT('Ctrl Pts',(20.8246620716843,64.5495453070113,25.1111331179916));
#16834=CARTESIAN_POINT('Ctrl Pts',(20.3462104413528,64.2772410051789,25.0740887453277));
#16835=CARTESIAN_POINT('Ctrl Pts',(19.7213583244172,64.2665677297147,25.0370443726639));
#16836=CARTESIAN_POINT('Ctrl Pts',(19.2300979593296,64.5225674811445,25.));
#16837=CARTESIAN_POINT('',(18.6629739994073,66.9990030778758,25.));
#16838=CARTESIAN_POINT('Origin',(20.,66.,25.));
#16839=CARTESIAN_POINT('',(18.3354783565503,65.9987788995443,25.0714803633902));
#16840=CARTESIAN_POINT('Ctrl Pts',(18.6629725798064,66.9990042518227,25.));
#16841=CARTESIAN_POINT('Ctrl Pts',(18.4510073780992,66.7145501177189,25.0238267877967));
#16842=CARTESIAN_POINT('Ctrl Pts',(18.3378311247794,66.3559373297411,25.0476535755935));
#16843=CARTESIAN_POINT('Ctrl Pts',(18.3354783565503,65.9987788995443,25.0714803633902));
#16844=CARTESIAN_POINT('',(18.334,66.,24.));
#16845=CARTESIAN_POINT('',(18.334,66.,30.));
#16846=CARTESIAN_POINT('Origin',(20.,66.,24.));
#16847=CARTESIAN_POINT('Ctrl Pts',(18.3354783565503,65.9987788995443,25.0714803633902));
#16848=CARTESIAN_POINT('Ctrl Pts',(18.3342449015815,65.8115361295435,25.0839717212025));
#16849=CARTESIAN_POINT('Ctrl Pts',(18.3634707598459,65.6246930829332,25.0964630790149));
#16850=CARTESIAN_POINT('Ctrl Pts',(18.4248899822037,65.4491448037961,25.1089544368272));
#16851=CARTESIAN_POINT('Ctrl Pts',(18.6070348375451,64.9285387999851,25.1459988094911));
#16852=CARTESIAN_POINT('Ctrl Pts',(19.0723133853053,64.5072678395834,25.1830431821549));
#16853=CARTESIAN_POINT('Ctrl Pts',(19.6082885066022,64.3778809436282,25.2200875548188));
#16854=CARTESIAN_POINT('Ctrl Pts',(20.144263627899,64.2484940476731,25.2571319274826));
#16855=CARTESIAN_POINT('Ctrl Pts',(20.7509353227326,64.4109912161645,25.2941763001465));
#16856=CARTESIAN_POINT('Ctrl Pts',(21.1504371661837,64.7911273133782,25.3312206728103));
#16857=CARTESIAN_POINT('Ctrl Pts',(21.5499390096347,65.1712634105918,25.3682650454742));
#16858=CARTESIAN_POINT('Ctrl Pts',(21.7422710017031,65.7690384365276,25.405309418138));
#16859=CARTESIAN_POINT('Ctrl Pts',(21.6395392863716,66.3108402179399,25.4423537908019));
#16860=CARTESIAN_POINT('Ctrl Pts',(21.5368075710401,66.8526419993522,25.4793981634657));
#16861=CARTESIAN_POINT('Ctrl Pts',(21.1390121483087,67.338470536241,25.5164425361296));
#16862=CARTESIAN_POINT('Ctrl Pts',(20.6281313316149,67.5460304956708,25.5534869087934));
#16863=CARTESIAN_POINT('Ctrl Pts',(20.1172505149211,67.7535904551005,25.5905312814573));
#16864=CARTESIAN_POINT('Ctrl Pts',(19.4932843042648,67.6828818370712,25.6275756541211));
#16865=CARTESIAN_POINT('Ctrl Pts',(19.0418023582524,67.3662475693096,25.664620026785));
#16866=CARTESIAN_POINT('Ctrl Pts',(18.6076787271156,67.0617870714379,25.7002401389867));
#16867=CARTESIAN_POINT('Ctrl Pts',(18.3330311784649,66.5299478078385,25.7358602511885));
#16868=CARTESIAN_POINT('Ctrl Pts',(18.3313535993656,65.999608307577,25.7714803633902));
#16869=CARTESIAN_POINT('Origin',(20.,66.,30.));
#16870=CARTESIAN_POINT('',(18.3344266367885,66.0015125423676,26.4714803633902));
#16871=CARTESIAN_POINT('',(18.336702599684,65.9999597908982,26.2785196366098));
#16872=CARTESIAN_POINT('',(18.334,66.,30.));
#16873=CARTESIAN_POINT('Ctrl Pts',(18.336702599684,65.9999597908982,26.2785196366098));
#16874=CARTESIAN_POINT('Ctrl Pts',(18.3367626127225,66.2804571745203,26.2598345237089));
#16875=CARTESIAN_POINT('Ctrl Pts',(18.403933281346,66.5609816891737,26.241149410808));
#16876=CARTESIAN_POINT('Ctrl Pts',(18.538053161419,66.8046575644459,26.2224642979072));
#16877=CARTESIAN_POINT('Ctrl Pts',(18.8039539801836,67.2877598063567,26.1854199252433));
#16878=CARTESIAN_POINT('Ctrl Pts',(19.3330018469889,67.6260267250789,26.1483755525794));
#16879=CARTESIAN_POINT('Ctrl Pts',(19.8830898233452,67.6646600613318,26.1113311799156));
#16880=CARTESIAN_POINT('Ctrl Pts',(20.4331777997015,67.7032933975846,26.0742868072517));
#16881=CARTESIAN_POINT('Ctrl Pts',(21.004305885609,67.4422931513682,26.0372424345879));
#16882=CARTESIAN_POINT('Ctrl Pts',(21.3351230484566,67.0010994880608,26.000198061924));
#16883=CARTESIAN_POINT('Ctrl Pts',(21.6659402113041,66.5599058247535,25.9631536892602));
#16884=CARTESIAN_POINT('Ctrl Pts',(21.7564464510919,65.9385187443552,25.9261093165963));
#16885=CARTESIAN_POINT('Ctrl Pts',(21.5652075467208,65.4212945794869,25.8890649439325));
#16886=CARTESIAN_POINT('Ctrl Pts',(21.3739686423498,64.9040704146186,25.8520205712686));
#16887=CARTESIAN_POINT('Ctrl Pts',(20.9009845938199,64.4910091652803,25.8149761986048));
#16888=CARTESIAN_POINT('Ctrl Pts',(20.3627356721069,64.3711410197133,25.7779318259409));
#16889=CARTESIAN_POINT('Ctrl Pts',(19.8244867503938,64.2512728741463,25.7408874532771));
#16890=CARTESIAN_POINT('Ctrl Pts',(19.2209729554976,64.4245978323507,25.7038430806132));
#16891=CARTESIAN_POINT('Ctrl Pts',(18.8283073656578,64.8117885522048,25.6667987079493));
#16892=CARTESIAN_POINT('Ctrl Pts',(18.5163917617,65.1193551695888,25.6373723508362));
#16893=CARTESIAN_POINT('Ctrl Pts',(18.3375211159894,65.5618708197218,25.607945993723));
#16894=CARTESIAN_POINT('Ctrl Pts',(18.3334665914316,66.0014781595158,25.5785196366098));
#16895=CARTESIAN_POINT('Ctrl Pts',(18.3313535993656,65.999608307577,25.7714803633902));
#16896=CARTESIAN_POINT('Ctrl Pts',(18.3312865218232,65.9784028274413,25.7729046238523));
#16897=CARTESIAN_POINT('Ctrl Pts',(18.3316558627703,65.9571997450949,25.7743288843144));
#16898=CARTESIAN_POINT('Ctrl Pts',(18.3324688774983,65.9360136919907,25.7757531447766));
#16899=CARTESIAN_POINT('Ctrl Pts',(18.3536150241253,65.3849739999272,25.8127975174404));
#16900=CARTESIAN_POINT('Ctrl Pts',(18.6749049987477,64.8454545332941,25.8498418901043));
#16901=CARTESIAN_POINT('Ctrl Pts',(19.1493178421315,64.5643463136364,25.8868862627681));
#16902=CARTESIAN_POINT('Ctrl Pts',(19.6237306855153,64.2832380939788,25.923930635432));
#16903=CARTESIAN_POINT('Ctrl Pts',(20.2512663976604,64.2605411212966,25.9609750080958));
#16904=CARTESIAN_POINT('Ctrl Pts',(20.7447484473589,64.5066438345424,25.9980193807597));
#16905=CARTESIAN_POINT('Ctrl Pts',(21.2382304970574,64.7527465477881,26.0350637534235));
#16906=CARTESIAN_POINT('Ctrl Pts',(21.5976588843092,65.2676489469618,26.0721081260874));
#16907=CARTESIAN_POINT('Ctrl Pts',(21.658554031172,65.8157206294381,26.1091524987512));
#16908=CARTESIAN_POINT('Ctrl Pts',(21.7194491780347,66.3637923119144,26.1461968714151));
#16909=CARTESIAN_POINT('Ctrl Pts',(21.4818110845084,66.9450332776934,26.1832412440789));
#16910=CARTESIAN_POINT('Ctrl Pts',(21.0543866531954,67.2934566893157,26.2202856167428));
#16911=CARTESIAN_POINT('Ctrl Pts',(20.6269622218823,67.641880100938,26.2573299894066));
#16912=CARTESIAN_POINT('Ctrl Pts',(20.0097514527824,67.7574859584036,26.2943743620705));
#16913=CARTESIAN_POINT('Ctrl Pts',(19.4852026247108,67.587370511937,26.3314187347344));
#16914=CARTESIAN_POINT('Ctrl Pts',(18.9606537966392,67.4172550654703,26.3684631073982));
#16915=CARTESIAN_POINT('Ctrl Pts',(18.5287669095959,66.9614183150713,26.4055074800621));
#16916=CARTESIAN_POINT('Ctrl Pts',(18.3871816596723,66.4284602460038,26.4425518527259));
#16917=CARTESIAN_POINT('Ctrl Pts',(18.3503263056037,66.2897285748037,26.452194689614));
#16918=CARTESIAN_POINT('Ctrl Pts',(18.3331414170134,66.145771262262,26.4618375265021));
#16919=CARTESIAN_POINT('Ctrl Pts',(18.3344266367885,66.0015125423676,26.4714803633902));
#16920=CARTESIAN_POINT('Origin',(20.,66.,30.));
#16921=CARTESIAN_POINT('',(18.3365469699001,65.9994718481762,27.1714803633902));
#16922=CARTESIAN_POINT('',(18.3333666250123,65.9985354189832,26.9785196366098));
#16923=CARTESIAN_POINT('',(18.334,66.,30.));
#16924=CARTESIAN_POINT('Ctrl Pts',(18.3333666250123,65.9985354189832,26.9785196366098));
#16925=CARTESIAN_POINT('Ctrl Pts',(18.3374453090457,66.4429099055735,26.9487674263587));
#16926=CARTESIAN_POINT('Ctrl Pts',(18.5206884737916,66.8902539804794,26.9190152161076));
#16927=CARTESIAN_POINT('Ctrl Pts',(18.8387597051665,67.1984497345904,26.8892630058565));
#16928=CARTESIAN_POINT('Ctrl Pts',(19.2347890801025,67.5821831874113,26.8522186331926));
#16929=CARTESIAN_POINT('Ctrl Pts',(19.8398377253218,67.7501998299206,26.8151742605288));
#16930=CARTESIAN_POINT('Ctrl Pts',(20.3770234062671,67.6256119294545,26.778129887865));
#16931=CARTESIAN_POINT('Ctrl Pts',(20.9142090872123,67.5010240289883,26.7410855152011));
#16932=CARTESIAN_POINT('Ctrl Pts',(21.3835318038834,67.0838315855467,26.7040411425372));
#16933=CARTESIAN_POINT('Ctrl Pts',(21.5702203790488,66.5649500924812,26.6669967698734));
#16934=CARTESIAN_POINT('Ctrl Pts',(21.7569089542143,66.0460685994156,26.6299523972095));
#16935=CARTESIAN_POINT('Ctrl Pts',(21.6609633878742,65.425498056726,26.5929080245457));
#16936=CARTESIAN_POINT('Ctrl Pts',(21.3262899920358,64.9872237156599,26.5558636518818));
#16937=CARTESIAN_POINT('Ctrl Pts',(20.9916165961973,64.5489493745937,26.518819279218));
#16938=CARTESIAN_POINT('Ctrl Pts',(20.4182153708605,64.292971235151,26.4817749065541));
#16939=CARTESIAN_POINT('Ctrl Pts',(19.8684865341392,64.3364300148676,26.4447305338903));
#16940=CARTESIAN_POINT('Ctrl Pts',(19.3187576974179,64.3798887945842,26.4076861612264));
#16941=CARTESIAN_POINT('Ctrl Pts',(18.792701249312,64.7227844934602,26.3706417885625));
#16942=CARTESIAN_POINT('Ctrl Pts',(18.5310499106212,65.2082011254479,26.3335974158987));
#16943=CARTESIAN_POINT('Ctrl Pts',(18.4013750221315,65.4487745080989,26.3152381561357));
#16944=CARTESIAN_POINT('Ctrl Pts',(18.336643633224,65.7243540530003,26.2968788963728));
#16945=CARTESIAN_POINT('Ctrl Pts',(18.336702599684,65.9999597908982,26.2785196366098));
#16946=CARTESIAN_POINT('Ctrl Pts',(18.3344266367885,66.0015125423676,26.4714803633902));
#16947=CARTESIAN_POINT('Ctrl Pts',(18.3380787773415,65.5915802247284,26.498881899166));
#16948=CARTESIAN_POINT('Ctrl Pts',(18.4908762313393,65.1792140559604,26.5262834349417));
#16949=CARTESIAN_POINT('Ctrl Pts',(18.7652753975701,64.8774063579416,26.5536849707175));
#16950=CARTESIAN_POINT('Ctrl Pts',(19.1362379981954,64.4693899266831,26.5907293433813));
#16951=CARTESIAN_POINT('Ctrl Pts',(19.72944681225,64.263436451902,26.6277737160452));
#16952=CARTESIAN_POINT('Ctrl Pts',(20.2734377511034,64.3537943263354,26.664818088709));
#16953=CARTESIAN_POINT('Ctrl Pts',(20.8174286899568,64.4441522007688,26.7018624613729));
#16954=CARTESIAN_POINT('Ctrl Pts',(21.3122017536091,64.8308214244166,26.7389068340368));
#16955=CARTESIAN_POINT('Ctrl Pts',(21.5313390817275,65.336854536141,26.7759512067006));
#16956=CARTESIAN_POINT('Ctrl Pts',(21.7504764098458,65.8428876478653,26.8129955793644));
#16957=CARTESIAN_POINT('Ctrl Pts',(21.6939780024301,66.4682846476661,26.8500399520283));
#16958=CARTESIAN_POINT('Ctrl Pts',(21.387698627229,66.9268515681741,26.8870843246921));
#16959=CARTESIAN_POINT('Ctrl Pts',(21.0814192520278,67.3854184886821,26.924128697356));
#16960=CARTESIAN_POINT('Ctrl Pts',(20.5253589090411,67.6771553298973,26.9611730700199));
#16961=CARTESIAN_POINT('Ctrl Pts',(19.973981762085,67.668557568227,26.9982174426837));
#16962=CARTESIAN_POINT('Ctrl Pts',(19.4226046151289,67.6599598065567,27.0352618153476));
#16963=CARTESIAN_POINT('Ctrl Pts',(18.8759106642033,67.3510274420009,27.0723061880114));
#16964=CARTESIAN_POINT('Ctrl Pts',(18.5840778162202,66.8831340061794,27.1093505606753));
#16965=CARTESIAN_POINT('Ctrl Pts',(18.4209264748504,66.6215546733526,27.1300604949136));
#16966=CARTESIAN_POINT('Ctrl Pts',(18.3374307693608,66.310292807312,27.1507704291519));
#16967=CARTESIAN_POINT('Ctrl Pts',(18.3365469699001,65.9994718481762,27.1714803633902));
#16968=CARTESIAN_POINT('Origin',(20.,66.,30.));
#16969=CARTESIAN_POINT('',(18.3324919306138,65.9987669699924,27.8714803633902));
#16970=CARTESIAN_POINT('',(18.3319383951835,66.0009590761175,27.6785196366098));
#16971=CARTESIAN_POINT('',(18.334,66.,30.));
#16972=CARTESIAN_POINT('Ctrl Pts',(18.3319383951835,66.0009590761175,27.6785196366098));
#16973=CARTESIAN_POINT('Ctrl Pts',(18.3315522952949,66.0572154624142,27.6747447016723));
#16974=CARTESIAN_POINT('Ctrl Pts',(18.3341516128123,66.1134357482357,27.6709697667349));
#16975=CARTESIAN_POINT('Ctrl Pts',(18.3398539528156,66.1693395171271,27.6671948317974));
#16976=CARTESIAN_POINT('Ctrl Pts',(18.3958124293553,66.7179370644852,27.6301504591336));
#16977=CARTESIAN_POINT('Ctrl Pts',(18.7505914623534,67.2360540833893,27.5931060864697));
#16978=CARTESIAN_POINT('Ctrl Pts',(19.2418371848642,67.4865900296292,27.5560617138059));
#16979=CARTESIAN_POINT('Ctrl Pts',(19.733082907375,67.7371259758691,27.519017341142));
#16980=CARTESIAN_POINT('Ctrl Pts',(20.3607953193985,67.7200808494449,27.4819729684782));
#16981=CARTESIAN_POINT('Ctrl Pts',(20.8377208668613,67.4432548354856,27.4449285958143));
#16982=CARTESIAN_POINT('Ctrl Pts',(21.3146464143242,67.1664288215262,27.4078842231505));
#16983=CARTESIAN_POINT('Ctrl Pts',(21.6407850972264,66.6298219200317,27.3708398504866));
#16984=CARTESIAN_POINT('Ctrl Pts',(21.6668894380612,66.0789960097809,27.3337954778227));
#16985=CARTESIAN_POINT('Ctrl Pts',(21.692993778896,65.52817009953,27.2967511051589));
#16986=CARTESIAN_POINT('Ctrl Pts',(21.4190637776633,64.9631251805227,27.259706732495));
#16987=CARTESIAN_POINT('Ctrl Pts',(20.970455189559,64.6424369270067,27.2226623598312));
#16988=CARTESIAN_POINT('Ctrl Pts',(20.5218466014546,64.3217486734907,27.1856179871673));
#16989=CARTESIAN_POINT('Ctrl Pts',(19.8985594264786,64.2454170854659,27.1485736145035));
#16990=CARTESIAN_POINT('Ctrl Pts',(19.3858221505611,64.4483730011308,27.1115292418396));
#16991=CARTESIAN_POINT('Ctrl Pts',(18.8730848746436,64.6513289167956,27.0744848691758));
#16992=CARTESIAN_POINT('Ctrl Pts',(18.4708974977846,65.1335723361501,27.0374404965119));
#16993=CARTESIAN_POINT('Ctrl Pts',(18.3633088616814,65.6744191773935,27.0003961238481));
#16994=CARTESIAN_POINT('Ctrl Pts',(18.3421301035647,65.7808845518395,26.9931039614353));
#16995=CARTESIAN_POINT('Ctrl Pts',(18.3323669538567,65.8896207904243,26.9858117990225));
#16996=CARTESIAN_POINT('Ctrl Pts',(18.3333666250123,65.9985354189832,26.9785196366098));
#16997=CARTESIAN_POINT('Ctrl Pts',(18.3365469699001,65.9994718481762,27.1714803633902));
#16998=CARTESIAN_POINT('Ctrl Pts',(18.3358498953606,65.7543196540673,27.1878148018157));
#16999=CARTESIAN_POINT('Ctrl Pts',(18.3865445959424,65.5094417423179,27.2041492402413));
#17000=CARTESIAN_POINT('Ctrl Pts',(18.4900815811632,65.2894314428002,27.2204836786668));
#17001=CARTESIAN_POINT('Ctrl Pts',(18.7248899391301,64.7904768223294,27.2575280513307));
#17002=CARTESIAN_POINT('Ctrl Pts',(19.2314784001046,64.419422088475,27.2945724239945));
#17003=CARTESIAN_POINT('Ctrl Pts',(19.7780221138092,64.3460691902049,27.3316167966584));
#17004=CARTESIAN_POINT('Ctrl Pts',(20.3245658275138,64.2727162919348,27.3686611693222));
#17005=CARTESIAN_POINT('Ctrl Pts',(20.9110647939486,64.497065229249,27.4057055419861));
#17006=CARTESIAN_POINT('Ctrl Pts',(21.2691255443732,64.9164495130527,27.4427499146499));
#17007=CARTESIAN_POINT('Ctrl Pts',(21.6271862947977,65.3358337968564,27.4797942873138));
#17008=CARTESIAN_POINT('Ctrl Pts',(21.756808829212,65.9502534271496,27.5168386599777));
#17009=CARTESIAN_POINT('Ctrl Pts',(21.598675324677,66.4785378895678,27.5538830326415));
#17010=CARTESIAN_POINT('Ctrl Pts',(21.4405418201421,67.006822351986,27.5909274053054));
#17011=CARTESIAN_POINT('Ctrl Pts',(20.9946522766579,67.4489716465293,27.6279717779692));
#17012=CARTESIAN_POINT('Ctrl Pts',(20.4650545244661,67.602649554542,27.6650161506331));
#17013=CARTESIAN_POINT('Ctrl Pts',(19.9354567722743,67.7563274625547,27.7020605232969));
#17014=CARTESIAN_POINT('Ctrl Pts',(19.3221508113749,67.6215339840369,27.7391048959608));
#17015=CARTESIAN_POINT('Ctrl Pts',(18.9057975191576,67.2599532674978,27.7761492686246));
#17016=CARTESIAN_POINT('Ctrl Pts',(18.5486455209627,66.949785729893,27.8079263002132));
#17017=CARTESIAN_POINT('Ctrl Pts',(18.3364187640716,66.4727395436526,27.8397033318017));
#17018=CARTESIAN_POINT('Ctrl Pts',(18.3324919306138,65.9987669699924,27.8714803633902));
#17019=CARTESIAN_POINT('Origin',(20.,66.,30.));
#17020=CARTESIAN_POINT('',(18.3327118712203,66.00131037449,28.5714803633902));
#17021=CARTESIAN_POINT('',(18.3362664966243,66.0008554996272,28.3785196366098));
#17022=CARTESIAN_POINT('',(18.334,66.,30.));
#17023=CARTESIAN_POINT('Ctrl Pts',(18.3362664966243,66.0008554996272,28.3785196366098));
#17024=CARTESIAN_POINT('Ctrl Pts',(18.335230442349,66.2235152604115,28.3636776043221));
#17025=CARTESIAN_POINT('Ctrl Pts',(18.3767829793478,66.4458041872034,28.3488355720344));
#17026=CARTESIAN_POINT('Ctrl Pts',(18.4627526155864,66.6493313864273,28.3339935397468));
#17027=CARTESIAN_POINT('Ctrl Pts',(18.6773250663718,67.157316901426,28.2969491670829));
#17028=CARTESIAN_POINT('Ctrl Pts',(19.1685967388456,67.5484250087499,28.2599047944191));
#17029=CARTESIAN_POINT('Ctrl Pts',(19.7117520475599,67.6436769415562,28.2228604217552));
#17030=CARTESIAN_POINT('Ctrl Pts',(20.2549073562742,67.7389288743626,28.1858160490914));
#17031=CARTESIAN_POINT('Ctrl Pts',(20.8499463012292,67.5383246326514,28.1487716764275));
#17032=CARTESIAN_POINT('Ctrl Pts',(21.2245673509439,67.1336646652802,28.1117273037636));
#17033=CARTESIAN_POINT('Ctrl Pts',(21.5991884006587,66.7290046979089,28.0746829310998));
#17034=CARTESIAN_POINT('Ctrl Pts',(21.7533915551334,66.1202890048776,28.037638558436));
#17035=CARTESIAN_POINT('Ctrl Pts',(21.6166104162258,65.5860778667307,28.0005941857721));
#17036=CARTESIAN_POINT('Ctrl Pts',(21.4798292773182,65.0518667285838,27.9635498131083));
#17037=CARTESIAN_POINT('Ctrl Pts',(21.0520638450283,64.5921601453213,27.9265054404444));
#17038=CARTESIAN_POINT('Ctrl Pts',(20.5290679994459,64.417328896371,27.8894610677805));
#17039=CARTESIAN_POINT('Ctrl Pts',(20.0060721538635,64.2424976474206,27.8524166951167));
#17040=CARTESIAN_POINT('Ctrl Pts',(19.3878458949885,64.3525417327825,27.8153723224528));
#17041=CARTESIAN_POINT('Ctrl Pts',(18.9573017255916,64.6971028133696,27.778327949789));
#17042=CARTESIAN_POINT('Ctrl Pts',(18.5706313246055,65.0065520654206,27.7450585120626));
#17043=CARTESIAN_POINT('Ctrl Pts',(18.3353411892483,65.5051575930141,27.7117890743362));
#17044=CARTESIAN_POINT('Ctrl Pts',(18.3319383951835,66.0009590761175,27.6785196366098));
#17045=CARTESIAN_POINT('Ctrl Pts',(18.3324919306138,65.9987669699924,27.8714803633902));
#17046=CARTESIAN_POINT('Ctrl Pts',(18.3318410211319,65.9202015697327,27.8767477044655));
#17047=CARTESIAN_POINT('Ctrl Pts',(18.3369133962315,65.8417206205816,27.8820150455409));
#17048=CARTESIAN_POINT('Ctrl Pts',(18.3479976916752,65.7640981587772,27.8872823866162));
#17049=CARTESIAN_POINT('Ctrl Pts',(18.425951779945,65.218191721156,27.92432675928));
#17050=CARTESIAN_POINT('Ctrl Pts',(18.8012605800197,64.714746800474,27.9613711319439));
#17051=CARTESIAN_POINT('Ctrl Pts',(19.3021753989644,64.4841497001422,27.9984155046077));
#17052=CARTESIAN_POINT('Ctrl Pts',(19.803090217909,64.2535525998103,28.0354598772716));
#17053=CARTESIAN_POINT('Ctrl Pts',(20.4296110557237,64.2958033198288,28.0725042499354));
#17054=CARTESIAN_POINT('Ctrl Pts',(20.8950296472222,64.5915670992272,28.1095486225993));
#17055=CARTESIAN_POINT('Ctrl Pts',(21.3604482387207,64.8873308786256,28.1465929952632));
#17056=CARTESIAN_POINT('Ctrl Pts',(21.664764583903,65.436607717404,28.183637367927));
#17057=CARTESIAN_POINT('Ctrl Pts',(21.6687175343226,65.9880377244764,28.2206817405909));
#17058=CARTESIAN_POINT('Ctrl Pts',(21.6726704847421,66.5394677315488,28.2577261132547));
#17059=CARTESIAN_POINT('Ctrl Pts',(21.3762600403988,67.0930509069152,28.2947704859186));
#17060=CARTESIAN_POINT('Ctrl Pts',(20.9151294539268,67.3954566951163,28.3318148585824));
#17061=CARTESIAN_POINT('Ctrl Pts',(20.4539988674548,67.6978624833174,28.3688592312463));
#17062=CARTESIAN_POINT('Ctrl Pts',(19.8281481388542,67.7490908843532,28.4059036039102));
#17063=CARTESIAN_POINT('Ctrl Pts',(19.3239788781539,67.525698773745,28.442947976574));
#17064=CARTESIAN_POINT('Ctrl Pts',(18.8198096174536,67.3023066631369,28.4799923492379));
#17065=CARTESIAN_POINT('Ctrl Pts',(18.4373218246536,66.8042940408847,28.5170367219017));
#17066=CARTESIAN_POINT('Ctrl Pts',(18.3515494410261,66.2595612837239,28.5540810945655));
#17067=CARTESIAN_POINT('Ctrl Pts',(18.3381207099022,66.1742766102555,28.5598808508404));
#17068=CARTESIAN_POINT('Ctrl Pts',(18.3319650040854,66.0878467427289,28.5656806071153));
#17069=CARTESIAN_POINT('Ctrl Pts',(18.3327118712203,66.00131037449,28.5714803633902));
#17070=CARTESIAN_POINT('Origin',(20.,66.,30.));
#17071=CARTESIAN_POINT('',(18.3366137112403,66.0004031163585,29.2714803633902));
#17072=CARTESIAN_POINT('',(18.3350591421361,65.9985780813516,29.0785196366098));
#17073=CARTESIAN_POINT('',(18.334,66.,30.));
#17074=CARTESIAN_POINT('Ctrl Pts',(18.3350591421361,65.9985780813516,29.0785196366098));
#17075=CARTESIAN_POINT('Ctrl Pts',(18.3382113409887,66.3865573365257,29.0526105069719));
#17076=CARTESIAN_POINT('Ctrl Pts',(18.4733909534641,66.7765166182576,29.026701377334));
#17077=CARTESIAN_POINT('Ctrl Pts',(18.7211704627318,67.0720801205599,29.0007922476961));
#17078=CARTESIAN_POINT('Ctrl Pts',(19.0754408148456,67.4946711021229,28.9637478750323));
#17079=CARTESIAN_POINT('Ctrl Pts',(19.6598960683787,67.7242913634506,28.9267035023684));
#17080=CARTESIAN_POINT('Ctrl Pts',(20.2070779973473,67.6558621540768,28.8896591297046));
#17081=CARTESIAN_POINT('Ctrl Pts',(20.7542599263159,67.587432944703,28.8526147570407));
#17082=CARTESIAN_POINT('Ctrl Pts',(21.2641685307198,67.2209542646277,28.8155703843768));
#17083=CARTESIAN_POINT('Ctrl Pts',(21.5034595982802,66.7241339700834,28.778526011713));
#17084=CARTESIAN_POINT('Ctrl Pts',(21.7427506658405,66.2273136755392,28.7414816390491));
#17085=CARTESIAN_POINT('Ctrl Pts',(21.7114241965572,65.600151766526,28.7044372663853));
#17086=CARTESIAN_POINT('Ctrl Pts',(21.4238157992737,65.1296498750344,28.6673928937215));
#17087=CARTESIAN_POINT('Ctrl Pts',(21.1362074019901,64.6591479835428,28.6303485210576));
#17088=CARTESIAN_POINT('Ctrl Pts',(20.5923170767064,64.3453061095728,28.5933041483937));
#17089=CARTESIAN_POINT('Ctrl Pts',(20.0410397399286,64.3317444710009,28.5562597757299));
#17090=CARTESIAN_POINT('Ctrl Pts',(19.4897624031508,64.318182832429,28.519215403066));
#17091=CARTESIAN_POINT('Ctrl Pts',(18.9310980548789,64.6049014292553,28.4821710304022));
#17092=CARTESIAN_POINT('Ctrl Pts',(18.6207024952914,65.0606921890052,28.4451266577383));
#17093=CARTESIAN_POINT('Ctrl Pts',(18.4346686291561,65.3338678661887,28.4229243173622));
#17094=CARTESIAN_POINT('Ctrl Pts',(18.337816340286,65.6677765990296,28.400721976986));
#17095=CARTESIAN_POINT('Ctrl Pts',(18.3362664966243,66.0008554996272,28.3785196366098));
#17096=CARTESIAN_POINT('Ctrl Pts',(18.3327118712203,66.00131037449,28.5714803633902));
#17097=CARTESIAN_POINT('Ctrl Pts',(18.3367354156621,65.5351191241736,28.6027249797792));
#17098=CARTESIAN_POINT('Ctrl Pts',(18.5410870786598,65.0658369847815,28.6339695961681));
#17099=CARTESIAN_POINT('Ctrl Pts',(18.8878468378532,64.7558630906061,28.6652142125571));
#17100=CARTESIAN_POINT('Ctrl Pts',(19.2989735927628,64.3883505467185,28.702258585221));
#17101=CARTESIAN_POINT('Ctrl Pts',(19.9102840770369,64.2447783510127,28.7393029578848));
#17102=CARTESIAN_POINT('Ctrl Pts',(20.4420305825988,64.3908479657171,28.7763473305487));
#17103=CARTESIAN_POINT('Ctrl Pts',(20.9737770881607,64.5369175804214,28.8133917032125));
#17104=CARTESIAN_POINT('Ctrl Pts',(21.4259596150103,64.9726290055359,28.8504360758764));
#17105=CARTESIAN_POINT('Ctrl Pts',(21.5916505399959,65.4985921182107,28.8874804485402));
#17106=CARTESIAN_POINT('Ctrl Pts',(21.7573414649814,66.0245552308856,28.9245248212041));
#17107=CARTESIAN_POINT('Ctrl Pts',(21.6365407881028,66.6407700311209,28.9615691938679));
#17108=CARTESIAN_POINT('Ctrl Pts',(21.2845292764339,67.0652444993399,28.9986135665318));
#17109=CARTESIAN_POINT('Ctrl Pts',(20.932517764765,67.4897189675588,29.0356579391956));
#17110=CARTESIAN_POINT('Ctrl Pts',(20.3492954183058,67.7224531037614,29.0727023118595));
#17111=CARTESIAN_POINT('Ctrl Pts',(19.8017562604999,67.6569431870581,29.1097466845233));
#17112=CARTESIAN_POINT('Ctrl Pts',(19.2542171026941,67.5914332703549,29.1467910571872));
#17113=CARTESIAN_POINT('Ctrl Pts',(18.7423611335417,67.2276793007459,29.183835429851));
#17114=CARTESIAN_POINT('Ctrl Pts',(18.500423717754,66.7321422533326,29.2208798025149));
#17115=CARTESIAN_POINT('Ctrl Pts',(18.3902660153803,66.5065168683279,29.23774665614));
#17116=CARTESIAN_POINT('Ctrl Pts',(18.3360655678455,66.2535713188655,29.2546135097651));
#17117=CARTESIAN_POINT('Ctrl Pts',(18.3366137112403,66.0004031163585,29.2714803633902));
#17118=CARTESIAN_POINT('Origin',(20.,66.,30.));
#17119=CARTESIAN_POINT('',(18.3341898066152,65.9984774012779,29.9714803633902));
#17120=CARTESIAN_POINT('',(18.331239919894,65.9999810457215,29.7785196366098));
#17121=CARTESIAN_POINT('',(18.334,66.,30.));
#17122=CARTESIAN_POINT('Ctrl Pts',(18.3312400241975,65.9999810464378,29.7785196366098));
#17123=CARTESIAN_POINT('Ctrl Pts',(18.3313325829903,66.5504109935318,29.7415434096217));
#17124=CARTESIAN_POINT('Ctrl Pts',(18.6304405504474,67.1009271285011,29.7045671826336));
#17125=CARTESIAN_POINT('Ctrl Pts',(19.0923261408273,67.400317441034,29.6675909556455));
#17126=CARTESIAN_POINT('Ctrl Pts',(19.5550629674809,67.7002595176819,29.6305465829816));
#17127=CARTESIAN_POINT('Ctrl Pts',(20.1811779549493,67.7481492896818,29.5935022103178));
#17128=CARTESIAN_POINT('Ctrl Pts',(20.6841485631442,67.5220714549051,29.5564578376539));
#17129=CARTESIAN_POINT('Ctrl Pts',(21.1871191713391,67.2959936201285,29.5194134649901));
#17130=CARTESIAN_POINT('Ctrl Pts',(21.5669454002605,66.7959481785752,29.4823690923262));
#17131=CARTESIAN_POINT('Ctrl Pts',(21.6498112926465,66.2507657650985,29.4453247196624));
#17132=CARTESIAN_POINT('Ctrl Pts',(21.7326771850326,65.7055833516217,29.4082803469985));
#17133=CARTESIAN_POINT('Ctrl Pts',(21.5185827408833,65.1152639662215,29.3712359743347));
#17134=CARTESIAN_POINT('Ctrl Pts',(21.105501791179,64.7499493770293,29.3341916016708));
#17135=CARTESIAN_POINT('Ctrl Pts',(20.6924208414747,64.3846347878371,29.2971472290069));
#17136=CARTESIAN_POINT('Ctrl Pts',(20.0803533862155,64.2443249948529,29.2601028563431));
#17137=CARTESIAN_POINT('Ctrl Pts',(19.549393538298,64.3932285206161,29.2230584836792));
#17138=CARTESIAN_POINT('Ctrl Pts',(19.0184336903805,64.5421320463792,29.1860141110154));
#17139=CARTESIAN_POINT('Ctrl Pts',(18.5685814498048,64.9802488908897,29.1489697383516));
#17140=CARTESIAN_POINT('Ctrl Pts',(18.4056980548641,65.5070881640441,29.1119253656877));
#17141=CARTESIAN_POINT('Ctrl Pts',(18.356736605199,65.6654518484674,29.1007901226617));
#17142=CARTESIAN_POINT('Ctrl Pts',(18.3337043880097,65.8318320981489,29.0896548796358));
#17143=CARTESIAN_POINT('Ctrl Pts',(18.3350591421361,65.9985780813516,29.0785196366098));
#17144=CARTESIAN_POINT('Ctrl Pts',(18.3366137112403,66.0004031163585,29.2714803633902));
#17145=CARTESIAN_POINT('Ctrl Pts',(18.3372694455005,65.6975424679157,29.291657882429));
#17146=CARTESIAN_POINT('Ctrl Pts',(18.4162754187729,65.3943631826101,29.3118354014677));
#17147=CARTESIAN_POINT('Ctrl Pts',(18.5715624112669,65.1372559125187,29.3320129205065));
#17148=CARTESIAN_POINT('Ctrl Pts',(18.8566573829902,64.6652267443359,29.3690572931703));
#17149=CARTESIAN_POINT('Ctrl Pts',(19.3988661888596,64.3484885331883,29.4061016658342));
#17150=CARTESIAN_POINT('Ctrl Pts',(19.950063408744,64.3319869178441,29.443146038498));
#17151=CARTESIAN_POINT('Ctrl Pts',(20.5012606286283,64.3154853024999,29.4801904111619));
#17152=CARTESIAN_POINT('Ctrl Pts',(21.0614462625275,64.5992202829592,29.5172347838257));
#17153=CARTESIAN_POINT('Ctrl Pts',(21.3742683400236,65.0533491483137,29.5542791564896));
#17154=CARTESIAN_POINT('Ctrl Pts',(21.6870904175196,65.5074780136683,29.5913235291534));
#17155=CARTESIAN_POINT('Ctrl Pts',(21.7525489386125,66.1320007639182,29.6283679018173));
#17156=CARTESIAN_POINT('Ctrl Pts',(21.5406887958389,66.6411234980611,29.6654122744811));
#17157=CARTESIAN_POINT('Ctrl Pts',(21.3288286530653,67.150246232204,29.702456647145));
#17158=CARTESIAN_POINT('Ctrl Pts',(20.8396498464252,67.5439689502399,29.7395010198089));
#17159=CARTESIAN_POINT('Ctrl Pts',(20.2970102247823,67.6421163880079,29.7765453924727));
#17160=CARTESIAN_POINT('Ctrl Pts',(19.7543706031394,67.740263825776,29.8135897651366));
#17161=CARTESIAN_POINT('Ctrl Pts',(19.1582701664937,67.5428359832763,29.8506341378004));
#17162=CARTESIAN_POINT('Ctrl Pts',(18.7814962057965,67.1401797265787,29.8876785104642));
#17163=CARTESIAN_POINT('Ctrl Pts',(18.4973832733844,66.8365498004747,29.9156124614396));
#17164=CARTESIAN_POINT('Ctrl Pts',(18.3379832198998,66.4162234004879,29.9435464124149));
#17165=CARTESIAN_POINT('Ctrl Pts',(18.3341898066152,65.9984774012779,29.9714803633902));
#17166=CARTESIAN_POINT('Origin',(20.,66.,30.));
#17167=CARTESIAN_POINT('',(18.3314457742944,66.0005306220934,30.6714803633902));
#17168=CARTESIAN_POINT('',(18.3350038845013,66.001433884838,30.4785196366098));
#17169=CARTESIAN_POINT('',(18.334,66.,30.));
#17170=CARTESIAN_POINT('Ctrl Pts',(18.3350038845013,66.001433884838,30.4785196366098));
#17171=CARTESIAN_POINT('Ctrl Pts',(18.3336511769542,66.1661251266506,30.4675206849353));
#17172=CARTESIAN_POINT('Ctrl Pts',(18.3561120206751,66.3304555620997,30.4565217332608));
#17173=CARTESIAN_POINT('Ctrl Pts',(18.4038997873377,66.4870573697509,30.4455227815864));
#17174=CARTESIAN_POINT('Ctrl Pts',(18.5648485658592,67.0144908828857,30.4084784089225));
#17175=CARTESIAN_POINT('Ctrl Pts',(19.0130898719618,67.4542557510803,30.3714340362587));
#17176=CARTESIAN_POINT('Ctrl Pts',(19.54349966267,67.6051069161607,30.3343896635948));
#17177=CARTESIAN_POINT('Ctrl Pts',(20.0739094533782,67.7559580812411,30.297345290931));
#17178=CARTESIAN_POINT('Ctrl Pts',(20.6864877286921,67.6178955432072,30.2603009182671));
#17179=CARTESIAN_POINT('Ctrl Pts',(21.1009066144049,67.2540994365077,30.2232565456033));
#17180=CARTESIAN_POINT('Ctrl Pts',(21.5153255001178,66.8903033298081,30.1862121729394));
#17181=CARTESIAN_POINT('Ctrl Pts',(21.7315849962297,66.3007736544428,30.1491678002756));
#17182=CARTESIAN_POINT('Ctrl Pts',(21.6507205013744,65.7552907916899,30.1121234276117));
#17183=CARTESIAN_POINT('Ctrl Pts',(21.5698560065191,65.2098079289371,30.0750790549479));
#17184=CARTESIAN_POINT('Ctrl Pts',(21.1918675206966,64.7083718787967,30.038034682284));
#17185=CARTESIAN_POINT('Ctrl Pts',(20.6897300137602,64.4804496459782,30.0009903096202));
#17186=CARTESIAN_POINT('Ctrl Pts',(20.1875925068238,64.2525274131597,29.9639459369563));
#17187=CARTESIAN_POINT('Ctrl Pts',(19.5613059787735,64.2981189976632,29.9269015642925));
#17188=CARTESIAN_POINT('Ctrl Pts',(19.0974714700439,64.5963607931863,29.8898571916286));
#17189=CARTESIAN_POINT('Ctrl Pts',(18.6327837057788,64.8951512250401,29.852744673289));
#17190=CARTESIAN_POINT('Ctrl Pts',(18.3311471242406,65.4475222595322,29.8156321549494));
#17191=CARTESIAN_POINT('Ctrl Pts',(18.3312400241975,65.9999810464378,29.7785196366098));
#17192=CARTESIAN_POINT('Ctrl Pts',(18.3341898066152,65.9984774012779,29.9714803633902));
#17193=CARTESIAN_POINT('Ctrl Pts',(18.3329526169784,65.8622330792747,29.9805907850787));
#17194=CARTESIAN_POINT('Ctrl Pts',(18.348267041402,65.72626323012,29.9897012067673));
#17195=CARTESIAN_POINT('Ctrl Pts',(18.3812048191077,65.5947057023479,29.9988116284558));
#17196=CARTESIAN_POINT('Ctrl Pts',(18.5151348778648,65.0597726057102,30.0358560011197));
#17197=CARTESIAN_POINT('Ctrl Pts',(18.9404424801278,64.59779108333,30.0729003737835));
#17198=CARTESIAN_POINT('Ctrl Pts',(19.462498497129,64.4201729715564,30.1099447464474));
#17199=CARTESIAN_POINT('Ctrl Pts',(19.9845545141302,64.2425548597828,30.1469891191112));
#17200=CARTESIAN_POINT('Ctrl Pts',(20.6033589458697,64.3493001586158,30.1840334917751));
#17201=CARTESIAN_POINT('Ctrl Pts',(21.0357347064309,64.6915601185824,30.2210778644389));
#17202=CARTESIAN_POINT('Ctrl Pts',(21.468110466992,65.033820078549,30.2581222371028));
#17203=CARTESIAN_POINT('Ctrl Pts',(21.7140575563749,65.6115946996491,30.2951666097666));
#17204=CARTESIAN_POINT('Ctrl Pts',(21.6610257462864,66.1604829447737,30.3322109824305));
#17205=CARTESIAN_POINT('Ctrl Pts',(21.6079939361978,66.7093711898982,30.3692553550943));
#17206=CARTESIAN_POINT('Ctrl Pts',(21.2559832266379,67.2293730590472,30.4062997277582));
#17207=CARTESIAN_POINT('Ctrl Pts',(20.7660806458043,67.4825254633609,30.4433441004221));
#17208=CARTESIAN_POINT('Ctrl Pts',(20.2761780649708,67.7356778676746,30.4803884730859));
#17209=CARTESIAN_POINT('Ctrl Pts',(19.6483836128637,67.7219808071531,30.5174328457497));
#17210=CARTESIAN_POINT('Ctrl Pts',(19.1699883856417,67.4477023262466,30.5544772184136));
#17211=CARTESIAN_POINT('Ctrl Pts',(18.6915931584198,67.1734238453401,30.5915215910774));
#17212=CARTESIAN_POINT('Ctrl Pts',(18.3625971560829,66.6385639440485,30.6285659637413));
#17213=CARTESIAN_POINT('Ctrl Pts',(18.3335554238786,66.0878850391431,30.6656103364052));
#17214=CARTESIAN_POINT('Ctrl Pts',(18.3320214459357,66.0587982998317,30.6675670120668));
#17215=CARTESIAN_POINT('Ctrl Pts',(18.3313243191979,66.0296674266187,30.6695236877285));
#17216=CARTESIAN_POINT('Ctrl Pts',(18.3314457742944,66.0005306220934,30.6714803633902));
#17217=CARTESIAN_POINT('Origin',(20.,66.,30.));
#17218=CARTESIAN_POINT('',(18.3357539380163,66.0011866318746,31.3714803633902));
#17219=CARTESIAN_POINT('',(18.3362976425678,65.9991726430109,31.1785196366098));
#17220=CARTESIAN_POINT('',(18.334,66.,30.));
#17221=CARTESIAN_POINT('Ctrl Pts',(18.3362976425678,65.9991726430109,31.1785196366098));
#17222=CARTESIAN_POINT('Ctrl Pts',(18.3377856536118,66.3302224149229,31.1564535875851));
#17223=CARTESIAN_POINT('Ctrl Pts',(18.4333702676718,66.662063920961,31.1343875385604));
#17224=CARTESIAN_POINT('Ctrl Pts',(18.6172644901874,66.9342394126736,31.1123214895358));
#17225=CARTESIAN_POINT('Ctrl Pts',(18.9259851905709,67.3911662659444,31.0752771168719));
#17226=CARTESIAN_POINT('Ctrl Pts',(19.4835935086859,67.6799332504904,31.038232744208));
#17227=CARTESIAN_POINT('Ctrl Pts',(20.0349169045382,67.6683949113045,31.0011883715442));
#17228=CARTESIAN_POINT('Ctrl Pts',(20.5862403003904,67.6568565721186,30.9641439988803));
#17229=CARTESIAN_POINT('Ctrl Pts',(21.13127877398,67.3450129092009,30.9270996262165));
#17230=CARTESIAN_POINT('Ctrl Pts',(21.4206119935396,66.8755697197258,30.8900552535526));
#17231=CARTESIAN_POINT('Ctrl Pts',(21.7099452130993,66.4061265302508,30.8530108808888));
#17232=CARTESIAN_POINT('Ctrl Pts',(21.743573178629,65.7790838142184,30.8159665082249));
#17233=CARTESIAN_POINT('Ctrl Pts',(21.5061070713104,65.2813886585656,30.7789221355611));
#17234=CARTESIAN_POINT('Ctrl Pts',(21.2686409639919,64.7836935029129,30.7418777628972));
#17235=CARTESIAN_POINT('Ctrl Pts',(20.7600807838251,64.4153459076396,30.7048333902334));
#17236=CARTESIAN_POINT('Ctrl Pts',(20.2131536776213,64.344908981353,30.6677890175695));
#17237=CARTESIAN_POINT('Ctrl Pts',(19.6662265714174,64.2744720550664,30.6307446449057));
#17238=CARTESIAN_POINT('Ctrl Pts',(19.0809325391764,64.5019457977663,30.5937002722418));
#17239=CARTESIAN_POINT('Ctrl Pts',(18.7251136485261,64.9232337481538,30.556655899578));
#17240=CARTESIAN_POINT('Ctrl Pts',(18.4749419723296,65.2194358764815,30.5306104785886));
#17241=CARTESIAN_POINT('Ctrl Pts',(18.3382070840956,65.6114464702889,30.5045650575992));
#17242=CARTESIAN_POINT('Ctrl Pts',(18.3350038845013,66.001433884838,30.4785196366098));
#17243=CARTESIAN_POINT('Ctrl Pts',(18.3314457742944,66.0005306220934,30.6714803633902));
#17244=CARTESIAN_POINT('Ctrl Pts',(18.3336237436472,65.478040672012,30.7065680603924));
#17245=CARTESIAN_POINT('Ctrl Pts',(18.5990309619734,64.9536434051272,30.7416557573945));
#17246=CARTESIAN_POINT('Ctrl Pts',(19.0223181288011,64.6476319050944,30.7767434543967));
#17247=CARTESIAN_POINT('Ctrl Pts',(19.4692100279994,64.3245555844701,30.8137878270606));
#17248=CARTESIAN_POINT('Ctrl Pts',(20.0920812884675,64.2449008517406,30.8508321997244));
#17249=CARTESIAN_POINT('Ctrl Pts',(20.6058937634283,64.4451192801928,30.8878765723883));
#17250=CARTESIAN_POINT('Ctrl Pts',(21.1197062383891,64.645337708645,30.9249209450521));
#17251=CARTESIAN_POINT('Ctrl Pts',(21.5244599278425,65.1254292982789,30.961965317716));
#17252=CARTESIAN_POINT('Ctrl Pts',(21.6349315780197,65.6656946895675,30.9990096903798));
#17253=CARTESIAN_POINT('Ctrl Pts',(21.745403228197,66.2059600808562,31.0360540630437));
#17254=CARTESIAN_POINT('Ctrl Pts',(21.561592839098,66.8063992737996,31.0730984357076));
#17255=CARTESIAN_POINT('Ctrl Pts',(21.1676156621277,67.1922394771788,31.1101428083714));
#17256=CARTESIAN_POINT('Ctrl Pts',(20.7736384851573,67.578079680558,31.1471871810353));
#17257=CARTESIAN_POINT('Ctrl Pts',(20.1694945203157,67.7493208943729,31.1842315536991));
#17258=CARTESIAN_POINT('Ctrl Pts',(19.6316519353517,67.6275997691876,31.221275926363));
#17259=CARTESIAN_POINT('Ctrl Pts',(19.0938093503877,67.5058786440022,31.2583202990268));
#17260=CARTESIAN_POINT('Ctrl Pts',(18.6222681453012,67.0911951798166,31.2953646716907));
#17261=CARTESIAN_POINT('Ctrl Pts',(18.4328148553804,66.5733166907331,31.3324090443545));
#17262=CARTESIAN_POINT('Ctrl Pts',(18.3662083381997,66.391244991186,31.3454328173664));
#17263=CARTESIAN_POINT('Ctrl Pts',(18.3344687445157,66.1964180729821,31.3584565903783));
#17264=CARTESIAN_POINT('Ctrl Pts',(18.3357539380163,66.0011866318746,31.3714803633902));
#17265=CARTESIAN_POINT('Origin',(20.,66.,30.));
#17266=CARTESIAN_POINT('',(18.3357307739255,65.9988024507997,32.0714803633902));
#17267=CARTESIAN_POINT('',(18.3319842739515,65.9990126572197,31.8785196366098));
#17268=CARTESIAN_POINT('',(18.334,66.,30.));
#17269=CARTESIAN_POINT('Ctrl Pts',(18.3319842739515,65.9990126572197,31.8785196366098));
#17270=CARTESIAN_POINT('Ctrl Pts',(18.3354516324952,66.4928187659276,31.8453864902349));
#17271=CARTESIAN_POINT('Ctrl Pts',(18.5685743286719,66.9894689012208,31.81225334386));
#17272=CARTESIAN_POINT('Ctrl Pts',(18.9525270673117,67.2990616711976,31.7791201974851));
#17273=CARTESIAN_POINT('Ctrl Pts',(19.3818037853917,67.6452005441947,31.7420758248213));
#17274=CARTESIAN_POINT('Ctrl Pts',(19.9996220148489,67.7575128015186,31.7050314521574));
#17275=CARTESIAN_POINT('Ctrl Pts',(20.5232559753395,67.5846021439342,31.6679870794935));
#17276=CARTESIAN_POINT('Ctrl Pts',(21.04688993583,67.4116914863498,31.6309427068297));
#17277=CARTESIAN_POINT('Ctrl Pts',(21.4763396273538,66.9535579138571,31.5938983341658));
#17278=CARTESIAN_POINT('Ctrl Pts',(21.615080419582,66.4198523652096,31.556853961502));
#17279=CARTESIAN_POINT('Ctrl Pts',(21.7538212118103,65.8861468165621,31.5198095888381));
#17280=CARTESIAN_POINT('Ctrl Pts',(21.601853104743,65.2768692917598,31.4827652161743));
#17281=CARTESIAN_POINT('Ctrl Pts',(21.2287196948773,64.8708371766171,31.4457208435104));
#17282=CARTESIAN_POINT('Ctrl Pts',(20.8555862850116,64.4648050614744,31.4086764708466));
#17283=CARTESIAN_POINT('Ctrl Pts',(20.2612875723476,64.2620183559913,31.3716320981827));
#17284=CARTESIAN_POINT('Ctrl Pts',(19.7177863434849,64.3552762474003,31.3345877255189));
#17285=CARTESIAN_POINT('Ctrl Pts',(19.1742851146223,64.4485341388093,31.297543352855));
#17286=CARTESIAN_POINT('Ctrl Pts',(18.681581369561,64.8378366271104,31.2604989801912));
#17287=CARTESIAN_POINT('Ctrl Pts',(18.4651460383564,65.3450312322588,31.2234546075273));
#17288=CARTESIAN_POINT('Ctrl Pts',(18.3776337333931,65.550107587928,31.2084762838881));
#17289=CARTESIAN_POINT('Ctrl Pts',(18.3352875881185,65.7744577147142,31.193497960249));
#17290=CARTESIAN_POINT('Ctrl Pts',(18.3362976425678,65.9991726430109,31.1785196366098));
#17291=CARTESIAN_POINT('Ctrl Pts',(18.3357539380163,66.0011866318746,31.3714803633902));
#17292=CARTESIAN_POINT('Ctrl Pts',(18.3381243047699,65.6411084669653,31.3955009630422));
#17293=CARTESIAN_POINT('Ctrl Pts',(18.4528345838942,65.2796542426953,31.4195215626941));
#17294=CARTESIAN_POINT('Ctrl Pts',(18.6683273035712,64.9943116113947,31.4435421623461));
#17295=CARTESIAN_POINT('Ctrl Pts',(19.000658416438,64.5542585351211,31.4805865350099));
#17296=CARTESIAN_POINT('Ctrl Pts',(19.5726860169266,64.295225896555,31.5176309076738));
#17297=CARTESIAN_POINT('Ctrl Pts',(20.1226390176602,64.3357521288171,31.5546752803376));
#17298=CARTESIAN_POINT('Ctrl Pts',(20.6725920183937,64.3762783610791,31.5917196530015));
#17299=CARTESIAN_POINT('Ctrl Pts',(21.2004704193721,64.7163634641693,31.6287640256654));
#17300=CARTESIAN_POINT('Ctrl Pts',(21.4647066757619,65.200377802104,31.6658083983292));
#17301=CARTESIAN_POINT('Ctrl Pts',(21.7289429321517,65.6843921400386,31.7028527709931));
#17302=CARTESIAN_POINT('Ctrl Pts',(21.7295370439529,66.3123357128176,31.7398971436569));
#17303=CARTESIAN_POINT('Ctrl Pts',(21.4662171339133,66.7968491837283,31.7769415163207));
#17304=CARTESIAN_POINT('Ctrl Pts',(21.2028972238738,67.281362654639,31.8139858889846));
#17305=CARTESIAN_POINT('Ctrl Pts',(20.6756632919933,67.6224460236814,31.8510302616485));
#17306=CARTESIAN_POINT('Ctrl Pts',(20.1257879613633,67.6640128287263,31.8880746343123));
#17307=CARTESIAN_POINT('Ctrl Pts',(19.5759126307332,67.7055796337712,31.9251190069762));
#17308=CARTESIAN_POINT('Ctrl Pts',(19.0033959013535,67.4476298748186,31.96216337964));
#17309=CARTESIAN_POINT('Ctrl Pts',(18.6702326956076,67.0082064379672,31.9992077523039));
#17310=CARTESIAN_POINT('Ctrl Pts',(18.4535684353736,66.7224385253258,32.023298622666));
#17311=CARTESIAN_POINT('Ctrl Pts',(18.3381320961367,66.3599213639141,32.0473894930281));
#17312=CARTESIAN_POINT('Ctrl Pts',(18.3357307739255,65.9988024507997,32.0714803633902));
#17313=CARTESIAN_POINT('Origin',(20.,66.,30.));
#17314=CARTESIAN_POINT('',(18.3314318999871,65.9994875421513,32.7714803633902));
#17315=CARTESIAN_POINT('',(18.3333052932669,66.0014544402739,32.5785196366098));
#17316=CARTESIAN_POINT('',(18.334,66.,30.));
#17317=CARTESIAN_POINT('Ctrl Pts',(18.3333052932669,66.0014544402739,32.5785196366098));
#17318=CARTESIAN_POINT('Ctrl Pts',(18.3323271062934,66.1083233110254,32.5713637655485));
#17319=CARTESIAN_POINT('Ctrl Pts',(18.3417256310295,66.2150208191139,32.5642078944873));
#17320=CARTESIAN_POINT('Ctrl Pts',(18.3621249858483,66.319571914139,32.557052023426));
#17321=CARTESIAN_POINT('Ctrl Pts',(18.4677279649323,66.8608099679505,32.5200076507622));
#17322=CARTESIAN_POINT('Ctrl Pts',(18.8681427916334,67.3445261805719,32.4829632780983));
#17323=CARTESIAN_POINT('Ctrl Pts',(19.3801317611667,67.5493624936648,32.4459189054345));
#17324=CARTESIAN_POINT('Ctrl Pts',(19.8921207307,67.7541988067578,32.4088745327706));
#17325=CARTESIAN_POINT('Ctrl Pts',(20.5156838430653,67.6801552203222,32.3718301601068));
#17326=CARTESIAN_POINT('Ctrl Pts',(20.9654663464417,67.3611155366749,32.3347857874429));
#17327=CARTESIAN_POINT('Ctrl Pts',(21.4152488498181,67.0420758530276,32.297741414779));
#17328=CARTESIAN_POINT('Ctrl Pts',(21.6912507442055,66.4780400721686,32.2606970421152));
#17329=CARTESIAN_POINT('Ctrl Pts',(21.667168131068,65.9271220675347,32.2236526694513));
#17330=CARTESIAN_POINT('Ctrl Pts',(21.6430855179306,65.3762040629009,32.1866082967875));
#17331=CARTESIAN_POINT('Ctrl Pts',(21.3189183972682,64.8384038344924,32.1495639241236));
#17332=CARTESIAN_POINT('Ctrl Pts',(20.8430120230428,64.5598293506342,32.1125195514598));
#17333=CARTESIAN_POINT('Ctrl Pts',(20.3671056488173,64.281254866776,32.0754751787959));
#17334=CARTESIAN_POINT('Ctrl Pts',(19.7394600210288,64.2619061274682,32.0384308061321));
#17335=CARTESIAN_POINT('Ctrl Pts',(19.2472981308988,64.5106374965976,32.0013864334682));
#17336=CARTESIAN_POINT('Ctrl Pts',(18.7551362407689,64.7593688657269,31.9643420608044));
#17337=CARTESIAN_POINT('Ctrl Pts',(18.3984580882975,65.2761803432934,31.9272976881405));
#17338=CARTESIAN_POINT('Ctrl Pts',(18.3404866154132,65.8245688264118,31.8902533154767));
#17339=CARTESIAN_POINT('Ctrl Pts',(18.3343658598854,65.8824688878111,31.8863420891877));
#17340=CARTESIAN_POINT('Ctrl Pts',(18.3315749670979,65.9407209570542,31.8824308628987));
#17341=CARTESIAN_POINT('Ctrl Pts',(18.3319842739515,65.9990126572197,31.8785196366098));
#17342=CARTESIAN_POINT('Ctrl Pts',(18.3357307739255,65.9988024507997,32.0714803633902));
#17343=CARTESIAN_POINT('Ctrl Pts',(18.3344395987906,65.8046311899893,32.0844338656919));
#17344=CARTESIAN_POINT('Ctrl Pts',(18.3658284528694,65.6108641826254,32.0973873679937));
#17345=CARTESIAN_POINT('Ctrl Pts',(18.431732805963,65.4296498325619,32.1103408702954));
#17346=CARTESIAN_POINT('Ctrl Pts',(18.620205804176,64.9114137787584,32.1473852429593));
#17347=CARTESIAN_POINT('Ctrl Pts',(19.0909614827139,64.4958387859018,32.1844296156231));
#17348=CARTESIAN_POINT('Ctrl Pts',(19.6285727786963,64.3731001491597,32.221473988287));
#17349=CARTESIAN_POINT('Ctrl Pts',(20.1661840746786,64.2503615124175,32.2585183609508));
#17350=CARTESIAN_POINT('Ctrl Pts',(20.7706509881054,64.4204592317899,32.2955627336147));
#17351=CARTESIAN_POINT('Ctrl Pts',(21.1653575635997,64.8055532434009,32.3326071062786));
#17352=CARTESIAN_POINT('Ctrl Pts',(21.5600641390939,65.190647255012,32.3696514789424));
#17353=CARTESIAN_POINT('Ctrl Pts',(21.7450103766556,65.7907375588616,32.4066958516063));
#17354=CARTESIAN_POINT('Ctrl Pts',(21.63556123827,66.3312110222473,32.4437402242701));
#17355=CARTESIAN_POINT('Ctrl Pts',(21.5261120998843,66.871684485633,32.480784596934));
#17356=CARTESIAN_POINT('Ctrl Pts',(21.1222675855513,67.3525411085547,32.5178289695978));
#17357=CARTESIAN_POINT('Ctrl Pts',(20.6088348926125,67.5537314371952,32.5548733422617));
#17358=CARTESIAN_POINT('Ctrl Pts',(20.0954021996737,67.7549217658357,32.5919177149255));
#17359=CARTESIAN_POINT('Ctrl Pts',(19.472381328129,67.676445800195,32.6289620875894));
#17360=CARTESIAN_POINT('Ctrl Pts',(19.0248788897283,67.3542156865465,32.6660064602532));
#17361=CARTESIAN_POINT('Ctrl Pts',(18.6001645498948,67.0483944479364,32.7011644279655));
#17362=CARTESIAN_POINT('Ctrl Pts',(18.3335479895291,66.5230122843236,32.7363223956779));
#17363=CARTESIAN_POINT('Ctrl Pts',(18.3314318999871,65.9994875421513,32.7714803633902));
#17364=CARTESIAN_POINT('Origin',(20.,66.,30.));
#17365=CARTESIAN_POINT('',(18.3342212861325,66.001521965989,33.4714803633902));
#17366=CARTESIAN_POINT('',(18.3367009922703,66.0000736897305,33.2785196366098));
#17367=CARTESIAN_POINT('',(18.334,66.,30.));
#17368=CARTESIAN_POINT('Ctrl Pts',(18.3367009922703,66.0000736897305,33.2785196366098));
#17369=CARTESIAN_POINT('Ctrl Pts',(18.3365930524491,66.2736326347662,33.2602966681983));
#17370=CARTESIAN_POINT('Ctrl Pts',(18.4003187084924,66.5471442261593,33.2420736997869));
#17371=CARTESIAN_POINT('Ctrl Pts',(18.5281535749071,66.7864024867719,33.2238507313754));
#17372=CARTESIAN_POINT('Ctrl Pts',(18.7880213595606,67.2727761646991,33.1868063587115));
#17373=CARTESIAN_POINT('Ctrl Pts',(19.3128164190146,67.6176001101629,33.1497619860477));
#17374=CARTESIAN_POINT('Ctrl Pts',(19.8623822062184,67.6630760996231,33.1127176133838));
#17375=CARTESIAN_POINT('Ctrl Pts',(20.4119479934222,67.7085520890833,33.07567324072));
#17376=CARTESIAN_POINT('Ctrl Pts',(20.9862845083758,67.4546801225399,33.0386288680561));
#17377=CARTESIAN_POINT('Ctrl Pts',(21.3225640589931,67.0176370080482,33.0015844953923));
#17378=CARTESIAN_POINT('Ctrl Pts',(21.6588436096103,66.5805938935566,32.9645401227284));
#17379=CARTESIAN_POINT('Ctrl Pts',(21.7570661958914,65.9603796311168,32.9274957500646));
#17380=CARTESIAN_POINT('Ctrl Pts',(21.5722832293577,65.4408164729121,32.8904513774007));
#17381=CARTESIAN_POINT('Ctrl Pts',(21.387500262824,64.9212533147075,32.8534070047369));
#17382=CARTESIAN_POINT('Ctrl Pts',(20.9197117434757,64.5023412607381,32.816362632073));
#17383=CARTESIAN_POINT('Ctrl Pts',(20.382986903752,64.3757827110126,32.7793182594091));
#17384=CARTESIAN_POINT('Ctrl Pts',(19.8462620640284,64.2492241612871,32.7422738867453));
#17385=CARTESIAN_POINT('Ctrl Pts',(19.2406009039295,64.4150191158055,32.7052295140814));
#17386=CARTESIAN_POINT('Ctrl Pts',(18.8431658896135,64.7972965405656,32.6681851414176));
#17387=CARTESIAN_POINT('Ctrl Pts',(18.5225034999409,65.1057293361823,32.638296639815));
#17388=CARTESIAN_POINT('Ctrl Pts',(18.337390965392,65.555086641388,32.6084081382124));
#17389=CARTESIAN_POINT('Ctrl Pts',(18.3333052932669,66.0014544402739,32.5785196366098));
#17390=CARTESIAN_POINT('Ctrl Pts',(18.3314318999871,65.9994875421513,32.7714803633902));
#17391=CARTESIAN_POINT('Ctrl Pts',(18.3313183609503,65.9713977596598,32.7733667683417));
#17392=CARTESIAN_POINT('Ctrl Pts',(18.3319662848669,65.9433133244466,32.7752531732933));
#17393=CARTESIAN_POINT('Ctrl Pts',(18.3333921073574,65.9152684381647,32.7771395782448));
#17394=CARTESIAN_POINT('Ctrl Pts',(18.3613917686438,65.3645355650877,32.8141839509086));
#17395=CARTESIAN_POINT('Ctrl Pts',(18.6893750964734,64.82905408059,32.8512283235725));
#17396=CARTESIAN_POINT('Ctrl Pts',(19.167250465381,64.5538708501677,32.8882726962364));
#17397=CARTESIAN_POINT('Ctrl Pts',(19.6451258342887,64.2786876197455,32.9253170689002));
#17398=CARTESIAN_POINT('Ctrl Pts',(20.2728932442745,64.2638026433987,32.9623614415641));
#17399=CARTESIAN_POINT('Ctrl Pts',(20.763273974189,64.5160275792031,32.9994058142279));
#17400=CARTESIAN_POINT('Ctrl Pts',(21.2536547041036,64.7682525150074,33.0364501868918));
#17401=CARTESIAN_POINT('Ctrl Pts',(21.6066487539469,65.2875873629629,33.0734945595556));
#17402=CARTESIAN_POINT('Ctrl Pts',(21.6607190996507,65.8363742763029,33.1105389322195));
#17403=CARTESIAN_POINT('Ctrl Pts',(21.7147894453546,66.3851611896429,33.1475833048833));
#17404=CARTESIAN_POINT('Ctrl Pts',(21.4699360869189,66.9634001683674,33.1846276775472));
#17405=CARTESIAN_POINT('Ctrl Pts',(21.0382087398405,67.3064776760442,33.221672050211));
#17406=CARTESIAN_POINT('Ctrl Pts',(20.6064813927622,67.649555183721,33.2587164228749));
#17407=CARTESIAN_POINT('Ctrl Pts',(19.9878800570411,67.75747122035,33.2957607955387));
#17408=CARTESIAN_POINT('Ctrl Pts',(19.46548887784,67.5808412840736,33.3328051682026));
#17409=CARTESIAN_POINT('Ctrl Pts',(18.9430976986389,67.4042113477973,33.3698495408664));
#17410=CARTESIAN_POINT('Ctrl Pts',(18.5169166759577,66.9430354386155,33.4068939135303));
#17411=CARTESIAN_POINT('Ctrl Pts',(18.3819746329741,66.4083567278835,33.4439382861942));
#17412=CARTESIAN_POINT('Ctrl Pts',(18.3485319992028,66.2758475119791,33.4531189785928));
#17413=CARTESIAN_POINT('Ctrl Pts',(18.3329771223643,66.1388237896396,33.4622996709915));
#17414=CARTESIAN_POINT('Ctrl Pts',(18.3342212861325,66.001521965989,33.4714803633902));
#17415=CARTESIAN_POINT('Origin',(20.,66.,30.));
#17416=CARTESIAN_POINT('',(18.3366059400397,65.999580177369,34.1714803633902));
#17417=CARTESIAN_POINT('',(18.3335757493505,65.9985070366392,33.9785196366098));
#17418=CARTESIAN_POINT('',(18.334,66.,30.));
#17419=CARTESIAN_POINT('Ctrl Pts',(18.3335757493505,65.9985070366392,33.9785196366098));
#17420=CARTESIAN_POINT('Ctrl Pts',(18.3376145958483,66.4361202143717,33.9492295708481));
#17421=CARTESIAN_POINT('Ctrl Pts',(18.5146051520986,66.8766244384234,33.9199395050864));
#17422=CARTESIAN_POINT('Ctrl Pts',(18.8239357934279,67.1839061408327,33.8906494393247));
#17423=CARTESIAN_POINT('Ctrl Pts',(19.2151592084583,67.5725381770135,33.8536050666609));
#17424=CARTESIAN_POINT('Ctrl Pts',(19.8180701191298,67.7480711967276,33.816560693997));
#17425=CARTESIAN_POINT('Ctrl Pts',(20.3567646288979,67.6301778340091,33.7795163213331));
#17426=CARTESIAN_POINT('Ctrl Pts',(20.895459138666,67.5122844712905,33.7424719486693));
#17427=CARTESIAN_POINT('Ctrl Pts',(21.3699372475307,67.1009647261393,33.7054275760055));
#17428=CARTESIAN_POINT('Ctrl Pts',(21.5630684345601,66.5844466094772,33.6683832033416));
#17429=CARTESIAN_POINT('Ctrl Pts',(21.7561996215896,66.0679284928152,33.6313388306778));
#17430=CARTESIAN_POINT('Ctrl Pts',(21.6679838867839,65.4462120046424,33.5942944580139));
#17431=CARTESIAN_POINT('Ctrl Pts',(21.3387904867984,65.0038068447832,33.55725008535));
#17432=CARTESIAN_POINT('Ctrl Pts',(21.009597086813,64.5614016849239,33.5202057126862));
#17433=CARTESIAN_POINT('Ctrl Pts',(20.4394260216479,64.2983078533782,33.4831613400223));
#17434=CARTESIAN_POINT('Ctrl Pts',(19.8891987914095,64.3349222653105,33.4461169673585));
#17435=CARTESIAN_POINT('Ctrl Pts',(19.3389715611711,64.3715366772429,33.4090725946947));
#17436=CARTESIAN_POINT('Ctrl Pts',(18.8086881658594,64.7078593326534,33.3720282220308));
#17437=CARTESIAN_POINT('Ctrl Pts',(18.54101672313,65.1899823655538,33.3349838493669));
#17438=CARTESIAN_POINT('Ctrl Pts',(18.4050189434904,65.4349381266877,33.3161624451146));
#17439=CARTESIAN_POINT('Ctrl Pts',(18.3368124767972,65.7175311656414,33.2973410408622));
#17440=CARTESIAN_POINT('Ctrl Pts',(18.3367009922703,66.0000736897305,33.2785196366098));
#17441=CARTESIAN_POINT('Ctrl Pts',(18.3342212861325,66.001521965989,33.4714803633902));
#17442=CARTESIAN_POINT('Ctrl Pts',(18.3379973609565,65.5848067610909,33.4993440436554));
#17443=CARTESIAN_POINT('Ctrl Pts',(18.4965162756366,65.1655298511734,33.5272077239205));
#17444=CARTESIAN_POINT('Ctrl Pts',(18.779340888906,64.8621280210291,33.5550714041857));
#17445=CARTESIAN_POINT('Ctrl Pts',(19.1553522511079,64.4587595371892,33.5921157768496));
#17446=CARTESIAN_POINT('Ctrl Pts',(19.7510780387978,64.2602040817917,33.6291601495134));
#17447=CARTESIAN_POINT('Ctrl Pts',(20.29390240791,64.3573245366126,33.6662045221773));
#17448=CARTESIAN_POINT('Ctrl Pts',(20.8367267770223,64.4544449914334,33.7032488948411));
#17449=CARTESIAN_POINT('Ctrl Pts',(21.3266497275569,64.8472413564726,33.740293267505));
#17450=CARTESIAN_POINT('Ctrl Pts',(21.5394728754595,65.3559622892128,33.7773376401688));
#17451=CARTESIAN_POINT('Ctrl Pts',(21.7522960233621,65.864683221953,33.8143820128327));
#17452=CARTESIAN_POINT('Ctrl Pts',(21.6880193686326,66.4893287223942,33.8514263854965));
#17453=CARTESIAN_POINT('Ctrl Pts',(21.3760571740258,66.944048708093,33.8884707581604));
#17454=CARTESIAN_POINT('Ctrl Pts',(21.0640949794191,67.3987686937919,33.9255151308242));
#17455=CARTESIAN_POINT('Ctrl Pts',(20.5044472449351,67.6835631647483,33.9625595034881));
#17456=CARTESIAN_POINT('Ctrl Pts',(19.9532197864407,67.6681045833766,33.9996038761519));
#17457=CARTESIAN_POINT('Ctrl Pts',(19.4019923279463,67.6526460020049,34.0366482488158));
#17458=CARTESIAN_POINT('Ctrl Pts',(18.8591851454414,67.3369343683051,34.0736926214796));
#17459=CARTESIAN_POINT('Ctrl Pts',(18.5731974903607,66.8654455050557,34.1107369941435));
#17460=CARTESIAN_POINT('Ctrl Pts',(18.4168817669606,66.607738148026,34.1309847838924));
#17461=CARTESIAN_POINT('Ctrl Pts',(18.337291379463,66.3034920391225,34.1512325736413));
#17462=CARTESIAN_POINT('Ctrl Pts',(18.3366059400397,65.999580177369,34.1714803633902));
#17463=CARTESIAN_POINT('Origin',(20.,66.,30.));
#17464=CARTESIAN_POINT('',(18.332682423241,65.9986976781594,34.8714803633902));
#17465=CARTESIAN_POINT('',(18.3317911471719,66.0008588710395,34.6785196366098));
#17466=CARTESIAN_POINT('',(18.334,66.,30.));
#17467=CARTESIAN_POINT('Ctrl Pts',(18.3317911471719,66.0008588710395,34.6785196366098));
#17468=CARTESIAN_POINT('Ctrl Pts',(18.3314810976279,66.050216623889,34.6752068461617));
#17469=CARTESIAN_POINT('Ctrl Pts',(18.3334818189716,66.0995488884736,34.6718940557137));
#17470=CARTESIAN_POINT('Ctrl Pts',(18.3378751477734,66.1486671473684,34.6685812652656));
#17471=CARTESIAN_POINT('Ctrl Pts',(18.3870023448957,66.6979186365989,34.6315368926018));
#17472=CARTESIAN_POINT('Ctrl Pts',(18.73530640953,67.220410386499,34.594492519938));
#17473=CARTESIAN_POINT('Ctrl Pts',(19.2233963781913,67.4770401011375,34.5574481472741));
#17474=CARTESIAN_POINT('Ctrl Pts',(19.7114863468526,67.7336698157761,34.5204037746102));
#17475=CARTESIAN_POINT('Ctrl Pts',(20.3393622195409,67.7244374951531,34.4833594019464));
#17476=CARTESIAN_POINT('Ctrl Pts',(20.8196957251835,67.4535679248572,34.4463150292825));
#17477=CARTESIAN_POINT('Ctrl Pts',(21.300029230826,67.1826983545613,34.4092706566187));
#17478=CARTESIAN_POINT('Ctrl Pts',(21.6328203694228,66.6501915345925,34.3722262839548));
#17479=CARTESIAN_POINT('Ctrl Pts',(21.6657773241773,66.0997331185797,34.335181911291));
#17480=CARTESIAN_POINT('Ctrl Pts',(21.6987342789318,65.5492747025669,34.2981375386271));
#17481=CARTESIAN_POINT('Ctrl Pts',(21.4318570498441,64.9808646905101,34.2610931659632));
#17482=CARTESIAN_POINT('Ctrl Pts',(20.9872739303598,64.6546186634519,34.2240487932994));
#17483=CARTESIAN_POINT('Ctrl Pts',(20.5426908108755,64.3283726363937,34.1870044206355));
#17484=CARTESIAN_POINT('Ctrl Pts',(19.9204018009947,64.2442905943341,34.1499600479717));
#17485=CARTESIAN_POINT('Ctrl Pts',(19.4051785874718,64.440850147818,34.1129156753078));
#17486=CARTESIAN_POINT('Ctrl Pts',(18.8899553739489,64.6374097013019,34.075871302644));
#17487=CARTESIAN_POINT('Ctrl Pts',(18.481797956784,65.1146108503293,34.0388269299801));
#17488=CARTESIAN_POINT('Ctrl Pts',(18.3674872078961,65.6540769511668,34.0017825573163));
#17489=CARTESIAN_POINT('Ctrl Pts',(18.3435591301517,65.7670005994404,33.9940282504141));
#17490=CARTESIAN_POINT('Ctrl Pts',(18.3325064975594,65.8826525038369,33.986273943512));
#17491=CARTESIAN_POINT('Ctrl Pts',(18.3335757493505,65.9985070366392,33.9785196366098));
#17492=CARTESIAN_POINT('Ctrl Pts',(18.3366059400397,65.999580177369,34.1714803633902));
#17493=CARTESIAN_POINT('Ctrl Pts',(18.3360373327868,65.7474696582416,34.1882769463052));
#17494=CARTESIAN_POINT('Ctrl Pts',(18.3897676052821,65.4955891531532,34.2050735292201));
#17495=CARTESIAN_POINT('Ctrl Pts',(18.4990410118861,65.2706966028902,34.2218701121351));
#17496=CARTESIAN_POINT('Ctrl Pts',(18.7400403161485,64.7747026567731,34.2589144847989));
#17497=CARTESIAN_POINT('Ctrl Pts',(19.2512070523296,64.4099808573381,34.2959588574628));
#17498=CARTESIAN_POINT('Ctrl Pts',(19.7986212717497,64.3434349426867,34.3330032301266));
#17499=CARTESIAN_POINT('Ctrl Pts',(20.3460354911699,64.2768890280352,34.3700476027905));
#17500=CARTESIAN_POINT('Ctrl Pts',(20.929697193829,64.5085189981672,34.4070919754543));
#17501=CARTESIAN_POINT('Ctrl Pts',(21.2825112793764,64.932326689458,34.4441363481182));
#17502=CARTESIAN_POINT('Ctrl Pts',(21.6353253649239,65.3561343807487,34.481180720782));
#17503=CARTESIAN_POINT('Ctrl Pts',(21.7572918333596,65.9721197931981,34.5182250934459));
#17504=CARTESIAN_POINT('Ctrl Pts',(21.5925964660647,66.498395342926,34.5552694661097));
#17505=CARTESIAN_POINT('Ctrl Pts',(21.4279010987698,67.0246708926539,34.5923138387736));
#17506=CARTESIAN_POINT('Ctrl Pts',(20.9765438957441,67.4612365796603,34.6293582114374));
#17507=CARTESIAN_POINT('Ctrl Pts',(20.4450747207132,67.6083124241619,34.6664025841013));
#17508=CARTESIAN_POINT('Ctrl Pts',(19.9136055456824,67.7553882686635,34.7034469567651));
#17509=CARTESIAN_POINT('Ctrl Pts',(19.3020243986463,67.6129742706603,34.740491329429));
#17510=CARTESIAN_POINT('Ctrl Pts',(18.8902029978432,67.2462397444944,34.7775357020928));
#17511=CARTESIAN_POINT('Ctrl Pts',(18.5420761503954,66.9362263887159,34.808850589192));
#17512=CARTESIAN_POINT('Ctrl Pts',(18.3366957110857,66.465915724442,34.8401654762911));
#17513=CARTESIAN_POINT('Ctrl Pts',(18.332682423241,65.9986976781594,34.8714803633902));
#17514=CARTESIAN_POINT('Origin',(20.,66.,30.));
#17515=CARTESIAN_POINT('',(18.3325226254757,66.0012132166996,35.5714803633902));
#17516=CARTESIAN_POINT('',(18.3361559304958,66.0009441564151,35.3785196366098));
#17517=CARTESIAN_POINT('',(18.334,66.,30.));
#17518=CARTESIAN_POINT('',(21.2690708798523,67.0793586530486,36.));
#17519=CARTESIAN_POINT('Ctrl Pts',(18.3325226254757,66.0012132166996,35.5714803633902));
#17520=CARTESIAN_POINT('Ctrl Pts',(18.3364573202891,65.5283746677229,35.6031871242686));
#17521=CARTESIAN_POINT('Ctrl Pts',(18.5476201467709,65.0525511517719,35.6348938851469));
#17522=CARTESIAN_POINT('Ctrl Pts',(18.9034043931841,64.742267480559,35.6666006460253));
#17523=CARTESIAN_POINT('Ctrl Pts',(19.3190824330385,64.3797497200092,35.7036450186892));
#17524=CARTESIAN_POINT('Ctrl Pts',(19.9321723852594,64.2431980531274,35.7406893913531));
#17525=CARTESIAN_POINT('Ctrl Pts',(20.4620470219442,64.396190694787,35.7777337640169));
#17526=CARTESIAN_POINT('Ctrl Pts',(20.991921658629,64.5491833364465,35.8147781366808));
#17527=CARTESIAN_POINT('Ctrl Pts',(21.4385809797777,64.9917202866474,35.8518225093446));
#17528=CARTESIAN_POINT('Ctrl Pts',(21.5975925396924,65.518769581225,35.8888668820084));
#17529=CARTESIAN_POINT('Ctrl Pts',(21.7566040996072,66.0458188758026,35.9259112546723));
#17530=CARTESIAN_POINT('Ctrl Pts',(21.627967898288,66.6573805147569,35.9629556273362));
#17531=CARTESIAN_POINT('Ctrl Pts',(21.2690708798523,67.0793586530486,36.));
#17532=CARTESIAN_POINT('',(18.7285278825024,67.0812050123663,36.));
#17533=CARTESIAN_POINT('Origin',(20.,66.,36.));
#17534=CARTESIAN_POINT('Ctrl Pts',(18.7285264260868,67.0812061322332,36.));
#17535=CARTESIAN_POINT('Ctrl Pts',(19.0793427026358,67.4926761270889,35.9636818543909));
#17536=CARTESIAN_POINT('Ctrl Pts',(19.6492096450092,67.7187174715531,35.9273637087819));
#17537=CARTESIAN_POINT('Ctrl Pts',(20.1865491476251,67.6581952048996,35.8910455631728));
#17538=CARTESIAN_POINT('Ctrl Pts',(20.7346334302361,67.596462719312,35.8540011905089));
#17539=CARTESIAN_POINT('Ctrl Pts',(21.2488764127446,67.2365916395225,35.8169568178451));
#17540=CARTESIAN_POINT('Ctrl Pts',(21.4942849783746,66.7428459429767,35.7799124451812));
#17541=CARTESIAN_POINT('Ctrl Pts',(21.7396935440046,66.249100246431,35.7428680725174));
#17542=CARTESIAN_POINT('Ctrl Pts',(21.7162676927562,65.6214799331291,35.7058236998535));
#17543=CARTESIAN_POINT('Ctrl Pts',(21.4345599518354,65.1474062012195,35.6687793271897));
#17544=CARTESIAN_POINT('Ctrl Pts',(21.1528522109146,64.6733324693098,35.6317349545258));
#17545=CARTESIAN_POINT('Ctrl Pts',(20.6128625803214,64.3528053187923,35.594690581862));
#17546=CARTESIAN_POINT('Ctrl Pts',(20.0617849940283,64.3323991219251,35.5576462091981));
#17547=CARTESIAN_POINT('Ctrl Pts',(19.5107074077351,64.3119929250578,35.5206018365343));
#17548=CARTESIAN_POINT('Ctrl Pts',(18.948541865742,64.5917076818407,35.4835574638704));
#17549=CARTESIAN_POINT('Ctrl Pts',(18.6325042241011,65.0435931575014,35.4465130912065));
#17550=CARTESIAN_POINT('Ctrl Pts',(18.4391461016429,65.32006568997,35.423848606341));
#17551=CARTESIAN_POINT('Ctrl Pts',(18.3379194624106,65.6609857867967,35.4011841214754));
#17552=CARTESIAN_POINT('Ctrl Pts',(18.3361559304958,66.0009441564151,35.3785196366098));
#17553=CARTESIAN_POINT('Origin',(20.,66.,37.5459252805377));
#17554=CARTESIAN_POINT('',(17.9445921240961,66.0018230781907,25.3540747194623));
#17555=CARTESIAN_POINT('',(17.9470733212015,65.9984939638888,25.2959252805377));
#17556=CARTESIAN_POINT('',(17.94525,66.0000000000002,37.5459252805377));
#17557=CARTESIAN_POINT('',(21.8174278887594,66.9586205879593,25.));
#17558=CARTESIAN_POINT('Ctrl Pts',(17.9470733212015,65.9984939638888,25.2959252805377));
#17559=CARTESIAN_POINT('Ctrl Pts',(17.9500635365654,66.4524190943363,25.2713722656862));
#17560=CARTESIAN_POINT('Ctrl Pts',(18.3216914342811,67.5959824757237,25.2097748781708));
#17561=CARTESIAN_POINT('Ctrl Pts',(20.2159933450493,68.4179588201339,25.1111331179916));
#17562=CARTESIAN_POINT('Ctrl Pts',(21.4986774253635,67.5629326473988,25.0370443726639));
#17563=CARTESIAN_POINT('Ctrl Pts',(21.8174278887594,66.9586205879593,25.));
#17564=CARTESIAN_POINT('',(22.0570978955383,65.924544719602,25.));
#17565=CARTESIAN_POINT('Origin',(20.,66.,25.));
#17566=CARTESIAN_POINT('Ctrl Pts',(17.9445921240961,66.0018230781907,25.3540747194623));
#17567=CARTESIAN_POINT('Ctrl Pts',(17.9432975429406,66.1421866078242,25.3464567039116));
#17568=CARTESIAN_POINT('Ctrl Pts',(18.0204258713679,66.9636910465588,25.3017943156971));
#17569=CARTESIAN_POINT('Ctrl Pts',(19.1263753077513,68.2659593106943,25.2200875548188));
#17570=CARTESIAN_POINT('Ctrl Pts',(21.4138495931967,67.965112977645,25.109680663882));
#17571=CARTESIAN_POINT('Ctrl Pts',(22.080681931349,66.5910225805,25.0363181456091));
#17572=CARTESIAN_POINT('Ctrl Pts',(22.0571001530702,65.9245445252813,25.));
#17573=CARTESIAN_POINT('Origin',(20.,66.,37.5459252805377));
#17574=CARTESIAN_POINT('',(17.9485832333138,65.9999504083724,26.0540747194623));
#17575=CARTESIAN_POINT('',(17.9419860794096,65.9995169087598,25.9959252805377));
#17576=CARTESIAN_POINT('',(17.94525,66.0000000000002,37.5459252805377));
#17577=CARTESIAN_POINT('Ctrl Pts',(17.9419860794096,65.9995169087598,25.9959252805377));
#17578=CARTESIAN_POINT('Ctrl Pts',(17.9440551104146,66.6536075979329,25.9603051683359));
#17579=CARTESIAN_POINT('Ctrl Pts',(18.6350687743765,67.991716020834,25.8876406834704));
#17580=CARTESIAN_POINT('Ctrl Pts',(20.9141747100121,68.249987107151,25.7779318259409));
#17581=CARTESIAN_POINT('Ctrl Pts',(22.3860297127563,66.4524069399739,25.6667987079494));
#17582=CARTESIAN_POINT('Ctrl Pts',(21.6743955698345,64.2406214035846,25.5556655899578));
#17583=CARTESIAN_POINT('Ctrl Pts',(19.4296920915163,63.6393770033003,25.4445324719662));
#17584=CARTESIAN_POINT('Ctrl Pts',(18.0884941577881,64.8537199906368,25.3579523688262));
#17585=CARTESIAN_POINT('Ctrl Pts',(17.9455520477338,65.7675593410441,25.30841663835));
#17586=CARTESIAN_POINT('Ctrl Pts',(17.9470733212015,65.9984939638888,25.2959252805377));
#17587=CARTESIAN_POINT('Ctrl Pts',(17.9485832333138,65.9999504083724,26.0540747194623));
#17588=CARTESIAN_POINT('Ctrl Pts',(17.948657249995,66.3458999876025,26.0353896065614));
#17589=CARTESIAN_POINT('Ctrl Pts',(18.1957459993379,67.3778154487128,25.9796601209967));
#17590=CARTESIAN_POINT('Ctrl Pts',(19.8298599336245,68.4226484781515,25.8868862627681));
#17591=CARTESIAN_POINT('Ctrl Pts',(21.9430509921809,67.4569397340099,25.7757531447766));
#17592=CARTESIAN_POINT('Ctrl Pts',(22.2779267956692,65.1577888874642,25.664620026785));
#17593=CARTESIAN_POINT('Ctrl Pts',(20.5278716209092,63.6294498681163,25.5534869087934));
#17594=CARTESIAN_POINT('Ctrl Pts',(18.4479227214906,64.22679670444,25.4499718063526));
#17595=CARTESIAN_POINT('Ctrl Pts',(17.9495927449455,65.459636294612,25.3835010765755));
#17596=CARTESIAN_POINT('Ctrl Pts',(17.9445921240961,66.0018230781907,25.3540747194623));
#17597=CARTESIAN_POINT('Origin',(20.,66.,37.5459252805377));
#17598=CARTESIAN_POINT('',(17.9444688311789,65.998193668761,26.7540747194623));
#17599=CARTESIAN_POINT('',(17.9457761896405,66.0018654840515,26.6959252805377));
#17600=CARTESIAN_POINT('',(17.94525,66.0000000000002,37.5459252805377));
#17601=CARTESIAN_POINT('Ctrl Pts',(17.9457761896405,66.0018654840515,26.6959252805377));
#17602=CARTESIAN_POINT('Ctrl Pts',(17.9441910723939,66.1797860150858,26.6862824436496));
#17603=CARTESIAN_POINT('Ctrl Pts',(18.0468091346947,67.0394145421733,26.6395952340976));
#17604=CARTESIAN_POINT('Ctrl Pts',(19.2507940995179,68.310165311319,26.5558636518818));
#17605=CARTESIAN_POINT('Ctrl Pts',(21.5344924689199,67.8824201691326,26.4447305338903));
#17606=CARTESIAN_POINT('Ctrl Pts',(22.4137605469628,65.7318111515436,26.3335974158987));
#17607=CARTESIAN_POINT('Ctrl Pts',(21.0838647269646,63.8266568213479,26.2224642979072));
#17608=CARTESIAN_POINT('Ctrl Pts',(18.7619637584228,63.9106363014535,26.1113311799156));
#17609=CARTESIAN_POINT('Ctrl Pts',(17.9542068529918,65.2670451819344,26.0358181741258));
#17610=CARTESIAN_POINT('Ctrl Pts',(17.9419033497697,65.9733632711195,25.9973495409998));
#17611=CARTESIAN_POINT('Ctrl Pts',(17.9419860794096,65.9995169087598,25.9959252805377));
#17612=CARTESIAN_POINT('Ctrl Pts',(17.9444688311789,65.998193668761,26.7540747194623));
#17613=CARTESIAN_POINT('Ctrl Pts',(17.9494992489566,66.5462599810788,26.7243225092112));
#17614=CARTESIAN_POINT('Ctrl Pts',(18.4568949548124,67.7849444524044,26.6575259262962));
#17615=CARTESIAN_POINT('Ctrl Pts',(20.5486976409782,68.3658195058375,26.5536849707175));
#17616=CARTESIAN_POINT('Ctrl Pts',(22.2852057779767,66.8221949443221,26.4425518527259));
#17617=CARTESIAN_POINT('Ctrl Pts',(21.9302043029995,64.5260653118046,26.3314187347344));
#17618=CARTESIAN_POINT('Ctrl Pts',(19.8086025603331,63.5789385134492,26.2202856167428));
#17619=CARTESIAN_POINT('Ctrl Pts',(18.1894355754228,64.6343488156836,26.1278376116521));
#17620=CARTESIAN_POINT('Ctrl Pts',(17.9485105074231,65.6600339078047,26.0724339792253));
#17621=CARTESIAN_POINT('Ctrl Pts',(17.9485832333138,65.9999504083724,26.0540747194623));
#17622=CARTESIAN_POINT('Origin',(20.,66.,37.5459252805377));
#17623=CARTESIAN_POINT('',(17.9427073334353,66.0011828701398,27.4540747194623));
#17624=CARTESIAN_POINT('',(17.9483912883566,65.9993486074671,27.3959252805377));
#17625=CARTESIAN_POINT('',(17.94525,66.0000000000002,37.5459252805377));
#17626=CARTESIAN_POINT('Ctrl Pts',(17.9483912883566,65.999348607467,27.3959252805377));
#17627=CARTESIAN_POINT('Ctrl Pts',(17.9494813165331,66.3826975665212,27.3752153462993));
#17628=CARTESIAN_POINT('Ctrl Pts',(18.2366610493634,67.453268789384,27.3174610393972));
#17629=CARTESIAN_POINT('Ctrl Pts',(19.9621345909966,68.4283200411723,27.2226623598312));
#17630=CARTESIAN_POINT('Ctrl Pts',(22.0195745485331,67.3488849730689,27.1115292418396));
#17631=CARTESIAN_POINT('Ctrl Pts',(22.2286203516014,65.0348973043881,27.0003961238481));
#17632=CARTESIAN_POINT('Ctrl Pts',(20.3979451669564,63.6042095721724,26.8892630058565));
#17633=CARTESIAN_POINT('Ctrl Pts',(18.3935017636324,64.300123176515,26.787772724753));
#17634=CARTESIAN_POINT('Ctrl Pts',(17.9502805328587,65.496278191333,26.7233268163134));
#17635=CARTESIAN_POINT('Ctrl Pts',(17.9457761896405,66.0018654840515,26.6959252805377));
#17636=CARTESIAN_POINT('Ctrl Pts',(17.9427073334353,66.0011828701398,27.4540747194623));
#17637=CARTESIAN_POINT('Ctrl Pts',(17.9422311397102,66.0705663093613,27.4502997845249));
#17638=CARTESIAN_POINT('Ctrl Pts',(17.9768968009426,66.8203451915429,27.4094804769235));
#17639=CARTESIAN_POINT('Ctrl Pts',(18.8966146610587,68.1634952415589,27.3316167966584));
#17640=CARTESIAN_POINT('Ctrl Pts',(21.2191694244532,68.1004277622309,27.2204836786668));
#17641=CARTESIAN_POINT('Ctrl Pts',(22.4258923392674,66.1149661220525,27.1093505606753));
#17642=CARTESIAN_POINT('Ctrl Pts',(21.4123431135179,64.0242829635948,26.9982174426837));
#17643=CARTESIAN_POINT('Ctrl Pts',(19.1061618600091,63.7418537970392,26.8870843246921));
#17644=CARTESIAN_POINT('Ctrl Pts',(18.0164474023229,65.0484776654923,26.8057034169517));
#17645=CARTESIAN_POINT('Ctrl Pts',(17.9432358934196,65.8638645372895,26.7613668818751));
#17646=CARTESIAN_POINT('Ctrl Pts',(17.9444688311789,65.998193668761,26.7540747194623));
#17647=CARTESIAN_POINT('Origin',(20.,66.,37.5459252805377));
#17648=CARTESIAN_POINT('',(17.9480453685107,66.0010551247654,28.1540747194623));
#17649=CARTESIAN_POINT('',(17.9433900326703,65.9984792506554,28.0959252805377));
#17650=CARTESIAN_POINT('',(17.94525,66.0000000000002,37.5459252805377));
#17651=CARTESIAN_POINT('Ctrl Pts',(17.9433900326703,65.9984792506554,28.0959252805377));
#17652=CARTESIAN_POINT('Ctrl Pts',(17.9482331665523,66.5830501664587,28.0641482489491));
#17653=CARTESIAN_POINT('Ctrl Pts',(18.5151173418414,67.8573001141241,27.9953268446968));
#17654=CARTESIAN_POINT('Ctrl Pts',(20.6768128607374,68.3324014127664,27.8894610677805));
#17655=CARTESIAN_POINT('Ctrl Pts',(22.3266175536682,66.6964357531696,27.778327949789));
#17656=CARTESIAN_POINT('Ctrl Pts',(21.8470102861031,64.4230646811199,27.6671948317974));
#17657=CARTESIAN_POINT('Ctrl Pts',(19.6769465082846,63.592966879896,27.5560617138059));
#17658=CARTESIAN_POINT('Ctrl Pts',(18.1518517268107,64.7100346416723,27.4656385300526));
#17659=CARTESIAN_POINT('Ctrl Pts',(17.9475315561177,65.6969917822298,27.4122597189632));
#17660=CARTESIAN_POINT('Ctrl Pts',(17.9483912883566,65.999348607467,27.3959252805377));
#17661=CARTESIAN_POINT('Ctrl Pts',(17.9480453685107,66.0010551247654,28.1540747194623));
#17662=CARTESIAN_POINT('Ctrl Pts',(17.9467675578732,66.2756710572213,28.1392326871747));
#17663=CARTESIAN_POINT('Ctrl Pts',(18.1259278433178,67.2341046560269,28.0873462822231));
#17664=CARTESIAN_POINT('Ctrl Pts',(19.5805009712835,68.3921102462499,27.9984155046077));
#17665=CARTESIAN_POINT('Ctrl Pts',(21.7821629259284,67.6498685313834,27.8872823866162));
#17666=CARTESIAN_POINT('Ctrl Pts',(22.3527192254304,65.3976021983889,27.7761492686246));
#17667=CARTESIAN_POINT('Ctrl Pts',(20.7699742878597,63.6966740436017,27.6650161506331));
#17668=CARTESIAN_POINT('Ctrl Pts',(18.5602181548524,64.0900099607333,27.557657967579));
#17669=CARTESIAN_POINT('Ctrl Pts',(17.9469041468234,65.3896894143134,27.4873441571887));
#17670=CARTESIAN_POINT('Ctrl Pts',(17.9427073334353,66.0011828701398,27.4540747194623));
#17671=CARTESIAN_POINT('Origin',(20.,66.,37.5459252805377));
#17672=CARTESIAN_POINT('',(17.9465562858968,65.9982462861091,28.8540747194623));
#17673=CARTESIAN_POINT('',(17.943661294952,66.0016161416468,28.7959252805377));
#17674=CARTESIAN_POINT('',(17.94525,66.0000000000002,37.5459252805377));
#17675=CARTESIAN_POINT('Ctrl Pts',(17.943661294952,66.0016161416468,28.7959252805377));
#17676=CARTESIAN_POINT('Ctrl Pts',(17.9427401513473,66.1083451948514,28.7901255242628));
#17677=CARTESIAN_POINT('Ctrl Pts',(17.9988247250069,66.8958068468452,28.747281395324));
#17678=CARTESIAN_POINT('Ctrl Pts',(19.0161588257614,68.2204117957101,28.6673928937215));
#17679=CARTESIAN_POINT('Ctrl Pts',(21.3318253046188,68.0308651744107,28.5562597757299));
#17680=CARTESIAN_POINT('Ctrl Pts',(22.4285528445608,65.982590811414,28.4451266577383));
#17681=CARTESIAN_POINT('Ctrl Pts',(21.3025732342425,63.9502500230349,28.3339935397468));
#17682=CARTESIAN_POINT('Ctrl Pts',(18.9844273311818,63.7939210909379,28.2228604217552));
#17683=CARTESIAN_POINT('Ctrl Pts',(17.9928405311673,65.1240506743191,28.1435043353522));
#17684=CARTESIAN_POINT('Ctrl Pts',(17.9425872377976,65.9015811377,28.101192621613));
#17685=CARTESIAN_POINT('Ctrl Pts',(17.9433900326703,65.9984792506554,28.0959252805377));
#17686=CARTESIAN_POINT('Ctrl Pts',(17.9465562858968,65.9982462861091,28.8540747194623));
#17687=CARTESIAN_POINT('Ctrl Pts',(17.9504440293497,66.476757915502,28.8281655898244));
#17688=CARTESIAN_POINT('Ctrl Pts',(18.3555440463461,67.6453698738043,28.7652120875227));
#17689=CARTESIAN_POINT('Ctrl Pts',(20.301369074849,68.4098438841618,28.6652142125571));
#17690=CARTESIAN_POINT('Ctrl Pts',(22.1880462145232,67.053861769123,28.5540810945655));
#17691=CARTESIAN_POINT('Ctrl Pts',(22.0721373380047,64.7333438833879,28.442947976574));
#17692=CARTESIAN_POINT('Ctrl Pts',(20.059726811216,63.5721195306752,28.3318148585824));
#17693=CARTESIAN_POINT('Ctrl Pts',(18.2687136043545,64.4913061498983,28.2355237728786));
#17694=CARTESIAN_POINT('Ctrl Pts',(17.9499568578648,65.5902544819065,28.1762770598385));
#17695=CARTESIAN_POINT('Ctrl Pts',(17.9480453685107,66.0010551247654,28.1540747194623));
#17696=CARTESIAN_POINT('Origin',(20.,66.,37.5459252805377));
#17697=CARTESIAN_POINT('',(17.9418458735908,65.9999766228671,29.5540747194623));
#17698=CARTESIAN_POINT('',(17.9484736033439,66.000497180875,29.4959252805377));
#17699=CARTESIAN_POINT('',(17.94525,66.0000000000002,37.5459252805377));
#17700=CARTESIAN_POINT('Ctrl Pts',(17.9484736033439,66.000497180875,29.4959252805377));
#17701=CARTESIAN_POINT('Ctrl Pts',(17.94779755434,66.312740496662,29.4790584269126));
#17702=CARTESIAN_POINT('Ctrl Pts',(18.1614618714719,67.3098805675566,29.4251472006236));
#17703=CARTESIAN_POINT('Ctrl Pts',(19.7114877817388,68.4114171556518,29.3341916016708));
#17704=CARTESIAN_POINT('Ctrl Pts',(21.8694279673096,67.5502938668842,29.2230584836792));
#17705=CARTESIAN_POINT('Ctrl Pts',(22.316394097231,65.2702806121721,29.1119253656877));
#17706=CARTESIAN_POINT('Ctrl Pts',(20.6433051769832,63.6581352626753,29.0007922476961));
#17707=CARTESIAN_POINT('Ctrl Pts',(18.4994791622271,64.1616335930124,28.8954588859795));
#17708=CARTESIAN_POINT('Ctrl Pts',(17.9486237066817,65.4266422691452,28.8271698969266));
#17709=CARTESIAN_POINT('Ctrl Pts',(17.943661294952,66.0016161416468,28.7959252805377));
#17710=CARTESIAN_POINT('Ctrl Pts',(17.9418460022328,65.9999766237505,29.5540747194623));
#17711=CARTESIAN_POINT('Ctrl Pts',(17.9419601590032,66.6788457316685,29.5170984924742));
#17712=CARTESIAN_POINT('Ctrl Pts',(18.6804456694416,68.0380478699251,29.4430778928223));
#17713=CARTESIAN_POINT('Ctrl Pts',(20.9956693718085,68.2151328103185,29.3320129205064));
#17714=CARTESIAN_POINT('Ctrl Pts',(22.4010378181641,66.3649496692051,29.2208798025149));
#17715=CARTESIAN_POINT('Ctrl Pts',(21.6088819494082,64.1807502265562,29.1097466845233));
#17716=CARTESIAN_POINT('Ctrl Pts',(19.3442139955776,63.6615997815364,28.9986135665318));
#17717=CARTESIAN_POINT('Ctrl Pts',(18.0677943199381,64.9047212114679,28.9133895781781));
#17718=CARTESIAN_POINT('Ctrl Pts',(17.9448854089212,65.7925912386986,28.8652099624883));
#17719=CARTESIAN_POINT('Ctrl Pts',(17.9465562858968,65.9982462861091,28.8540747194623));
#17720=CARTESIAN_POINT('Origin',(20.,66.,37.5459252805377));
#17721=CARTESIAN_POINT('',(17.9464881342612,66.0017684723116,30.2540747194623));
#17722=CARTESIAN_POINT('',(17.9454840967242,65.9981221130107,30.1959252805377));
#17723=CARTESIAN_POINT('',(17.94525,66.0000000000002,37.5459252805377));
#17724=CARTESIAN_POINT('Ctrl Pts',(17.9454840967242,65.9981221130106,30.1959252805377));
#17725=CARTESIAN_POINT('Ctrl Pts',(17.9501626777246,66.5133463578346,30.1679913295624));
#17726=CARTESIAN_POINT('Ctrl Pts',(18.4074704589656,67.7192338664832,30.1030130059232));
#17727=CARTESIAN_POINT('Ctrl Pts',(20.4322511218479,68.3898391088773,30.0009903096202));
#17728=CARTESIAN_POINT('Ctrl Pts',(22.2422273876527,66.9330532357364,29.8898571916286));
#17729=CARTESIAN_POINT('Ctrl Pts',(22.0000288950678,64.622300316632,29.778724073637));
#17730=CARTESIAN_POINT('Ctrl Pts',(19.9273252373466,63.5724723734772,29.6675909556455));
#17731=CARTESIAN_POINT('Ctrl Pts',(18.2256189202363,64.5665458908114,29.573324691279));
#17732=CARTESIAN_POINT('Ctrl Pts',(17.9492823488248,65.626966017977,29.5161027995764));
#17733=CARTESIAN_POINT('Ctrl Pts',(17.9484736033439,66.000497180875,29.4959252805377));
#17734=CARTESIAN_POINT('Ctrl Pts',(17.9464881342612,66.0017684723116,30.2540747194623));
#17735=CARTESIAN_POINT('Ctrl Pts',(17.9448197814205,66.2048893181186,30.2430757677879));
#17736=CARTESIAN_POINT('Ctrl Pts',(18.0658215769606,67.0901756412105,30.1950324434495));
#17737=CARTESIAN_POINT('Ctrl Pts',(19.3356363974357,68.3359777115578,30.1099447464474));
#17738=CARTESIAN_POINT('Ctrl Pts',(21.602194400799,67.8251421772989,29.9988116284558));
#17739=CARTESIAN_POINT('Ctrl Pts',(22.402361026794,65.6438646854799,29.8876785104642));
#17740=CARTESIAN_POINT('Ctrl Pts',(21.0037922850585,63.7885362508592,29.7765453924727));
#17741=CARTESIAN_POINT('Ctrl Pts',(18.6865133351581,63.957226481817,29.6654122744811));
#17742=CARTESIAN_POINT('Ctrl Pts',(17.9424133819219,65.3173543283634,29.5912553834777));
#17743=CARTESIAN_POINT('Ctrl Pts',(17.9418457918466,65.9987254957184,29.5541428651381));
#17744=CARTESIAN_POINT('Ctrl Pts',(17.9418460022328,65.9999766237505,29.5540747194623));
#17745=CARTESIAN_POINT('Origin',(20.,66.,37.5459252805377));
#17746=CARTESIAN_POINT('',(17.9480837821526,65.9989795847701,30.9540747194623));
#17747=CARTESIAN_POINT('',(17.9420997627439,66.0006544392236,30.8959252805377));
#17748=CARTESIAN_POINT('',(17.94525,66.0000000000002,37.5459252805377));
#17749=CARTESIAN_POINT('Ctrl Pts',(17.9420997627439,66.0006544392236,30.8959252805377));
#17750=CARTESIAN_POINT('Ctrl Pts',(17.9419499669099,66.0365901229561,30.893968604876));
#17751=CARTESIAN_POINT('Ctrl Pts',(17.9590876919192,66.752725177529,30.8549675565505));
#17752=CARTESIAN_POINT('Ctrl Pts',(18.7920501669056,68.1069003771858,30.7789221355611));
#17753=CARTESIAN_POINT('Ctrl Pts',(21.1149084810719,68.1575799121915,30.6677890175695));
#17754=CARTESIAN_POINT('Ctrl Pts',(22.4173586709909,66.2335573900417,30.556655899578));
#17755=CARTESIAN_POINT('Ctrl Pts',(21.507347058909,64.0957739517965,30.4455227815864));
#17756=CARTESIAN_POINT('Ctrl Pts',(19.2177520899114,63.700813142474,30.3343896635948));
#17757=CARTESIAN_POINT('Ctrl Pts',(18.0396474365576,64.9805047783244,30.2511904965786));
#17758=CARTESIAN_POINT('Ctrl Pts',(17.9439582171286,65.8300860862183,30.2050357022262));
#17759=CARTESIAN_POINT('Ctrl Pts',(17.9454840967242,65.9981221130106,30.1959252805377));
#17760=CARTESIAN_POINT('Ctrl Pts',(17.9480837821526,65.9989795847701,30.9540747194623));
#17761=CARTESIAN_POINT('Ctrl Pts',(17.9499190106596,66.407277615284,30.9320086704376));
#17762=CARTESIAN_POINT('Ctrl Pts',(18.2657185279594,67.503640125688,30.8728982487491));
#17763=CARTESIAN_POINT('Ctrl Pts',(20.0508159985709,68.4280833180919,30.7767434543967));
#17764=CARTESIAN_POINT('Ctrl Pts',(22.0674747085496,67.2742524062426,30.6656103364052));
#17765=CARTESIAN_POINT('Ctrl Pts',(22.1918991902521,64.954175538114,30.5544772184136));
#17766=CARTESIAN_POINT('Ctrl Pts',(20.3102112607245,63.5912783807532,30.4433441004221));
#17767=CARTESIAN_POINT('Ctrl Pts',(18.3589378352584,64.3496381873999,30.3432099341049));
#17768=CARTESIAN_POINT('Ctrl Pts',(17.9504387791389,65.520780092933,30.2801201404517));
#17769=CARTESIAN_POINT('Ctrl Pts',(17.9464881342612,66.0017684723116,30.2540747194623));
#17770=CARTESIAN_POINT('Origin',(20.,66.,37.5459252805377));
#17771=CARTESIAN_POINT('',(17.9427639177081,65.9987822673605,31.6540747194623));
#17772=CARTESIAN_POINT('',(17.9474132077665,66.0014635245165,31.5959252805377));
#17773=CARTESIAN_POINT('',(17.94525,66.0000000000002,37.5459252805377));
#17774=CARTESIAN_POINT('Ctrl Pts',(17.9474132077665,66.0014635245165,31.5959252805377));
#17775=CARTESIAN_POINT('Ctrl Pts',(17.9458281229253,66.2422509216447,31.5829015075258));
#17776=CARTESIAN_POINT('Ctrl Pts',(18.0963189550609,67.1660077074065,31.53283336185));
#17777=CARTESIAN_POINT('Ctrl Pts',(19.4639280035177,68.3687124800713,31.4457208435104));
#17778=CARTESIAN_POINT('Ctrl Pts',(21.6992788050032,67.7351148496642,31.3345877255189));
#17779=CARTESIAN_POINT('Ctrl Pts',(22.3793827611878,65.5134718153893,31.2234546075273));
#17780=CARTESIAN_POINT('Ctrl Pts',(20.8817819627404,63.737118525233,31.1123214895358));
#17781=CARTESIAN_POINT('Ctrl Pts',(18.6177165071394,64.0266543253153,31.0031450472058));
#17782=CARTESIAN_POINT('Ctrl Pts',(17.9447859467341,65.3562449404663,30.9310129775398));
#17783=CARTESIAN_POINT('Ctrl Pts',(17.9420997627439,66.0006544392236,30.8959252805377));
#17784=CARTESIAN_POINT('Ctrl Pts',(17.9427639177081,65.9987822673605,31.6540747194623));
#17785=CARTESIAN_POINT('Ctrl Pts',(17.9470403612663,66.6078147414705,31.6209415730874));
#17786=CARTESIAN_POINT('Ctrl Pts',(18.5560215546316,67.9052027566069,31.5507640540487));
#17787=CARTESIAN_POINT('Ctrl Pts',(20.7615158115174,68.3061362783054,31.4435421623461));
#17788=CARTESIAN_POINT('Ctrl Pts',(22.3504925588018,66.6110283105753,31.3324090443545));
#17789=CARTESIAN_POINT('Ctrl Pts',(21.7882060017851,64.3566831831669,31.2212759263629));
#17790=CARTESIAN_POINT('Ctrl Pts',(19.5892829288324,63.6063662868436,31.1101428083714));
#17791=CARTESIAN_POINT('Ctrl Pts',(18.1282339615618,64.7607922561806,31.0210757394045));
#17792=CARTESIAN_POINT('Ctrl Pts',(17.9468380382272,65.7218289251557,30.9690530431015));
#17793=CARTESIAN_POINT('Ctrl Pts',(17.9480837821526,65.9989795847701,30.9540747194623));
#17794=CARTESIAN_POINT('Origin',(20.,66.,37.5459252805377));
#17795=CARTESIAN_POINT('',(17.9443931880793,66.0017938242215,32.3540747194623));
#17796=CARTESIAN_POINT('',(17.9473846384895,65.9985230106727,32.2959252805377));
#17797=CARTESIAN_POINT('',(17.94525,66.0000000000002,37.5459252805377));
#17798=CARTESIAN_POINT('Ctrl Pts',(17.9473846384895,65.9985230106727,32.2959252805377));
#17799=CARTESIAN_POINT('Ctrl Pts',(17.9503462932394,66.443906616148,32.2718344101756));
#17800=CARTESIAN_POINT('Ctrl Pts',(18.311644403633,67.5785299615268,32.2106991671496));
#17801=CARTESIAN_POINT('Ctrl Pts',(20.1830643623602,68.4217058941771,32.1125195514598));
#17802=CARTESIAN_POINT('Ctrl Pts',(22.133845733665,67.1596871921246,32.0013864334682));
#17803=CARTESIAN_POINT('Ctrl Pts',(22.1316475021699,64.8362771269967,31.8902533154767));
#17804=CARTESIAN_POINT('Ctrl Pts',(20.1784815758609,63.5779520389273,31.7791201974851));
#17805=CARTESIAN_POINT('Ctrl Pts',(18.3099987609922,64.4240616204181,31.6810108525055));
#17806=CARTESIAN_POINT('Ctrl Pts',(17.9503366838091,65.5573635189058,31.6199458801896));
#17807=CARTESIAN_POINT('Ctrl Pts',(17.9474132077665,66.0014635245165,31.5959252805377));
#17808=CARTESIAN_POINT('Ctrl Pts',(17.9443931880793,66.0017938242215,32.3540747194623));
#17809=CARTESIAN_POINT('Ctrl Pts',(17.9431867476929,66.1335998339314,32.3469188484011));
#17810=CARTESIAN_POINT('Ctrl Pts',(18.0147855633186,66.9464311477664,32.302718604676));
#17811=CARTESIAN_POINT('Ctrl Pts',(19.0978804119286,68.2548505746783,32.221473988287));
#17812=CARTESIAN_POINT('Ctrl Pts',(21.4050826420595,67.9808870826703,32.1103408702955));
#17813=CARTESIAN_POINT('Ctrl Pts',(22.4262979346632,65.8939377656472,31.9992077523039));
#17814=CARTESIAN_POINT('Ctrl Pts',(21.2268698593072,63.9040607800724,31.8880746343123));
#17815=CARTESIAN_POINT('Ctrl Pts',(18.9045621995861,63.8324698639393,31.7769415163208));
#17816=CARTESIAN_POINT('Ctrl Pts',(17.978302645581,65.1745805746697,31.6989415447041));
#17817=CARTESIAN_POINT('Ctrl Pts',(17.9422591018274,65.9268885873393,31.6579859457513));
#17818=CARTESIAN_POINT('Ctrl Pts',(17.9427639177081,65.9987822673605,31.6540747194623));
#17819=CARTESIAN_POINT('Origin',(20.,66.,37.5459252805377));
#17820=CARTESIAN_POINT('',(17.9485812508208,66.0000908847383,33.0540747194623));
#17821=CARTESIAN_POINT('',(17.9420826509595,65.9993679635266,32.9959252805377));
#17822=CARTESIAN_POINT('',(17.94525,66.0000000000002,37.5459252805377));
#17823=CARTESIAN_POINT('Ctrl Pts',(17.9420826509595,65.9993679635266,32.9959252805377));
#17824=CARTESIAN_POINT('Ctrl Pts',(17.9446925158973,66.6450537162148,32.9607673128253));
#17825=CARTESIAN_POINT('Ctrl Pts',(18.6199954325073,67.9757741595962,32.8885649724491));
#17826=CARTESIAN_POINT('Ctrl Pts',(20.8860623082748,68.2612088768015,32.7793182594092));
#17827=CARTESIAN_POINT('Ctrl Pts',(22.3802991314904,66.4820249405198,32.6681851414175));
#17828=CARTESIAN_POINT('Ctrl Pts',(21.6959925019048,64.261672806363,32.5570520234261));
#17829=CARTESIAN_POINT('Ctrl Pts',(19.4594467809617,63.6323061397115,32.4459189054344));
#17830=CARTESIAN_POINT('Ctrl Pts',(18.0952173579541,64.836624342483,32.358876657805));
#17831=CARTESIAN_POINT('Ctrl Pts',(17.9457921762395,65.7590431798503,32.3088787828394));
#17832=CARTESIAN_POINT('Ctrl Pts',(17.9473846384895,65.9985230106727,32.2959252805377));
#17833=CARTESIAN_POINT('Ctrl Pts',(17.9485812508208,66.0000908847383,33.0540747194623));
#17834=CARTESIAN_POINT('Ctrl Pts',(17.9484481239615,66.3374829869665,33.0358517510509));
#17835=CARTESIAN_POINT('Ctrl Pts',(18.1868160160139,67.360562003179,32.9805844099755));
#17836=CARTESIAN_POINT('Ctrl Pts',(19.7997191989097,68.420342634033,32.8882726962363));
#17837=CARTESIAN_POINT('Ctrl Pts',(21.924781541228,67.4810087386156,32.7771395782448));
#17838=CARTESIAN_POINT('Ctrl Pts',(22.2882080583246,65.1861973537148,32.6660064602532));
#17839=CARTESIAN_POINT('Ctrl Pts',(20.5573764974643,63.6362101816373,32.5548733422617));
#17840=CARTESIAN_POINT('Ctrl Pts',(18.4607079236377,64.210156628494,32.4508960953314));
#17841=CARTESIAN_POINT('Ctrl Pts',(17.9494322245733,65.4512690734646,32.3839632210649));
#17842=CARTESIAN_POINT('Ctrl Pts',(17.9443931880793,66.0017938242215,32.3540747194623));
#17843=CARTESIAN_POINT('Origin',(20.,66.,37.5459252805377));
#17844=CARTESIAN_POINT('',(17.944726753288,65.9981586635862,33.7540747194623));
#17845=CARTESIAN_POINT('',(17.9455229217772,66.0018771066122,33.6959252805377));
#17846=CARTESIAN_POINT('',(17.94525,66.0000000000002,37.5459252805377));
#17847=CARTESIAN_POINT('Ctrl Pts',(17.9455229217772,66.0018771066122,33.6959252805377));
#17848=CARTESIAN_POINT('Ctrl Pts',(17.9439884406831,66.1712173960156,33.686744588139));
#17849=CARTESIAN_POINT('Ctrl Pts',(18.0405829995419,67.0221239091327,33.6405195230765));
#17850=CARTESIAN_POINT('Ctrl Pts',(19.2221041132247,68.3006629449443,33.55725008535));
#17851=CARTESIAN_POINT('Ctrl Pts',(21.5109476208589,67.9013703706408,33.4461169673585));
#17852=CARTESIAN_POINT('Ctrl Pts',(22.416912395611,65.7618687952487,33.3349838493669));
#17853=CARTESIAN_POINT('Ctrl Pts',(21.1108238171316,63.8403142715337,33.2238507313754));
#17854=CARTESIAN_POINT('Ctrl Pts',(18.7880655596257,63.8953891307446,33.1127176133838));
#17855=CARTESIAN_POINT('Ctrl Pts',(17.9584343459935,65.2498852778546,33.0367424631046));
#17856=CARTESIAN_POINT('Ctrl Pts',(17.9419426183449,65.9647236174436,32.9978116854892));
#17857=CARTESIAN_POINT('Ctrl Pts',(17.9420826509595,65.9993679635266,32.9959252805377));
#17858=CARTESIAN_POINT('Ctrl Pts',(17.944726753288,65.9981586635862,33.7540747194623));
#17859=CARTESIAN_POINT('Ctrl Pts',(17.9497080377066,66.5378859606725,33.7247846537006));
#17860=CARTESIAN_POINT('Ctrl Pts',(18.4440788206969,67.7683042539906,33.6584502152751));
#17861=CARTESIAN_POINT('Ctrl Pts',(20.5192141482499,68.3724644440178,33.5550714041857));
#17862=CARTESIAN_POINT('Ctrl Pts',(22.2747973910883,66.850569042428,33.4439382861942));
#17863=CARTESIAN_POINT('Ctrl Pts',(21.9483965247762,64.5501993772306,33.3328051682026));
#17864=CARTESIAN_POINT('Ctrl Pts',(19.8387464716884,63.5767443045379,33.221672050211));
#17865=CARTESIAN_POINT('Ctrl Pts',(18.1984100230512,64.617098038126,33.1287619006309));
#17866=CARTESIAN_POINT('Ctrl Pts',(17.9487187495192,65.6516189451392,33.0728961237147));
#17867=CARTESIAN_POINT('Ctrl Pts',(17.9485812508208,66.0000908847383,33.0540747194623));
#17868=CARTESIAN_POINT('Origin',(20.,66.,37.5459252805377));
#17869=CARTESIAN_POINT('',(17.9425257260813,66.0010592828743,34.4540747194623));
#17870=CARTESIAN_POINT('',(17.9484640187855,65.9994822145552,34.3959252805377));
#17871=CARTESIAN_POINT('',(17.94525,66.0000000000002,37.5459252805377));
#17872=CARTESIAN_POINT('Ctrl Pts',(17.9484640187855,65.9994822145552,34.3959252805377));
#17873=CARTESIAN_POINT('Ctrl Pts',(17.9493094009313,66.3743098843859,34.3756774907888));
#17874=CARTESIAN_POINT('Ctrl Pts',(18.227064603961,67.4360705115979,34.318385328376));
#17875=CARTESIAN_POINT('Ctrl Pts',(19.9319188439973,68.4276607754887,34.2240487932994));
#17876=CARTESIAN_POINT('Ctrl Pts',(22.0026322577385,67.3739126856969,34.1129156753079));
#17877=CARTESIAN_POINT('Ctrl Pts',(22.2404578093089,65.0627055872007,34.0017825573163));
#17878=CARTESIAN_POINT('Ctrl Pts',(20.4277281887608,63.6093472479493,33.8906494393247));
#17879=CARTESIAN_POINT('Ctrl Pts',(18.4056138422819,64.2833181305728,33.7886970137318));
#17880=CARTESIAN_POINT('Ctrl Pts',(17.9501801185026,65.487924185085,33.7237889608028));
#17881=CARTESIAN_POINT('Ctrl Pts',(17.9455229217772,66.0018771066122,33.6959252805377));
#17882=CARTESIAN_POINT('Ctrl Pts',(17.9425257260813,66.0010592828744,34.4540747194623));
#17883=CARTESIAN_POINT('Ctrl Pts',(17.942143328542,66.061934338497,34.4507619290142));
#17884=CARTESIAN_POINT('Ctrl Pts',(17.972203902059,66.8031450877885,34.4104047659023));
#17885=CARTESIAN_POINT('Ctrl Pts',(18.869777083907,68.1495967375546,34.3330032301266));
#17886=CARTESIAN_POINT('Ctrl Pts',(21.1929366566675,68.1154368741692,34.221870112135));
#17887=CARTESIAN_POINT('Ctrl Pts',(22.4242738572048,66.1451456586872,34.1107369941435));
#17888=CARTESIAN_POINT('Ctrl Pts',(21.4368201000595,64.0420115549533,33.9996038761519));
#17889=CARTESIAN_POINT('Ctrl Pts',(19.1343320873597,63.7309054758618,33.8884707581604));
#17890=CARTESIAN_POINT('Ctrl Pts',(18.0221618776052,65.0312099164754,33.8066277059305));
#17891=CARTESIAN_POINT('Ctrl Pts',(17.9434079987156,65.8552702474544,33.7618290263645));
#17892=CARTESIAN_POINT('Ctrl Pts',(17.944726753288,65.9981586635862,33.7540747194623));
#17893=CARTESIAN_POINT('Origin',(20.,66.,37.5459252805377));
#17894=CARTESIAN_POINT('',(17.9479090025127,66.0011644690241,35.1540747194623));
#17895=CARTESIAN_POINT('',(17.9436249754829,65.9983937900349,35.0959252805377));
#17896=CARTESIAN_POINT('',(17.94525,66.0000000000002,37.5459252805377));
#17897=CARTESIAN_POINT('Ctrl Pts',(17.9436249754829,65.9983937900349,35.0959252805377));
#17898=CARTESIAN_POINT('Ctrl Pts',(17.9485747373069,66.5746340545001,35.0646103934386));
#17899=CARTESIAN_POINT('Ctrl Pts',(18.5015294598482,67.8408719871184,34.9962511336756));
#17900=CARTESIAN_POINT('Ctrl Pts',(20.6477355083213,68.3406417811724,34.8908475012488));
#17901=CARTESIAN_POINT('Ctrl Pts',(22.3177707056507,66.7253356370374,34.7797143832572));
#17902=CARTESIAN_POINT('Ctrl Pts',(21.8664911119801,64.4461711240172,34.6685812652656));
#17903=CARTESIAN_POINT('Ctrl Pts',(19.7069252952836,63.5891332828492,34.5574481472741));
#17904=CARTESIAN_POINT('Ctrl Pts',(18.1601824626538,64.6927474056976,34.4665628190314));
#17905=CARTESIAN_POINT('Ctrl Pts',(17.9477627308186,65.6885433855173,34.4127218634526));
#17906=CARTESIAN_POINT('Ctrl Pts',(17.9484640187855,65.9994822145552,34.3959252805377));
#17907=CARTESIAN_POINT('Ctrl Pts',(17.9479090025127,66.0011644690241,35.1540747194623));
#17908=CARTESIAN_POINT('Ctrl Pts',(17.9465290092682,66.2671875841058,35.139694831664));
#17909=CARTESIAN_POINT('Ctrl Pts',(18.1181887624162,67.2168116767709,35.0882705712019));
#17910=CARTESIAN_POINT('Ctrl Pts',(19.5507726973617,68.3866954932114,34.999801938076));
#17911=CARTESIAN_POINT('Ctrl Pts',(21.761489833587,67.6719231014153,34.8886688200844));
#17912=CARTESIAN_POINT('Ctrl Pts',(22.3600352949887,65.4269244270303,34.7775357020928));
#17913=CARTESIAN_POINT('Ctrl Pts',(20.7985769670495,63.7064353263736,34.6664025841013));
#17914=CARTESIAN_POINT('Ctrl Pts',(18.5745658426963,64.0738149722658,34.5585822565578));
#17915=CARTESIAN_POINT('Ctrl Pts',(17.9464193843856,65.3812156870209,34.4878063016781));
#17916=CARTESIAN_POINT('Ctrl Pts',(17.9425257260813,66.0010592828744,34.4540747194623));
#17917=CARTESIAN_POINT('Origin',(20.,66.,37.5459252805377));
#17918=CARTESIAN_POINT('',(17.9473272485919,65.9976786215907,35.8540747194623));
#17919=CARTESIAN_POINT('',(17.9434278899737,66.0014963127332,35.7959252805377));
#17920=CARTESIAN_POINT('',(17.94525,66.0000000000002,37.5459252805377));
#17921=CARTESIAN_POINT('',(19.4698297828115,64.0148256743283,36.));
#17922=CARTESIAN_POINT('Ctrl Pts',(19.4698297828115,64.0148256743282,36.));
#17923=CARTESIAN_POINT('Ctrl Pts',(18.809740437582,64.1911123142462,35.9629556273362));
#17924=CARTESIAN_POINT('Ctrl Pts',(18.0750704080787,64.8872090652857,35.9143138671569));
#17925=CARTESIAN_POINT('Ctrl Pts',(17.94571015716,65.7834096722511,35.8656721069777));
#17926=CARTESIAN_POINT('Ctrl Pts',(17.9473272485919,65.9976786215907,35.8540747194623));
#17927=CARTESIAN_POINT('',(20.5313110481438,64.0112682685522,36.));
#17928=CARTESIAN_POINT('Origin',(20.,66.,36.));
#17929=CARTESIAN_POINT('Ctrl Pts',(20.5313117419429,64.0112661051077,36.));
#17930=CARTESIAN_POINT('Ctrl Pts',(19.886791318144,63.8399704354172,35.9636818543909));
#17931=CARTESIAN_POINT('Ctrl Pts',(18.5070307177422,64.1592653630963,35.8956569479035));
#17932=CARTESIAN_POINT('Ctrl Pts',(17.9482807196063,65.4183240387177,35.8276320414161));
#17933=CARTESIAN_POINT('Ctrl Pts',(17.9434278899737,66.0014963127332,35.7959252805377));
#17934=CARTESIAN_POINT('Origin',(20.,50.,-32.));
#17935=CARTESIAN_POINT('',(22.5134612402277,50.000273003858,-25.387416697508));
#17936=CARTESIAN_POINT('',(22.5157646541248,49.9966173859026,-25.112583302492));
#17937=CARTESIAN_POINT('',(22.5175,50.,-32.));
#17938=CARTESIAN_POINT('',(21.9134659966651,51.6359872033749,-25.));
#17939=CARTESIAN_POINT('Ctrl Pts',(22.5157646541248,49.9966173859026,-25.112583302492));
#17940=CARTESIAN_POINT('Ctrl Pts',(22.5105547734392,50.5891788966502,-25.0750555349947));
#17941=CARTESIAN_POINT('Ctrl Pts',(22.2992218280841,51.1848035603044,-25.0375277674973));
#17942=CARTESIAN_POINT('Ctrl Pts',(21.9134659966651,51.6359872033749,-25.));
#17943=CARTESIAN_POINT('',(22.5175,50.,-25.));
#17944=CARTESIAN_POINT('Origin',(20.,50.,-25.));
#17945=CARTESIAN_POINT('',(17.4825,50.,-25.));
#17946=CARTESIAN_POINT('Ctrl Pts',(22.5175,50.,-25.));
#17947=CARTESIAN_POINT('Ctrl Pts',(22.5175,50.3222180082023,-25.));
#17948=CARTESIAN_POINT('Ctrl Pts',(22.4519182005811,50.6620957154615,-24.965994767533));
#17949=CARTESIAN_POINT('Ctrl Pts',(22.1930921359231,51.2808669639972,-24.8434341672334));
#17950=CARTESIAN_POINT('Ctrl Pts',(22.0001401774783,51.560142465796,-24.75619390213));
#17951=CARTESIAN_POINT('Ctrl Pts',(21.5595215410958,52.0007611021785,-24.5883213994305));
#17952=CARTESIAN_POINT('Ctrl Pts',(21.2804542351089,52.1932581515168,-24.4956547875015));
#17953=CARTESIAN_POINT('Ctrl Pts',(20.6625974062016,52.4517149721102,-24.3600905047278));
#17954=CARTESIAN_POINT('Ctrl Pts',(20.3231274362054,52.5175,-24.3199761284063));
#17955=CARTESIAN_POINT('Ctrl Pts',(20.,52.5175,-24.3199761284063));
#17956=CARTESIAN_POINT('Ctrl Pts',(19.6768725637946,52.5175,-24.3199761284063));
#17957=CARTESIAN_POINT('Ctrl Pts',(19.3374025937983,52.4517149721102,-24.3600905047278));
#17958=CARTESIAN_POINT('Ctrl Pts',(18.719545764891,52.1932581515168,-24.4956547875015));
#17959=CARTESIAN_POINT('Ctrl Pts',(18.4404784589043,52.0007611021785,-24.5883213994305));
#17960=CARTESIAN_POINT('Ctrl Pts',(17.9998598225217,51.560142465796,-24.75619390213));
#17961=CARTESIAN_POINT('Ctrl Pts',(17.8069078640769,51.2808669639972,-24.8434341672334));
#17962=CARTESIAN_POINT('Ctrl Pts',(17.5480817994189,50.6620957154614,-24.965994767533));
#17963=CARTESIAN_POINT('Ctrl Pts',(17.4825,50.3222180082023,-25.));
#17964=CARTESIAN_POINT('Ctrl Pts',(17.4825,50.,-25.));
#17965=CARTESIAN_POINT('',(18.0829273529947,51.6385409730469,-25.));
#17966=CARTESIAN_POINT('Origin',(20.,50.,-25.));
#17967=CARTESIAN_POINT('Ctrl Pts',(18.0829198466036,51.6385462881155,-25.));
#17968=CARTESIAN_POINT('Ctrl Pts',(18.6057517157272,52.2473168557604,-25.0509462733027));
#17969=CARTESIAN_POINT('Ctrl Pts',(19.445447411393,52.5873619676629,-25.1018925466053));
#17970=CARTESIAN_POINT('Ctrl Pts',(20.2440955124524,52.5095730776923,-25.152838819908));
#17971=CARTESIAN_POINT('Ctrl Pts',(21.0694439951791,52.4291835516607,-25.2054883276388));
#17972=CARTESIAN_POINT('Ctrl Pts',(21.8509544003932,51.9025549819737,-25.2581378353696));
#17973=CARTESIAN_POINT('Ctrl Pts',(22.2348332639616,51.1677991119336,-25.3107873431004));
#17974=CARTESIAN_POINT('Ctrl Pts',(22.4210736218415,50.8113293784386,-25.3363304612363));
#17975=CARTESIAN_POINT('Ctrl Pts',(22.5137217010458,50.4058718100902,-25.3618735793722));
#17976=CARTESIAN_POINT('Ctrl Pts',(22.5134612402277,50.000273003858,-25.387416697508));
#17977=CARTESIAN_POINT('Origin',(20.,50.,-32.));
#17978=CARTESIAN_POINT('',(22.5187558030321,49.9979044734253,-26.387416697508));
#17979=CARTESIAN_POINT('',(22.5213591508609,50.0006703125801,-26.112583302492));
#17980=CARTESIAN_POINT('',(22.5175,50.,-32.));
#17981=CARTESIAN_POINT('Ctrl Pts',(22.5213591508609,50.0006703125801,-26.112583302492));
#17982=CARTESIAN_POINT('Ctrl Pts',(22.5214869459678,50.0371266568132,-26.1102687557771));
#17983=CARTESIAN_POINT('Ctrl Pts',(22.5207639649754,50.0735777470678,-26.1079542090622));
#17984=CARTESIAN_POINT('Ctrl Pts',(22.5191743291001,50.1099909212014,-26.1056396623473));
#17985=CARTESIAN_POINT('Ctrl Pts',(22.4830145290993,50.9382894734454,-26.0529901546165));
#17986=CARTESIAN_POINT('Ctrl Pts',(21.9984162027216,51.7469688557767,-26.0003406468856));
#17987=CARTESIAN_POINT('Ctrl Pts',(21.2850580716506,52.1695270068173,-25.9476911391548));
#17988=CARTESIAN_POINT('Ctrl Pts',(20.5716999405796,52.592085157858,-25.895041631424));
#17989=CARTESIAN_POINT('Ctrl Pts',(19.6295820048153,52.6285220776079,-25.8423921236932));
#17990=CARTESIAN_POINT('Ctrl Pts',(18.8858121581489,52.2621196683134,-25.7897426159623));
#17991=CARTESIAN_POINT('Ctrl Pts',(18.1420423114825,51.8957172590189,-25.7370931082315));
#17992=CARTESIAN_POINT('Ctrl Pts',(17.596620553914,51.1264755206799,-25.6844436005007));
#17993=CARTESIAN_POINT('Ctrl Pts',(17.4967796369456,50.303516827856,-25.6317940927699));
#17994=CARTESIAN_POINT('Ctrl Pts',(17.3969387199773,49.4805581350321,-25.5791445850391));
#17995=CARTESIAN_POINT('Ctrl Pts',(17.7426786436092,48.6038824877232,-25.5264950773082));
#17996=CARTESIAN_POINT('Ctrl Pts',(18.3773140075671,48.0701216980594,-25.4738455695774));
#17997=CARTESIAN_POINT('Ctrl Pts',(19.0119493715251,47.5363609083956,-25.4211960618466));
#17998=CARTESIAN_POINT('Ctrl Pts',(19.935480175809,47.3455149763769,-25.3685465541158));
#17999=CARTESIAN_POINT('Ctrl Pts',(20.7291490582878,47.5857187856067,-25.3158970463849));
#18000=CARTESIAN_POINT('Ctrl Pts',(21.5228179407665,47.8259225948365,-25.2632475386541));
#18001=CARTESIAN_POINT('Ctrl Pts',(22.1866249014401,48.4971761453148,-25.2105980309233));
#18002=CARTESIAN_POINT('Ctrl Pts',(22.4195857619951,49.291445495894,-25.1579485231925));
#18003=CARTESIAN_POINT('Ctrl Pts',(22.4864956680838,49.5195717465001,-25.142826782959));
#18004=CARTESIAN_POINT('Ctrl Pts',(22.5178639653183,49.7578458885432,-25.1277050427255));
#18005=CARTESIAN_POINT('Ctrl Pts',(22.5157646541248,49.9966173859026,-25.112583302492));
#18006=CARTESIAN_POINT('Ctrl Pts',(22.5134612402277,50.000273003858,-25.387416697508));
#18007=CARTESIAN_POINT('Ctrl Pts',(22.5131848388748,49.569851032566,-25.414523087103));
#18008=CARTESIAN_POINT('Ctrl Pts',(22.408279656946,49.1392700064923,-25.4416294766979));
#18009=CARTESIAN_POINT('Ctrl Pts',(22.1995628098958,48.766905021273,-25.4687358662929));
#18010=CARTESIAN_POINT('Ctrl Pts',(21.7941661703386,48.0436499710456,-25.5213853740237));
#18011=CARTESIAN_POINT('Ctrl Pts',(20.9971255693015,47.5400230409839,-25.5740348817546));
#18012=CARTESIAN_POINT('Ctrl Pts',(20.169891281729,47.4841783887763,-25.6266843894854));
#18013=CARTESIAN_POINT('Ctrl Pts',(19.3426569941565,47.4283337365687,-25.6793338972162));
#18014=CARTESIAN_POINT('Ctrl Pts',(18.4852290200485,47.8202713622153,-25.731983404947));
#18015=CARTESIAN_POINT('Ctrl Pts',(17.9862469875704,48.4823913860756,-25.7846329126778));
#18016=CARTESIAN_POINT('Ctrl Pts',(17.4872649550924,49.1445114099359,-25.8372824204087));
#18017=CARTESIAN_POINT('Ctrl Pts',(17.3467288642442,50.07681383201,-25.8899319281395));
#18018=CARTESIAN_POINT('Ctrl Pts',(17.6283799117207,50.856613802331,-25.9425814358703));
#18019=CARTESIAN_POINT('Ctrl Pts',(17.9100309591972,51.6364137726519,-25.9952309436011));
#18020=CARTESIAN_POINT('Ctrl Pts',(18.6138691449983,52.2637112912197,-26.0478804513319));
#18021=CARTESIAN_POINT('Ctrl Pts',(19.4208044095907,52.4541505214686,-26.1005299590628));
#18022=CARTESIAN_POINT('Ctrl Pts',(20.227739674183,52.6445897517174,-26.1531794667936));
#18023=CARTESIAN_POINT('Ctrl Pts',(21.1377720175666,52.3981706936473,-26.2058289745244));
#18024=CARTESIAN_POINT('Ctrl Pts',(21.7383600126164,51.8265936565345,-26.2584784822553));
#18025=CARTESIAN_POINT('Ctrl Pts',(22.2286383806489,51.3599978216689,-26.3014578873395));
#18026=CARTESIAN_POINT('Ctrl Pts',(22.5127043733564,50.6767181159384,-26.3444372924238));
#18027=CARTESIAN_POINT('Ctrl Pts',(22.5187558030321,49.9979044734253,-26.387416697508));
#18028=CARTESIAN_POINT('Origin',(20.,50.,-32.));
#18029=CARTESIAN_POINT('',(22.5196059184078,50.0018577146135,-27.387416697508));
#18030=CARTESIAN_POINT('',(22.514511951768,50.001528002557,-27.112583302492));
#18031=CARTESIAN_POINT('',(22.5175,50.,-32.));
#18032=CARTESIAN_POINT('Ctrl Pts',(22.514511951768,50.001528002557,-27.112583302492));
#18033=CARTESIAN_POINT('Ctrl Pts',(22.5162681753221,50.3148132588407,-27.0928324688287));
#18034=CARTESIAN_POINT('Ctrl Pts',(22.4619720370514,50.6275116919841,-27.0730816351654));
#18035=CARTESIAN_POINT('Ctrl Pts',(22.3488346564514,50.9172322204891,-27.0533308015021));
#18036=CARTESIAN_POINT('Ctrl Pts',(22.0472459996842,51.6895359857549,-27.0006812937713));
#18037=CARTESIAN_POINT('Ctrl Pts',(21.327538634317,52.2985615564516,-26.9480317860404));
#18038=CARTESIAN_POINT('Ctrl Pts',(20.5159808446024,52.4682180646552,-26.8953822783096));
#18039=CARTESIAN_POINT('Ctrl Pts',(19.7044230548878,52.6378745728588,-26.8427327705788));
#18040=CARTESIAN_POINT('Ctrl Pts',(18.8010148408259,52.3681620185693,-26.790083262848));
#18041=CARTESIAN_POINT('Ctrl Pts',(18.2153027880988,51.7813472751723,-26.7374337551172));
#18042=CARTESIAN_POINT('Ctrl Pts',(17.6295907353717,51.1945325317753,-26.6847842473863));
#18043=CARTESIAN_POINT('Ctrl Pts',(17.3615748439794,50.2906155992708,-26.6321347396555));
#18044=CARTESIAN_POINT('Ctrl Pts',(17.5327556249479,49.4793798671285,-26.5794852319247));
#18045=CARTESIAN_POINT('Ctrl Pts',(17.7039364059165,48.6681441349862,-26.5268357241938));
#18046=CARTESIAN_POINT('Ctrl Pts',(18.3143138592458,47.9495896032061,-26.474186216463));
#18047=CARTESIAN_POINT('Ctrl Pts',(19.0871834798727,47.6494493128525,-26.4215367087322));
#18048=CARTESIAN_POINT('Ctrl Pts',(19.8600531004996,47.3493090224989,-26.3688872010014));
#18049=CARTESIAN_POINT('Ctrl Pts',(20.795414888424,47.4675829735717,-26.3162376932706));
#18050=CARTESIAN_POINT('Ctrl Pts',(21.4692351455743,47.9506788101863,-26.2635881855397));
#18051=CARTESIAN_POINT('Ctrl Pts',(22.1134333126076,48.4125370715641,-26.2132532245238));
#18052=CARTESIAN_POINT('Ctrl Pts',(22.5185799623133,49.207846104737,-26.1629182635079));
#18053=CARTESIAN_POINT('Ctrl Pts',(22.5213591508609,50.0006703125801,-26.112583302492));
#18054=CARTESIAN_POINT('Ctrl Pts',(22.5187558030321,49.9979044734253,-26.387416697508));
#18055=CARTESIAN_POINT('Ctrl Pts',(22.5201173376092,49.8451755655187,-26.3970868001546));
#18056=CARTESIAN_POINT('Ctrl Pts',(22.5074051519233,49.6926727397414,-26.4067569028011));
#18057=CARTESIAN_POINT('Ctrl Pts',(22.4798014410344,49.5429148261515,-26.4164270054477));
#18058=CARTESIAN_POINT('Ctrl Pts',(22.3295112276869,48.7275480490366,-26.4690765131785));
#18059=CARTESIAN_POINT('Ctrl Pts',(21.737787154276,47.9935495109622,-26.5217260209094));
#18060=CARTESIAN_POINT('Ctrl Pts',(20.9728803238817,47.6736637582043,-26.5743755286402));
#18061=CARTESIAN_POINT('Ctrl Pts',(20.2079734934874,47.3537780054464,-26.627025036371));
#18062=CARTESIAN_POINT('Ctrl Pts',(19.2698839061096,47.4480050380052,-26.6796745441019));
#18063=CARTESIAN_POINT('Ctrl Pts',(18.5838792098904,47.9136297340241,-26.7323240518327));
#18064=CARTESIAN_POINT('Ctrl Pts',(17.8978745136712,48.3792544300429,-26.7849735595635));
#18065=CARTESIAN_POINT('Ctrl Pts',(17.4639547086106,49.216276789522,-26.8376230672943));
#18066=CARTESIAN_POINT('Ctrl Pts',(17.4788312425904,50.0452448160541,-26.8902725750251));
#18067=CARTESIAN_POINT('Ctrl Pts',(17.4937077765703,50.8742128425862,-26.9429220827559));
#18068=CARTESIAN_POINT('Ctrl Pts',(17.9573806495906,51.6951265361713,-26.9955715904868));
#18069=CARTESIAN_POINT('Ctrl Pts',(18.6596505630897,52.1358374778744,-27.0482210982176));
#18070=CARTESIAN_POINT('Ctrl Pts',(19.3619204765888,52.5765484195774,-27.1008706059484));
#18071=CARTESIAN_POINT('Ctrl Pts',(20.3027874305667,52.6370566093984,-27.1535201136792));
#18072=CARTESIAN_POINT('Ctrl Pts',(21.0557238258934,52.289931418589,-27.2061696214101));
#18073=CARTESIAN_POINT('Ctrl Pts',(21.80866022122,51.9428062277797,-27.2588191291409));
#18074=CARTESIAN_POINT('Ctrl Pts',(22.3736660578954,51.18804765634,-27.3114686368717));
#18075=CARTESIAN_POINT('Ctrl Pts',(22.494604468072,50.3678141060487,-27.3641181446025));
#18076=CARTESIAN_POINT('Ctrl Pts',(22.5124437608419,50.2468237075311,-27.3718843289044));
#18077=CARTESIAN_POINT('Ctrl Pts',(22.5206208613874,50.1244086788925,-27.3796505132062));
#18078=CARTESIAN_POINT('Ctrl Pts',(22.5196059184078,50.0018577146135,-27.387416697508));
#18079=CARTESIAN_POINT('Origin',(20.,50.,-32.));
#18080=CARTESIAN_POINT('',(22.5135351409985,50.0002853817648,-28.387416697508));
#18081=CARTESIAN_POINT('',(22.5160872418661,49.9978763965905,-28.112583302492));
#18082=CARTESIAN_POINT('',(22.5175,50.,-32.));
#18083=CARTESIAN_POINT('Ctrl Pts',(22.5160872418661,49.9978763965905,-28.112583302492));
#18084=CARTESIAN_POINT('Ctrl Pts',(22.5112878705318,50.5868020213575,-28.0753961818803));
#18085=CARTESIAN_POINT('Ctrl Pts',(22.3047333820125,51.1787611658199,-28.0382090612686));
#18086=CARTESIAN_POINT('Ctrl Pts',(21.9270451822179,51.6262950900966,-28.0010219406569));
#18087=CARTESIAN_POINT('Ctrl Pts',(21.3923144080189,52.2599134079022,-27.9483724329261));
#18088=CARTESIAN_POINT('Ctrl Pts',(20.5145481122645,52.6040330619851,-27.8957229251952));
#18089=CARTESIAN_POINT('Ctrl Pts',(19.6916682954148,52.5026526660411,-27.8430734174644));
#18090=CARTESIAN_POINT('Ctrl Pts',(18.8687884785652,52.4012722700971,-27.7904239097336));
#18091=CARTESIAN_POINT('Ctrl Pts',(18.1007951406203,51.8543918241262,-27.7377744020028));
#18092=CARTESIAN_POINT('Ctrl Pts',(17.7358463859764,51.1099312104162,-27.685124894272));
#18093=CARTESIAN_POINT('Ctrl Pts',(17.3708976313326,50.3654705967061,-27.6324753865411));
#18094=CARTESIAN_POINT('Ctrl Pts',(17.4089934599897,49.4234298152568,-27.5798258788103));
#18095=CARTESIAN_POINT('Ctrl Pts',(17.8328637006338,48.7108688315972,-27.5271763710795));
#18096=CARTESIAN_POINT('Ctrl Pts',(18.2567339412778,47.9983078479377,-27.4745268633487));
#18097=CARTESIAN_POINT('Ctrl Pts',(19.0663785939088,47.5152266620678,-27.4218773556178));
#18098=CARTESIAN_POINT('Ctrl Pts',(19.8947575807264,47.4806225790254,-27.369227847887));
#18099=CARTESIAN_POINT('Ctrl Pts',(20.723136567544,47.446018495983,-27.3165783401562));
#18100=CARTESIAN_POINT('Ctrl Pts',(21.5702498885484,47.8598915157682,-27.2639288324254));
#18101=CARTESIAN_POINT('Ctrl Pts',(22.052071574967,48.5346190055783,-27.2112793246946));
#18102=CARTESIAN_POINT('Ctrl Pts',(22.3531436134977,48.9562305405835,-27.178380650627));
#18103=CARTESIAN_POINT('Ctrl Pts',(22.5115866359416,49.4796933442159,-27.1454819765595));
#18104=CARTESIAN_POINT('Ctrl Pts',(22.514511951768,50.001528002557,-27.112583302492));
#18105=CARTESIAN_POINT('Ctrl Pts',(22.5196059184078,50.0018577146135,-27.387416697508));
#18106=CARTESIAN_POINT('Ctrl Pts',(22.5137402304142,49.2935955420337,-27.432300020937));
#18107=CARTESIAN_POINT('Ctrl Pts',(22.2008545185939,48.5807930337343,-27.477183344366));
#18108=CARTESIAN_POINT('Ctrl Pts',(21.6717030769048,48.1122109708708,-27.522066667795));
#18109=CARTESIAN_POINT('Ctrl Pts',(21.0509922918832,47.5625499151274,-27.5747161755258));
#18110=CARTESIAN_POINT('Ctrl Pts',(20.1326997381625,47.3489363327836,-27.6273656832566));
#18111=CARTESIAN_POINT('Ctrl Pts',(19.3331193645885,47.5682087134236,-27.6800151909875));
#18112=CARTESIAN_POINT('Ctrl Pts',(18.5335389910145,47.7874810940636,-27.7326646987183));
#18113=CARTESIAN_POINT('Ctrl Pts',(17.8526707975874,48.4396394376874,-27.7853142064491));
#18114=CARTESIAN_POINT('Ctrl Pts',(17.5991760340398,49.2290376662104,-27.8379637141799));
#18115=CARTESIAN_POINT('Ctrl Pts',(17.3456812704923,50.0184358947333,-27.8906132219108));
#18116=CARTESIAN_POINT('Ctrl Pts',(17.5195599368243,50.9450740081554,-27.9432627296416));
#18117=CARTESIAN_POINT('Ctrl Pts',(18.041986779737,51.588874714119,-27.9959122373724));
#18118=CARTESIAN_POINT('Ctrl Pts',(18.5644136226497,52.2326754200825,-28.0485617451032));
#18119=CARTESIAN_POINT('Ctrl Pts',(19.4353886421431,52.5936387185874,-28.101211252834));
#18120=CARTESIAN_POINT('Ctrl Pts',(20.260068559922,52.5081273847708,-28.1538607605649));
#18121=CARTESIAN_POINT('Ctrl Pts',(21.0847484777008,52.4226160509542,-28.2065102682957));
#18122=CARTESIAN_POINT('Ctrl Pts',(21.8631332937651,51.8906300848161,-28.2591597760265));
#18123=CARTESIAN_POINT('Ctrl Pts',(22.2423540874804,51.1533372355938,-28.3118092837573));
#18124=CARTESIAN_POINT('Ctrl Pts',(22.423880972783,50.8004070252958,-28.3370117550076));
#18125=CARTESIAN_POINT('Ctrl Pts',(22.5139441053345,50.400433151388,-28.3622142262578));
#18126=CARTESIAN_POINT('Ctrl Pts',(22.5135351409985,50.0002853817648,-28.387416697508));
#18127=CARTESIAN_POINT('Origin',(20.,50.,-32.));
#18128=CARTESIAN_POINT('',(22.5185977288488,49.9978738300597,-29.387416697508));
#18129=CARTESIAN_POINT('',(22.5214168327014,50.00056091356,-29.112583302492));
#18130=CARTESIAN_POINT('',(22.5175,50.,-32.));
#18131=CARTESIAN_POINT('Ctrl Pts',(22.5214168327014,50.00056091356,-29.112583302492));
#18132=CARTESIAN_POINT('Ctrl Pts',(22.5215115546983,50.0316502586541,-29.1106094026627));
#18133=CARTESIAN_POINT('Ctrl Pts',(22.5209857633104,50.0627363262992,-29.1086355028334));
#18134=CARTESIAN_POINT('Ctrl Pts',(22.5198294794022,50.0937989242928,-29.1066616030042));
#18135=CARTESIAN_POINT('Ctrl Pts',(22.4889881075843,50.9223265268352,-29.0540120952734));
#18136=CARTESIAN_POINT('Ctrl Pts',(22.0095890011769,51.7341568754072,-29.0013625875425));
#18137=CARTESIAN_POINT('Ctrl Pts',(21.298960454951,52.1612590266266,-28.9487130798117));
#18138=CARTESIAN_POINT('Ctrl Pts',(20.588331908725,52.588361177846,-28.8960635720809));
#18139=CARTESIAN_POINT('Ctrl Pts',(19.6464739226806,52.6307351317128,-28.8434140643501));
#18140=CARTESIAN_POINT('Ctrl Pts',(18.9003634921058,52.2691713010304,-28.7907645566192));
#18141=CARTESIAN_POINT('Ctrl Pts',(18.1542530615311,51.9076074703479,-28.7381150488884));
#18142=CARTESIAN_POINT('Ctrl Pts',(17.603890186426,51.1421058551164,-28.6854655411576));
#18143=CARTESIAN_POINT('Ctrl Pts',(17.4987735070085,50.3196949709328,-28.6328160334268));
#18144=CARTESIAN_POINT('Ctrl Pts',(17.3936568275909,49.4972840867492,-28.5801665256959));
#18145=CARTESIAN_POINT('Ctrl Pts',(17.733786343861,48.6179639336134,-28.5275170179651));
#18146=CARTESIAN_POINT('Ctrl Pts',(18.3649695117957,48.0803609329424,-28.4748675102343));
#18147=CARTESIAN_POINT('Ctrl Pts',(18.9961526797304,47.5427579322714,-28.4222180025035));
#18148=CARTESIAN_POINT('Ctrl Pts',(19.9183894993297,47.3468720840651,-28.3695684947727));
#18149=CARTESIAN_POINT('Ctrl Pts',(20.7135979329253,47.5815052555246,-28.3169189870418));
#18150=CARTESIAN_POINT('Ctrl Pts',(21.5088063665209,47.816138426984,-28.264269479311));
#18151=CARTESIAN_POINT('Ctrl Pts',(22.1769864141127,48.4812906181093,-28.2116199715802));
#18152=CARTESIAN_POINT('Ctrl Pts',(22.4152288115867,49.275425204436,-28.1589704638494));
#18153=CARTESIAN_POINT('Ctrl Pts',(22.4851971044864,49.508650868411,-28.1435080767302));
#18154=CARTESIAN_POINT('Ctrl Pts',(22.5180828181915,49.7530014010348,-28.1280456896111));
#18155=CARTESIAN_POINT('Ctrl Pts',(22.5160872418661,49.9978763965905,-28.112583302492));
#18156=CARTESIAN_POINT('Ctrl Pts',(22.5135351409985,50.0002853817648,-28.387416697508));
#18157=CARTESIAN_POINT('Ctrl Pts',(22.513089753761,49.5644999255914,-28.4148637339886));
#18158=CARTESIAN_POINT('Ctrl Pts',(22.4053395245617,49.1285082196138,-28.4423107704692));
#18159=CARTESIAN_POINT('Ctrl Pts',(22.1915653615212,48.7528512927249,-28.4697578069498));
#18160=CARTESIAN_POINT('Ctrl Pts',(21.7814990704807,48.0322579313851,-28.5224073146806));
#18161=CARTESIAN_POINT('Ctrl Pts',(20.9813097170337,47.533670941012,-28.5750568224115));
#18162=CARTESIAN_POINT('Ctrl Pts',(20.1537509759774,47.4831171521003,-28.6277063301423));
#18163=CARTESIAN_POINT('Ctrl Pts',(19.3261922349211,47.4325633631885,-28.6803558378731));
#18164=CARTESIAN_POINT('Ctrl Pts',(18.4712641062555,47.8300427757381,-28.7330053456039));
#18165=CARTESIAN_POINT('Ctrl Pts',(17.9765352565092,48.4953641422999,-28.7856548533347));
#18166=CARTESIAN_POINT('Ctrl Pts',(17.4818064067629,49.1606855088617,-28.8383043610656));
#18167=CARTESIAN_POINT('Ctrl Pts',(17.3472768359358,50.0938488294357,-28.8909538687964));
#18168=CARTESIAN_POINT('Ctrl Pts',(17.6339334791313,50.8718187031622,-28.9436033765272));
#18169=CARTESIAN_POINT('Ctrl Pts',(17.9205901223267,51.6497885768887,-28.996252884258));
#18170=CARTESIAN_POINT('Ctrl Pts',(18.6284329795446,52.2725650037676,-29.0489023919889));
#18171=CARTESIAN_POINT('Ctrl Pts',(19.4365722555317,52.4578217610763,-29.1015518997197));
#18172=CARTESIAN_POINT('Ctrl Pts',(20.2447115315189,52.643078518385,-29.1542014074505));
#18173=CARTESIAN_POINT('Ctrl Pts',(21.1531472262752,52.3908156061234,-29.2068509151813));
#18174=CARTESIAN_POINT('Ctrl Pts',(21.7500538319779,51.8153925794714,-29.2595004229121));
#18175=CARTESIAN_POINT('Ctrl Pts',(22.2334649316189,51.3493801825317,-29.3021391811108));
#18176=CARTESIAN_POINT('Ctrl Pts',(22.5125521775403,50.671415443866,-29.3447779393094));
#18177=CARTESIAN_POINT('Ctrl Pts',(22.5185977288488,49.9978738300597,-29.387416697508));
#18178=CARTESIAN_POINT('Origin',(20.,50.,-32.));
#18179=CARTESIAN_POINT('',(22.5197498940917,50.0018038620106,-30.387416697508));
#18180=CARTESIAN_POINT('',(22.5146148548194,50.0015907043193,-30.112583302492));
#18181=CARTESIAN_POINT('',(22.5175,50.,-32.));
#18182=CARTESIAN_POINT('Ctrl Pts',(22.5146148548194,50.0015907043193,-30.112583302492));
#18183=CARTESIAN_POINT('Ctrl Pts',(22.5164165725427,50.3094409506913,-30.0931731157143));
#18184=CARTESIAN_POINT('Ctrl Pts',(22.4640313740575,50.6166994268775,-30.0737629289367));
#18185=CARTESIAN_POINT('Ctrl Pts',(22.3546757956077,50.9021312216285,-30.054352742159));
#18186=CARTESIAN_POINT('Ctrl Pts',(22.0580523040901,51.6763557902278,-30.0017032344282));
#18187=CARTESIAN_POINT('Ctrl Pts',(21.3422702745872,52.2899909457831,-29.9490537266973));
#18188=CARTESIAN_POINT('Ctrl Pts',(20.5318186054112,52.4648545219549,-29.8964042189665));
#18189=CARTESIAN_POINT('Ctrl Pts',(19.7213669362353,52.6397180981267,-29.8437547112357));
#18190=CARTESIAN_POINT('Ctrl Pts',(18.8162456273862,52.375810094915,-29.7911052035048));
#18191=CARTESIAN_POINT('Ctrl Pts',(18.2267776602203,51.792769192383,-29.738455695774));
#18192=CARTESIAN_POINT('Ctrl Pts',(17.6373096930544,51.209728289851,-29.6858061880432));
#18193=CARTESIAN_POINT('Ctrl Pts',(17.3634950675715,50.3075544879986,-29.6331566803124));
#18194=CARTESIAN_POINT('Ctrl Pts',(17.5294634803876,49.4952345606944,-29.5805071725816));
#18195=CARTESIAN_POINT('Ctrl Pts',(17.6954318932037,48.6829146333902,-29.5278576648508));
#18196=CARTESIAN_POINT('Ctrl Pts',(18.3011833443186,47.9604485806342,-29.4752081571199));
#18197=CARTESIAN_POINT('Ctrl Pts',(19.0721096249166,47.655355401064,-29.4225586493891));
#18198=CARTESIAN_POINT('Ctrl Pts',(19.8430359055145,47.3502622214937,-29.3699091416583));
#18199=CARTESIAN_POINT('Ctrl Pts',(20.7791370155955,47.4625419151092,-29.3172596339275));
#18200=CARTESIAN_POINT('Ctrl Pts',(21.4560457520219,47.9412941901733,-29.2646101261967));
#18201=CARTESIAN_POINT('Ctrl Pts',(22.1075762827091,48.4020974078818,-29.2139345182951));
#18202=CARTESIAN_POINT('Ctrl Pts',(22.518985050346,49.2024092350691,-29.1632589103935));
#18203=CARTESIAN_POINT('Ctrl Pts',(22.5214168327014,50.00056091356,-29.112583302492));
#18204=CARTESIAN_POINT('Ctrl Pts',(22.5185977288488,49.9978738300597,-29.387416697508));
#18205=CARTESIAN_POINT('Ctrl Pts',(22.5200171064876,49.8397393843069,-29.3974274470402));
#18206=CARTESIAN_POINT('Ctrl Pts',(22.5063859100399,49.6818487495533,-29.4074381965724));
#18207=CARTESIAN_POINT('Ctrl Pts',(22.4768148244427,49.5270021587398,-29.4174489461046));
#18208=CARTESIAN_POINT('Ctrl Pts',(22.3212916945558,48.7126179057026,-29.4700984538354));
#18209=CARTESIAN_POINT('Ctrl Pts',(21.7248679181332,47.9824325406707,-29.5227479615663));
#18210=CARTESIAN_POINT('Ctrl Pts',(20.9579231445072,47.6674644950945,-29.5753974692971));
#18211=CARTESIAN_POINT('Ctrl Pts',(20.1909783708812,47.3524964495183,-29.6280469770279));
#18212=CARTESIAN_POINT('Ctrl Pts',(19.2535126000518,47.4527457233978,-29.6806964847587));
#18213=CARTESIAN_POINT('Ctrl Pts',(18.5705116833604,47.922765832889,-29.7333459924896));
#18214=CARTESIAN_POINT('Ctrl Pts',(17.887510766669,48.3927859423803,-29.7859955002204));
#18215=CARTESIAN_POINT('Ctrl Pts',(17.4589747041155,49.2325768874833,-29.8386450079512));
#18216=CARTESIAN_POINT('Ctrl Pts',(17.4791738029899,50.0614322137804,-29.891294515682));
#18217=CARTESIAN_POINT('Ctrl Pts',(17.4993729018644,50.8902875400776,-29.9439440234128));
#18218=CARTESIAN_POINT('Ctrl Pts',(17.9683071621667,51.7082072475688,-29.9965935311437));
#18219=CARTESIAN_POINT('Ctrl Pts',(18.6733923679848,52.1443998748141,-30.0492430388745));
#18220=CARTESIAN_POINT('Ctrl Pts',(19.378477573803,52.5805925020594,-30.1018925466053));
#18221=CARTESIAN_POINT('Ctrl Pts',(20.3197137251369,52.6350580490587,-30.1545420543361));
#18222=CARTESIAN_POINT('Ctrl Pts',(21.0704057259808,52.2831053883275,-30.207191562067));
#18223=CARTESIAN_POINT('Ctrl Pts',(21.8210977268248,51.9311527275964,-30.2598410697978));
#18224=CARTESIAN_POINT('Ctrl Pts',(22.3812455771788,51.1727818591349,-30.3124905775286));
#18225=CARTESIAN_POINT('Ctrl Pts',(22.4969147671484,50.3517886837562,-30.3651400852594));
#18226=CARTESIAN_POINT('Ctrl Pts',(22.5132284220151,50.2359981321448,-30.3725656226756));
#18227=CARTESIAN_POINT('Ctrl Pts',(22.5207007373935,50.1189619300123,-30.3799911600918));
#18228=CARTESIAN_POINT('Ctrl Pts',(22.5197498940917,50.0018038620106,-30.387416697508));
#18229=CARTESIAN_POINT('Origin',(20.,50.,-32.));
#18230=CARTESIAN_POINT('',(22.5135563364326,50.0003713189448,-31.387416697508));
#18231=CARTESIAN_POINT('',(22.5159430076381,49.9979064240735,-31.112583302492));
#18232=CARTESIAN_POINT('',(22.5175,50.,-32.));
#18233=CARTESIAN_POINT('Ctrl Pts',(22.5159430076381,49.9979064240735,-31.112583302492));
#18234=CARTESIAN_POINT('Ctrl Pts',(22.5112750114203,50.5815220951261,-31.0757368287659));
#18235=CARTESIAN_POINT('Ctrl Pts',(22.3088213343573,51.1680598664448,-31.0388903550399));
#18236=CARTESIAN_POINT('Ctrl Pts',(21.9374478949046,51.6138880066437,-31.0020438813138));
#18237=CARTESIAN_POINT('Ctrl Pts',(21.406796606077,52.2509267715613,-30.949394373583));
#18238=CARTESIAN_POINT('Ctrl Pts',(20.5312579962154,52.6006754821119,-30.8967448658522));
#18239=CARTESIAN_POINT('Ctrl Pts',(19.7077441799491,52.5045808789307,-30.8440953581213));
#18240=CARTESIAN_POINT('Ctrl Pts',(18.8842303636827,52.4084862757494,-30.7914458503905));
#18241=CARTESIAN_POINT('Ctrl Pts',(18.1127413410116,51.8665483588361,-30.7387963426597));
#18242=CARTESIAN_POINT('Ctrl Pts',(17.7430199284747,51.1244464416753,-30.6861468349288));
#18243=CARTESIAN_POINT('Ctrl Pts',(17.3732985159378,50.3823445245144,-30.633497327198));
#18244=CARTESIAN_POINT('Ctrl Pts',(17.4053447135351,49.440078607106,-30.5808478194672));
#18245=CARTESIAN_POINT('Ctrl Pts',(17.8246308649064,48.7248106142456,-30.5281983117364));
#18246=CARTESIAN_POINT('Ctrl Pts',(18.2439170162777,48.0095426213853,-30.4755488040056));
#18247=CARTESIAN_POINT('Ctrl Pts',(19.050443121423,47.5212725530731,-30.4228992962748));
#18248=CARTESIAN_POINT('Ctrl Pts',(19.878582835266,47.4813502197473,-30.3702497885439));
#18249=CARTESIAN_POINT('Ctrl Pts',(20.7067225491089,47.4414278864215,-30.3176002808131));
#18250=CARTESIAN_POINT('Ctrl Pts',(21.5564758716496,47.8498532880821,-30.2649507730823));
#18251=CARTESIAN_POINT('Ctrl Pts',(22.0426200561537,48.521472979734,-30.2123012653514));
#18252=CARTESIAN_POINT('Ctrl Pts',(22.3495384543439,48.9454880076317,-30.1790619443983));
#18253=CARTESIAN_POINT('Ctrl Pts',(22.511529471131,49.4744070526688,-30.1458226234451));
#18254=CARTESIAN_POINT('Ctrl Pts',(22.5146148548194,50.0015907043193,-30.112583302492));
#18255=CARTESIAN_POINT('Ctrl Pts',(22.5197498940917,50.0018038620106,-30.387416697508));
#18256=CARTESIAN_POINT('Ctrl Pts',(22.5139589449867,49.2882726126943,-30.4326406678226));
#18257=CARTESIAN_POINT('Ctrl Pts',(22.1957352286107,48.5702211005946,-30.4778646381373));
#18258=CARTESIAN_POINT('Ctrl Pts',(21.6595471291725,48.1015158787921,-30.5230886084519));
#18259=CARTESIAN_POINT('Ctrl Pts',(21.0353197716417,47.5558517315029,-30.5757381161827));
#18260=CARTESIAN_POINT('Ctrl Pts',(20.1156745269951,47.3481389192203,-30.6283876239135));
#18261=CARTESIAN_POINT('Ctrl Pts',(19.3175185820202,47.5725408867429,-30.6810371316444));
#18262=CARTESIAN_POINT('Ctrl Pts',(18.5193626370453,47.7969428542654,-30.7336866393752));
#18263=CARTESIAN_POINT('Ctrl Pts',(17.8426959917422,48.4534596015932,-30.786336147106));
#18264=CARTESIAN_POINT('Ctrl Pts',(17.5942751798161,49.2444692448522,-30.8389856548368));
#18265=CARTESIAN_POINT('Ctrl Pts',(17.3458543678901,50.0354788881112,-30.8916351625677));
#18266=CARTESIAN_POINT('Ctrl Pts',(17.5256793893411,50.9609814273015,-30.9442846702985));
#18267=CARTESIAN_POINT('Ctrl Pts',(18.0522293052598,51.6014143602248,-30.9969341780293));
#18268=CARTESIAN_POINT('Ctrl Pts',(18.5787792211785,52.2418472931482,-31.0495836857601));
#18269=CARTESIAN_POINT('Ctrl Pts',(19.4520540315648,52.5972106198046,-31.102233193491));
#18270=CARTESIAN_POINT('Ctrl Pts',(20.2761678808566,52.5064057799978,-31.1548827012218));
#18271=CARTESIAN_POINT('Ctrl Pts',(21.1002817301483,52.415600940191,-31.2075322089526));
#18272=CARTESIAN_POINT('Ctrl Pts',(21.8752346183454,51.8786279339211,-31.2601817166834));
#18273=CARTESIAN_POINT('Ctrl Pts',(22.2497134381471,51.1389153079327,-31.3128312244142));
#18274=CARTESIAN_POINT('Ctrl Pts',(22.4265475064497,50.7896127943817,-31.3376930487788));
#18275=CARTESIAN_POINT('Ctrl Pts',(22.5140815132308,50.3951022088419,-31.3625548731434));
#18276=CARTESIAN_POINT('Ctrl Pts',(22.5135563364326,50.0003713189448,-31.387416697508));
#18277=CARTESIAN_POINT('Origin',(20.,50.,-32.));
#18278=CARTESIAN_POINT('',(22.518438676647,49.9978466804791,-32.387416697508));
#18279=CARTESIAN_POINT('',(22.5214653521749,50.000465985833,-32.112583302492));
#18280=CARTESIAN_POINT('',(22.5175,50.,-32.));
#18281=CARTESIAN_POINT('Ctrl Pts',(22.5214653521749,50.000465985833,-32.112583302492));
#18282=CARTESIAN_POINT('Ctrl Pts',(22.5215314384593,50.0261887418618,-32.1109500495483));
#18283=CARTESIAN_POINT('Ctrl Pts',(22.5211715019415,50.0519096037782,-32.1093167966047));
#18284=CARTESIAN_POINT('Ctrl Pts',(22.5203798163051,50.0776171696253,-32.1076835436611));
#18285=CARTESIAN_POINT('Ctrl Pts',(22.4948590546864,50.9063257245881,-32.0550340359302));
#18286=CARTESIAN_POINT('Ctrl Pts',(22.0206825923804,51.7212175581987,-32.0023845281994));
#18287=CARTESIAN_POINT('Ctrl Pts',(21.312811117861,52.1528738495971,-31.9497350204686));
#18288=CARTESIAN_POINT('Ctrl Pts',(20.6049396433416,52.5845301409955,-31.8970855127378));
#18289=CARTESIAN_POINT('Ctrl Pts',(19.6633731566088,52.6329508901818,-31.844436005007));
#18290=CARTESIAN_POINT('Ctrl Pts',(18.9149565061977,52.2761852868376,-31.7917864972761));
#18291=CARTESIAN_POINT('Ctrl Pts',(18.1665398557866,51.9194196834934,-31.7391369895453));
#18292=CARTESIAN_POINT('Ctrl Pts',(17.6112730416973,51.1574677276187,-31.6864874818145));
#18293=CARTESIAN_POINT('Ctrl Pts',(17.5008778302588,50.3357487515487,-31.6338379740837));
#18294=CARTESIAN_POINT('Ctrl Pts',(17.3904826188202,49.5140297754786,-31.5811884663529));
#18295=CARTESIAN_POINT('Ctrl Pts',(17.7249590100325,48.6325437792133,-31.528538958622));
#18296=CARTESIAN_POINT('Ctrl Pts',(18.3526772182592,48.0908990345672,-31.4758894508912));
#18297=CARTESIAN_POINT('Ctrl Pts',(18.980395426486,47.5492542899211,-31.4232399431604));
#18298=CARTESIAN_POINT('Ctrl Pts',(19.9013554517273,47.3474507968943,-31.3705904354295));
#18299=CARTESIAN_POINT('Ctrl Pts',(20.6980540714064,47.5769731002625,-31.3179409276987));
#18300=CARTESIAN_POINT('Ctrl Pts',(21.4947526910856,47.8064954036307,-31.2652914199679));
#18301=CARTESIAN_POINT('Ctrl Pts',(22.1671899052026,48.467343503394,-31.2126419122371));
#18302=CARTESIAN_POINT('Ctrl Pts',(22.4105265283643,49.2599319629178,-31.1599924045063));
#18303=CARTESIAN_POINT('Ctrl Pts',(22.4835653296022,49.4978316682992,-31.1441893705015));
#18304=CARTESIAN_POINT('Ctrl Pts',(22.5179450581875,49.7476002926395,-31.1283863364967));
#18305=CARTESIAN_POINT('Ctrl Pts',(22.5159430076381,49.9979064240735,-31.112583302492));
#18306=CARTESIAN_POINT('Ctrl Pts',(22.5135563364326,50.0003713189448,-31.387416697508));
#18307=CARTESIAN_POINT('Ctrl Pts',(22.5129693543042,49.5591866004592,-31.4152043808743));
#18308=CARTESIAN_POINT('Ctrl Pts',(22.4023771380614,49.1177266735126,-31.4429920642405));
#18309=CARTESIAN_POINT('Ctrl Pts',(22.1835122430109,48.7388049647084,-31.4707797476067));
#18310=CARTESIAN_POINT('Ctrl Pts',(21.7688274766669,48.0208594931794,-31.5234292553375));
#18311=CARTESIAN_POINT('Ctrl Pts',(20.9654531925725,47.5274207958285,-31.5760787630683));
#18312=CARTESIAN_POINT('Ctrl Pts',(20.1375869056597,47.4821818024699,-31.6287282707992));
#18313=CARTESIAN_POINT('Ctrl Pts',(19.309720618747,47.4369428091112,-31.68137777853));
#18314=CARTESIAN_POINT('Ctrl Pts',(18.457362329016,47.8399035197448,-31.7340272862608));
#18315=CARTESIAN_POINT('Ctrl Pts',(17.9669157054634,48.508387823953,-31.7866767939917));
#18316=CARTESIAN_POINT('Ctrl Pts',(17.4764690819109,49.1768721281611,-31.8393263017225));
#18317=CARTESIAN_POINT('Ctrl Pts',(17.3479341245368,50.1108800259438,-31.8919758094533));
#18318=CARTESIAN_POINT('Ctrl Pts',(17.6395802016597,50.8869932401243,-31.9446253171841));
#18319=CARTESIAN_POINT('Ctrl Pts',(17.9312262787826,51.6631064543048,-31.9972748249149));
#18320=CARTESIAN_POINT('Ctrl Pts',(18.6430533904026,52.2813249848831,-32.0499243326458));
#18321=CARTESIAN_POINT('Ctrl Pts',(19.4523655400881,52.4613888621549,-32.1025738403766));
#18322=CARTESIAN_POINT('Ctrl Pts',(20.2616776897736,52.6414527394267,-32.1552233481074));
#18323=CARTESIAN_POINT('Ctrl Pts',(21.1684748775248,52.3833619633919,-32.2078728558382));
#18324=CARTESIAN_POINT('Ctrl Pts',(21.7616743877694,51.8041180626279,-32.2605223635691));
#18325=CARTESIAN_POINT('Ctrl Pts',(22.2382452047924,51.3387590488808,-32.302820474882));
#18326=CARTESIAN_POINT('Ctrl Pts',(22.5124087275473,50.6661161816974,-32.345118586195));
#18327=CARTESIAN_POINT('Ctrl Pts',(22.518438676647,49.9978466804791,-32.387416697508));
#18328=CARTESIAN_POINT('Origin',(20.,50.,-32.));
#18329=CARTESIAN_POINT('',(22.519890696217,50.0017467019843,-33.387416697508));
#18330=CARTESIAN_POINT('',(22.5147220745132,50.001651275808,-33.112583302492));
#18331=CARTESIAN_POINT('',(22.5175,50.,-32.));
#18332=CARTESIAN_POINT('Ctrl Pts',(22.5147220745132,50.001651275808,-33.112583302492));
#18333=CARTESIAN_POINT('Ctrl Pts',(22.5165646035554,50.3040663516863,-33.0935137626));
#18334=CARTESIAN_POINT('Ctrl Pts',(22.4660534290505,50.6058866921801,-33.0744442227079));
#18335=CARTESIAN_POINT('Ctrl Pts',(22.3604198375119,50.8869932548441,-33.0553746828159));
#18336=CARTESIAN_POINT('Ctrl Pts',(22.0687737555491,51.6631064819043,-33.0027251750851));
#18337=CARTESIAN_POINT('Ctrl Pts',(21.3569466321163,52.2813250227421,-32.9500756673542));
#18338=CARTESIAN_POINT('Ctrl Pts',(20.5476344690001,52.4613889030021,-32.8974261596234));
#18339=CARTESIAN_POINT('Ctrl Pts',(19.7383223058839,52.6414527832621,-32.8447766518926));
#18340=CARTESIAN_POINT('Ctrl Pts',(18.8315251030843,52.3833620029443,-32.7921271441618));
#18341=CARTESIAN_POINT('Ctrl Pts',(18.2383255829953,51.8041180925676,-32.739477636431));
#18342=CARTESIAN_POINT('Ctrl Pts',(17.6451260629064,51.224874182191,-32.6868281287001));
#18343=CARTESIAN_POINT('Ctrl Pts',(17.3655242255282,50.3244771417555,-32.6341786209693));
#18344=CARTESIAN_POINT('Ctrl Pts',(17.5262733119833,49.5111082773736,-32.5815291132385));
#18345=CARTESIAN_POINT('Ctrl Pts',(17.6870223984385,48.6977394129917,-32.5288796055077));
#18346=CARTESIAN_POINT('Ctrl Pts',(18.2881224087269,47.9713987246632,-32.4762300977768));
#18347=CARTESIAN_POINT('Ctrl Pts',(19.0570737939997,47.6613617181153,-32.423580590046));
#18348=CARTESIAN_POINT('Ctrl Pts',(19.8260251792725,47.3513247115674,-32.3709310823152));
#18349=CARTESIAN_POINT('Ctrl Pts',(20.7628279395296,47.4575913867999,-32.3182815745844));
#18350=CARTESIAN_POINT('Ctrl Pts',(21.4427967891924,47.9319873625737,-32.2656320668535));
#18351=CARTESIAN_POINT('Ctrl Pts',(22.1016721629015,48.3916669875728,-32.2146158120664));
#18352=CARTESIAN_POINT('Ctrl Pts',(22.5194010823779,49.1969905165226,-32.1635995572792));
#18353=CARTESIAN_POINT('Ctrl Pts',(22.5214653521749,50.000465985833,-32.112583302492));
#18354=CARTESIAN_POINT('Ctrl Pts',(22.518438676647,49.9978466804791,-32.387416697508));
#18355=CARTESIAN_POINT('Ctrl Pts',(22.5199143546754,49.8343045669821,-32.3977680939259));
#18356=CARTESIAN_POINT('Ctrl Pts',(22.5053314531976,49.6710243753477,-32.4081194903437));
#18357=CARTESIAN_POINT('Ctrl Pts',(22.4737266469647,49.5111082854868,-32.4184708867615));
#18358=CARTESIAN_POINT('Ctrl Pts',(22.3129775631772,48.6977394346029,-32.4711203944923));
#18359=CARTESIAN_POINT('Ctrl Pts',(21.7118775628641,47.9713987583282,-32.5237699022232));
#18360=CARTESIAN_POINT('Ctrl Pts',(20.9429261903522,47.6613617569254,-32.576419409954));
#18361=CARTESIAN_POINT('Ctrl Pts',(20.1739748178403,47.3513247555226,-32.6290689176848));
#18362=CARTESIAN_POINT('Ctrl Pts',(19.2371720731297,47.4575914289917,-32.6817184254156));
#18363=CARTESIAN_POINT('Ctrl Pts',(18.5572032347511,47.9319873968928,-32.7343679331465));
#18364=CARTESIAN_POINT('Ctrl Pts',(17.8772343963725,48.4063833647939,-32.7870174408773));
#18365=CARTESIAN_POINT('Ctrl Pts',(17.4540994643259,49.2489086271271,-32.8396669486081));
#18366=CARTESIAN_POINT('Ctrl Pts',(17.4796202255211,50.0776171683373,-32.8923164563389));
#18367=CARTESIAN_POINT('Ctrl Pts',(17.5051409867163,50.9063257095475,-32.9449659640698));
#18368=CARTESIAN_POINT('Ctrl Pts',(17.9793174411532,51.7212175296348,-32.9976154718006));
#18369=CARTESIAN_POINT('Ctrl Pts',(18.6871889039254,52.1528738138698,-33.0502649795314));
#18370=CARTESIAN_POINT('Ctrl Pts',(19.3950603666975,52.5845300981048,-33.1029144872622));
#18371=CARTESIAN_POINT('Ctrl Pts',(20.3366268378049,52.6329508464875,-33.155563994993));
#18372=CARTESIAN_POINT('Ctrl Pts',(21.0850434757959,52.2761852490638,-33.2082135027239));
#18373=CARTESIAN_POINT('Ctrl Pts',(21.8334601137868,51.9194196516402,-33.2608630104547));
#18374=CARTESIAN_POINT('Ctrl Pts',(22.3887269186614,51.1574677084102,-33.3135125181855));
#18375=CARTESIAN_POINT('Ctrl Pts',(22.4991221282679,50.3357487459767,-33.3661620259163));
#18376=CARTESIAN_POINT('Ctrl Pts',(22.5139776892953,50.2251724244374,-33.3732469164469));
#18377=CARTESIAN_POINT('Ctrl Pts',(22.5207773824235,50.1135138238392,-33.3803318069775));
#18378=CARTESIAN_POINT('Ctrl Pts',(22.519890696217,50.0017467019843,-33.387416697508));
#18379=CARTESIAN_POINT('Origin',(20.,50.,-32.));
#18380=CARTESIAN_POINT('',(22.5135830750733,50.000456715329,-34.387416697508));
#18381=CARTESIAN_POINT('',(22.5158014821082,49.9979396994526,-34.112583302492));
#18382=CARTESIAN_POINT('',(22.5175,50.,-32.));
#18383=CARTESIAN_POINT('Ctrl Pts',(22.5158014821082,49.9979396994526,-34.112583302492));
#18384=CARTESIAN_POINT('Ctrl Pts',(22.5112690113793,50.5762422161602,-34.0760774756516));
#18385=CARTESIAN_POINT('Ctrl Pts',(22.3128670252218,51.1573545057524,-34.0395716488111));
#18386=CARTESIAN_POINT('Ctrl Pts',(21.9477707270638,51.6014143868006,-34.0030658219707));
#18387=CARTESIAN_POINT('Ctrl Pts',(21.421220802407,52.241847330352,-33.9504163142399));
#18388=CARTESIAN_POINT('Ctrl Pts',(20.5479459775285,52.5972106629057,-33.897766806509));
#18389=CARTESIAN_POINT('Ctrl Pts',(19.7238321145605,52.506405821592,-33.8451172987782));
#18390=CARTESIAN_POINT('Ctrl Pts',(18.8997182515924,52.4156009802783,-33.7924677910474));
#18391=CARTESIAN_POINT('Ctrl Pts',(18.1247653505348,51.8786279650973,-33.7398182833166));
#18392=CARTESIAN_POINT('Ctrl Pts',(17.7502865245185,51.1389153268333,-33.6871687755857));
#18393=CARTESIAN_POINT('Ctrl Pts',(17.3758076985023,50.3992026885692,-33.6345192678549));
#18394=CARTESIAN_POINT('Ctrl Pts',(17.4018029475274,49.456750427222,-33.5818697601241));
#18395=CARTESIAN_POINT('Ctrl Pts',(17.8164877207532,48.7388049437786,-33.5292202523933));
#18396=CARTESIAN_POINT('Ctrl Pts',(18.2311724939791,48.0208594603352,-33.4765707446625));
#18397=CARTESIAN_POINT('Ctrl Pts',(19.0345467914056,47.5274207547956,-33.4239212369316));
#18398=CARTESIAN_POINT('Ctrl Pts',(19.8624130920569,47.4821817606862,-33.3712717292008));
#18399=CARTESIAN_POINT('Ctrl Pts',(20.6902793927082,47.4369427665768,-33.31862222147));
#18400=CARTESIAN_POINT('Ctrl Pts',(21.5426376965843,47.8399034838976,-33.2659727137392));
#18401=CARTESIAN_POINT('Ctrl Pts',(22.0330843282759,48.5083877991994,-33.2133232060084));
#18402=CARTESIAN_POINT('Ctrl Pts',(22.345892231496,48.9347485151121,-33.1797432381696));
#18403=CARTESIAN_POINT('Ctrl Pts',(22.5114775250207,49.4691219867189,-33.1461632703308));
#18404=CARTESIAN_POINT('Ctrl Pts',(22.5147220745132,50.001651275808,-33.112583302492));
#18405=CARTESIAN_POINT('Ctrl Pts',(22.519890696217,50.0017467019843,-33.387416697508));
#18406=CARTESIAN_POINT('Ctrl Pts',(22.5141882061925,49.2829457408508,-33.4329813147083));
#18407=CARTESIAN_POINT('Ctrl Pts',(22.1905707471301,48.5596562513103,-33.4785459319085));
#18408=CARTESIAN_POINT('Ctrl Pts',(21.6473227544031,48.0908990662491,-33.5241105491088));
#18409=CARTESIAN_POINT('Ctrl Pts',(21.0196045565934,47.5492543305917,-33.5767600568396));
#18410=CARTESIAN_POINT('Ctrl Pts',(20.0986445466357,47.3474508409138,-33.6294095645704));
#18411=CARTESIAN_POINT('Ctrl Pts',(19.3019459401779,47.5769731404731,-33.6820590723013));
#18412=CARTESIAN_POINT('Ctrl Pts',(18.5052473337201,47.8064954400324,-33.7347085800321));
#18413=CARTESIAN_POINT('Ctrl Pts',(17.8328101307623,48.4673435288288,-33.7873580877629));
#18414=CARTESIAN_POINT('Ctrl Pts',(17.5894735116388,49.2599319751995,-33.8400075954937));
#18415=CARTESIAN_POINT('Ctrl Pts',(17.3461368925154,50.0525204215702,-33.8926571032246));
#18416=CARTESIAN_POINT('Ctrl Pts',(17.5319008572263,50.9768492255152,-33.9453066109554));
#18417=CARTESIAN_POINT('Ctrl Pts',(18.0625521372478,51.613887979861,-33.9979561186862));
#18418=CARTESIAN_POINT('Ctrl Pts',(18.5932034172692,52.2509267342067,-34.050605626417));
#18419=CARTESIAN_POINT('Ctrl Pts',(19.468742012601,52.6006754389532,-34.1032551341478));
#18420=CARTESIAN_POINT('Ctrl Pts',(20.292255815201,52.5045808373667,-34.1559046418787));
#18421=CARTESIAN_POINT('Ctrl Pts',(21.115769617801,52.4084862357801,-34.2085541496095));
#18422=CARTESIAN_POINT('Ctrl Pts',(21.8872586276691,51.8665483278603,-34.2612036573403));
#18423=CARTESIAN_POINT('Ctrl Pts',(22.2569800340703,51.1244464230148,-34.3138531650711));
#18424=CARTESIAN_POINT('Ctrl Pts',(22.4291754564946,50.7788171227519,-34.3383743425501));
#18425=CARTESIAN_POINT('Ctrl Pts',(22.5142205709798,50.3897688065706,-34.3628955200291));
#18426=CARTESIAN_POINT('Ctrl Pts',(22.5135830750733,50.000456715329,-34.387416697508));
#18427=CARTESIAN_POINT('Origin',(20.,50.,-32.));
#18428=CARTESIAN_POINT('',(22.5182787891679,49.9978231920092,-35.387416697508));
#18429=CARTESIAN_POINT('',(22.5215054096331,50.0003700141344,-35.112583302492));
#18430=CARTESIAN_POINT('',(22.5175,50.,-32.));
#18431=CARTESIAN_POINT('Ctrl Pts',(22.5215054096331,50.0003700141344,-35.112583302492));
#18432=CARTESIAN_POINT('Ctrl Pts',(22.5215475819598,50.0207269166612,-35.111290696434));
#18433=CARTESIAN_POINT('Ctrl Pts',(22.5213221499952,50.0410828615022,-35.109998090376));
#18434=CARTESIAN_POINT('Ctrl Pts',(22.5208262388437,50.0614322147998,-35.108705484318));
#18435=CARTESIAN_POINT('Ctrl Pts',(22.500627139634,50.890287554852,-35.0560559765872));
#18436=CARTESIAN_POINT('Ctrl Pts',(22.0316928715497,51.7082072759168,-35.0034064688563));
#18437=CARTESIAN_POINT('Ctrl Pts',(21.3266076540305,52.1443999104008,-34.9507569611255));
#18438=CARTESIAN_POINT('Ctrl Pts',(20.6215224365114,52.5805925448848,-34.8981074533947));
#18439=CARTESIAN_POINT('Ctrl Pts',(19.6802862695575,52.635058092788,-34.8454579456639));
#18440=CARTESIAN_POINT('Ctrl Pts',(18.9295942562556,52.2831054262161,-34.792808437933));
#18441=CARTESIAN_POINT('Ctrl Pts',(18.1789022429538,51.9311527596443,-34.7401589302022));
#18442=CARTESIAN_POINT('Ctrl Pts',(17.618754383304,51.1727818785975,-34.6875094224714));
#18443=CARTESIAN_POINT('Ctrl Pts',(17.5030851914148,50.3517886895942,-34.6348599147406));
#18444=CARTESIAN_POINT('Ctrl Pts',(17.3874159995256,49.5307955005909,-34.5822104070097));
#18445=CARTESIAN_POINT('Ctrl Pts',(17.7162254753971,48.6471800036312,-34.5295608992789));
#18446=CARTESIAN_POINT('Ctrl Pts',(18.340452843287,48.1015158472865,-34.4769113915481));
#18447=CARTESIAN_POINT('Ctrl Pts',(18.9646802111769,47.5558516909418,-34.4242618838173));
#18448=CARTESIAN_POINT('Ctrl Pts',(19.8843254710852,47.3481388752122,-34.3716123760865));
#18449=CARTESIAN_POINT('Ctrl Pts',(20.6824814293057,47.5725408464587,-34.3189628683556));
#18450=CARTESIAN_POINT('Ctrl Pts',(21.4806373875261,47.7969428177052,-34.2663133606248));
#18451=CARTESIAN_POINT('Ctrl Pts',(22.1573040440586,48.4534595759279,-34.213663852894));
#18452=CARTESIAN_POINT('Ctrl Pts',(22.4057248601073,49.2444692323139,-34.1610143451632));
#18453=CARTESIAN_POINT('Ctrl Pts',(22.4818970135361,49.4870129525554,-34.1448706642728));
#18454=CARTESIAN_POINT('Ctrl Pts',(22.5178058405196,49.7422015859551,-34.1287269833824));
#18455=CARTESIAN_POINT('Ctrl Pts',(22.5158014821082,49.9979396994526,-34.112583302492));
#18456=CARTESIAN_POINT('Ctrl Pts',(22.5135830750733,50.000456715329,-34.387416697508));
#18457=CARTESIAN_POINT('Ctrl Pts',(22.5128518012425,49.5538754252223,-34.4155450277599));
#18458=CARTESIAN_POINT('Ctrl Pts',(22.3993753556208,49.1069470475986,-34.4436733580117));
#18459=CARTESIAN_POINT('Ctrl Pts',(22.1753690989929,48.7248106354076,-34.4718016882636));
#18460=CARTESIAN_POINT('Ctrl Pts',(21.7560829545797,48.0095426544173,-34.5244511959944));
#18461=CARTESIAN_POINT('Ctrl Pts',(20.9495568628189,47.521272594208,-34.5771007037253));
#18462=CARTESIAN_POINT('Ctrl Pts',(20.121417162719,47.4813502615447,-34.6297502114561));
#18463=CARTESIAN_POINT('Ctrl Pts',(19.2932774626192,47.4414279288815,-34.6823997191869));
#18464=CARTESIAN_POINT('Ctrl Pts',(18.4435241541804,47.8498533237643,-34.7350492269177));
#18465=CARTESIAN_POINT('Ctrl Pts',(17.9573799777439,48.5214730042706,-34.7876987346485));
#18466=CARTESIAN_POINT('Ctrl Pts',(17.4712358013075,49.1930926847769,-34.8403482423793));
#18467=CARTESIAN_POINT('Ctrl Pts',(17.3487007568734,50.1279066509067,-34.8929977501102));
#18468=CARTESIAN_POINT('Ctrl Pts',(17.6453242434686,50.9021312066576,-34.945647257841));
#18469=CARTESIAN_POINT('Ctrl Pts',(17.9419477300637,51.6763557624084,-34.9982967655718));
#18470=CARTESIAN_POINT('Ctrl Pts',(18.6577297476881,52.2899909077803,-35.0509462733026));
#18471=CARTESIAN_POINT('Ctrl Pts',(19.4681814034145,52.4648544810502,-35.1035957810335));
#18472=CARTESIAN_POINT('Ctrl Pts',(20.2786330591408,52.6397180543201,-35.1562452887643));
#18473=CARTESIAN_POINT('Ctrl Pts',(21.1837543529692,52.375810055488,-35.2088947964951));
#18474=CARTESIAN_POINT('Ctrl Pts',(21.7732223103528,51.7927691626316,-35.261544304226));
#18475=CARTESIAN_POINT('Ctrl Pts',(22.2429813246144,51.3281320069191,-35.3035017686533));
#18476=CARTESIAN_POINT('Ctrl Pts',(22.5122745698353,50.6608192775936,-35.3454592330807));
#18477=CARTESIAN_POINT('Ctrl Pts',(22.5182787891679,49.9978231920092,-35.387416697508));
#18478=CARTESIAN_POINT('Origin',(20.,50.,-32.));
#18479=CARTESIAN_POINT('',(22.5200280234191,50.0016863229039,-36.387416697508));
#18480=CARTESIAN_POINT('',(22.5148335005971,50.0017093727271,-36.112583302492));
#18481=CARTESIAN_POINT('',(22.5175,50.,-32.));
#18482=CARTESIAN_POINT('Ctrl Pts',(22.5148335005971,50.0017093727271,-36.112583302492));
#18483=CARTESIAN_POINT('Ctrl Pts',(22.5167121752117,50.29868917153,-36.0938544094856));
#18484=CARTESIAN_POINT('Ctrl Pts',(22.4680382958723,50.5950732095141,-36.0751255164792));
#18485=CARTESIAN_POINT('Ctrl Pts',(22.3660665601341,50.8718187176302,-36.0563966234728));
#18486=CARTESIAN_POINT('Ctrl Pts',(22.0794099121816,51.6497886042672,-36.0037471157419));
#18487=CARTESIAN_POINT('Ctrl Pts',(21.3715670432168,52.2725650414812,-35.9510976080111));
#18488=CARTESIAN_POINT('Ctrl Pts',(20.5634277538184,52.4578218018643,-35.8984481002803));
#18489=CARTESIAN_POINT('Ctrl Pts',(19.7552884644201,52.6430785622474,-35.8457985925495));
#18490=CARTESIAN_POINT('Ctrl Pts',(18.8468527545881,52.3908156457995,-35.7931490848187));
#18491=CARTESIAN_POINT('Ctrl Pts',(18.2499461389797,51.8153926095982,-35.7404995770879));
#18492=CARTESIAN_POINT('Ctrl Pts',(17.6530395233712,51.239969573397,-35.687850069357));
#18493=CARTESIAN_POINT('Ctrl Pts',(17.3676620019863,50.3413864174424,-35.6352005616262));
#18494=CARTESIAN_POINT('Ctrl Pts',(17.5231851344541,49.5270021508903,-35.5825510538954));
#18495=CARTESIAN_POINT('Ctrl Pts',(17.6787082669219,48.7126178843383,-35.5299015461645));
#18496=CARTESIAN_POINT('Ctrl Pts',(18.2751320532423,47.9824325071888,-35.4772520384337));
#18497=CARTESIAN_POINT('Ctrl Pts',(19.0420768395959,47.6674644563856,-35.4246025307029));
#18498=CARTESIAN_POINT('Ctrl Pts',(19.8090216259494,47.3524964055824,-35.3719530229721));
#18499=CARTESIAN_POINT('Ctrl Pts',(20.7464874123362,47.4527456811256,-35.3193035152413));
#18500=CARTESIAN_POINT('Ctrl Pts',(21.4294883403622,47.9227657984169,-35.2666540075104));
#18501=CARTESIAN_POINT('Ctrl Pts',(22.0957208089051,48.3812463804461,-35.2152971058376));
#18502=CARTESIAN_POINT('Ctrl Pts',(22.5198298488346,49.1915640867918,-35.1639402041648));
#18503=CARTESIAN_POINT('Ctrl Pts',(22.5215054096331,50.0003700141344,-35.112583302492));
#18504=CARTESIAN_POINT('Ctrl Pts',(22.5182787891679,49.9978231920092,-35.387416697508));
#18505=CARTESIAN_POINT('Ctrl Pts',(22.5198088476208,49.8288715417166,-35.3981087408115));
#18506=CARTESIAN_POINT('Ctrl Pts',(22.5042412842967,49.6602002082423,-35.408800784115));
#18507=CARTESIAN_POINT('Ctrl Pts',(22.4705364786134,49.495234569071,-35.4194928274184));
#18508=CARTESIAN_POINT('Ctrl Pts',(22.3045680685516,48.6829146552474,-35.4721423351492));
#18509=CARTESIAN_POINT('Ctrl Pts',(21.6988166274892,47.9604486144809,-35.5247918428801));
#18510=CARTESIAN_POINT('Ctrl Pts',(20.9278903596849,47.6553554399738,-35.5774413506109));
#18511=CARTESIAN_POINT('Ctrl Pts',(20.1569640918805,47.3502622654666,-35.6300908583417));
#18512=CARTESIAN_POINT('Ctrl Pts',(19.2208629973343,47.4625419572188,-35.6827403660725));
#18513=CARTESIAN_POINT('Ctrl Pts',(18.5439542721414,47.941294224338,-35.7353898738034));
#18514=CARTESIAN_POINT('Ctrl Pts',(17.8670455469485,48.4200464914572,-35.7880393815342));
#18515=CARTESIAN_POINT('Ctrl Pts',(17.4493291911088,49.2652713339433,-35.840688889265));
#18516=CARTESIAN_POINT('Ctrl Pts',(17.4801705624149,50.0937989227362,-35.8933383969958));
#18517=CARTESIAN_POINT('Ctrl Pts',(17.5110119337209,50.9223265115291,-35.9459879047267));
#18518=CARTESIAN_POINT('Ctrl Pts',(17.9904110321727,51.7341568466287,-35.9986374124574));
#18519=CARTESIAN_POINT('Ctrl Pts',(18.7010395666056,52.1612589907602,-36.0512869201883));
#18520=CARTESIAN_POINT('Ctrl Pts',(19.4116681010385,52.5883611348917,-36.1039364279191));
#18521=CARTESIAN_POINT('Ctrl Pts',(20.3535260714527,52.630735088055,-36.15658593565));
#18522=CARTESIAN_POINT('Ctrl Pts',(21.0996364896456,52.2691712633729,-36.2092354433808));
#18523=CARTESIAN_POINT('Ctrl Pts',(21.8457469078385,51.9076074386908,-36.2618849511116));
#18524=CARTESIAN_POINT('Ctrl Pts',(22.3961097738102,51.1421058361633,-36.3145344588424));
#18525=CARTESIAN_POINT('Ctrl Pts',(22.5012264514832,50.3196949656275,-36.3671839665732));
#18526=CARTESIAN_POINT('Ctrl Pts',(22.5146915818506,50.2143466057627,-36.3739282102181));
#18527=CARTESIAN_POINT('Ctrl Pts',(22.5208507388777,50.1080644308405,-36.3806724538631));
#18528=CARTESIAN_POINT('Ctrl Pts',(22.5200280234191,50.0016863229039,-36.387416697508));
#18529=CARTESIAN_POINT('Origin',(20.,50.,-32.));
#18530=CARTESIAN_POINT('',(22.5136153256948,50.0005414263439,-37.387416697508));
#18531=CARTESIAN_POINT('',(22.5156628463169,49.9979761585217,-37.112583302492));
#18532=CARTESIAN_POINT('',(22.5175,50.,-32.));
#18533=CARTESIAN_POINT('Ctrl Pts',(22.5156628463169,49.9979761585217,-37.112583302492));
#18534=CARTESIAN_POINT('Ctrl Pts',(22.5112697173306,50.5709622635485,-37.0764181225372));
#18535=CARTESIAN_POINT('Ctrl Pts',(22.3168705700426,51.146645177931,-37.0402529425824));
#18536=CARTESIAN_POINT('Ctrl Pts',(21.958013252757,51.5888747404873,-37.0040877626276));
#18537=CARTESIAN_POINT('Ctrl Pts',(21.4355864011749,52.2326754571354,-36.9514382548968));
#18538=CARTESIAN_POINT('Ctrl Pts',(20.5646113672267,52.5936387616293,-36.898788747166));
#18539=CARTESIAN_POINT('Ctrl Pts',(19.739931435762,52.5081274263933,-36.8461392394351));
#18540=CARTESIAN_POINT('Ctrl Pts',(18.9152515042972,52.4226160911573,-36.7934897317043));
#18541=CARTESIAN_POINT('Ctrl Pts',(18.1368666753158,51.8906301161915,-36.7408402239735));
#18542=CARTESIAN_POINT('Ctrl Pts',(17.7576458753074,51.1533372547338,-36.6881907162427));
#18543=CARTESIAN_POINT('Ctrl Pts',(17.3784250752991,50.4160443932761,-36.6355412085118));
#18544=CARTESIAN_POINT('Ctrl Pts',(17.3983683042637,49.4734446453265,-36.582891700781));
#18545=CARTESIAN_POINT('Ctrl Pts',(17.8084346021093,48.7528512720282,-36.5302421930502));
#18546=CARTESIAN_POINT('Ctrl Pts',(18.2185008999548,48.0322578987299,-36.4775926853194));
#18547=CARTESIAN_POINT('Ctrl Pts',(19.0186902666813,47.5336709000828,-36.4249431775885));
#18548=CARTESIAN_POINT('Ctrl Pts',(19.8462490214711,47.4831171103322,-36.3722936698577));
#18549=CARTESIAN_POINT('Ctrl Pts',(20.6738077762609,47.4325633205815,-36.3196441621269));
#18550=CARTESIAN_POINT('Ctrl Pts',(21.5287359191141,47.8300427397272,-36.2669946543961));
#18551=CARTESIAN_POINT('Ctrl Pts',(22.0234647770705,48.4953641173301,-36.2143451466653));
#18552=CARTESIAN_POINT('Ctrl Pts',(22.3422048319556,48.9240121919327,-36.1804245319408));
#18553=CARTESIAN_POINT('Ctrl Pts',(22.511430961121,49.4638378961434,-36.1465039172164));
#18554=CARTESIAN_POINT('Ctrl Pts',(22.5148335005971,50.0017093727271,-36.112583302492));
#18555=CARTESIAN_POINT('Ctrl Pts',(22.5200280234191,50.0016863229039,-36.387416697508));
#18556=CARTESIAN_POINT('Ctrl Pts',(22.5144281411516,49.2776147449956,-36.4333219615939));
#18557=CARTESIAN_POINT('Ctrl Pts',(22.1853609537679,48.5490986296555,-36.4792272256798));
#18558=CARTESIAN_POINT('Ctrl Pts',(21.6350304610706,48.0803609647987,-36.5251324897657));
#18559=CARTESIAN_POINT('Ctrl Pts',(21.0038473036104,47.5427579730497,-36.5777819974966));
#18560=CARTESIAN_POINT('Ctrl Pts',(20.0816104993157,47.3468721280956,-36.6304315052273));
#18561=CARTESIAN_POINT('Ctrl Pts',(19.2864020789169,47.5815052956607,-36.6830810129581));
#18562=CARTESIAN_POINT('Ctrl Pts',(18.491193658518,47.8161384632257,-36.735730520689));
#18563=CARTESIAN_POINT('Ctrl Pts',(17.823013622015,48.4812906433099,-36.7883800284198));
#18564=CARTESIAN_POINT('Ctrl Pts',(17.5847712284946,49.2754252164592,-36.8410295361507));
#18565=CARTESIAN_POINT('Ctrl Pts',(17.3465288349741,50.0695597896084,-36.8936790438815));
#18566=CARTESIAN_POINT('Ctrl Pts',(17.5382240844361,50.9926767558226,-36.9463285516123));
#18567=CARTESIAN_POINT('Ctrl Pts',(18.0729548497615,51.6262950631108,-36.9989780593431));
#18568=CARTESIAN_POINT('Ctrl Pts',(18.607685615087,52.2599133703989,-37.0516275670739));
#18569=CARTESIAN_POINT('Ctrl Pts',(19.4854518962758,52.604033018761,-37.1042770748047));
#18570=CARTESIAN_POINT('Ctrl Pts',(20.308331699469,52.5026526245038,-37.1569265825356));
#18571=CARTESIAN_POINT('Ctrl Pts',(21.1312115026622,52.4012722302467,-37.2095760902664));
#18572=CARTESIAN_POINT('Ctrl Pts',(21.8992048278599,51.8543917933704,-37.2622255979972));
#18573=CARTESIAN_POINT('Ctrl Pts',(22.2641535764485,51.1099311920064,-37.314875105728));
#18574=CARTESIAN_POINT('Ctrl Pts',(22.4317649133932,50.7680200683765,-37.3390556363214));
#18575=CARTESIAN_POINT('Ctrl Pts',(22.5143611435832,50.3844329124877,-37.3632361669147));
#18576=CARTESIAN_POINT('Ctrl Pts',(22.5136153256948,50.0005414263439,-37.387416697508));
#18577=CARTESIAN_POINT('Origin',(20.,50.,-32.));
#18578=CARTESIAN_POINT('',(22.51811817366,49.9978011072146,-38.387416697508));
#18579=CARTESIAN_POINT('',(22.5215367446411,50.0002732851607,-38.112583302492));
#18580=CARTESIAN_POINT('',(22.5175,50.,-32.));
#18581=CARTESIAN_POINT('Ctrl Pts',(22.5215367446411,50.0002732851607,-38.112583302492));
#18582=CARTESIAN_POINT('Ctrl Pts',(22.5215600436793,50.0152649335192,-38.1116313433196));
#18583=CARTESIAN_POINT('Ctrl Pts',(22.5214377828025,50.0302561917135,-38.1106793841472));
#18584=CARTESIAN_POINT('Ctrl Pts',(22.5211687992195,50.0452448167457,-38.1097274249749));
#18585=CARTESIAN_POINT('Ctrl Pts',(22.5062922649704,50.8742128569845,-38.057077917244));
#18586=CARTESIAN_POINT('Ctrl Pts',(22.0426193843105,51.6951265643069,-38.0044284095132));
#18587=CARTESIAN_POINT('Ctrl Pts',(21.3403494591696,52.1358375133504,-37.9517789017824));
#18588=CARTESIAN_POINT('Ctrl Pts',(20.6380795340287,52.5765484623939,-37.8991293940516));
#18589=CARTESIAN_POINT('Ctrl Pts',(19.6972125644067,52.6370566531585,-37.8464798863208));
#18590=CARTESIAN_POINT('Ctrl Pts',(18.9442761565781,52.2899314565743,-37.7938303785899));
#18591=CARTESIAN_POINT('Ctrl Pts',(18.1913397487494,51.9428062599901,-37.7411808708591));
#18592=CARTESIAN_POINT('Ctrl Pts',(17.6263339027141,51.1880476760571,-37.6885313631283));
#18593=CARTESIAN_POINT('Ctrl Pts',(17.5053954905343,50.3678141121614,-37.6358818553975));
#18594=CARTESIAN_POINT('Ctrl Pts',(17.3844570783544,49.5475805482657,-37.5832323476667));
#18595=CARTESIAN_POINT('Ctrl Pts',(17.7075861000302,48.6618720044072,-37.5305828399358));
#18596=CARTESIAN_POINT('Ctrl Pts',(18.3282968953505,48.112210939538,-37.477933332205));
#18597=CARTESIAN_POINT('Ctrl Pts',(18.9490076906708,47.5625498746688,-37.4252838244742));
#18598=CARTESIAN_POINT('Ctrl Pts',(19.8673002596356,47.3489362887889,-37.3726343167434));
#18599=CARTESIAN_POINT('Ctrl Pts',(20.6668806464798,47.5682086730699,-37.3199848090125));
#18600=CARTESIAN_POINT('Ctrl Pts',(21.4664610333241,47.7874810573509,-37.2673353012817));
#18601=CARTESIAN_POINT('Ctrl Pts',(22.1473292380478,48.4396394117927,-37.2146857935509));
#18602=CARTESIAN_POINT('Ctrl Pts',(22.4008240058016,49.2290376534148,-37.1620362858201));
#18603=CARTESIAN_POINT('Ctrl Pts',(22.4801920952911,49.4761947479739,-37.145551958044));
#18604=CARTESIAN_POINT('Ctrl Pts',(22.517665263511,49.7368053091528,-37.129067630268));
#18605=CARTESIAN_POINT('Ctrl Pts',(22.5156628463169,49.9979761585217,-37.112583302492));
#18606=CARTESIAN_POINT('Ctrl Pts',(22.5136153256948,50.0005414263439,-37.387416697508));
#18607=CARTESIAN_POINT('Ctrl Pts',(22.5127372360958,49.5485663176867,-37.4158856746455));
#18608=CARTESIAN_POINT('Ctrl Pts',(22.3963340756929,49.0961693598541,-37.444354651783));
#18609=CARTESIAN_POINT('Ctrl Pts',(22.1671362634044,48.710868852972,-37.4728236289205));
#18610=CARTESIAN_POINT('Ctrl Pts',(21.7432660297921,47.9983078811531,-37.5254731366513));
#18611=CARTESIAN_POINT('Ctrl Pts',(20.9336213905881,47.5152267033671,-37.5781226443822));
#18612=CARTESIAN_POINT('Ctrl Pts',(20.1052424175224,47.4806226208699,-37.630772152113));
#18613=CARTESIAN_POINT('Ctrl Pts',(19.2768634444567,47.4460185383727,-37.6834216598438));
#18614=CARTESIAN_POINT('Ctrl Pts',(18.4297501375294,47.8598915511643,-37.7360711675746));
#18615=CARTESIAN_POINT('Ctrl Pts',(17.9479284590968,48.5346190298311,-37.7887206753054));
#18616=CARTESIAN_POINT('Ctrl Pts',(17.4661067806642,49.209346508498,-37.8413701830363));
#18617=CARTESIAN_POINT('Ctrl Pts',(17.3495767307262,50.1449284530401,-37.8940196907671));
#18618=CARTESIAN_POINT('Ctrl Pts',(17.6511653825088,50.9172322053898,-37.9466691984979));
#18619=CARTESIAN_POINT('Ctrl Pts',(17.9527540342914,51.6895359577395,-37.9993187062287));
#18620=CARTESIAN_POINT('Ctrl Pts',(18.6724613877946,52.2985615178968,-38.0519682139595));
#18621=CARTESIAN_POINT('Ctrl Pts',(19.4840191639997,52.4682180234673,-38.1046177216904));
#18622=CARTESIAN_POINT('Ctrl Pts',(20.2955769402048,52.6378745290377,-38.1572672294212));
#18623=CARTESIAN_POINT('Ctrl Pts',(21.1989851391119,52.3681619800214,-38.209916737152));
#18624=CARTESIAN_POINT('Ctrl Pts',(21.7846971822037,51.7813472460311,-38.2625662448829));
#18625=CARTESIAN_POINT('Ctrl Pts',(22.2476734241463,51.3174993817714,-38.3041830624246));
#18626=CARTESIAN_POINT('Ctrl Pts',(22.5121494139052,50.6555223852163,-38.3457998799663));
#18627=CARTESIAN_POINT('Ctrl Pts',(22.51811817366,49.9978011072146,-38.387416697508));
#18628=CARTESIAN_POINT('Origin',(20.,50.,-32.));
#18629=CARTESIAN_POINT('',(22.5201576955115,50.0015647648602,-39.387416697508));
#18630=CARTESIAN_POINT('',(22.5149457203491,50.0017607375679,-39.112583302492));
#18631=CARTESIAN_POINT('',(22.5175,50.,-32.));
#18632=CARTESIAN_POINT('',(18.086534003335,51.635987203375,-40.));
#18633=CARTESIAN_POINT('Ctrl Pts',(22.5201576955115,50.0015647648602,-39.387416697508));
#18634=CARTESIAN_POINT('Ctrl Pts',(22.5146850116671,49.2723762340521,-39.4336626084796));
#18635=CARTESIAN_POINT('Ctrl Pts',(22.1801325379537,48.5389628969671,-39.4799085194511));
#18636=CARTESIAN_POINT('Ctrl Pts',(21.6226859420216,48.0701217693743,-39.5261544304226));
#18637=CARTESIAN_POINT('Ctrl Pts',(20.9880506143681,47.5363609664587,-39.5788039381534));
#18638=CARTESIAN_POINT('Ctrl Pts',(20.0645199255084,47.34551492175,-39.6314534458842));
#18639=CARTESIAN_POINT('Ctrl Pts',(19.2708509938193,47.5857187771834,-39.6841029536151));
#18640=CARTESIAN_POINT('Ctrl Pts',(18.4771820621302,47.8259226326167,-39.7367524613459));
#18641=CARTESIAN_POINT('Ctrl Pts',(17.8133748876117,48.4971763881921,-39.7894019690767));
#18642=CARTESIAN_POINT('Ctrl Pts',(17.5804140263325,49.2914457293263,-39.8420514768075));
#18643=CARTESIAN_POINT('Ctrl Pts',(17.3474531650532,50.0857150704605,-39.8947009845383));
#18644=CARTESIAN_POINT('Ctrl Pts',(17.5453386170133,51.0029999971535,-39.9473504922692));
#18645=CARTESIAN_POINT('Ctrl Pts',(18.086534003335,51.635987203375,-40.));
#18646=CARTESIAN_POINT('',(21.9170726842248,51.6385409294649,-40.));
#18647=CARTESIAN_POINT('Origin',(20.,50.,-40.));
#18648=CARTESIAN_POINT('Ctrl Pts',(21.9170801928212,51.6385462459494,-40.));
#18649=CARTESIAN_POINT('Ctrl Pts',(21.3942483348109,52.247316763458,-39.9490537266974));
#18650=CARTESIAN_POINT('Ctrl Pts',(20.554552609146,52.5873620245221,-39.8981074533947));
#18651=CARTESIAN_POINT('Ctrl Pts',(19.7559044863995,52.5095731650181,-39.847161180092));
#18652=CARTESIAN_POINT('Ctrl Pts',(18.9305559812605,52.4291836704717,-39.7945116723612));
#18653=CARTESIAN_POINT('Ctrl Pts',(18.1490455625112,51.9025550055059,-39.7418621646304));
#18654=CARTESIAN_POINT('Ctrl Pts',(17.765166694843,51.1677991047107,-39.6892126568996));
#18655=CARTESIAN_POINT('Ctrl Pts',(17.3812878271748,50.4330432039155,-39.6365631491687));
#18656=CARTESIAN_POINT('Ctrl Pts',(17.3950405105878,49.490160067291,-39.5839136414379));
#18657=CARTESIAN_POINT('Ctrl Pts',(17.8004371569179,48.766905015811,-39.5312641337071));
#18658=CARTESIAN_POINT('Ctrl Pts',(18.2058338032481,48.0436499643311,-39.4786146259763));
#18659=CARTESIAN_POINT('Ctrl Pts',(19.0028744124954,47.5400229979957,-39.4259651182455));
#18660=CARTESIAN_POINT('Ctrl Pts',(19.8301087131647,47.484178338697,-39.3733156105146));
#18661=CARTESIAN_POINT('Ctrl Pts',(20.657343013834,47.4283336793982,-39.3206661027838));
#18662=CARTESIAN_POINT('Ctrl Pts',(21.5147710059253,47.8202713271361,-39.268016595053));
#18663=CARTESIAN_POINT('Ctrl Pts',(22.0137530473082,48.4823913654697,-39.2153670873221));
#18664=CARTESIAN_POINT('Ctrl Pts',(22.3384617672062,48.9132608802729,-39.1811058257121));
#18665=CARTESIAN_POINT('Ctrl Pts',(22.5113809799459,49.4585433263153,-39.146844564102));
#18666=CARTESIAN_POINT('Ctrl Pts',(22.5149457203491,50.0017607375679,-39.112583302492));
#18667=CARTESIAN_POINT('Origin',(20.,-50.,-32.));
#18668=CARTESIAN_POINT('',(22.5134613473905,-49.9997270421583,-25.387416697508));
#18669=CARTESIAN_POINT('',(22.5157642476295,-50.0033830516534,-25.112583302492));
#18670=CARTESIAN_POINT('',(22.5175,-50.,-32.));
#18671=CARTESIAN_POINT('',(21.9134659966651,-48.3640127966251,-25.));
#18672=CARTESIAN_POINT('Ctrl Pts',(22.5157642476295,-50.0033830516534,-25.112583302492));
#18673=CARTESIAN_POINT('Ctrl Pts',(22.5105545148632,-49.4108213760461,-25.0750555349946));
#18674=CARTESIAN_POINT('Ctrl Pts',(22.2992218280841,-48.8151964396956,-25.0375277674973));
#18675=CARTESIAN_POINT('Ctrl Pts',(21.9134659966651,-48.3640127966251,-25.));
#18676=CARTESIAN_POINT('',(22.5175,-50.,-25.));
#18677=CARTESIAN_POINT('Origin',(20.,-50.,-25.));
#18678=CARTESIAN_POINT('',(17.4825,-50.,-25.));
#18679=CARTESIAN_POINT('Ctrl Pts',(22.5175,-50.,-25.));
#18680=CARTESIAN_POINT('Ctrl Pts',(22.5175,-49.6777819917977,-25.));
#18681=CARTESIAN_POINT('Ctrl Pts',(22.4519182005811,-49.3379042845385,-24.965994767533));
#18682=CARTESIAN_POINT('Ctrl Pts',(22.1930921359231,-48.7191330360028,-24.8434341672334));
#18683=CARTESIAN_POINT('Ctrl Pts',(22.0001401774783,-48.439857534204,-24.75619390213));
#18684=CARTESIAN_POINT('Ctrl Pts',(21.5595215410958,-47.9992388978215,-24.5883213994305));
#18685=CARTESIAN_POINT('Ctrl Pts',(21.2804542351089,-47.8067418484832,-24.4956547875015));
#18686=CARTESIAN_POINT('Ctrl Pts',(20.6625974062016,-47.5482850278898,-24.3600905047278));
#18687=CARTESIAN_POINT('Ctrl Pts',(20.3231274362054,-47.4825,-24.3199761284063));
#18688=CARTESIAN_POINT('Ctrl Pts',(20.,-47.4825,-24.3199761284063));
#18689=CARTESIAN_POINT('Ctrl Pts',(19.6768725637946,-47.4825,-24.3199761284063));
#18690=CARTESIAN_POINT('Ctrl Pts',(19.3374025937983,-47.5482850278898,-24.3600905047278));
#18691=CARTESIAN_POINT('Ctrl Pts',(18.719545764891,-47.8067418484832,-24.4956547875015));
#18692=CARTESIAN_POINT('Ctrl Pts',(18.4404784589043,-47.9992388978215,-24.5883213994305));
#18693=CARTESIAN_POINT('Ctrl Pts',(17.9998598225217,-48.439857534204,-24.75619390213));
#18694=CARTESIAN_POINT('Ctrl Pts',(17.8069078640769,-48.7191330360028,-24.8434341672334));
#18695=CARTESIAN_POINT('Ctrl Pts',(17.5480817994189,-49.3379042845386,-24.965994767533));
#18696=CARTESIAN_POINT('Ctrl Pts',(17.4825,-49.6777819917977,-25.));
#18697=CARTESIAN_POINT('Ctrl Pts',(17.4825,-50.,-25.));
#18698=CARTESIAN_POINT('',(18.0829272567075,-48.3614591395872,-25.));
#18699=CARTESIAN_POINT('Origin',(20.,-50.,-25.));
#18700=CARTESIAN_POINT('Ctrl Pts',(18.082919744614,-48.3614538208575,-25.));
#18701=CARTESIAN_POINT('Ctrl Pts',(18.6057515849863,-47.7526833829372,-25.0509462733027));
#18702=CARTESIAN_POINT('Ctrl Pts',(19.4454473582538,-47.4126378852296,-25.1018925466053));
#18703=CARTESIAN_POINT('Ctrl Pts',(20.2440955154214,-47.4904266963984,-25.152838819908));
#18704=CARTESIAN_POINT('Ctrl Pts',(21.0694440561323,-47.5708161409938,-25.2054883276388));
#18705=CARTESIAN_POINT('Ctrl Pts',(21.8509544963761,-48.0974449571186,-25.2581378353696));
#18706=CARTESIAN_POINT('Ctrl Pts',(22.234833370557,-48.8322009067204,-25.3107873431004));
#18707=CARTESIAN_POINT('Ctrl Pts',(22.4210737335855,-49.188670678815,-25.3363304612363));
#18708=CARTESIAN_POINT('Ctrl Pts',(22.5137218121911,-49.5941282464848,-25.3618735793722));
#18709=CARTESIAN_POINT('Ctrl Pts',(22.5134613473905,-49.9997270421583,-25.387416697508));
#18710=CARTESIAN_POINT('Origin',(20.,-50.,-32.));
#18711=CARTESIAN_POINT('',(22.51875591101,-50.0020955263397,-26.387416697508));
#18712=CARTESIAN_POINT('',(22.5213592474396,-49.9993296992679,-26.112583302492));
#18713=CARTESIAN_POINT('',(22.5175,-50.,-32.));
#18714=CARTESIAN_POINT('Ctrl Pts',(22.5213592474396,-49.9993296992679,-26.112583302492));
#18715=CARTESIAN_POINT('Ctrl Pts',(22.5214870426669,-49.9628733533498,-26.1102687557771));
#18716=CARTESIAN_POINT('Ctrl Pts',(22.5207640617796,-49.9264222613598,-26.1079542090622));
#18717=CARTESIAN_POINT('Ctrl Pts',(22.5191744259947,-49.8900090854379,-26.1056396623473));
#18718=CARTESIAN_POINT('Ctrl Pts',(22.4830146280504,-49.0617104925164,-26.0529901546164));
#18719=CARTESIAN_POINT('Ctrl Pts',(21.9984162961223,-48.253031042163,-26.0003406468856));
#18720=CARTESIAN_POINT('Ctrl Pts',(21.2850581295563,-47.8304728873339,-25.9476911391548));
#18721=CARTESIAN_POINT('Ctrl Pts',(20.5716999629903,-47.4079147325048,-25.895041631424));
#18722=CARTESIAN_POINT('Ctrl Pts',(19.6295819617865,-47.3714778732001,-25.8423921236932));
#18723=CARTESIAN_POINT('Ctrl Pts',(18.8858121000221,-47.7378802757919,-25.7897426159623));
#18724=CARTESIAN_POINT('Ctrl Pts',(18.1420422382578,-48.1042826783837,-25.7370931082315));
#18725=CARTESIAN_POINT('Ctrl Pts',(17.5966205159329,-48.8735243428719,-25.6844436005007));
#18726=CARTESIAN_POINT('Ctrl Pts',(17.4967795653299,-49.6964831019948,-25.6317940927699));
#18727=CARTESIAN_POINT('Ctrl Pts',(17.3969386147268,-50.5194418611176,-25.5791445850391));
#18728=CARTESIAN_POINT('Ctrl Pts',(17.7426784358456,-51.3961177148752,-25.5264950773082));
#18729=CARTESIAN_POINT('Ctrl Pts',(18.3773138867814,-51.9298784728165,-25.4738455695774));
#18730=CARTESIAN_POINT('Ctrl Pts',(19.0119493377171,-52.4636392307578,-25.4211960618466));
#18731=CARTESIAN_POINT('Ctrl Pts',(19.9354804184698,-52.654484892883,-25.3685465541157));
#18732=CARTESIAN_POINT('Ctrl Pts',(20.7291491830128,-52.4142811943913,-25.3158970463849));
#18733=CARTESIAN_POINT('Ctrl Pts',(21.5228179475557,-52.1740774958997,-25.2632475386541));
#18734=CARTESIAN_POINT('Ctrl Pts',(22.1866243958889,-51.5028244367913,-25.2105980309233));
#18735=CARTESIAN_POINT('Ctrl Pts',(22.4195852547467,-50.708555063528,-25.1579485231925));
#18736=CARTESIAN_POINT('Ctrl Pts',(22.4864951603479,-50.4804288064068,-25.142826782959));
#18737=CARTESIAN_POINT('Ctrl Pts',(22.5178634992192,-50.2421546154428,-25.1277050427255));
#18738=CARTESIAN_POINT('Ctrl Pts',(22.5157642476295,-50.0033830516534,-25.112583302492));
#18739=CARTESIAN_POINT('Ctrl Pts',(22.5134613473905,-49.9997270421583,-25.387416697508));
#18740=CARTESIAN_POINT('Ctrl Pts',(22.5131849418113,-50.4301490022454,-25.414523087103));
#18741=CARTESIAN_POINT('Ctrl Pts',(22.4082797518455,-50.8607300059878,-25.4416294766979));
#18742=CARTESIAN_POINT('Ctrl Pts',(22.1995628957716,-51.2330949928824,-25.4687358662929));
#18743=CARTESIAN_POINT('Ctrl Pts',(21.7941662386876,-51.9563500463638,-25.5213853740237));
#18744=CARTESIAN_POINT('Ctrl Pts',(20.9971256164018,-52.4599770702478,-25.5740348817545));
#18745=CARTESIAN_POINT('Ctrl Pts',(20.1698912949398,-52.5158217407964,-25.6266843894854));
#18746=CARTESIAN_POINT('Ctrl Pts',(19.3426569734778,-52.5716664113451,-25.6793338972162));
#18747=CARTESIAN_POINT('Ctrl Pts',(18.4852289528396,-52.1797287285584,-25.731983404947));
#18748=CARTESIAN_POINT('Ctrl Pts',(17.9862468973199,-51.5176086672518,-25.7846329126778));
#18749=CARTESIAN_POINT('Ctrl Pts',(17.4872648418001,-50.8554886059452,-25.8372824204087));
#18750=CARTESIAN_POINT('Ctrl Pts',(17.3467287513987,-49.9231861661186,-25.8899319281395));
#18751=CARTESIAN_POINT('Ctrl Pts',(17.6283798121799,-49.1433861673454,-25.9425814358703));
#18752=CARTESIAN_POINT('Ctrl Pts',(17.9100308729611,-48.3635861685722,-25.9952309436011));
#18753=CARTESIAN_POINT('Ctrl Pts',(18.6138690849249,-47.7362886108523,-26.047880451332));
#18754=CARTESIAN_POINT('Ctrl Pts',(19.4208043833602,-47.5458493696428,-26.1005299590628));
#18755=CARTESIAN_POINT('Ctrl Pts',(20.2277396817955,-47.3554101284333,-26.1531794667936));
#18756=CARTESIAN_POINT('Ctrl Pts',(21.1377720667024,-47.6018292037341,-26.2058289745244));
#18757=CARTESIAN_POINT('Ctrl Pts',(21.7383600880492,-48.173406266917,-26.2584784822553));
#18758=CARTESIAN_POINT('Ctrl Pts',(22.2286384775488,-48.6400021230645,-26.3014578873395));
#18759=CARTESIAN_POINT('Ctrl Pts',(22.5127044815768,-49.3232818559675,-26.3444372924237));
#18760=CARTESIAN_POINT('Ctrl Pts',(22.51875591101,-50.0020955263397,-26.387416697508));
#18761=CARTESIAN_POINT('Origin',(20.,-50.,-32.));
#18762=CARTESIAN_POINT('',(22.5196060265899,-49.9981422852793,-27.387416697508));
#18763=CARTESIAN_POINT('',(22.5145120517532,-49.9984719976714,-27.112583302492));
#18764=CARTESIAN_POINT('',(22.5175,-50.,-32.));
#18765=CARTESIAN_POINT('Ctrl Pts',(22.5145120517532,-49.9984719976714,-27.112583302492));
#18766=CARTESIAN_POINT('Ctrl Pts',(22.5162682753667,-49.6851867289941,-27.0928324688287));
#18767=CARTESIAN_POINT('Ctrl Pts',(22.4619721349342,-49.372488283433,-27.0730816351654));
#18768=CARTESIAN_POINT('Ctrl Pts',(22.3488347498514,-49.0827677433124,-27.0533308015021));
#18769=CARTESIAN_POINT('Ctrl Pts',(22.0472460811345,-48.310463947083,-27.0006812937713));
#18770=CARTESIAN_POINT('Ctrl Pts',(21.3275386873248,-47.701438351122,-26.9480317860405));
#18771=CARTESIAN_POINT('Ctrl Pts',(20.515980865224,-47.5317818366054,-26.8953822783096));
#18772=CARTESIAN_POINT('Ctrl Pts',(19.7044230431231,-47.3621253220887,-26.8427327705788));
#18773=CARTESIAN_POINT('Ctrl Pts',(18.8010147927311,-47.6318378890163,-26.790083262848));
#18774=CARTESIAN_POINT('Ctrl Pts',(18.2153027169047,-48.2186526549655,-26.7374337551172));
#18775=CARTESIAN_POINT('Ctrl Pts',(17.6295906410783,-48.8054674209146,-26.6847842473863));
#18776=CARTESIAN_POINT('Ctrl Pts',(17.3615747398177,-49.7093843858853,-26.6321347396555));
#18777=CARTESIAN_POINT('Ctrl Pts',(17.5327555271831,-50.5206201517315,-26.5794852319247));
#18778=CARTESIAN_POINT('Ctrl Pts',(17.7039363145486,-51.3318559175777,-26.5268357241939));
#18779=CARTESIAN_POINT('Ctrl Pts',(18.3143137905401,-52.0504104842994,-26.474186216463));
#18780=CARTESIAN_POINT('Ctrl Pts',(19.0871834427573,-52.3505507840466,-26.4215367087322));
#18781=CARTESIAN_POINT('Ctrl Pts',(19.8600530949745,-52.6506910837937,-26.3688872010014));
#18782=CARTESIAN_POINT('Ctrl Pts',(20.7954149234172,-52.5324171165662,-26.3162376932706));
#18783=CARTESIAN_POINT('Ctrl Pts',(21.4692352056584,-52.0493212652077,-26.2635881855397));
#18784=CARTESIAN_POINT('Ctrl Pts',(22.1134333966795,-51.5874629897342,-26.2132532245238));
#18785=CARTESIAN_POINT('Ctrl Pts',(22.518580056272,-50.792153943755,-26.1629182635079));
#18786=CARTESIAN_POINT('Ctrl Pts',(22.5213592474396,-49.9993296992679,-26.112583302492));
#18787=CARTESIAN_POINT('Ctrl Pts',(22.51875591101,-50.0020955263397,-26.387416697508));
#18788=CARTESIAN_POINT('Ctrl Pts',(22.5201174455325,-50.1548244405144,-26.3970868001546));
#18789=CARTESIAN_POINT('Ctrl Pts',(22.5074052592067,-50.3073272725945,-26.4067569028011));
#18790=CARTESIAN_POINT('Ctrl Pts',(22.4798015470764,-50.4570851924628,-26.4164270054477));
#18791=CARTESIAN_POINT('Ctrl Pts',(22.3295113269701,-51.2724520037605,-26.4690765131785));
#18792=CARTESIAN_POINT('Ctrl Pts',(21.7377872289705,-52.006450575291,-26.5217260209094));
#18793=CARTESIAN_POINT('Ctrl Pts',(20.9728803659084,-52.3263363422347,-26.5743755286402));
#18794=CARTESIAN_POINT('Ctrl Pts',(20.2079735028462,-52.6462221091785,-26.627025036371));
#18795=CARTESIAN_POINT('Ctrl Pts',(19.2698838747213,-52.5519950715356,-26.6796745441018));
#18796=CARTESIAN_POINT('Ctrl Pts',(18.5838791489413,-52.0863703552799,-26.7323240518326));
#18797=CARTESIAN_POINT('Ctrl Pts',(17.8978744231613,-51.6207456390243,-26.7849735595635));
#18798=CARTESIAN_POINT('Ctrl Pts',(17.4639545997261,-50.7837232441561,-26.8376230672943));
#18799=CARTESIAN_POINT('Ctrl Pts',(17.4788311344027,-49.9547551821562,-26.8902725750251));
#18800=CARTESIAN_POINT('Ctrl Pts',(17.4937076690793,-49.1257871201564,-26.942922082756));
#18801=CARTESIAN_POINT('Ctrl Pts',(17.9573805618677,-48.304873391025,-26.9955715904868));
#18802=CARTESIAN_POINT('Ctrl Pts',(18.6596505054912,-47.8641624303278,-27.0482210982176));
#18803=CARTESIAN_POINT('Ctrl Pts',(19.3619204491148,-47.4234514696305,-27.1008706059484));
#18804=CARTESIAN_POINT('Ctrl Pts',(20.3027874435735,-47.3629432773675,-27.1535201136792));
#18805=CARTESIAN_POINT('Ctrl Pts',(21.0557238712505,-47.7100684831199,-27.2061696214101));
#18806=CARTESIAN_POINT('Ctrl Pts',(21.8086602989275,-48.0571936888723,-27.2588191291409));
#18807=CARTESIAN_POINT('Ctrl Pts',(22.3736661598227,-48.81195229264,-27.3114686368717));
#18808=CARTESIAN_POINT('Ctrl Pts',(22.4946045751828,-49.6321858781341,-27.3641181446025));
#18809=CARTESIAN_POINT('Ctrl Pts',(22.5124438687173,-49.7531762818444,-27.3718843289044));
#18810=CARTESIAN_POINT('Ctrl Pts',(22.5206209696132,-49.8755913157382,-27.3796505132062));
#18811=CARTESIAN_POINT('Ctrl Pts',(22.5196060265899,-49.9981422852793,-27.387416697508));
#18812=CARTESIAN_POINT('Origin',(20.,-50.,-32.));
#18813=CARTESIAN_POINT('',(22.5135352489342,-49.9997146182226,-28.387416697508));
#18814=CARTESIAN_POINT('',(22.5160873419658,-50.0021236034949,-28.112583302492));
#18815=CARTESIAN_POINT('',(22.5175,-50.,-32.));
#18816=CARTESIAN_POINT('Ctrl Pts',(22.5160873419658,-50.0021236034949,-28.112583302492));
#18817=CARTESIAN_POINT('Ctrl Pts',(22.5112879704401,-49.4131979553026,-28.0753961818803));
#18818=CARTESIAN_POINT('Ctrl Pts',(22.3047334737028,-48.821238787295,-28.0382090612686));
#18819=CARTESIAN_POINT('Ctrl Pts',(21.9270452588827,-48.3737048452096,-28.0010219406569));
#18820=CARTESIAN_POINT('Ctrl Pts',(21.3923144634106,-47.7400865021905,-27.9483724329261));
#18821=CARTESIAN_POINT('Ctrl Pts',(20.5145481327378,-47.3959668343932,-27.8957229251952));
#18822=CARTESIAN_POINT('Ctrl Pts',(19.6916682831495,-47.4973472343812,-27.8430734174644));
#18823=CARTESIAN_POINT('Ctrl Pts',(18.8687884335611,-47.5987276343691,-27.7904239097336));
#18824=CARTESIAN_POINT('Ctrl Pts',(18.1007950650571,-48.1456081021423,-27.7377744020028));
#18825=CARTESIAN_POINT('Ctrl Pts',(17.7358462958969,-48.89006874545,-27.685124894272));
#18826=CARTESIAN_POINT('Ctrl Pts',(17.3708975267368,-49.6345293887576,-27.6324753865411));
#18827=CARTESIAN_POINT('Ctrl Pts',(17.4089933569204,-50.5765702075996,-27.5798258788103));
#18828=CARTESIAN_POINT('Ctrl Pts',(17.8328636144219,-51.289131219645,-27.5271763710795));
#18829=CARTESIAN_POINT('Ctrl Pts',(18.2567338719235,-52.0016922316905,-27.4745268633487));
#18830=CARTESIAN_POINT('Ctrl Pts',(19.0663785567431,-52.4847734369395,-27.4218773556178));
#18831=CARTESIAN_POINT('Ctrl Pts',(19.8947575765285,-52.5193775212888,-27.369227847887));
#18832=CARTESIAN_POINT('Ctrl Pts',(20.723136596314,-52.5539816056381,-27.3165783401562));
#18833=CARTESIAN_POINT('Ctrl Pts',(21.5702499510653,-52.1401085690878,-27.2639288324254));
#18834=CARTESIAN_POINT('Ctrl Pts',(22.0520716566289,-51.4653810525637,-27.2112793246946));
#18835=CARTESIAN_POINT('Ctrl Pts',(22.3531437071225,-51.0437695008659,-27.178380650627));
#18836=CARTESIAN_POINT('Ctrl Pts',(22.511586735828,-50.5203066766564,-27.1454819765595));
#18837=CARTESIAN_POINT('Ctrl Pts',(22.5145120517532,-49.9984719976714,-27.112583302492));
#18838=CARTESIAN_POINT('Ctrl Pts',(22.5196060265899,-49.9981422852793,-27.387416697508));
#18839=CARTESIAN_POINT('Ctrl Pts',(22.5137403383433,-50.7064044882707,-27.432300020937));
#18840=CARTESIAN_POINT('Ctrl Pts',(22.2008546131046,-51.4192070272122,-27.477183344366));
#18841=CARTESIAN_POINT('Ctrl Pts',(21.6717031486973,-51.8877891102062,-27.522066667795));
#18842=CARTESIAN_POINT('Ctrl Pts',(21.0509923370266,-52.4374501895634,-27.5747161755258));
#18843=CARTESIAN_POINT('Ctrl Pts',(20.1326997438602,-52.6510637810572,-27.6273656832566));
#18844=CARTESIAN_POINT('Ctrl Pts',(19.333119335948,-52.4317913909958,-27.6800151909875));
#18845=CARTESIAN_POINT('Ctrl Pts',(18.5335389280356,-52.2125190009344,-27.7326646987183));
#18846=CARTESIAN_POINT('Ctrl Pts',(17.8526707053774,-51.5603606293177,-27.7853142064491));
#18847=CARTESIAN_POINT('Ctrl Pts',(17.5991759309459,-50.7709623668994,-27.8379637141799));
#18848=CARTESIAN_POINT('Ctrl Pts',(17.3456811565143,-49.9815641044811,-27.8906132219107));
#18849=CARTESIAN_POINT('Ctrl Pts',(17.5195598303094,-49.0549259512611,-27.9432627296416));
#18850=CARTESIAN_POINT('Ctrl Pts',(18.0419866956553,-48.4111252176501,-27.9959122373724));
#18851=CARTESIAN_POINT('Ctrl Pts',(18.5644135610011,-47.7673244840391,-28.0485617451032));
#18852=CARTESIAN_POINT('Ctrl Pts',(19.4353886178977,-47.4063611700371,-28.1012112528341));
#18853=CARTESIAN_POINT('Ctrl Pts',(20.2600685710903,-47.4918725075265,-28.1538607605649));
#18854=CARTESIAN_POINT('Ctrl Pts',(21.0847485242829,-47.5773838450159,-28.2065102682957));
#18855=CARTESIAN_POINT('Ctrl Pts',(21.8631333737715,-48.1093698339967,-28.2591597760265));
#18856=CARTESIAN_POINT('Ctrl Pts',(22.2423541837709,-48.8466627148794,-28.3118092837573));
#18857=CARTESIAN_POINT('Ctrl Pts',(22.4238810768686,-49.1995929403326,-28.3370117550075));
#18858=CARTESIAN_POINT('Ctrl Pts',(22.5139442132876,-49.5995668314161,-28.3622142262578));
#18859=CARTESIAN_POINT('Ctrl Pts',(22.5135352489342,-49.9997146182226,-28.387416697508));
#18860=CARTESIAN_POINT('Origin',(20.,-50.,-32.));
#18861=CARTESIAN_POINT('',(22.5185978370021,-50.0021261700316,-29.387416697508));
#18862=CARTESIAN_POINT('',(22.5214169330132,-49.9994390864176,-29.112583302492));
#18863=CARTESIAN_POINT('',(22.5175,-50.,-32.));
#18864=CARTESIAN_POINT('Ctrl Pts',(22.5214169330132,-49.9994390864176,-29.112583302492));
#18865=CARTESIAN_POINT('Ctrl Pts',(22.5215116550139,-49.9683497400867,-29.1106094026627));
#18866=CARTESIAN_POINT('Ctrl Pts',(22.5209858636051,-49.9372636712048,-29.1086355028335));
#18867=CARTESIAN_POINT('Ctrl Pts',(22.5198295796509,-49.9062010719754,-29.1066616030042));
#18868=CARTESIAN_POINT('Ctrl Pts',(22.488988206606,-49.077673436471,-29.0540120952734));
#18869=CARTESIAN_POINT('Ctrl Pts',(22.0095890811262,-48.2658430556014,-29.0013625875425));
#18870=CARTESIAN_POINT('Ctrl Pts',(21.2989605066287,-47.8387408873901,-28.9487130798117));
#18871=CARTESIAN_POINT('Ctrl Pts',(20.5883319321312,-47.4116387191788,-28.8960635720809));
#18872=CARTESIAN_POINT('Ctrl Pts',(19.6464739086159,-47.3692647636258,-28.8434140643501));
#18873=CARTESIAN_POINT('Ctrl Pts',(18.900363448358,-47.7308286086929,-28.7907645566192));
#18874=CARTESIAN_POINT('Ctrl Pts',(18.1542529881,-48.0923924537599,-28.7381150488884));
#18875=CARTESIAN_POINT('Ctrl Pts',(17.6038900910993,-48.8578940994471,-28.6854655411576));
#18876=CARTESIAN_POINT('Ctrl Pts',(17.4987734074998,-49.6803050163489,-28.6328160334268));
#18877=CARTESIAN_POINT('Ctrl Pts',(17.3936567239004,-50.5027159332509,-28.580166525696));
#18878=CARTESIAN_POINT('Ctrl Pts',(17.7337862537023,-51.3820361213676,-28.5275170179651));
#18879=CARTESIAN_POINT('Ctrl Pts',(18.3649694467479,-51.9196391434274,-28.4748675102343));
#18880=CARTESIAN_POINT('Ctrl Pts',(18.9961526397934,-52.4572421654872,-28.4222180025035));
#18881=CARTESIAN_POINT('Ctrl Pts',(19.9183894960826,-52.6531280214901,-28.3695684947727));
#18882=CARTESIAN_POINT('Ctrl Pts',(20.7135979613149,-52.4184948406945,-28.3169189870418));
#18883=CARTESIAN_POINT('Ctrl Pts',(21.5088064265471,-52.1838616598988,-28.264269479311));
#18884=CARTESIAN_POINT('Ctrl Pts',(22.1769865007224,-51.5187094423045,-28.2116199715802));
#18885=CARTESIAN_POINT('Ctrl Pts',(22.4152289076743,-50.7245748243869,-28.1589704638494));
#18886=CARTESIAN_POINT('Ctrl Pts',(22.4851972033575,-50.4913491511343,-28.1435080767302));
#18887=CARTESIAN_POINT('Ctrl Pts',(22.5180829183707,-50.246998608791,-28.1280456896111));
#18888=CARTESIAN_POINT('Ctrl Pts',(22.5160873419658,-50.0021236034949,-28.112583302492));
#18889=CARTESIAN_POINT('Ctrl Pts',(22.5135352489342,-49.9997146182226,-28.387416697508));
#18890=CARTESIAN_POINT('Ctrl Pts',(22.5130898616776,-50.4355000931096,-28.4148637339886));
#18891=CARTESIAN_POINT('Ctrl Pts',(22.4053396278516,-50.8714918178098,-28.4423107704692));
#18892=CARTESIAN_POINT('Ctrl Pts',(22.1915654556312,-51.2471487608302,-28.4697578069498));
#18893=CARTESIAN_POINT('Ctrl Pts',(21.7814991469819,-51.9677421531138,-28.5224073146806));
#18894=CARTESIAN_POINT('Ctrl Pts',(20.9813097591729,-52.4663291648967,-28.5750568224115));
#18895=CARTESIAN_POINT('Ctrl Pts',(20.1537509825797,-52.5168829559793,-28.6277063301423));
#18896=CARTESIAN_POINT('Ctrl Pts',(19.3261922059864,-52.5674367470618,-28.6803558378731));
#18897=CARTESIAN_POINT('Ctrl Pts',(18.4712640406088,-52.1699573174439,-28.7330053456039));
#18898=CARTESIAN_POINT('Ctrl Pts',(17.976535169618,-51.504635922312,-28.7856548533348));
#18899=CARTESIAN_POINT('Ctrl Pts',(17.4818062986271,-50.8393145271801,-28.8383043610656));
#18900=CARTESIAN_POINT('Ctrl Pts',(17.347276722023,-49.9061511665343,-28.8909538687964));
#18901=CARTESIAN_POINT('Ctrl Pts',(17.633933377528,-49.1281812594003,-28.9436033765272));
#18902=CARTESIAN_POINT('Ctrl Pts',(17.9205900330329,-48.3502113522664,-28.996252884258));
#18903=CARTESIAN_POINT('Ctrl Pts',(18.628432920647,-47.7274348986443,-29.0489023919888));
#18904=CARTESIAN_POINT('Ctrl Pts',(19.4365722313371,-47.5421781333803,-29.1015518997197));
#18905=CARTESIAN_POINT('Ctrl Pts',(20.2447115420273,-47.3569213681163,-29.1542014074505));
#18906=CARTESIAN_POINT('Ctrl Pts',(21.1531472757935,-47.6091842912105,-29.2068509151813));
#18907=CARTESIAN_POINT('Ctrl Pts',(21.7500539071284,-48.1846073425723,-29.2595004229122));
#18908=CARTESIAN_POINT('Ctrl Pts',(22.233465027528,-48.6506197595234,-29.3021391811108));
#18909=CARTESIAN_POINT('Ctrl Pts',(22.512552285434,-49.3285845273022,-29.3447779393094));
#18910=CARTESIAN_POINT('Ctrl Pts',(22.5185978370021,-50.0021261700316,-29.387416697508));
#18911=CARTESIAN_POINT('Origin',(20.,-50.,-32.));
#18912=CARTESIAN_POINT('',(22.5197500022945,-49.9981961379119,-30.387416697508));
#18913=CARTESIAN_POINT('',(22.5146149548606,-49.9984092956174,-30.112583302492));
#18914=CARTESIAN_POINT('',(22.5175,-50.,-32.));
#18915=CARTESIAN_POINT('Ctrl Pts',(22.5146149548606,-49.9984092956174,-30.112583302492));
#18916=CARTESIAN_POINT('Ctrl Pts',(22.5164166726556,-49.6905590369979,-30.0931731157143));
#18917=CARTESIAN_POINT('Ctrl Pts',(22.4640314720864,-49.3833005485878,-30.0737629289366));
#18918=CARTESIAN_POINT('Ctrl Pts',(22.354675889286,-49.0978687424812,-30.054352742159));
#18919=CARTESIAN_POINT('Ctrl Pts',(22.0580523859675,-48.3236441430802,-30.0017032344282));
#18920=CARTESIAN_POINT('Ctrl Pts',(21.3422703279879,-47.7100089631121,-29.9490537266973));
#18921=CARTESIAN_POINT('Ctrl Pts',(20.531818626569,-47.5351453799835,-29.8964042189665));
#18922=CARTESIAN_POINT('Ctrl Pts',(19.7213669251501,-47.3602817968549,-29.8437547112357));
#18923=CARTESIAN_POINT('Ctrl Pts',(18.8162455802918,-47.6241898105659,-29.7911052035049));
#18924=CARTESIAN_POINT('Ctrl Pts',(18.2267775896746,-48.2072307362936,-29.738455695774));
#18925=CARTESIAN_POINT('Ctrl Pts',(17.6373095990573,-48.7902716620213,-29.6858061880432));
#18926=CARTESIAN_POINT('Ctrl Pts',(17.363494962681,-49.6924454997657,-29.6331566803124));
#18927=CARTESIAN_POINT('Ctrl Pts',(17.5294633821,-50.5047654593872,-29.5805071725816));
#18928=CARTESIAN_POINT('Ctrl Pts',(17.6954318015189,-51.3170854190086,-29.5278576648508));
#18929=CARTESIAN_POINT('Ctrl Pts',(18.301183276733,-52.0395515005071,-29.4752081571199));
#18930=CARTESIAN_POINT('Ctrl Pts',(19.0721095880014,-52.3446446922152,-29.4225586493891));
#18931=CARTESIAN_POINT('Ctrl Pts',(19.8430358992699,-52.6497378839233,-29.3699091416583));
#18932=CARTESIAN_POINT('Ctrl Pts',(20.7791370465926,-52.5374581858409,-29.3172596339275));
#18933=CARTESIAN_POINT('Ctrl Pts',(21.4560458099491,-52.0587058917301,-29.2646101261966));
#18934=CARTESIAN_POINT('Ctrl Pts',(22.1075763665567,-51.597902655689,-29.2139345182951));
#18935=CARTESIAN_POINT('Ctrl Pts',(22.5189851505611,-50.797590796662,-29.1632589103935));
#18936=CARTESIAN_POINT('Ctrl Pts',(22.5214169330132,-49.9994390864176,-29.112583302492));
#18937=CARTESIAN_POINT('Ctrl Pts',(22.5185978370021,-50.0021261700316,-29.387416697508));
#18938=CARTESIAN_POINT('Ctrl Pts',(22.5200172147018,-50.160260622575,-29.3974274470402));
#18939=CARTESIAN_POINT('Ctrl Pts',(22.5063860176688,-50.3181512641088,-29.4074381965724));
#18940=CARTESIAN_POINT('Ctrl Pts',(22.4768149308017,-50.4729978615716,-29.4174489461046));
#18941=CARTESIAN_POINT('Ctrl Pts',(22.3212917942364,-51.28738214958,-29.4700984538354));
#18942=CARTESIAN_POINT('Ctrl Pts',(21.7248679922022,-52.0175675459674,-29.5227479615663));
#18943=CARTESIAN_POINT('Ctrl Pts',(20.9579231856422,-52.3325356050689,-29.5753974692971));
#18944=CARTESIAN_POINT('Ctrl Pts',(20.1909783790822,-52.6475036641704,-29.6280469770279));
#18945=CARTESIAN_POINT('Ctrl Pts',(19.2535125679963,-52.547254385986,-29.6806964847587));
#18946=CARTESIAN_POINT('Ctrl Pts',(18.5705116219756,-52.0772342563112,-29.7333459924895));
#18947=CARTESIAN_POINT('Ctrl Pts',(17.8875106759548,-51.6072141266365,-29.7859955002204));
#18948=CARTESIAN_POINT('Ctrl Pts',(17.4589745949992,-50.7674231454713,-29.8386450079512));
#18949=CARTESIAN_POINT('Ctrl Pts',(17.479173694741,-49.9385677835816,-29.891294515682));
#18950=CARTESIAN_POINT('Ctrl Pts',(17.4993727944828,-49.1097124216919,-29.9439440234129));
#18951=CARTESIAN_POINT('Ctrl Pts',(17.9683070749221,-48.2917926790776,-29.9965935311437));
#18952=CARTESIAN_POINT('Ctrl Pts',(18.6733923110178,-47.8556000331014,-30.0492430388745));
#18953=CARTESIAN_POINT('Ctrl Pts',(19.3784775471136,-47.4194073871252,-30.1018925466053));
#18954=CARTESIAN_POINT('Ctrl Pts',(20.319713738866,-47.3649418377871,-30.1545420543362));
#18955=CARTESIAN_POINT('Ctrl Pts',(21.070405771946,-47.7168945136317,-30.207191562067));
#18956=CARTESIAN_POINT('Ctrl Pts',(21.8210978050261,-48.0688471894763,-30.2598410697978));
#18957=CARTESIAN_POINT('Ctrl Pts',(22.3812456794339,-48.8272180905037,-30.3124905775286));
#18958=CARTESIAN_POINT('Ctrl Pts',(22.4969148743706,-49.6482113011374,-30.3651400852594));
#18959=CARTESIAN_POINT('Ctrl Pts',(22.5132285299378,-49.764001857721,-30.3725656226756));
#18960=CARTESIAN_POINT('Ctrl Pts',(22.5207008456371,-49.8810380648793,-30.3799911600918));
#18961=CARTESIAN_POINT('Ctrl Pts',(22.5197500022945,-49.9981961379119,-30.387416697508));
#18962=CARTESIAN_POINT('Origin',(20.,-50.,-32.));
#18963=CARTESIAN_POINT('',(22.5135564443693,-49.9996286810393,-31.387416697508));
#18964=CARTESIAN_POINT('',(22.5159431077322,-50.0020935760098,-31.112583302492));
#18965=CARTESIAN_POINT('',(22.5175,-50.,-32.));
#18966=CARTESIAN_POINT('Ctrl Pts',(22.5159431077322,-50.0020935760098,-31.112583302492));
#18967=CARTESIAN_POINT('Ctrl Pts',(22.5112751113286,-49.4184778817386,-31.0757368287659));
#18968=CARTESIAN_POINT('Ctrl Pts',(22.3088214262113,-48.8319400870852,-31.0388903550399));
#18969=CARTESIAN_POINT('Ctrl Pts',(21.9374479719839,-48.3861119291495,-31.0020438813138));
#18970=CARTESIAN_POINT('Ctrl Pts',(21.4067966620449,-47.7490731388881,-30.949394373583));
#18971=CARTESIAN_POINT('Ctrl Pts',(20.5312580173509,-47.399324414423,-30.8967448658522));
#18972=CARTESIAN_POINT('Ctrl Pts',(19.707744168322,-47.4954190214273,-30.8440953581213));
#18973=CARTESIAN_POINT('Ctrl Pts',(18.884230319293,-47.5915136284316,-30.7914458503905));
#18974=CARTESIAN_POINT('Ctrl Pts',(18.112741265929,-48.1334515669052,-30.7387963426597));
#18975=CARTESIAN_POINT('Ctrl Pts',(17.7430198386832,-48.8755535135898,-30.6861468349289));
#18976=CARTESIAN_POINT('Ctrl Pts',(17.3732984114373,-49.6176554602744,-30.633497327198));
#18977=CARTESIAN_POINT('Ctrl Pts',(17.4053446103095,-50.5599214151699,-30.5808478194672));
#18978=CARTESIAN_POINT('Ctrl Pts',(17.8246307783617,-51.2751894364864,-30.5281983117364));
#18979=CARTESIAN_POINT('Ctrl Pts',(18.2439169464138,-51.9904574578029,-30.4755488040056));
#18980=CARTESIAN_POINT('Ctrl Pts',(19.0504430836459,-52.4787275455404,-30.4228992962747));
#18981=CARTESIAN_POINT('Ctrl Pts',(19.8785828304355,-52.5186498804545,-30.3702497885439));
#18982=CARTESIAN_POINT('Ctrl Pts',(20.7067225772251,-52.5585722153686,-30.3176002808131));
#18983=CARTESIAN_POINT('Ctrl Pts',(21.5564759335723,-52.1501467974592,-30.2649507730823));
#18984=CARTESIAN_POINT('Ctrl Pts',(22.0426201374171,-51.4785270790876,-30.2123012653515));
#18985=CARTESIAN_POINT('Ctrl Pts',(22.3495385478177,-51.054512034321,-30.1790619443983));
#18986=CARTESIAN_POINT('Ctrl Pts',(22.5115295710495,-50.5255929682414,-30.1458226234451));
#18987=CARTESIAN_POINT('Ctrl Pts',(22.5146149548606,-49.9984092956174,-30.112583302492));
#18988=CARTESIAN_POINT('Ctrl Pts',(22.5197500022945,-49.9981961379119,-30.387416697508));
#18989=CARTESIAN_POINT('Ctrl Pts',(22.5139590529408,-50.7117274178686,-30.4326406678226));
#18990=CARTESIAN_POINT('Ctrl Pts',(22.1957353228996,-51.4297789608027,-30.4778646381373));
#18991=CARTESIAN_POINT('Ctrl Pts',(21.6595472004365,-51.8984842027323,-30.5230886084519));
#18992=CARTESIAN_POINT('Ctrl Pts',(21.0353198161003,-52.4441483734534,-30.5757381161827));
#18993=CARTESIAN_POINT('Ctrl Pts',(20.1156745319623,-52.6518611946555,-30.6283876239135));
#18994=CARTESIAN_POINT('Ctrl Pts',(19.3175185527131,-52.4274592174967,-30.6810371316444));
#18995=CARTESIAN_POINT('Ctrl Pts',(18.519362573464,-52.2030572403379,-30.7336866393752));
#18996=CARTESIAN_POINT('Ctrl Pts',(17.8426958991036,-51.5465404648181,-30.786336147106));
#18997=CARTESIAN_POINT('Ctrl Pts',(17.5942750765099,-50.7555307875917,-30.8389856548368));
#18998=CARTESIAN_POINT('Ctrl Pts',(17.3458542539162,-49.9645211103653,-30.8916351625677));
#18999=CARTESIAN_POINT('Ctrl Pts',(17.5256792830892,-49.0390185314322,-30.9442846702985));
#19000=CARTESIAN_POINT('Ctrl Pts',(18.0522292216189,-48.3985855710075,-30.9969341780293));
#19001=CARTESIAN_POINT('Ctrl Pts',(18.5787791601487,-47.7581526105828,-31.0495836857601));
#19002=CARTESIAN_POINT('Ctrl Pts',(19.452054008035,-47.4027892686665,-31.102233193491));
#19003=CARTESIAN_POINT('Ctrl Pts',(20.2761678927157,-47.4935941123726,-31.1548827012218));
#19004=CARTESIAN_POINT('Ctrl Pts',(21.1002817773964,-47.5843989560786,-31.2075322089526));
#19005=CARTESIAN_POINT('Ctrl Pts',(21.8752346988714,-48.1213719854071,-31.2601817166834));
#19006=CARTESIAN_POINT('Ctrl Pts',(22.2497135347539,-48.8610846431602,-31.3128312244142));
#19007=CARTESIAN_POINT('Ctrl Pts',(22.4265476106501,-49.2103871717109,-31.3376930487788));
#19008=CARTESIAN_POINT('Ctrl Pts',(22.5140816211901,-49.6048977741917,-31.3625548731434));
#19009=CARTESIAN_POINT('Ctrl Pts',(22.5135564443693,-49.9996286810393,-31.387416697508));
#19010=CARTESIAN_POINT('Origin',(20.,-50.,-32.));
#19011=CARTESIAN_POINT('',(22.5184387847934,-50.0021533196134,-32.387416697508));
#19012=CARTESIAN_POINT('',(22.5214654524887,-49.9995340141484,-32.112583302492));
#19013=CARTESIAN_POINT('',(22.5175,-50.,-32.));
#19014=CARTESIAN_POINT('Ctrl Pts',(22.5214654524887,-49.9995340141484,-32.112583302492));
#19015=CARTESIAN_POINT('Ctrl Pts',(22.5215315387758,-49.9738112570963,-32.1109500495483));
#19016=CARTESIAN_POINT('Ctrl Pts',(22.5211716022436,-49.9480903941566,-32.1093167966047));
#19017=CARTESIAN_POINT('Ctrl Pts',(22.5203799165757,-49.9223828272867,-32.107683543661));
#19018=CARTESIAN_POINT('Ctrl Pts',(22.4948591539416,-49.0936742393547,-32.0550340359302));
#19019=CARTESIAN_POINT('Ctrl Pts',(22.0206826727711,-48.2787823733245,-32.0023845281994));
#19020=CARTESIAN_POINT('Ctrl Pts',(21.3128111700898,-47.8471260647531,-31.9497350204686));
#19021=CARTESIAN_POINT('Ctrl Pts',(20.6049396674085,-47.4154697561817,-31.8970855127378));
#19022=CARTESIAN_POINT('Ctrl Pts',(19.6633731432164,-47.3670490050691,-31.8444360050069));
#19023=CARTESIAN_POINT('Ctrl Pts',(18.9149564630304,-47.7238146226069,-31.7917864972761));
#19024=CARTESIAN_POINT('Ctrl Pts',(18.1665397828444,-48.0805802401446,-31.7391369895453));
#19025=CARTESIAN_POINT('Ctrl Pts',(17.6112729466644,-48.8425322263327,-31.6864874818145));
#19026=CARTESIAN_POINT('Ctrl Pts',(17.5008777308339,-49.6642512350939,-31.6338379740837));
#19027=CARTESIAN_POINT('Ctrl Pts',(17.3904825150034,-50.4859702438552,-31.5811884663529));
#19028=CARTESIAN_POINT('Ctrl Pts',(17.7249589195224,-51.3674562751895,-31.528538958622));
#19029=CARTESIAN_POINT('Ctrl Pts',(18.3526771527223,-51.9091010413843,-31.4758894508912));
#19030=CARTESIAN_POINT('Ctrl Pts',(18.9803953859221,-52.4507458075792,-31.4232399431604));
#19031=CARTESIAN_POINT('Ctrl Pts',(19.9013554478028,-52.6525493086346,-31.3705904354296));
#19032=CARTESIAN_POINT('Ctrl Pts',(20.6980540991777,-52.423026996135,-31.3179409276987));
#19033=CARTESIAN_POINT('Ctrl Pts',(21.4947527505527,-52.1935046836355,-31.2652914199679));
#19034=CARTESIAN_POINT('Ctrl Pts',(22.1671899914219,-51.5326565575811,-31.2126419122371));
#19035=CARTESIAN_POINT('Ctrl Pts',(22.4105266242645,-50.740068066525,-31.1599924045063));
#19036=CARTESIAN_POINT('Ctrl Pts',(22.4835654284082,-50.502168351679,-31.1441893705015));
#19037=CARTESIAN_POINT('Ctrl Pts',(22.5179451583612,-50.2523997174019,-31.1283863364967));
#19038=CARTESIAN_POINT('Ctrl Pts',(22.5159431077322,-50.0020935760098,-31.112583302492));
#19039=CARTESIAN_POINT('Ctrl Pts',(22.5135564443693,-49.9996286810393,-31.387416697508));
#19040=CARTESIAN_POINT('Ctrl Pts',(22.5129694622158,-50.4408134184701,-31.4152043808743));
#19041=CARTESIAN_POINT('Ctrl Pts',(22.402377241224,-50.8822733643739,-31.4429920642405));
#19042=CARTESIAN_POINT('Ctrl Pts',(22.183512336775,-51.2611950894497,-31.4707797476067));
#19043=CARTESIAN_POINT('Ctrl Pts',(21.7688275526236,-51.9791405918085,-31.5234292553376));
#19044=CARTESIAN_POINT('Ctrl Pts',(20.9654532340308,-52.4725793103486,-31.5760787630683));
#19045=CARTESIAN_POINT('Ctrl Pts',(20.137586911568,-52.5178183056499,-31.6287282707992));
#19046=CARTESIAN_POINT('Ctrl Pts',(19.3097205891052,-52.5630573009512,-31.68137777853));
#19047=CARTESIAN_POINT('Ctrl Pts',(18.4573622627723,-52.1600965730137,-31.7340272862608));
#19048=CARTESIAN_POINT('Ctrl Pts',(17.966915618159,-51.4916122400996,-31.7866767939916));
#19049=CARTESIAN_POINT('Ctrl Pts',(17.4764689735458,-50.8231279071855,-31.8393263017225));
#19050=CARTESIAN_POINT('Ctrl Pts',(17.3479340106522,-49.8891199692948,-31.8919758094533));
#19051=CARTESIAN_POINT('Ctrl Pts',(17.6395801002989,-49.1130067217866,-31.9446253171841));
#19052=CARTESIAN_POINT('Ctrl Pts',(17.9312261899457,-48.3368934742784,-31.9972748249149));
#19053=CARTESIAN_POINT('Ctrl Pts',(18.6430533321328,-47.7186749171526,-32.0499243326458));
#19054=CARTESIAN_POINT('Ctrl Pts',(19.4523655165717,-47.5386110321486,-32.1025738403766));
#19055=CARTESIAN_POINT('Ctrl Pts',(20.2616777010105,-47.3585471471445,-32.1552233481074));
#19056=CARTESIAN_POINT('Ctrl Pts',(21.1684749277012,-47.6166379342622,-32.2078728558382));
#19057=CARTESIAN_POINT('Ctrl Pts',(21.7616744634189,-48.1958818598999,-32.2605223635691));
#19058=CARTESIAN_POINT('Ctrl Pts',(22.2382453009068,-48.6612408936304,-32.302820474882));
#19059=CARTESIAN_POINT('Ctrl Pts',(22.5124088354348,-49.3338837896983,-32.345118586195));
#19060=CARTESIAN_POINT('Ctrl Pts',(22.5184387847934,-50.0021533196134,-32.387416697508));
#19061=CARTESIAN_POINT('Origin',(20.,-50.,-32.));
#19062=CARTESIAN_POINT('',(22.5198908044257,-49.9982532979407,-33.387416697508));
#19063=CARTESIAN_POINT('',(22.5147221745587,-49.9983487241263,-33.112583302492));
#19064=CARTESIAN_POINT('',(22.5175,-50.,-32.));
#19065=CARTESIAN_POINT('Ctrl Pts',(22.5147221745587,-49.9983487241263,-33.112583302492));
#19066=CARTESIAN_POINT('Ctrl Pts',(22.5165647036742,-49.6959336362168,-33.0935137625999));
#19067=CARTESIAN_POINT('Ctrl Pts',(22.4660535271598,-49.3941132837153,-33.0744442227079));
#19068=CARTESIAN_POINT('Ctrl Pts',(22.3604199314187,-49.1130067098679,-33.0553746828159));
#19069=CARTESIAN_POINT('Ctrl Pts',(22.068773837853,-48.3368934519308,-33.0027251750851));
#19070=CARTESIAN_POINT('Ctrl Pts',(21.3569466861009,-47.7186748864979,-32.9500756673543));
#19071=CARTESIAN_POINT('Ctrl Pts',(20.5476344907871,-47.5386109990743,-32.8974261596234));
#19072=CARTESIAN_POINT('Ctrl Pts',(19.7383222954733,-47.3585471116506,-32.8447766518926));
#19073=CARTESIAN_POINT('Ctrl Pts',(18.8315250565977,-47.6166379022362,-32.7921271441618));
#19074=CARTESIAN_POINT('Ctrl Pts',(18.238325512909,-48.1958818356575,-32.7394776364309));
#19075=CARTESIAN_POINT('Ctrl Pts',(17.6451259692203,-48.7751257690787,-32.6868281287001));
#19076=CARTESIAN_POINT('Ctrl Pts',(17.3655241207184,-49.6755228453355,-32.6341786209693));
#19077=CARTESIAN_POINT('Ctrl Pts',(17.5262732135688,-50.4888917420764,-32.5815291132385));
#19078=CARTESIAN_POINT('Ctrl Pts',(17.6870223064191,-51.3022606388174,-32.5288796055077));
#19079=CARTESIAN_POINT('Ctrl Pts',(18.2881223406218,-52.0286013560425,-32.4762300977768));
#19080=CARTESIAN_POINT('Ctrl Pts',(19.0570737564864,-52.3386383749249,-32.423580590046));
#19081=CARTESIAN_POINT('Ctrl Pts',(19.8260251723511,-52.6486753938073,-32.3709310823152));
#19082=CARTESIAN_POINT('Ctrl Pts',(20.7628279698778,-52.542408714347,-32.3182815745844));
#19083=CARTESIAN_POINT('Ctrl Pts',(21.4427968465925,-52.0680127196999,-32.2656320668536));
#19084=CARTESIAN_POINT('Ctrl Pts',(22.1016722465143,-51.608333076413,-32.2146158120664));
#19085=CARTESIAN_POINT('Ctrl Pts',(22.5194011826095,-50.8030095154242,-32.1635995572792));
#19086=CARTESIAN_POINT('Ctrl Pts',(22.5214654524887,-49.9995340141484,-32.112583302492));
#19087=CARTESIAN_POINT('Ctrl Pts',(22.5184387847934,-50.0021533196134,-32.387416697508));
#19088=CARTESIAN_POINT('Ctrl Pts',(22.5199144628852,-50.1656954401332,-32.3977680939259));
#19089=CARTESIAN_POINT('Ctrl Pts',(22.5053315607811,-50.3289756387791,-32.4081194903437));
#19090=CARTESIAN_POINT('Ctrl Pts',(22.4737267531911,-50.4888917355071,-32.4184708867615));
#19091=CARTESIAN_POINT('Ctrl Pts',(22.3129776625007,-51.3022606213186,-32.4711203944923));
#19092=CARTESIAN_POINT('Ctrl Pts',(21.7118776363753,-52.0286013287837,-32.5237699022232));
#19093=CARTESIAN_POINT('Ctrl Pts',(20.9429262308432,-52.3386383435,-32.576419409954));
#19094=CARTESIAN_POINT('Ctrl Pts',(20.1739748253111,-52.6486753582164,-32.6290689176848));
#19095=CARTESIAN_POINT('Ctrl Pts',(19.2371720403724,-52.542408680184,-32.6817184254156));
#19096=CARTESIAN_POINT('Ctrl Pts',(18.5572031727947,-52.0680126919115,-32.7343679331465));
#19097=CARTESIAN_POINT('Ctrl Pts',(17.877234305217,-51.5936167036389,-32.7870174408773));
#19098=CARTESIAN_POINT('Ctrl Pts',(17.4540993550003,-50.7510914051262,-32.8396669486081));
#19099=CARTESIAN_POINT('Ctrl Pts',(17.4796201172914,-49.9223828283297,-32.8923164563389));
#19100=CARTESIAN_POINT('Ctrl Pts',(17.5051408795824,-49.0936742515332,-32.9449659640697));
#19101=CARTESIAN_POINT('Ctrl Pts',(17.9793173543814,-48.2787823964529,-32.9976154718006));
#19102=CARTESIAN_POINT('Ctrl Pts',(18.6871888475508,-47.8471260936818,-33.0502649795314));
#19103=CARTESIAN_POINT('Ctrl Pts',(19.3950603407203,-47.4154697909107,-33.1029144872622));
#19104=CARTESIAN_POINT('Ctrl Pts',(20.3366268522603,-47.3670490404488,-33.155563994993));
#19105=CARTESIAN_POINT('Ctrl Pts',(21.0850435223897,-47.7238146531926,-33.2082135027239));
#19106=CARTESIAN_POINT('Ctrl Pts',(21.833460192519,-48.0805802659364,-33.2608630104547));
#19107=CARTESIAN_POINT('Ctrl Pts',(22.3887270212377,-48.842532241886,-33.3135125181855));
#19108=CARTESIAN_POINT('Ctrl Pts',(22.4991222355848,-49.6642512396056,-33.3661620259163));
#19109=CARTESIAN_POINT('Ctrl Pts',(22.5139777972501,-49.7748275658933,-33.3732469164469));
#19110=CARTESIAN_POINT('Ctrl Pts',(22.5207774906703,-49.8864861712863,-33.3803318069775));
#19111=CARTESIAN_POINT('Ctrl Pts',(22.5198908044257,-49.9982532979407,-33.387416697508));
#19112=CARTESIAN_POINT('Origin',(20.,-50.,-32.));
#19113=CARTESIAN_POINT('',(22.5135831830112,-49.9995432846514,-34.387416697508));
#19114=CARTESIAN_POINT('',(22.5158015821966,-50.0020603006293,-34.112583302492));
#19115=CARTESIAN_POINT('',(22.5175,-50.,-32.));
#19116=CARTESIAN_POINT('Ctrl Pts',(22.5158015821966,-50.0020603006293,-34.112583302492));
#19117=CARTESIAN_POINT('Ctrl Pts',(22.5112691112874,-49.4237577609146,-34.0760774756515));
#19118=CARTESIAN_POINT('Ctrl Pts',(22.3128671172368,-48.8426454482035,-34.0395716488111));
#19119=CARTESIAN_POINT('Ctrl Pts',(21.9477708045538,-48.3985855494889,-34.0030658219707));
#19120=CARTESIAN_POINT('Ctrl Pts',(21.4212208589487,-47.7581525804585,-33.9504163142399));
#19121=CARTESIAN_POINT('Ctrl Pts',(20.5479459993279,-47.4027892337671,-33.897766806509));
#19122=CARTESIAN_POINT('Ctrl Pts',(19.7238321035734,-47.4935940786933,-33.8451172987782));
#19123=CARTESIAN_POINT('Ctrl Pts',(18.8997182078189,-47.5843989236195,-33.7924677910474));
#19124=CARTESIAN_POINT('Ctrl Pts',(18.1247652759306,-48.1213719601635,-33.7398182833166));
#19125=CARTESIAN_POINT('Ctrl Pts',(17.7502864350161,-48.8610846278562,-33.6871687755858));
#19126=CARTESIAN_POINT('Ctrl Pts',(17.3758075941016,-49.600797295549,-33.6345192678549));
#19127=CARTESIAN_POINT('Ctrl Pts',(17.4018028441609,-50.5432495943906,-33.5818697601241));
#19128=CARTESIAN_POINT('Ctrl Pts',(17.8164876338846,-51.2611951063967,-33.5292202523933));
#19129=CARTESIAN_POINT('Ctrl Pts',(18.2311724236082,-51.9791406184027,-33.4765707446625));
#19130=CARTESIAN_POINT('Ctrl Pts',(19.0345467529961,-52.4725793435733,-33.4239212369316));
#19131=CARTESIAN_POINT('Ctrl Pts',(19.8624130865832,-52.5178183394824,-33.3712717292008));
#19132=CARTESIAN_POINT('Ctrl Pts',(20.6902794201703,-52.5630573353916,-33.31862222147));
#19133=CARTESIAN_POINT('Ctrl Pts',(21.5426377579565,-52.1600966020395,-33.2659727137392));
#19134=CARTESIAN_POINT('Ctrl Pts',(22.03308440916,-51.4916122601428,-33.2133232060084));
#19135=CARTESIAN_POINT('Ctrl Pts',(22.3458923248248,-51.0652515272677,-33.1797432381696));
#19136=CARTESIAN_POINT('Ctrl Pts',(22.5114776249371,-50.5308780344015,-33.1461632703308));
#19137=CARTESIAN_POINT('Ctrl Pts',(22.5147221745587,-49.9983487241263,-33.112583302492));
#19138=CARTESIAN_POINT('Ctrl Pts',(22.5198908044257,-49.9982532979407,-33.387416697508));
#19139=CARTESIAN_POINT('Ctrl Pts',(22.5141883141564,-50.7170542899409,-33.4329813147083));
#19140=CARTESIAN_POINT('Ctrl Pts',(22.1905708411972,-51.4403438105407,-33.4785459319085));
#19141=CARTESIAN_POINT('Ctrl Pts',(21.6473228251422,-51.9091010157313,-33.5241105491088));
#19142=CARTESIAN_POINT('Ctrl Pts',(21.0196046003771,-52.4507457746479,-33.5767600568396));
#19143=CARTESIAN_POINT('Ctrl Pts',(20.0986445508716,-52.6525492729915,-33.6294095645704));
#19144=CARTESIAN_POINT('Ctrl Pts',(19.3019459102021,-52.4230269635761,-33.6820590723013));
#19145=CARTESIAN_POINT('Ctrl Pts',(18.5052472695326,-52.1935046541608,-33.7347085800321));
#19146=CARTESIAN_POINT('Ctrl Pts',(17.8328100376991,-51.5326565369863,-33.7873580877629));
#19147=CARTESIAN_POINT('Ctrl Pts',(17.5894734081264,-50.7400680565804,-33.8400075954937));
#19148=CARTESIAN_POINT('Ctrl Pts',(17.3461367785536,-49.9474795761745,-33.8926571032246));
#19149=CARTESIAN_POINT('Ctrl Pts',(17.5319007512416,-49.0231507325371,-33.9453066109554));
#19150=CARTESIAN_POINT('Ctrl Pts',(18.0625520540502,-48.3861119508357,-33.9979561186862));
#19151=CARTESIAN_POINT('Ctrl Pts',(18.5932033568587,-47.7490731691343,-34.050605626417));
#19152=CARTESIAN_POINT('Ctrl Pts',(19.4687419897878,-47.399324449369,-34.1032551341478));
#19153=CARTESIAN_POINT('Ctrl Pts',(20.292255827751,-47.495419055082,-34.1559046418787));
#19154=CARTESIAN_POINT('Ctrl Pts',(21.1157696657142,-47.5915136607951,-34.2085541496095));
#19155=CARTESIAN_POINT('Ctrl Pts',(21.8872587087114,-48.1334515919866,-34.2612036573403));
#19156=CARTESIAN_POINT('Ctrl Pts',(22.2569801309892,-48.8755535286994,-34.3138531650711));
#19157=CARTESIAN_POINT('Ctrl Pts',(22.4291755608078,-49.2211828438043,-34.3383743425501));
#19158=CARTESIAN_POINT('Ctrl Pts',(22.5142206789451,-49.610231176692,-34.3628955200291));
#19159=CARTESIAN_POINT('Ctrl Pts',(22.5135831830112,-49.9995432846514,-34.387416697508));
#19160=CARTESIAN_POINT('Origin',(20.,-50.,-32.));
#19161=CARTESIAN_POINT('',(22.5182788973074,-50.0021768080843,-35.387416697508));
#19162=CARTESIAN_POINT('',(22.5215055099484,-49.9996299858508,-35.112583302492));
#19163=CARTESIAN_POINT('',(22.5175,-50.,-32.));
#19164=CARTESIAN_POINT('Ctrl Pts',(22.5215055099484,-49.9996299858508,-35.112583302492));
#19165=CARTESIAN_POINT('Ctrl Pts',(22.5215476822769,-49.9792730825142,-35.111290696434));
#19166=CARTESIAN_POINT('Ctrl Pts',(22.5213222503032,-49.9589171368633,-35.109998090376));
#19167=CARTESIAN_POINT('Ctrl Pts',(22.520826339132,-49.9385677827562,-35.108705484318));
#19168=CARTESIAN_POINT('Ctrl Pts',(22.5006272391188,-49.1097124097289,-35.0560559765872));
#19169=CARTESIAN_POINT('Ctrl Pts',(22.0316929523784,-48.291792656124,-35.0034064688563));
#19170=CARTESIAN_POINT('Ctrl Pts',(21.3266077068082,-47.8556000042866,-34.9507569611255));
#19171=CARTESIAN_POINT('Ctrl Pts',(20.621522461238,-47.4194073524491,-34.8981074533947));
#19172=CARTESIAN_POINT('Ctrl Pts',(19.680286256838,-47.3649418023791,-34.8454579456639));
#19173=CARTESIAN_POINT('Ctrl Pts',(18.9295942136707,-47.716894482953,-34.792808437933));
#19174=CARTESIAN_POINT('Ctrl Pts',(18.1789021705034,-48.0688471635269,-34.7401589302022));
#19175=CARTESIAN_POINT('Ctrl Pts',(17.6187542885687,-48.8272180747446,-34.6875094224714));
#19176=CARTESIAN_POINT('Ctrl Pts',(17.5030850920777,-49.6482112964103,-34.6348599147406));
#19177=CARTESIAN_POINT('Ctrl Pts',(17.3874158955868,-50.4692045180759,-34.5822104070097));
#19178=CARTESIAN_POINT('Ctrl Pts',(17.7162253845396,-51.3528200501893,-34.5295608992789));
#19179=CARTESIAN_POINT('Ctrl Pts',(18.3404527772637,-51.8984842282426,-34.4769113915481));
#19180=CARTESIAN_POINT('Ctrl Pts',(18.9646801699878,-52.444148406296,-34.4242618838173));
#19181=CARTESIAN_POINT('Ctrl Pts',(19.8843254664833,-52.6518612302893,-34.3716123760864));
#19182=CARTESIAN_POINT('Ctrl Pts',(20.6824814564575,-52.4274592501151,-34.3189628683556));
#19183=CARTESIAN_POINT('Ctrl Pts',(21.4806374464317,-52.203057269941,-34.2663133606248));
#19184=CARTESIAN_POINT('Ctrl Pts',(22.1573041298847,-51.5465404855995,-34.213663852894));
#19185=CARTESIAN_POINT('Ctrl Pts',(22.4057249558165,-50.755530797744,-34.1610143451632));
#19186=CARTESIAN_POINT('Ctrl Pts',(22.4818971122757,-50.5129870678532,-34.1448706642728));
#19187=CARTESIAN_POINT('Ctrl Pts',(22.5178059406877,-50.2577984243011,-34.1287269833824));
#19188=CARTESIAN_POINT('Ctrl Pts',(22.5158015821966,-50.0020603006293,-34.112583302492));
#19189=CARTESIAN_POINT('Ctrl Pts',(22.5135831830112,-49.9995432846514,-34.387416697508));
#19190=CARTESIAN_POINT('Ctrl Pts',(22.512851909149,-50.4461245939351,-34.4155450277599));
#19191=CARTESIAN_POINT('Ctrl Pts',(22.3993754586544,-50.8930529907507,-34.4436733580118));
#19192=CARTESIAN_POINT('Ctrl Pts',(22.1753691924073,-51.2751894193514,-34.4718016882636));
#19193=CARTESIAN_POINT('Ctrl Pts',(21.7560830299892,-51.9904574310566,-34.5244511959944));
#19194=CARTESIAN_POINT('Ctrl Pts',(20.9495569035946,-52.4787275122331,-34.5771007037253));
#19195=CARTESIAN_POINT('Ctrl Pts',(20.1214171679329,-52.5186498466107,-34.6297502114561));
#19196=CARTESIAN_POINT('Ctrl Pts',(19.2932774322712,-52.5585721809883,-34.6823997191869));
#19197=CARTESIAN_POINT('Ctrl Pts',(18.4435240873424,-52.150146768567,-34.7350492269177));
#19198=CARTESIAN_POINT('Ctrl Pts',(17.95737989003,-51.4785270592201,-34.7876987346485));
#19199=CARTESIAN_POINT('Ctrl Pts',(17.4712356927177,-50.8069073498732,-34.8403482423793));
#19200=CARTESIAN_POINT('Ctrl Pts',(17.3487006430217,-49.8720933436008,-34.8929977501102));
#19201=CARTESIAN_POINT('Ctrl Pts',(17.6453241423544,-49.0978687546033,-34.945647257841));
#19202=CARTESIAN_POINT('Ctrl Pts',(17.9419476416872,-48.3236441656058,-34.9982967655718));
#19203=CARTESIAN_POINT('Ctrl Pts',(18.6577296900485,-47.7100089938833,-35.0509462733026));
#19204=CARTESIAN_POINT('Ctrl Pts',(19.4681813805772,-47.5351454131044,-35.1035957810335));
#19205=CARTESIAN_POINT('Ctrl Pts',(20.2786330711059,-47.3602818323255,-35.1562452887643));
#19206=CARTESIAN_POINT('Ctrl Pts',(21.1837544038018,-47.6241898424903,-35.2088947964951));
#19207=CARTESIAN_POINT('Ctrl Pts',(21.7732223864982,-48.2072307603836,-35.2615443042259));
#19208=CARTESIAN_POINT('Ctrl Pts',(22.2429814209321,-48.6718679360485,-35.3035017686533));
#19209=CARTESIAN_POINT('Ctrl Pts',(22.512274677717,-49.3391806940296,-35.3454592330807));
#19210=CARTESIAN_POINT('Ctrl Pts',(22.5182788973074,-50.0021768080843,-35.387416697508));
#19211=CARTESIAN_POINT('Origin',(20.,-50.,-32.));
#19212=CARTESIAN_POINT('',(22.5200281316337,-49.9983136770239,-36.387416697508));
#19213=CARTESIAN_POINT('',(22.514833600647,-49.998290627205,-36.112583302492));
#19214=CARTESIAN_POINT('',(22.5175,-50.,-32.));
#19215=CARTESIAN_POINT('Ctrl Pts',(22.514833600647,-49.998290627205,-36.112583302492));
#19216=CARTESIAN_POINT('Ctrl Pts',(22.5167122753364,-49.701310816587,-36.0938544094856));
#19217=CARTESIAN_POINT('Ctrl Pts',(22.4680383940606,-49.4049267668115,-36.0751255164792));
#19218=CARTESIAN_POINT('Ctrl Pts',(22.3660666542655,-49.1281812476854,-36.0563966234728));
#19219=CARTESIAN_POINT('Ctrl Pts',(22.0794099949087,-48.3502113300977,-36.003747115742));
#19220=CARTESIAN_POINT('Ctrl Pts',(21.3715670977831,-47.7274348681072,-35.9510976080111));
#19221=CARTESIAN_POINT('Ctrl Pts',(20.5634277762338,-47.5421781003539,-35.8984481002803));
#19222=CARTESIAN_POINT('Ctrl Pts',(19.7552884546845,-47.3569213326006,-35.8457985925495));
#19223=CARTESIAN_POINT('Ctrl Pts',(18.8468527087114,-47.6091842590845,-35.7931490848187));
#19224=CARTESIAN_POINT('Ctrl Pts',(18.2499460693557,-48.1846073181783,-35.7404995770878));
#19225=CARTESIAN_POINT('Ctrl Pts',(17.6530394299999,-48.7600303772722,-35.687850069357));
#19226=CARTESIAN_POINT('Ctrl Pts',(17.3676618972616,-49.658613568976,-35.6352005616262));
#19227=CARTESIAN_POINT('Ctrl Pts',(17.5231850359167,-50.4729978679274,-35.5825510538954));
#19228=CARTESIAN_POINT('Ctrl Pts',(17.6787081745718,-51.2873821668789,-35.5299015461646));
#19229=CARTESIAN_POINT('Ctrl Pts',(18.2751319846203,-52.017567573078,-35.4772520384337));
#19230=CARTESIAN_POINT('Ctrl Pts',(19.0420768014859,-52.3325356364118,-35.4246025307029));
#19231=CARTESIAN_POINT('Ctrl Pts',(19.8090216183516,-52.6475036997456,-35.3719530229721));
#19232=CARTESIAN_POINT('Ctrl Pts',(20.7464874420344,-52.5472544202141,-35.3193035152413));
#19233=CARTESIAN_POINT('Ctrl Pts',(21.4294883972328,-52.0772342842236,-35.2666540075104));
#19234=CARTESIAN_POINT('Ctrl Pts',(22.095720892281,-51.6187536839543,-35.2152971058376));
#19235=CARTESIAN_POINT('Ctrl Pts',(22.5198299490833,-50.8084359453709,-35.1639402041648));
#19236=CARTESIAN_POINT('Ctrl Pts',(22.5215055099484,-49.9996299858508,-35.112583302492));
#19237=CARTESIAN_POINT('Ctrl Pts',(22.5182788973074,-50.0021768080843,-35.387416697508));
#19238=CARTESIAN_POINT('Ctrl Pts',(22.519808955826,-50.171128465632,-35.3981087408115));
#19239=CARTESIAN_POINT('Ctrl Pts',(22.5042413918334,-50.3397998063493,-35.408800784115));
#19240=CARTESIAN_POINT('Ctrl Pts',(22.4705365847028,-50.5047654526046,-35.4194928274184));
#19241=CARTESIAN_POINT('Ctrl Pts',(22.304568167514,-51.3170854013106,-35.4721423351492));
#19242=CARTESIAN_POINT('Ctrl Pts',(21.6988167004395,-52.0395514731012,-35.5247918428801));
#19243=CARTESIAN_POINT('Ctrl Pts',(20.9278903995302,-52.3446446607096,-35.5774413506109));
#19244=CARTESIAN_POINT('Ctrl Pts',(20.1569640986209,-52.6497378483181,-35.6300908583417));
#19245=CARTESIAN_POINT('Ctrl Pts',(19.2208629638768,-52.5374581517444,-35.6827403660725));
#19246=CARTESIAN_POINT('Ctrl Pts',(18.5439542096161,-52.0587058640667,-35.7353898738034));
#19247=CARTESIAN_POINT('Ctrl Pts',(17.8670454553555,-51.579953576389,-35.7880393815342));
#19248=CARTESIAN_POINT('Ctrl Pts',(17.4493290815783,-50.7347286976071,-35.840688889265));
#19249=CARTESIAN_POINT('Ctrl Pts',(17.4801704542087,-49.9062010732358,-35.8933383969958));
#19250=CARTESIAN_POINT('Ctrl Pts',(17.5110118268392,-49.0776734488645,-35.9459879047266));
#19251=CARTESIAN_POINT('Ctrl Pts',(17.9904109458772,-48.2658430789037,-35.9986374124575));
#19252=CARTESIAN_POINT('Ctrl Pts',(18.7010395108258,-47.8387409164315,-36.0512869201883));
#19253=CARTESIAN_POINT('Ctrl Pts',(19.4116680757745,-47.4116387539593,-36.1039364279191));
#19254=CARTESIAN_POINT('Ctrl Pts',(20.3535260866337,-47.3692647989758,-36.1565859356499));
#19255=CARTESIAN_POINT('Ctrl Pts',(21.099636536866,-47.7308286391844,-36.2092354433808));
#19256=CARTESIAN_POINT('Ctrl Pts',(21.8457469870983,-48.092392479393,-36.2618849511116));
#19257=CARTESIAN_POINT('Ctrl Pts',(22.3961098767036,-48.8578941147936,-36.3145344588424));
#19258=CARTESIAN_POINT('Ctrl Pts',(22.5012265588905,-49.6803050206447,-36.3671839665732));
#19259=CARTESIAN_POINT('Ctrl Pts',(22.5146916898361,-49.7856533850333,-36.3739282102182));
#19260=CARTESIAN_POINT('Ctrl Pts',(22.5208508471277,-49.8919355645194,-36.3806724538631));
#19261=CARTESIAN_POINT('Ctrl Pts',(22.5200281316337,-49.9983136770239,-36.387416697508));
#19262=CARTESIAN_POINT('Origin',(20.,-50.,-32.));
#19263=CARTESIAN_POINT('',(22.5136154336298,-49.9994585736035,-37.387416697508));
#19264=CARTESIAN_POINT('',(22.5156629463979,-50.0020238415623,-37.112583302492));
#19265=CARTESIAN_POINT('',(22.5175,-50.,-32.));
#19266=CARTESIAN_POINT('Ctrl Pts',(22.5156629463979,-50.0020238415623,-37.112583302492));
#19267=CARTESIAN_POINT('Ctrl Pts',(22.5112698172375,-49.4290377137389,-37.0764181225372));
#19268=CARTESIAN_POINT('Ctrl Pts',(22.3168706622171,-48.8533547764504,-37.0402529425824));
#19269=CARTESIAN_POINT('Ctrl Pts',(21.9580133306554,-48.4111251962995,-37.0040877626276));
#19270=CARTESIAN_POINT('Ctrl Pts',(21.4355864582898,-47.7673244540371,-36.9514382548968));
#19271=CARTESIAN_POINT('Ctrl Pts',(20.5646113896891,-47.4063611351857,-36.898788747166));
#19272=CARTESIAN_POINT('Ctrl Pts',(19.7399314254149,-47.4918724738244,-36.8461392394351));
#19273=CARTESIAN_POINT('Ctrl Pts',(18.9152514611408,-47.5773838124631,-36.7934897317043));
#19274=CARTESIAN_POINT('Ctrl Pts',(18.1368666011931,-48.1093698085918,-36.7408402239735));
#19275=CARTESIAN_POINT('Ctrl Pts',(17.7576457860981,-48.8466626993815,-36.6881907162427));
#19276=CARTESIAN_POINT('Ctrl Pts',(17.378424971003,-49.5839555901713,-36.6355412085118));
#19277=CARTESIAN_POINT('Ctrl Pts',(17.3983682007606,-50.5265553756219,-36.582891700781));
#19278=CARTESIAN_POINT('Ctrl Pts',(17.8084345149201,-51.2471487775885,-36.5302421930502));
#19279=CARTESIAN_POINT('Ctrl Pts',(18.2185008290795,-51.967742179555,-36.4775926853194));
#19280=CARTESIAN_POINT('Ctrl Pts',(19.0186902276409,-52.4663291980374,-36.4249431775885));
#19281=CARTESIAN_POINT('Ctrl Pts',(19.8462490153544,-52.5168829897992,-36.3722936698577));
#19282=CARTESIAN_POINT('Ctrl Pts',(20.6738078030678,-52.567436781561,-36.3196441621269));
#19283=CARTESIAN_POINT('Ctrl Pts',(21.5287359799332,-52.1699573466022,-36.2669946543961));
#19284=CARTESIAN_POINT('Ctrl Pts',(22.0234648575718,-51.5046359425303,-36.2143451466652));
#19285=CARTESIAN_POINT('Ctrl Pts',(22.3422049251376,-51.0759878508744,-36.1804245319408));
#19286=CARTESIAN_POINT('Ctrl Pts',(22.5114310610355,-50.5361621251873,-36.1465039172164));
#19287=CARTESIAN_POINT('Ctrl Pts',(22.514833600647,-49.998290627205,-36.112583302492));
#19288=CARTESIAN_POINT('Ctrl Pts',(22.5200281316337,-49.9983136770239,-36.387416697508));
#19289=CARTESIAN_POINT('Ctrl Pts',(22.5144282491257,-50.7223852860246,-36.4333219615939));
#19290=CARTESIAN_POINT('Ctrl Pts',(22.1853610476112,-51.450901432647,-36.4792272256798));
#19291=CARTESIAN_POINT('Ctrl Pts',(21.6350305312817,-51.919639117633,-36.5251324897657));
#19292=CARTESIAN_POINT('Ctrl Pts',(21.0038473467175,-52.4572421324687,-36.5777819974965));
#19293=CARTESIAN_POINT('Ctrl Pts',(20.0816105028205,-52.6531279858382,-36.6304315052274));
#19294=CARTESIAN_POINT('Ctrl Pts',(19.2864020482738,-52.4184948081959,-36.6830810129582));
#19295=CARTESIAN_POINT('Ctrl Pts',(18.491193593727,-52.1838616305535,-36.735730520689));
#19296=CARTESIAN_POINT('Ctrl Pts',(17.8230135285305,-51.5187094218993,-36.7883800284198));
#19297=CARTESIAN_POINT('Ctrl Pts',(17.5847711247798,-50.7245748146517,-36.8410295361506));
#19298=CARTESIAN_POINT('Ctrl Pts',(17.3465287210292,-49.9304402074041,-36.8936790438814));
#19299=CARTESIAN_POINT('Ctrl Pts',(17.5382239787243,-49.0073232015632,-36.9463285516123));
#19300=CARTESIAN_POINT('Ctrl Pts',(18.0729547670113,-48.3737048670602,-36.9989780593431));
#19301=CARTESIAN_POINT('Ctrl Pts',(18.6076855552984,-47.7400865325572,-37.0516275670739));
#19302=CARTESIAN_POINT('Ctrl Pts',(19.4854518741773,-47.395966869392,-37.1042770748048));
#19303=CARTESIAN_POINT('Ctrl Pts',(20.308331712708,-47.4973472680142,-37.1569265825356));
#19304=CARTESIAN_POINT('Ctrl Pts',(21.1312115512386,-47.5987276666363,-37.2095760902664));
#19305=CARTESIAN_POINT('Ctrl Pts',(21.899204909421,-48.1456081270457,-37.2622255979972));
#19306=CARTESIAN_POINT('Ctrl Pts',(22.2641536736782,-48.8900687603565,-37.314875105728));
#19307=CARTESIAN_POINT('Ctrl Pts',(22.431765017819,-49.2319798986588,-37.3390556363213));
#19308=CARTESIAN_POINT('Ctrl Pts',(22.5143612515527,-49.6155670709948,-37.3632361669147));
#19309=CARTESIAN_POINT('Ctrl Pts',(22.5136154336298,-49.9994585736035,-37.387416697508));
#19310=CARTESIAN_POINT('Origin',(20.,-50.,-32.));
#19311=CARTESIAN_POINT('',(22.5181182812424,-50.0021988905331,-38.387416697508));
#19312=CARTESIAN_POINT('',(22.5215368448905,-49.9997267149633,-38.112583302492));
#19313=CARTESIAN_POINT('',(22.5175,-50.,-32.));
#19314=CARTESIAN_POINT('Ctrl Pts',(22.5215368448905,-49.9997267149633,-38.112583302492));
#19315=CARTESIAN_POINT('Ctrl Pts',(22.5215601439286,-49.9847350660108,-38.1116313433196));
#19316=CARTESIAN_POINT('Ctrl Pts',(22.5214378830458,-49.9697438072224,-38.1106793841472));
#19317=CARTESIAN_POINT('Ctrl Pts',(22.5211688994512,-49.9547551815961,-38.1097274249749));
#19318=CARTESIAN_POINT('Ctrl Pts',(22.5062923645566,-49.1257871084977,-38.057077917244));
#19319=CARTESIAN_POINT('Ctrl Pts',(22.0426194655824,-48.3048733682434,-38.0044284095132));
#19320=CARTESIAN_POINT('Ctrl Pts',(21.3403495125323,-47.8641624016026,-37.9517789017824));
#19321=CARTESIAN_POINT('Ctrl Pts',(20.6380795594823,-47.4234514349619,-37.8991293940516));
#19322=CARTESIAN_POINT('Ctrl Pts',(19.6972125523564,-47.3629432419346,-37.8464798863208));
#19323=CARTESIAN_POINT('Ctrl Pts',(18.9442761145565,-47.7100684523628,-37.7938303785899));
#19324=CARTESIAN_POINT('Ctrl Pts',(18.1913396767565,-48.0571936627911,-37.7411808708591));
#19325=CARTESIAN_POINT('Ctrl Pts',(17.6263338082825,-48.8119522766749,-37.6885313631283));
#19326=CARTESIAN_POINT('Ctrl Pts',(17.5053953913003,-49.6321858731847,-37.6358818553975));
#19327=CARTESIAN_POINT('Ctrl Pts',(17.3844569743181,-50.4524194696944,-37.5832323476667));
#19328=CARTESIAN_POINT('Ctrl Pts',(17.7075860088279,-51.3381280488302,-37.5305828399359));
#19329=CARTESIAN_POINT('Ctrl Pts',(18.3282968288376,-51.8877891355766,-37.477933332205));
#19330=CARTESIAN_POINT('Ctrl Pts',(18.9490076488472,-52.437450222323,-37.4252838244742));
#19331=CARTESIAN_POINT('Ctrl Pts',(19.8673002543568,-52.65106381668,-37.3726343167433));
#19332=CARTESIAN_POINT('Ctrl Pts',(20.6668806730142,-52.4317914236705,-37.3199848090125));
#19333=CARTESIAN_POINT('Ctrl Pts',(21.4664610916715,-52.212519030661,-37.2673353012817));
#19334=CARTESIAN_POINT('Ctrl Pts',(22.1473293234767,-51.5603606502849,-37.2146857935509));
#19335=CARTESIAN_POINT('Ctrl Pts',(22.4008241013141,-50.7709623772601,-37.1620362858201));
#19336=CARTESIAN_POINT('Ctrl Pts',(22.4801921939607,-50.523805272869,-37.145551958044));
#19337=CARTESIAN_POINT('Ctrl Pts',(22.5176653636715,-50.263194701322,-37.129067630268));
#19338=CARTESIAN_POINT('Ctrl Pts',(22.5156629463979,-50.0020238415623,-37.112583302492));
#19339=CARTESIAN_POINT('Ctrl Pts',(22.5136154336298,-49.9994585736035,-37.387416697508));
#19340=CARTESIAN_POINT('Ctrl Pts',(22.5127373439902,-50.4514337016458,-37.4158856746455));
#19341=CARTESIAN_POINT('Ctrl Pts',(22.3963341785868,-50.9038306788881,-37.444354651783));
#19342=CARTESIAN_POINT('Ctrl Pts',(22.1671363564595,-51.2891312023377,-37.4728236289205));
#19343=CARTESIAN_POINT('Ctrl Pts',(21.7432661046516,-52.0016922047957,-37.5254731366513));
#19344=CARTESIAN_POINT('Ctrl Pts',(20.9336214307039,-52.4847734034993,-37.5781226443822));
#19345=CARTESIAN_POINT('Ctrl Pts',(20.1052424220535,-52.5193774874071,-37.630772152113));
#19346=CARTESIAN_POINT('Ctrl Pts',(19.2768634134032,-52.5539815713149,-37.6834216598438));
#19347=CARTESIAN_POINT('Ctrl Pts',(18.42975007005,-52.140108540427,-37.7360711675746));
#19348=CARTESIAN_POINT('Ctrl Pts',(17.9479283709528,-51.4653810329258,-37.7887206753054));
#19349=CARTESIAN_POINT('Ctrl Pts',(17.4661066718556,-50.7906535254245,-37.8413701830363));
#19350=CARTESIAN_POINT('Ctrl Pts',(17.3495766170143,-49.85507154131,-37.8940196907671));
#19351=CARTESIAN_POINT('Ctrl Pts',(17.6511652816951,-49.0827677555387,-37.9466691984979));
#19352=CARTESIAN_POINT('Ctrl Pts',(17.9527539463759,-48.3104639697674,-37.9993187062287));
#19353=CARTESIAN_POINT('Ctrl Pts',(18.6724613305789,-47.7014383823393,-38.0519682139595));
#19354=CARTESIAN_POINT('Ctrl Pts',(19.4840191417411,-47.531781869955,-38.1046177216904));
#19355=CARTESIAN_POINT('Ctrl Pts',(20.2955769529033,-47.3621253575708,-38.1572672294212));
#19356=CARTESIAN_POINT('Ctrl Pts',(21.1989851910248,-47.6318379202303,-38.209916737152));
#19357=CARTESIAN_POINT('Ctrl Pts',(21.7846972590492,-48.2186526785622,-38.2625662448828));
#19358=CARTESIAN_POINT('Ctrl Pts',(22.2476735206997,-48.6825005620628,-38.3041830624246));
#19359=CARTESIAN_POINT('Ctrl Pts',(22.5121495212431,-49.3444775845434,-38.3457998799663));
#19360=CARTESIAN_POINT('Ctrl Pts',(22.5181182812424,-50.0021988905331,-38.387416697508));
#19361=CARTESIAN_POINT('Origin',(20.,-50.,-32.));
#19362=CARTESIAN_POINT('',(22.5201577888434,-49.9984351914864,-39.387416697508));
#19363=CARTESIAN_POINT('',(22.514945820706,-49.9982392595312,-39.112583302492));
#19364=CARTESIAN_POINT('',(22.5175,-50.,-32.));
#19365=CARTESIAN_POINT('',(18.086534003335,-48.364012796625,-40.));
#19366=CARTESIAN_POINT('Ctrl Pts',(22.5201577888434,-49.9984351914864,-39.387416697508));
#19367=CARTESIAN_POINT('Ctrl Pts',(22.5146851491745,-50.7276238121977,-39.4336626084795));
#19368=CARTESIAN_POINT('Ctrl Pts',(22.1801327508562,-51.4610373176228,-39.4799085194511));
#19369=CARTESIAN_POINT('Ctrl Pts',(21.6226860724328,-51.9298784151162,-39.5261544304226));
#19370=CARTESIAN_POINT('Ctrl Pts',(20.9880506508656,-52.4636391837647,-39.5788039381534));
#19371=CARTESIAN_POINT('Ctrl Pts',(20.064519663454,-52.6544849370069,-39.6314534458842));
#19372=CARTESIAN_POINT('Ctrl Pts',(19.2708508590834,-52.4142812011169,-39.6841029536151));
#19373=CARTESIAN_POINT('Ctrl Pts',(18.4771820547128,-52.1740774652269,-39.7367524613459));
#19374=CARTESIAN_POINT('Ctrl Pts',(17.813375433383,-51.5028242402046,-39.7894019690767));
#19375=CARTESIAN_POINT('Ctrl Pts',(17.5804145739582,-50.7085548746096,-39.8420514768075));
#19376=CARTESIAN_POINT('Ctrl Pts',(17.3474537145333,-49.9142855090145,-39.8947009845384));
#19377=CARTESIAN_POINT('Ctrl Pts',(17.5453386170133,-48.9970000028465,-39.9473504922692));
#19378=CARTESIAN_POINT('Ctrl Pts',(18.086534003335,-48.364012796625,-40.));
#19379=CARTESIAN_POINT('',(21.9170727734079,-48.3614591747396,-40.));
#19380=CARTESIAN_POINT('Origin',(20.,-50.,-40.));
#19381=CARTESIAN_POINT('Ctrl Pts',(21.917080287283,-48.3614538548662,-40.));
#19382=CARTESIAN_POINT('Ctrl Pts',(21.3942484559038,-47.752683457533,-39.9490537266974));
#19383=CARTESIAN_POINT('Ctrl Pts',(20.5545526583696,-47.4126378392115,-39.8981074533947));
#19384=CARTESIAN_POINT('Ctrl Pts',(19.7559044836509,-47.4904266257446,-39.847161180092));
#19385=CARTESIAN_POINT('Ctrl Pts',(18.9305559248023,-47.5708160448806,-39.7945116723612));
#19386=CARTESIAN_POINT('Ctrl Pts',(18.1490454735931,-48.0974449380489,-39.7418621646304));
#19387=CARTESIAN_POINT('Ctrl Pts',(17.7651665960889,-48.8322009125333,-39.6892126568995));
#19388=CARTESIAN_POINT('Ctrl Pts',(17.3812877185847,-49.5669568870177,-39.6365631491687));
#19389=CARTESIAN_POINT('Ctrl Pts',(17.3950404147854,-50.5098399428182,-39.5839136414379));
#19390=CARTESIAN_POINT('Ctrl Pts',(17.8004370773545,-51.2330949973265,-39.5312641337071));
#19391=CARTESIAN_POINT('Ctrl Pts',(18.2058337399236,-51.9563500518348,-39.4786146259763));
#19392=CARTESIAN_POINT('Ctrl Pts',(19.0028743688612,-52.4599771050508,-39.4259651182454));
#19393=CARTESIAN_POINT('Ctrl Pts',(19.8301087009278,-52.5158217813334,-39.3733156105146));
#19394=CARTESIAN_POINT('Ctrl Pts',(20.6573430329945,-52.5716664576159,-39.3206661027838));
#19395=CARTESIAN_POINT('Ctrl Pts',(21.5147710681904,-52.1797287569649,-39.268016595053));
#19396=CARTESIAN_POINT('Ctrl Pts',(22.01375313092,-51.5176086839439,-39.2153670873222));
#19397=CARTESIAN_POINT('Ctrl Pts',(22.3384618647093,-51.0867391465682,-39.1811058257121));
#19398=CARTESIAN_POINT('Ctrl Pts',(22.5113810821265,-50.5414566856712,-39.1468445641021));
#19399=CARTESIAN_POINT('Ctrl Pts',(22.514945820706,-49.9982392595312,-39.112583302492));
#19400=CARTESIAN_POINT('Origin',(20.,-50.,-42.2084234471774));
#19401=CARTESIAN_POINT('',(23.0782115777579,-49.9991816606551,-25.7915765528225));
#19402=CARTESIAN_POINT('',(23.0685693947188,-49.9996667583212,-25.7084234471775));
#19403=CARTESIAN_POINT('',(23.0735,-49.9999999999998,-42.2084234471774));
#19404=CARTESIAN_POINT('',(19.2062007174672,-52.9692229537457,-25.));
#19405=CARTESIAN_POINT('Ctrl Pts',(23.0685693947188,-49.9996667583212,-25.7084234471775));
#19406=CARTESIAN_POINT('Ctrl Pts',(23.0688873842183,-49.5044898373669,-25.6828803290416));
#19407=CARTESIAN_POINT('Ctrl Pts',(22.7226355830855,-47.989181422973,-25.6046877031749));
#19408=CARTESIAN_POINT('Ctrl Pts',(20.3515249129824,-46.3913842077397,-25.4738455695774));
#19409=CARTESIAN_POINT('Ctrl Pts',(17.1680748931287,-47.7313322718094,-25.315897046385));
#19410=CARTESIAN_POINT('Ctrl Pts',(16.5570912657335,-51.1345436021507,-25.1579485231925));
#19411=CARTESIAN_POINT('Ctrl Pts',(18.2239621276955,-52.7066289013681,-25.0526495077308));
#19412=CARTESIAN_POINT('Ctrl Pts',(19.2062007174672,-52.9692229537457,-25.));
#19413=CARTESIAN_POINT('',(20.7937992825328,-52.9692229537457,-25.));
#19414=CARTESIAN_POINT('Origin',(20.,-50.,-25.));
#19415=CARTESIAN_POINT('Ctrl Pts',(23.0782115777579,-49.9991816606551,-25.7915765528225));
#19416=CARTESIAN_POINT('Ctrl Pts',(23.0783675970752,-49.9546737841192,-25.7892620061076));
#19417=CARTESIAN_POINT('Ctrl Pts',(23.0574070137277,-48.8978876848609,-25.7342979516619));
#19418=CARTESIAN_POINT('Ctrl Pts',(21.8481507499307,-46.8799263624337,-25.6266843894854));
#19419=CARTESIAN_POINT('Ctrl Pts',(18.3975850974581,-46.7464741037567,-25.4687358662929));
#19420=CARTESIAN_POINT('Ctrl Pts',(16.3999441875489,-49.5638694433452,-25.3107873431005));
#19421=CARTESIAN_POINT('Ctrl Pts',(17.6525826922257,-52.7401247181454,-25.1545420543361));
#19422=CARTESIAN_POINT('Ctrl Pts',(19.8486501161164,-53.2252254607868,-25.0509462733027));
#19423=CARTESIAN_POINT('Ctrl Pts',(20.7956660331737,-52.9742969611506,-25.));
#19424=CARTESIAN_POINT('Origin',(20.,-50.,-42.2084234471774));
#19425=CARTESIAN_POINT('',(23.0698521513658,-49.9981345322115,-26.7915765528225));
#19426=CARTESIAN_POINT('',(23.0750332840076,-50.0025583317598,-26.7084234471774));
#19427=CARTESIAN_POINT('',(23.0735,-49.9999999999998,-42.2084234471774));
#19428=CARTESIAN_POINT('Ctrl Pts',(23.0750332840076,-50.0025583317598,-26.7084234471774));
#19429=CARTESIAN_POINT('Ctrl Pts',(23.0676453720462,-49.1738259322011,-26.6654440420932));
#19430=CARTESIAN_POINT('Ctrl Pts',(22.2960105484609,-47.3177698442431,-26.5698151292781));
#19431=CARTESIAN_POINT('Ctrl Pts',(19.1670202093295,-46.4705001000209,-26.4215367087323));
#19432=CARTESIAN_POINT('Ctrl Pts',(16.5891690739128,-48.7680163387323,-26.2635881855397));
#19433=CARTESIAN_POINT('Ctrl Pts',(17.1038912274563,-52.1826318884526,-26.1056396623473));
#19434=CARTESIAN_POINT('Ctrl Pts',(20.2442745697777,-53.6181279774832,-25.9476911391548));
#19435=CARTESIAN_POINT('Ctrl Pts',(22.6913964149601,-52.0718621316644,-25.8152857340982));
#19436=CARTESIAN_POINT('Ctrl Pts',(23.0682319438559,-50.5251491393848,-25.7355298367724));
#19437=CARTESIAN_POINT('Ctrl Pts',(23.0685693947188,-49.9996667583212,-25.7084234471775));
#19438=CARTESIAN_POINT('Ctrl Pts',(23.0698521513658,-49.9981345322115,-26.7915765528225));
#19439=CARTESIAN_POINT('Ctrl Pts',(23.0719962440276,-49.6156589519614,-26.7718257191592));
#19440=CARTESIAN_POINT('Ctrl Pts',(22.8290065354064,-48.2162500148277,-26.6994253777651));
#19441=CARTESIAN_POINT('Ctrl Pts',(20.7420732792926,-46.4502604182672,-26.5743755286402));
#19442=CARTESIAN_POINT('Ctrl Pts',(17.4332844917096,-47.4380994344961,-26.4164270054477));
#19443=CARTESIAN_POINT('Ctrl Pts',(16.4516596187905,-50.7487514207967,-26.2584784822553));
#19444=CARTESIAN_POINT('Ctrl Pts',(18.6872050080179,-53.3805021188932,-26.1005299590628));
#19445=CARTESIAN_POINT('Ctrl Pts',(22.0628244523097,-52.9536641922363,-25.9448959825852));
#19446=CARTESIAN_POINT('Ctrl Pts',(23.0748185910436,-50.9671043281552,-25.8419115138385));
#19447=CARTESIAN_POINT('Ctrl Pts',(23.0782115777579,-49.9991816606551,-25.7915765528225));
#19448=CARTESIAN_POINT('Origin',(20.,-50.,-42.2084234471774));
#19449=CARTESIAN_POINT('',(23.0717753507574,-50.0025926098673,-27.7915765528225));
#19450=CARTESIAN_POINT('',(23.0760711510323,-49.9977320015118,-27.7084234471775));
#19451=CARTESIAN_POINT('',(23.0735,-49.9999999999998,-42.2084234471774));
#19452=CARTESIAN_POINT('Ctrl Pts',(23.0760711510323,-49.9977320015118,-27.7084234471775));
#19453=CARTESIAN_POINT('Ctrl Pts',(23.0773102483044,-49.8481151574663,-27.7006572628756));
#19454=CARTESIAN_POINT('Ctrl Pts',(22.9996488588235,-48.6854877487299,-27.640241570843));
#19455=CARTESIAN_POINT('Ctrl Pts',(21.5183205224596,-46.7066670244563,-27.5271763710795));
#19456=CARTESIAN_POINT('Ctrl Pts',(18.0723367598354,-46.9282820340933,-27.369227847887));
#19457=CARTESIAN_POINT('Ctrl Pts',(16.3741060118888,-49.934929517492,-27.2112793246946));
#19458=CARTESIAN_POINT('Ctrl Pts',(17.963364296689,-53.000575988945,-27.053330801502));
#19459=CARTESIAN_POINT('Ctrl Pts',(21.3991757827366,-53.3456883625643,-26.8953822783096));
#19460=CARTESIAN_POINT('Ctrl Pts',(22.9766776415497,-51.388891073304,-26.7804131602014));
#19461=CARTESIAN_POINT('Ctrl Pts',(23.0766955189053,-50.1890180408823,-26.718093549824));
#19462=CARTESIAN_POINT('Ctrl Pts',(23.0750332840076,-50.0025583317598,-26.7084234471774));
#19463=CARTESIAN_POINT('Ctrl Pts',(23.0717753507574,-50.0025926098673,-27.7915765528225));
#19464=CARTESIAN_POINT('Ctrl Pts',(23.0659160187279,-49.2836003637029,-27.7543894322108));
#19465=CARTESIAN_POINT('Ctrl Pts',(22.4567168752833,-47.537712359323,-27.6645528038683));
#19466=CARTESIAN_POINT('Ctrl Pts',(19.556563602243,-46.4007357563187,-27.522066667795));
#19467=CARTESIAN_POINT('Ctrl Pts',(16.7437402241732,-48.4037194119704,-27.3641181446025));
#19468=CARTESIAN_POINT('Ctrl Pts',(16.883268566659,-51.8540023792524,-27.2061696214101));
#19469=CARTESIAN_POINT('Ctrl Pts',(19.8486424758461,-53.6233172761733,-27.0482210982176));
#19470=CARTESIAN_POINT('Ctrl Pts',(22.5632792878361,-52.2970308067085,-26.9100234086884));
#19471=CARTESIAN_POINT('Ctrl Pts',(23.0662807676534,-50.6352184987896,-26.8244752268901));
#19472=CARTESIAN_POINT('Ctrl Pts',(23.0698521513658,-49.9981345322115,-26.7915765528225));
#19473=CARTESIAN_POINT('Origin',(20.,-50.,-42.2084234471774));
#19474=CARTESIAN_POINT('',(23.0782820034225,-49.9993152063967,-28.7915765528225));
#19475=CARTESIAN_POINT('',(23.0686596177156,-49.9996515905093,-28.7084234471774));
#19476=CARTESIAN_POINT('',(23.0735,-49.9999999999998,-42.2084234471774));
#19477=CARTESIAN_POINT('Ctrl Pts',(23.0686596177156,-49.9996515905092,-28.7084234471774));
#19478=CARTESIAN_POINT('Ctrl Pts',(23.0691589034913,-49.5111295556534,-28.6832209759272));
#19479=CARTESIAN_POINT('Ctrl Pts',(22.7295044338491,-48.0027108479738,-28.6053689969462));
#19480=CARTESIAN_POINT('Ctrl Pts',(20.3740253245205,-46.3928620895824,-28.4748675102343));
#19481=CARTESIAN_POINT('Ctrl Pts',(17.1840251210985,-47.7149126304983,-28.3169189870418));
#19482=CARTESIAN_POINT('Ctrl Pts',(16.5471836864498,-51.1087823789649,-28.1589704638494));
#19483=CARTESIAN_POINT('Ctrl Pts',(19.0409058103903,-53.4973528915733,-28.0010219406569));
#19484=CARTESIAN_POINT('Ctrl Pts',(22.2388388670651,-52.7534484207361,-27.8508396017662));
#19485=CARTESIAN_POINT('Ctrl Pts',(23.0689100019457,-50.8624167605561,-27.7533067706064));
#19486=CARTESIAN_POINT('Ctrl Pts',(23.0760711510323,-49.9977320015118,-27.7084234471775));
#19487=CARTESIAN_POINT('Ctrl Pts',(23.0782820034225,-49.9993152063967,-28.7915765528225));
#19488=CARTESIAN_POINT('Ctrl Pts',(23.078397645158,-49.9613596528921,-28.7896026529933));
#19489=CARTESIAN_POINT('Ctrl Pts',(23.060634048498,-48.9111325473444,-28.7349792454332));
#19490=CARTESIAN_POINT('Ctrl Pts',(21.8681385615409,-46.8917211343748,-28.6277063301423));
#19491=CARTESIAN_POINT('Ctrl Pts',(18.4185250934885,-46.7365238921992,-28.4697578069498));
#19492=CARTESIAN_POINT('Ctrl Pts',(16.4027868246521,-49.5402211808024,-28.3118092837573));
#19493=CARTESIAN_POINT('Ctrl Pts',(17.648532337875,-52.7607859452632,-28.1538607605649));
#19494=CARTESIAN_POINT('Ctrl Pts',(21.0262820631638,-53.4782300506355,-27.9959122373724));
#19495=CARTESIAN_POINT('Ctrl Pts',(22.8973566155764,-51.6156342685664,-27.8751508347916));
#19496=CARTESIAN_POINT('Ctrl Pts',(23.0742116582373,-50.3015492449329,-27.8070389399417));
#19497=CARTESIAN_POINT('Ctrl Pts',(23.0717753507574,-50.0025926098673,-27.7915765528225));
#19498=CARTESIAN_POINT('Origin',(20.,-50.,-42.2084234471774));
#19499=CARTESIAN_POINT('',(23.0699777810384,-49.9980579821568,-29.7915765528225));
#19500=CARTESIAN_POINT('',(23.0748402987193,-50.0025957432343,-29.7084234471774));
#19501=CARTESIAN_POINT('',(23.0735,-49.9999999999998,-42.2084234471774));
#19502=CARTESIAN_POINT('Ctrl Pts',(23.0748402987193,-50.0025957432343,-29.7084234471774));
#19503=CARTESIAN_POINT('Ctrl Pts',(23.0674595627731,-49.1802997198265,-29.6657846889788));
#19504=CARTESIAN_POINT('Ctrl Pts',(22.3060144165507,-47.3305807981947,-29.5704964230494));
#19505=CARTESIAN_POINT('Ctrl Pts',(19.1896896511183,-46.4652106179844,-29.4225586493891));
#19506=CARTESIAN_POINT('Ctrl Pts',(16.5971711425799,-48.7461680323328,-29.2646101261967));
#19507=CARTESIAN_POINT('Ctrl Pts',(17.0898940665435,-52.1639367579875,-29.1066616030041));
#19508=CARTESIAN_POINT('Ctrl Pts',(20.2211215338182,-53.6197298387387,-28.9487130798117));
#19509=CARTESIAN_POINT('Ctrl Pts',(22.6842316286424,-52.0849997853531,-28.8159670278695));
#19510=CARTESIAN_POINT('Ctrl Pts',(23.0681158648922,-50.5316820401877,-28.735870483658));
#19511=CARTESIAN_POINT('Ctrl Pts',(23.0686596177156,-49.9996515905092,-28.7084234471774));
#19512=CARTESIAN_POINT('Ctrl Pts',(23.0699777810384,-49.9980579821568,-29.7915765528226));
#19513=CARTESIAN_POINT('Ctrl Pts',(23.0721774154546,-49.6222177557946,-29.7721663660449));
#19514=CARTESIAN_POINT('Ctrl Pts',(22.8347477112605,-48.2296051243342,-29.7001066715364));
#19515=CARTESIAN_POINT('Ctrl Pts',(20.7648507240798,-46.4550962552107,-29.5753974692971));
#19516=CARTESIAN_POINT('Ctrl Pts',(17.4497876216902,-47.4216757350208,-29.4174489461046));
#19517=CARTESIAN_POINT('Ctrl Pts',(16.4469245215085,-50.7259434096673,-29.2595004229122));
#19518=CARTESIAN_POINT('Ctrl Pts',(18.6655268957734,-53.3720202734039,-29.1015518997197));
#19519=CARTESIAN_POINT('Ctrl Pts',(22.0512087542155,-52.9659281134316,-28.9455772763565));
#19520=CARTESIAN_POINT('Ctrl Pts',(23.0753131520357,-50.9737419318929,-28.8422521607241));
#19521=CARTESIAN_POINT('Ctrl Pts',(23.0782820034225,-49.9993152063967,-28.7915765528225));
#19522=CARTESIAN_POINT('Origin',(20.,-50.,-42.2084234471774));
#19523=CARTESIAN_POINT('',(23.0715992618133,-50.0025559506913,-30.7915765528225));
#19524=CARTESIAN_POINT('',(23.0762469243503,-49.9977977477149,-30.7084234471774));
#19525=CARTESIAN_POINT('',(23.0735,-49.9999999999998,-42.2084234471774));
#19526=CARTESIAN_POINT('Ctrl Pts',(23.0762469243503,-49.9977977477149,-30.7084234471774));
#19527=CARTESIAN_POINT('Ctrl Pts',(23.0774077652693,-49.8547648430612,-30.7009979097613));
#19528=CARTESIAN_POINT('Ctrl Pts',(23.0036028704742,-48.6987851837245,-30.6409228646142));
#19529=CARTESIAN_POINT('Ctrl Pts',(21.5394357941431,-46.7164841598999,-30.5281983117364));
#19530=CARTESIAN_POINT('Ctrl Pts',(18.0920998235166,-46.9159676147846,-30.3702497885439));
#19531=CARTESIAN_POINT('Ctrl Pts',(16.3745989167479,-49.9116494367408,-30.2123012653515));
#19532=CARTESIAN_POINT('Ctrl Pts',(17.9441389105717,-52.98743602734,-30.054352742159));
#19533=CARTESIAN_POINT('Ctrl Pts',(21.3776656279966,-53.354605230716,-29.8964042189665));
#19534=CARTESIAN_POINT('Ctrl Pts',(22.9724077934703,-51.4022058860543,-29.7810944539727));
#19535=CARTESIAN_POINT('Ctrl Pts',(23.0765731516926,-50.1956548256145,-29.7184341967096));
#19536=CARTESIAN_POINT('Ctrl Pts',(23.0748402987193,-50.0025957432343,-29.7084234471774));
#19537=CARTESIAN_POINT('Ctrl Pts',(23.0715992618133,-50.0025559506913,-30.7915765528225));
#19538=CARTESIAN_POINT('Ctrl Pts',(23.0659003196299,-49.2900463831274,-30.7547300790965));
#19539=CARTESIAN_POINT('Ctrl Pts',(22.465560668895,-47.5507750303684,-30.6652340976396));
#19540=CARTESIAN_POINT('Ctrl Pts',(19.5796836114642,-46.3979626149297,-30.5230886084519));
#19541=CARTESIAN_POINT('Ctrl Pts',(16.7540570706331,-48.3828439502611,-30.3651400852594));
#19542=CARTESIAN_POINT('Ctrl Pts',(16.8714282629673,-51.8339514923121,-30.207191562067));
#19543=CARTESIAN_POINT('Ctrl Pts',(19.8253802980609,-53.6222709933982,-30.0492430388745));
#19544=CARTESIAN_POINT('Ctrl Pts',(22.5551894171279,-52.3102156517629,-29.9107047024597));
#19545=CARTESIAN_POINT('Ctrl Pts',(23.0662109778037,-50.6416722891319,-29.8248158737757));
#19546=CARTESIAN_POINT('Ctrl Pts',(23.0699777810384,-49.9980579821568,-29.7915765528226));
#19547=CARTESIAN_POINT('Origin',(20.,-50.,-42.2084234471774));
#19548=CARTESIAN_POINT('',(23.0783412386193,-49.9994310992988,-31.7915765528225));
#19549=CARTESIAN_POINT('',(23.0686854942479,-49.9995466737535,-31.7084234471775));
#19550=CARTESIAN_POINT('',(23.0735,-49.9999999999998,-42.2084234471774));
#19551=CARTESIAN_POINT('Ctrl Pts',(23.0686854942479,-49.9995466737535,-31.7084234471775));
#19552=CARTESIAN_POINT('Ctrl Pts',(23.0693266584817,-49.5176378585812,-31.6835616228129));
#19553=CARTESIAN_POINT('Ctrl Pts',(22.7361513781682,-48.0160365980268,-31.6060502907174));
#19554=CARTESIAN_POINT('Ctrl Pts',(20.3971790421746,-46.3953380678715,-31.4758894508912));
#19555=CARTESIAN_POINT('Ctrl Pts',(17.1987557115146,-47.6968783634582,-31.3179409276987));
#19556=CARTESIAN_POINT('Ctrl Pts',(16.5401353812306,-51.0865890006191,-31.1599924045063));
#19557=CARTESIAN_POINT('Ctrl Pts',(19.018469073759,-53.4911224380292,-31.0020438813138));
#19558=CARTESIAN_POINT('Ctrl Pts',(22.228377153031,-52.7661265353208,-30.8515208955375));
#19559=CARTESIAN_POINT('Ctrl Pts',(23.0691770205416,-50.8689152805637,-30.7536474174921));
#19560=CARTESIAN_POINT('Ctrl Pts',(23.0762469243503,-49.9977977477149,-30.7084234471774));
#19561=CARTESIAN_POINT('Ctrl Pts',(23.0783412386193,-49.9994310992988,-31.7915765528225));
#19562=CARTESIAN_POINT('Ctrl Pts',(23.0784219203286,-49.9680273678988,-31.7899432998789));
#19563=CARTESIAN_POINT('Ctrl Pts',(23.0638170352735,-48.9243704639443,-31.7356605392044));
#19564=CARTESIAN_POINT('Ctrl Pts',(21.888058303827,-46.9037805259858,-31.6287282707992));
#19565=CARTESIAN_POINT('Ctrl Pts',(18.4395124701376,-46.7264365197756,-31.4707797476067));
#19566=CARTESIAN_POINT('Ctrl Pts',(16.4058132196916,-49.5171329601522,-31.3128312244143));
#19567=CARTESIAN_POINT('Ctrl Pts',(17.6308538107017,-52.7456302598216,-31.1548827012217));
#19568=CARTESIAN_POINT('Ctrl Pts',(21.0039271972243,-53.4847481074805,-30.9969341780293));
#19569=CARTESIAN_POINT('Ctrl Pts',(22.8922345046466,-51.6289848188323,-30.8758321285629));
#19570=CARTESIAN_POINT('Ctrl Pts',(23.0740434733756,-50.308143210103,-30.8073795868273));
#19571=CARTESIAN_POINT('Ctrl Pts',(23.0715992618133,-50.0025559506913,-30.7915765528225));
#19572=CARTESIAN_POINT('Origin',(20.,-50.,-42.2084234471774));
#19573=CARTESIAN_POINT('',(23.070108680638,-49.9979840332082,-32.7915765528225));
#19574=CARTESIAN_POINT('',(23.0746461191906,-50.0026288889103,-32.7084234471774));
#19575=CARTESIAN_POINT('',(23.0735,-49.9999999999998,-42.2084234471774));
#19576=CARTESIAN_POINT('Ctrl Pts',(23.0746461191906,-50.0026288889103,-32.7084234471774));
#19577=CARTESIAN_POINT('Ctrl Pts',(23.0672844312647,-49.1867693456356,-32.6661253358645));
#19578=CARTESIAN_POINT('Ctrl Pts',(22.3159443950164,-47.3434040754006,-32.5711777168206));
#19579=CARTESIAN_POINT('Ctrl Pts',(19.2124032325014,-46.4600804856177,-32.4235805900461));
#19580=CARTESIAN_POINT('Ctrl Pts',(16.6052921443043,-48.7243443211601,-32.2656320668535));
#19581=CARTESIAN_POINT('Ctrl Pts',(17.0760594234942,-52.145206363393,-32.1076835436611));
#19582=CARTESIAN_POINT('Ctrl Pts',(20.1978746957691,-53.6210750394396,-31.9497350204685));
#19583=CARTESIAN_POINT('Ctrl Pts',(22.6771343927214,-52.0982945627933,-31.8166483216408));
#19584=CARTESIAN_POINT('Ctrl Pts',(23.067968874725,-50.5381688348235,-31.7362111305437));
#19585=CARTESIAN_POINT('Ctrl Pts',(23.0686854942479,-49.9995466737535,-31.7084234471775));
#19586=CARTESIAN_POINT('Ctrl Pts',(23.070108680638,-49.9979840332082,-32.7915765528225));
#19587=CARTESIAN_POINT('Ctrl Pts',(23.072358139719,-49.6287793568666,-32.7725070129305));
#19588=CARTESIAN_POINT('Ctrl Pts',(22.8404342309996,-48.2429602032945,-32.7007879653077));
#19589=CARTESIAN_POINT('Ctrl Pts',(20.7875967780819,-46.4600804380509,-32.576419409954));
#19590=CARTESIAN_POINT('Ctrl Pts',(17.4663956098388,-47.4053539771154,-32.4184708867615));
#19591=CARTESIAN_POINT('Ctrl Pts',(16.4423364860605,-50.7031141525378,-32.2605223635691));
#19592=CARTESIAN_POINT('Ctrl Pts',(18.6439026689266,-53.3633821101044,-32.1025738403766));
#19593=CARTESIAN_POINT('Ctrl Pts',(22.0395220840648,-52.978198375694,-31.9462585701278));
#19594=CARTESIAN_POINT('Ctrl Pts',(23.0758210664351,-50.9803573964871,-31.8425928076097));
#19595=CARTESIAN_POINT('Ctrl Pts',(23.0783412386193,-49.9994310992988,-31.7915765528225));
#19596=CARTESIAN_POINT('Origin',(20.,-50.,-42.2084234471774));
#19597=CARTESIAN_POINT('',(23.071426479794,-50.0025153263093,-33.7915765528226));
#19598=CARTESIAN_POINT('',(23.0764188231986,-49.997867531766,-33.7084234471775));
#19599=CARTESIAN_POINT('',(23.0735,-49.9999999999998,-42.2084234471774));
#19600=CARTESIAN_POINT('Ctrl Pts',(23.0764188231986,-49.997867531766,-33.7084234471775));
#19601=CARTESIAN_POINT('Ctrl Pts',(23.0775013376664,-49.8614161856796,-33.7013385566469));
#19602=CARTESIAN_POINT('Ctrl Pts',(23.0075099798091,-48.7120794545905,-33.6416041583855));
#19603=CARTESIAN_POINT('Ctrl Pts',(21.5604875088938,-46.7264365637634,-33.5292202523933));
#19604=CARTESIAN_POINT('Ctrl Pts',(18.1119417215434,-46.9037805675905,-33.3712717292008));
#19605=CARTESIAN_POINT('Ctrl Pts',(16.3752409525729,-49.8883725635259,-33.2133232060083));
#19606=CARTESIAN_POINT('Ctrl Pts',(17.9249989698413,-52.9741737611174,-33.0553746828159));
#19607=CARTESIAN_POINT('Ctrl Pts',(21.3560973128511,-53.3633820649098,-32.8974261596234));
#19608=CARTESIAN_POINT('Ctrl Pts',(22.9680910641118,-51.4155254173783,-32.7817757477439));
#19609=CARTESIAN_POINT('Ctrl Pts',(23.076447706724,-50.2022899444883,-32.7187748435953));
#19610=CARTESIAN_POINT('Ctrl Pts',(23.0746461191906,-50.0026288889103,-32.7084234471774));
#19611=CARTESIAN_POINT('Ctrl Pts',(23.0714264797939,-50.0025153263093,-33.7915765528226));
#19612=CARTESIAN_POINT('Ctrl Pts',(23.0658929944555,-49.2964923448543,-33.7550707259821));
#19613=CARTESIAN_POINT('Ctrl Pts',(22.4743382857738,-47.5638498555385,-33.6659153914109));
#19614=CARTESIAN_POINT('Ctrl Pts',(19.6028209524885,-46.3953380194348,-33.5241105491088));
#19615=CARTESIAN_POINT('Ctrl Pts',(16.7645077415746,-48.362035093299,-33.3661620259164));
#19616=CARTESIAN_POINT('Ctrl Pts',(16.8597169583261,-51.8138251316183,-33.2082135027239));
#19617=CARTESIAN_POINT('Ctrl Pts',(19.8021253015719,-53.621075088097,-33.0502649795314));
#19618=CARTESIAN_POINT('Ctrl Pts',(22.5470356567185,-52.3233918947014,-32.9113859962309));
#19619=CARTESIAN_POINT('Ctrl Pts',(23.0661475591835,-50.6481245834092,-32.8251565206613));
#19620=CARTESIAN_POINT('Ctrl Pts',(23.070108680638,-49.9979840332082,-32.7915765528225));
#19621=CARTESIAN_POINT('Origin',(20.,-50.,-42.2084234471774));
#19622=CARTESIAN_POINT('',(23.0783901429301,-49.9995482667377,-34.7915765528226));
#19623=CARTESIAN_POINT('',(23.0687181382264,-49.9994424172299,-34.7084234471775));
#19624=CARTESIAN_POINT('',(23.0735,-49.9999999999998,-42.2084234471774));
#19625=CARTESIAN_POINT('Ctrl Pts',(23.0687181382264,-49.9994424172299,-34.7084234471775));
#19626=CARTESIAN_POINT('Ctrl Pts',(23.0694964277012,-49.5241491644738,-34.6839022696985));
#19627=CARTESIAN_POINT('Ctrl Pts',(22.7427399824597,-48.0293655359017,-34.6067315844887));
#19628=CARTESIAN_POINT('Ctrl Pts',(20.420316382888,-46.3979626633313,-34.4769113915481));
#19629=CARTESIAN_POINT('Ctrl Pts',(17.213601799006,-47.6789390568155,-34.3189628683557));
#19630=CARTESIAN_POINT('Ctrl Pts',(16.5332297194947,-51.0643508156075,-34.1610143451632));
#19631=CARTESIAN_POINT('Ctrl Pts',(18.9960728162657,-53.4847480606549,-34.0030658219707));
#19632=CARTESIAN_POINT('Ctrl Pts',(22.217844613828,-52.7787838660493,-33.8522021893088));
#19633=CARTESIAN_POINT('Ctrl Pts',(23.0694569150187,-50.875418613757,-33.7539880643777));
#19634=CARTESIAN_POINT('Ctrl Pts',(23.0764188231986,-49.997867531766,-33.7084234471775));
#19635=CARTESIAN_POINT('Ctrl Pts',(23.0783901429301,-49.9995482667377,-34.7915765528226));
#19636=CARTESIAN_POINT('Ctrl Pts',(23.0784416291869,-49.9746954594268,-34.7902839467646));
#19637=CARTESIAN_POINT('Ctrl Pts',(23.06695636405,-48.9376046282268,-34.7363418329757));
#19638=CARTESIAN_POINT('Ctrl Pts',(21.9079002021205,-46.9159675733437,-34.6297502114561));
#19639=CARTESIAN_POINT('Ctrl Pts',(18.4605641851711,-46.7164841157783,-34.4718016882636));
#19640=CARTESIAN_POINT('Ctrl Pts',(16.4089878017039,-49.4940646468145,-34.3138531650711));
#19641=CARTESIAN_POINT('Ctrl Pts',(17.6132729627324,-52.7303613752562,-34.1559046418787));
#19642=CARTESIAN_POINT('Ctrl Pts',(20.98153093943,-53.4911224849404,-33.9979561186862));
#19643=CARTESIAN_POINT('Ctrl Pts',(22.887060184286,-51.6423364239543,-33.8765134223342));
#19644=CARTESIAN_POINT('Ctrl Pts',(23.0738735089191,-50.3147342431337,-33.8077202337129));
#19645=CARTESIAN_POINT('Ctrl Pts',(23.0714264797939,-50.0025153263093,-33.7915765528226));
#19646=CARTESIAN_POINT('Origin',(20.,-50.,-42.2084234471774));
#19647=CARTESIAN_POINT('',(23.070244715626,-49.9979131053482,-35.7915765528225));
#19648=CARTESIAN_POINT('',(23.0744509199104,-50.0026575649045,-35.7084234471775));
#19649=CARTESIAN_POINT('',(23.0735,-49.9999999999998,-42.2084234471774));
#19650=CARTESIAN_POINT('Ctrl Pts',(23.0744509199104,-50.0026575649045,-35.7084234471775));
#19651=CARTESIAN_POINT('Ctrl Pts',(23.0671206442753,-49.1932360925919,-35.6664659827501));
#19652=CARTESIAN_POINT('Ctrl Pts',(22.325805068483,-47.3562448982243,-35.5718590105919));
#19653=CARTESIAN_POINT('Ctrl Pts',(19.2351492861978,-46.4550963028444,-35.4246025307029));
#19654=CARTESIAN_POINT('Ctrl Pts',(16.613553108674,-48.7025732048773,-35.2666540075104));
#19655=CARTESIAN_POINT('Ctrl Pts',(17.0623453333896,-52.1263875225874,-35.108705484318));
#19656=CARTESIAN_POINT('Ctrl Pts',(20.1746196995926,-53.6222709447248,-34.9507569611255));
#19657=CARTESIAN_POINT('Ctrl Pts',(22.6699768333288,-52.111584321713,-34.817329615412));
#19658=CARTESIAN_POINT('Ctrl Pts',(23.0678253595906,-50.5446530047506,-34.7365517774293));
#19659=CARTESIAN_POINT('Ctrl Pts',(23.0687181382264,-49.9994424172299,-34.7084234471775));
#19660=CARTESIAN_POINT('Ctrl Pts',(23.070244715626,-49.9979131053482,-35.7915765528225));
#19661=CARTESIAN_POINT('Ctrl Pts',(23.0725383031763,-49.6353441091479,-35.7728476598162));
#19662=CARTESIAN_POINT('Ctrl Pts',(22.8460663522941,-48.2563155171469,-35.7014692590789));
#19663=CARTESIAN_POINT('Ctrl Pts',(20.81031035977,-46.4652105704865,-35.5774413506109));
#19664=CARTESIAN_POINT('Ctrl Pts',(17.4831080575873,-47.3891391955688,-35.4194928274184));
#19665=CARTESIAN_POINT('Ctrl Pts',(16.4378951318222,-50.6802559062359,-35.261544304226));
#19666=CARTESIAN_POINT('Ctrl Pts',(18.6223343534913,-53.3546052757928,-35.1035957810335));
#19667=CARTESIAN_POINT('Ctrl Pts',(22.0277621047601,-52.9904408764762,-34.946939863899));
#19668=CARTESIAN_POINT('Ctrl Pts',(23.0763445277092,-50.9869822753117,-34.8429334544954));
#19669=CARTESIAN_POINT('Ctrl Pts',(23.0783901429301,-49.9995482667377,-34.7915765528226));
#19670=CARTESIAN_POINT('Origin',(20.,-50.,-42.2084234471774));
#19671=CARTESIAN_POINT('',(23.0712572257215,-50.0024708151107,-36.7915765528225));
#19672=CARTESIAN_POINT('',(23.0765864796728,-49.9979412458126,-36.7084234471775));
#19673=CARTESIAN_POINT('',(23.0735,-49.9999999999998,-42.2084234471774));
#19674=CARTESIAN_POINT('Ctrl Pts',(23.0765864796728,-49.9979412458126,-36.7084234471775));
#19675=CARTESIAN_POINT('Ctrl Pts',(23.0775908951925,-49.868069099325,-36.7016792035325));
#19676=CARTESIAN_POINT('Ctrl Pts',(23.0113703825189,-48.7253704994309,-36.6422854521568));
#19677=CARTESIAN_POINT('Ctrl Pts',(21.581474885261,-46.7365239360518,-36.5302421930502));
#19678=CARTESIAN_POINT('Ctrl Pts',(18.1318614635619,-46.8917211761413,-36.3722936698578));
#19679=CARTESIAN_POINT('Ctrl Pts',(16.3760324359193,-49.8651002928142,-36.2143451466652));
#19680=CARTESIAN_POINT('Ctrl Pts',(17.905944580671,-52.960788870692,-36.0563966234728));
#19681=CARTESIAN_POINT('Ctrl Pts',(21.3344730862948,-53.3720202280932,-35.8984481002803));
#19682=CARTESIAN_POINT('Ctrl Pts',(22.963725640928,-51.4288475622717,-35.7824570415152));
#19683=CARTESIAN_POINT('Ctrl Pts',(23.0763188980065,-50.2089228755193,-35.7191154904809));
#19684=CARTESIAN_POINT('Ctrl Pts',(23.0744509199104,-50.0026575649045,-35.7084234471775));
#19685=CARTESIAN_POINT('Ctrl Pts',(23.0712572257215,-50.0024708151107,-36.7915765528225));
#19686=CARTESIAN_POINT('Ctrl Pts',(23.0658938563175,-49.302938396495,-36.7554113728678));
#19687=CARTESIAN_POINT('Ctrl Pts',(22.4830499320534,-47.5769365408491,-36.6665966851821));
#19688=CARTESIAN_POINT('Ctrl Pts',(19.625974670453,-46.3928620411136,-36.5251324897657));
#19689=CARTESIAN_POINT('Ctrl Pts',(16.775091810017,-48.3412937699339,-36.3671839665732));
#19690=CARTESIAN_POINT('Ctrl Pts',(16.8481351267915,-51.7936239871129,-36.2092354433808));
#19691=CARTESIAN_POINT('Ctrl Pts',(19.7788784632106,-53.6197298873777,-36.0512869201883));
#19692=CARTESIAN_POINT('Ctrl Pts',(22.538817759059,-52.3365588076076,-35.9120672900022));
#19693=CARTESIAN_POINT('Ctrl Pts',(23.0660907114569,-50.6545756868969,-35.825497167547));
#19694=CARTESIAN_POINT('Ctrl Pts',(23.070244715626,-49.9979131053482,-35.7915765528225));
#19695=CARTESIAN_POINT('Origin',(20.,-50.,-42.2084234471774));
#19696=CARTESIAN_POINT('',(23.0784283983202,-49.9996663588637,-37.7915765528226));
#19697=CARTESIAN_POINT('',(23.0687575115238,-49.9993389974064,-37.7084234471775));
#19698=CARTESIAN_POINT('',(23.0735,-49.9999999999998,-42.2084234471774));
#19699=CARTESIAN_POINT('Ctrl Pts',(23.0687575115238,-49.9993389974064,-37.7084234471775));
#19700=CARTESIAN_POINT('Ctrl Pts',(23.0696680463346,-49.5306635124935,-37.6842429165841));
#19701=CARTESIAN_POINT('Ctrl Pts',(22.749270481726,-48.0426974119101,-37.60741287826));
#19702=CARTESIAN_POINT('Ctrl Pts',(20.4434363918007,-46.4007358047025,-37.477933332205));
#19703=CARTESIAN_POINT('Ctrl Pts',(17.228562769865,-47.6610954290179,-37.3199848090125));
#19704=CARTESIAN_POINT('Ctrl Pts',(16.5264669908866,-51.0420687566668,-37.1620362858201));
#19705=CARTESIAN_POINT('Ctrl Pts',(18.9737179506262,-53.4782300038948,-37.0040877626276));
#19706=CARTESIAN_POINT('Ctrl Pts',(22.2072411043633,-52.7914200520352,-36.85288348308));
#19707=CARTESIAN_POINT('Ctrl Pts',(23.069749840591,-50.8819269817663,-36.7543287112634));
#19708=CARTESIAN_POINT('Ctrl Pts',(23.0765864796728,-49.9979412458126,-36.7084234471775));
#19709=CARTESIAN_POINT('Ctrl Pts',(23.0784283983202,-49.9996663588637,-37.7915765528226));
#19710=CARTESIAN_POINT('Ctrl Pts',(23.0784568430445,-49.981363743946,-37.7906245936502));
#19711=CARTESIAN_POINT('Ctrl Pts',(23.0700523868523,-48.9508348052474,-37.737023126747));
#19712=CARTESIAN_POINT('Ctrl Pts',(21.9276632661251,-46.9282819927009,-37.630772152113));
#19713=CARTESIAN_POINT('Ctrl Pts',(18.4816794571067,-46.7066669802649,-37.4728236289205));
#19714=CARTESIAN_POINT('Ctrl Pts',(16.4123103964255,-49.471017248116,-37.314875105728));
#19715=CARTESIAN_POINT('Ctrl Pts',(17.5957905404958,-52.7149798911831,-37.1569265825356));
#19716=CARTESIAN_POINT('Ctrl Pts',(20.9590942025022,-53.497352938559,-36.9989780593431));
#19717=CARTESIAN_POINT('Ctrl Pts',(22.8818334298203,-51.6556889545473,-36.8771947161054));
#19718=CARTESIAN_POINT('Ctrl Pts',(23.0737018849034,-50.3213223096376,-36.8080608805986));
#19719=CARTESIAN_POINT('Ctrl Pts',(23.0712572257215,-50.0024708151107,-36.7915765528225));
#19720=CARTESIAN_POINT('Origin',(20.,-50.,-42.2084234471774));
#19721=CARTESIAN_POINT('',(23.0703817199364,-49.9978503929169,-38.7915765528226));
#19722=CARTESIAN_POINT('',(23.0742548311415,-50.0026845243509,-38.7084234471775));
#19723=CARTESIAN_POINT('',(23.0735,-49.9999999999998,-42.2084234471774));
#19724=CARTESIAN_POINT('Ctrl Pts',(23.0742548311415,-50.0026845243509,-38.7084234471775));
#19725=CARTESIAN_POINT('Ctrl Pts',(23.0669678464909,-49.1997028226788,-38.6668066296357));
#19726=CARTESIAN_POINT('Ctrl Pts',(22.3355968763498,-47.3690990017349,-38.5725403043632));
#19727=CARTESIAN_POINT('Ctrl Pts',(19.257926730837,-46.4502604667964,-38.4256244713598));
#19728=CARTESIAN_POINT('Ctrl Pts',(16.6219537671653,-48.6808544802542,-38.2676759481673));
#19729=CARTESIAN_POINT('Ctrl Pts',(17.0487523255225,-52.107481564476,-38.1097274249749));
#19730=CARTESIAN_POINT('Ctrl Pts',(20.1513575221015,-53.6233172273567,-37.9517789017824));
#19731=CARTESIAN_POINT('Ctrl Pts',(22.6627587165777,-52.1248689098524,-37.8180109091833));
#19732=CARTESIAN_POINT('Ctrl Pts',(23.0676854922557,-50.5511346502516,-37.736892424315));
#19733=CARTESIAN_POINT('Ctrl Pts',(23.0687575115238,-49.9993389974064,-37.7084234471775));
#19734=CARTESIAN_POINT('Ctrl Pts',(23.0703817199364,-49.9978503929169,-38.7915765528226));
#19735=CARTESIAN_POINT('Ctrl Pts',(23.072717480822,-49.6419123660289,-38.7731883067018));
#19736=CARTESIAN_POINT('Ctrl Pts',(22.8516587059108,-48.2696526564415,-38.7021505528502));
#19737=CARTESIAN_POINT('Ctrl Pts',(20.8329798036235,-46.4705000476597,-38.5784632912678));
#19738=CARTESIAN_POINT('Ctrl Pts',(17.4999296646635,-47.373025224819,-38.4205147680753));
#19739=CARTESIAN_POINT('Ctrl Pts',(16.4335979353407,-50.6573730457065,-38.2625662448828));
#19740=CARTESIAN_POINT('Ctrl Pts',(18.600824198122,-53.3456884082951,-38.1046177216904));
#19741=CARTESIAN_POINT('Ctrl Pts',(22.0159280202989,-53.0026560286412,-37.9476211576702));
#19742=CARTESIAN_POINT('Ctrl Pts',(23.0768836655619,-50.9936168883794,-37.843274101381));
#19743=CARTESIAN_POINT('Ctrl Pts',(23.0784283983202,-49.9996663588637,-37.7915765528226));
#19744=CARTESIAN_POINT('Origin',(20.,-50.,-42.2084234471774));
#19745=CARTESIAN_POINT('',(23.0703065393339,-50.0033432771247,-39.7915765528225));
#19746=CARTESIAN_POINT('',(23.0767447721987,-49.9980895972328,-39.7084234471774));
#19747=CARTESIAN_POINT('',(23.0735,-49.9999999999998,-42.2084234471774));
#19748=CARTESIAN_POINT('',(20.7937992825328,-52.9692229537457,-40.));
#19749=CARTESIAN_POINT('Ctrl Pts',(20.7937992825328,-52.9692229537457,-40.));
#19750=CARTESIAN_POINT('Ctrl Pts',(21.7760378723045,-52.7066289013681,-39.9473504922692));
#19751=CARTESIAN_POINT('Ctrl Pts',(22.8758105836868,-51.6693936165595,-39.8778760098767));
#19752=CARTESIAN_POINT('Ctrl Pts',(23.0726592954589,-50.3288663223125,-39.8084015274842));
#19753=CARTESIAN_POINT('Ctrl Pts',(23.0703065393339,-50.0033432771247,-39.7915765528225));
#19754=CARTESIAN_POINT('',(19.2043379022879,-52.9742864271603,-40.));
#19755=CARTESIAN_POINT('Origin',(20.,-50.,-40.));
#19756=CARTESIAN_POINT('Ctrl Pts',(19.2043340224364,-52.9742969733088,-40.));
#19757=CARTESIAN_POINT('Ctrl Pts',(20.1513499766094,-53.2252255075611,-39.9490537266973));
#19758=CARTESIAN_POINT('Ctrl Pts',(22.2116710273535,-52.7701102416077,-39.8518615424232));
#19759=CARTESIAN_POINT('Ctrl Pts',(23.0700634780488,-50.8883224575133,-39.754669358149));
#19760=CARTESIAN_POINT('Ctrl Pts',(23.0767447721987,-49.9980895972329,-39.7084234471774));
#19761=CARTESIAN_POINT('Origin',(20.,50.,-42.2084234471774));
#19762=CARTESIAN_POINT('',(23.0782114598495,50.0008183538095,-25.7915765528225));
#19763=CARTESIAN_POINT('',(23.0685692638887,50.000333297858,-25.7084234471774));
#19764=CARTESIAN_POINT('',(23.0735,50.0000000000002,-42.2084234471774));
#19765=CARTESIAN_POINT('',(19.2062007174672,47.0307770462543,-25.));
#19766=CARTESIAN_POINT('Ctrl Pts',(23.0685692638887,50.000333297858,-25.7084234471774));
#19767=CARTESIAN_POINT('Ctrl Pts',(23.068887248526,50.495510231703,-25.6828803290416));
#19768=CARTESIAN_POINT('Ctrl Pts',(22.7226354451561,52.0108186486332,-25.6046877031749));
#19769=CARTESIAN_POINT('Ctrl Pts',(20.3515248813337,53.6086151161717,-25.4738455695774));
#19770=CARTESIAN_POINT('Ctrl Pts',(17.1680751579223,52.2686685512262,-25.3158970463849));
#19771=CARTESIAN_POINT('Ctrl Pts',(16.5570909615237,48.8654544718428,-25.1579485231925));
#19772=CARTESIAN_POINT('Ctrl Pts',(18.2239621276955,47.2933710986319,-25.0526495077308));
#19773=CARTESIAN_POINT('Ctrl Pts',(19.2062007174672,47.0307770462543,-25.));
#19774=CARTESIAN_POINT('',(20.7937992825328,47.0307770462543,-25.));
#19775=CARTESIAN_POINT('Origin',(20.,50.,-25.));
#19776=CARTESIAN_POINT('Ctrl Pts',(23.0782114598495,50.0008183538095,-25.7915765528225));
#19777=CARTESIAN_POINT('Ctrl Pts',(23.0783674790197,50.0453262282883,-25.7892620061076));
#19778=CARTESIAN_POINT('Ctrl Pts',(23.057406892625,51.1021122772341,-25.7342979516619));
#19779=CARTESIAN_POINT('Ctrl Pts',(21.8481506426783,53.1200734299207,-25.6266843894854));
#19780=CARTESIAN_POINT('Ctrl Pts',(18.3975852298821,53.2535259099818,-25.4687358662929));
#19781=CARTESIAN_POINT('Ctrl Pts',(16.3999441908908,50.4361302999107,-25.3107873431005));
#19782=CARTESIAN_POINT('Ctrl Pts',(17.6525830669794,47.2598757730875,-25.1545420543361));
#19783=CARTESIAN_POINT('Ctrl Pts',(19.8486498414593,46.7747744006132,-25.0509462733027));
#19784=CARTESIAN_POINT('Ctrl Pts',(20.7956658684167,47.0257030027424,-25.));
#19785=CARTESIAN_POINT('Origin',(20.,50.,-42.2084234471774));
#19786=CARTESIAN_POINT('',(23.0698520292984,50.0018654680674,-26.7915765528225));
#19787=CARTESIAN_POINT('',(23.0750331521824,49.9974416679533,-26.7084234471775));
#19788=CARTESIAN_POINT('',(23.0735,50.0000000000002,-42.2084234471774));
#19789=CARTESIAN_POINT('Ctrl Pts',(23.0750331521824,49.9974416679533,-26.7084234471775));
#19790=CARTESIAN_POINT('Ctrl Pts',(23.0676452399249,50.8261740335002,-26.6654440420932));
#19791=CARTESIAN_POINT('Ctrl Pts',(22.2960104470904,52.682230047647,-26.5698151292781));
#19792=CARTESIAN_POINT('Ctrl Pts',(19.1670202507297,53.5294997326245,-26.4215367087322));
#19793=CARTESIAN_POINT('Ctrl Pts',(16.5891692111351,51.2319836373097,-26.2635881855398));
#19794=CARTESIAN_POINT('Ctrl Pts',(17.1038913663152,47.8173681526091,-26.1056396623473));
#19795=CARTESIAN_POINT('Ctrl Pts',(20.2442745382167,46.3818722728576,-25.9476911391548));
#19796=CARTESIAN_POINT('Ctrl Pts',(22.6913963181601,47.9281378306177,-25.8152857340982));
#19797=CARTESIAN_POINT('Ctrl Pts',(23.0682318181854,49.4748509031148,-25.7355298367724));
#19798=CARTESIAN_POINT('Ctrl Pts',(23.0685692638887,50.000333297858,-25.7084234471774));
#19799=CARTESIAN_POINT('Ctrl Pts',(23.0698520292984,50.0018654680674,-26.7915765528225));
#19800=CARTESIAN_POINT('Ctrl Pts',(23.0719961218878,50.3843410331866,-26.7718257191592));
#19801=CARTESIAN_POINT('Ctrl Pts',(22.8290064229413,51.7837499147479,-26.6994253777651));
#19802=CARTESIAN_POINT('Ctrl Pts',(20.7420732493018,53.5497394380497,-26.5743755286402));
#19803=CARTESIAN_POINT('Ctrl Pts',(17.4332845947801,52.5619004681089,-26.4164270054477));
#19804=CARTESIAN_POINT('Ctrl Pts',(16.4516597580046,49.2512486007173,-26.2584784822552));
#19805=CARTESIAN_POINT('Ctrl Pts',(18.6872050642303,46.6194980305971,-26.1005299590628));
#19806=CARTESIAN_POINT('Ctrl Pts',(22.0628243622956,47.0463358989535,-25.9448959825852));
#19807=CARTESIAN_POINT('Ctrl Pts',(23.0748184763337,49.0328957310464,-25.8419115138385));
#19808=CARTESIAN_POINT('Ctrl Pts',(23.0782114598495,50.0008183538095,-25.7915765528225));
#19809=CARTESIAN_POINT('Origin',(20.,50.,-42.2084234471774));
#19810=CARTESIAN_POINT('',(23.0717752285503,49.997407390237,-27.7915765528225));
#19811=CARTESIAN_POINT('',(23.0760710189578,50.0022679983574,-27.7084234471775));
#19812=CARTESIAN_POINT('',(23.0735,50.0000000000002,-42.2084234471774));
#19813=CARTESIAN_POINT('Ctrl Pts',(23.0760710189578,50.0022679983574,-27.7084234471775));
#19814=CARTESIAN_POINT('Ctrl Pts',(23.0773101161764,50.1518848359786,-27.7006572628756));
#19815=CARTESIAN_POINT('Ctrl Pts',(22.9996487300235,51.314512194804,-27.640241570843));
#19816=CARTESIAN_POINT('Ctrl Pts',(21.518320457159,53.29333283432,-27.5271763710795));
#19817=CARTESIAN_POINT('Ctrl Pts',(18.0723368427983,53.0717178336273,-27.369227847887));
#19818=CARTESIAN_POINT('Ctrl Pts',(16.3741061672535,50.0650704804189,-27.2112793246946));
#19819=CARTESIAN_POINT('Ctrl Pts',(17.9633643847556,46.9994241385813,-27.0533308015021));
#19820=CARTESIAN_POINT('Ctrl Pts',(21.3991757215647,46.654311783583,-26.8953822783096));
#19821=CARTESIAN_POINT('Ctrl Pts',(22.9766775148259,48.6111089836517,-26.7804131602014));
#19822=CARTESIAN_POINT('Ctrl Pts',(23.0766953871467,49.8109819664833,-26.718093549824));
#19823=CARTESIAN_POINT('Ctrl Pts',(23.0750331521824,49.9974416679533,-26.7084234471775));
#19824=CARTESIAN_POINT('Ctrl Pts',(23.0717752285503,49.997407390237,-27.7915765528225));
#19825=CARTESIAN_POINT('Ctrl Pts',(23.0659158967544,50.7163996078025,-27.7543894322109));
#19826=CARTESIAN_POINT('Ctrl Pts',(22.4567167775476,52.4622875427393,-27.6645528038683));
#19827=CARTESIAN_POINT('Ctrl Pts',(19.5565636198783,53.5992641004309,-27.522066667795));
#19828=CARTESIAN_POINT('Ctrl Pts',(16.743740353733,51.5962805246318,-27.3641181446025));
#19829=CARTESIAN_POINT('Ctrl Pts',(16.8832686906281,48.1459976943029,-27.2061696214101));
#19830=CARTESIAN_POINT('Ctrl Pts',(19.8486424819224,46.3766828683592,-27.0482210982176));
#19831=CARTESIAN_POINT('Ctrl Pts',(22.5632791857677,47.7029692840987,-26.9100234086884));
#19832=CARTESIAN_POINT('Ctrl Pts',(23.0662806457067,49.3647815266923,-26.8244752268901));
#19833=CARTESIAN_POINT('Ctrl Pts',(23.0698520292984,50.0018654680674,-26.7915765528225));
#19834=CARTESIAN_POINT('Origin',(20.,50.,-42.2084234471774));
#19835=CARTESIAN_POINT('',(23.0782818809563,50.0006847935759,-28.7915765528225));
#19836=CARTESIAN_POINT('',(23.068659485942,50.0003484094753,-28.7084234471774));
#19837=CARTESIAN_POINT('',(23.0735,50.0000000000002,-42.2084234471774));
#19838=CARTESIAN_POINT('Ctrl Pts',(23.068659485942,50.0003484094753,-28.7084234471774));
#19839=CARTESIAN_POINT('Ctrl Pts',(23.0691587716964,50.4888704233529,-28.6832209759272));
#19840=CARTESIAN_POINT('Ctrl Pts',(22.7295043166397,51.9972890662579,-28.6053689969462));
#19841=CARTESIAN_POINT('Ctrl Pts',(20.3740253084567,53.6071377555246,-28.4748675102343));
#19842=CARTESIAN_POINT('Ctrl Pts',(17.1840252420261,52.2850872713679,-28.3169189870418));
#19843=CARTESIAN_POINT('Ctrl Pts',(16.5471838347117,48.8912176686634,-28.1589704638494));
#19844=CARTESIAN_POINT('Ctrl Pts',(19.0409058515914,46.5026472585805,-28.0010219406569));
#19845=CARTESIAN_POINT('Ctrl Pts',(22.238838770898,47.246551697553,-27.8508396017662));
#19846=CARTESIAN_POINT('Ctrl Pts',(23.0689098701799,49.1375832764411,-27.7533067706064));
#19847=CARTESIAN_POINT('Ctrl Pts',(23.0760710189578,50.0022679983574,-27.7084234471775));
#19848=CARTESIAN_POINT('Ctrl Pts',(23.0782818809564,50.0006847935759,-28.7915765528225));
#19849=CARTESIAN_POINT('Ctrl Pts',(23.0783975226873,50.0386403455705,-28.7896026529933));
#19850=CARTESIAN_POINT('Ctrl Pts',(23.060633926734,51.0888674093361,-28.7349792454332));
#19851=CARTESIAN_POINT('Ctrl Pts',(21.868138487219,53.1082787419663,-28.6277063301423));
#19852=CARTESIAN_POINT('Ctrl Pts',(18.4185251564057,53.2634759779658,-28.4697578069498));
#19853=CARTESIAN_POINT('Ctrl Pts',(16.4027869677635,50.4597788009081,-28.3118092837573));
#19854=CARTESIAN_POINT('Ctrl Pts',(17.6485324314252,47.2392141645673,-28.1538607605649));
#19855=CARTESIAN_POINT('Ctrl Pts',(21.026282022335,46.5217700877505,-27.9959122373724));
#19856=CARTESIAN_POINT('Ctrl Pts',(22.8973565003072,48.3843657956996,-27.8751508347916));
#19857=CARTESIAN_POINT('Ctrl Pts',(23.0742115359331,49.6984507670629,-27.8070389399417));
#19858=CARTESIAN_POINT('Ctrl Pts',(23.0717752285503,49.997407390237,-27.7915765528225));
#19859=CARTESIAN_POINT('Origin',(20.,50.,-42.2084234471774));
#19860=CARTESIAN_POINT('',(23.0699776589026,50.0019420177659,-29.7915765528226));
#19861=CARTESIAN_POINT('',(23.07484016668,49.9974042568772,-29.7084234471775));
#19862=CARTESIAN_POINT('',(23.0735,50.0000000000002,-42.2084234471774));
#19863=CARTESIAN_POINT('Ctrl Pts',(23.07484016668,49.9974042568772,-29.7084234471775));
#19864=CARTESIAN_POINT('Ctrl Pts',(23.0674594310508,50.819700244974,-29.6657846889788));
#19865=CARTESIAN_POINT('Ctrl Pts',(22.3060143175262,52.6694190871755,-29.5704964230494));
#19866=CARTESIAN_POINT('Ctrl Pts',(19.1896896859145,53.5347892302254,-29.4225586493891));
#19867=CARTESIAN_POINT('Ctrl Pts',(16.5971712887038,51.2538319138251,-29.2646101261966));
#19868=CARTESIAN_POINT('Ctrl Pts',(17.0898941915086,47.8360633349363,-29.1066616030042));
#19869=CARTESIAN_POINT('Ctrl Pts',(20.2211215243232,46.3802703166986,-28.9487130798117));
#19870=CARTESIAN_POINT('Ctrl Pts',(22.684231513376,47.9150003041815,-28.8159670278695));
#19871=CARTESIAN_POINT('Ctrl Pts',(23.0681157331418,49.4683179826435,-28.735870483658));
#19872=CARTESIAN_POINT('Ctrl Pts',(23.068659485942,50.0003484094753,-28.7084234471774));
#19873=CARTESIAN_POINT('Ctrl Pts',(23.0699776589026,50.0019420177659,-29.7915765528226));
#19874=CARTESIAN_POINT('Ctrl Pts',(23.0721772932313,50.3777822291758,-29.7721663660449));
#19875=CARTESIAN_POINT('Ctrl Pts',(22.8347475984832,51.7703948052325,-29.7001066715364));
#19876=CARTESIAN_POINT('Ctrl Pts',(20.7648506936511,53.5449036037592,-29.5753974692971));
#19877=CARTESIAN_POINT('Ctrl Pts',(17.4497877231476,52.5783241624032,-29.4174489461046));
#19878=CARTESIAN_POINT('Ctrl Pts',(16.4469246628638,49.2740566192138,-29.2595004229122));
#19879=CARTESIAN_POINT('Ctrl Pts',(18.665526948864,46.6279798607482,-29.1015518997197));
#19880=CARTESIAN_POINT('Ctrl Pts',(22.0512086726104,47.0340720045647,-28.9455772763565));
#19881=CARTESIAN_POINT('Ctrl Pts',(23.0753130296877,49.0262581068463,-28.8422521607241));
#19882=CARTESIAN_POINT('Ctrl Pts',(23.0782818809564,50.0006847935759,-28.7915765528225));
#19883=CARTESIAN_POINT('Origin',(20.,50.,-42.2084234471774));
#19884=CARTESIAN_POINT('',(23.071599139613,49.9974440494104,-30.7915765528225));
#19885=CARTESIAN_POINT('',(23.0762467922506,50.0022022521905,-30.7084234471775));
#19886=CARTESIAN_POINT('',(23.0735,50.0000000000002,-42.2084234471774));
#19887=CARTESIAN_POINT('Ctrl Pts',(23.0762467922506,50.0022022521905,-30.7084234471775));
#19888=CARTESIAN_POINT('Ctrl Pts',(23.0774076331198,50.1452351507021,-30.7009979097613));
#19889=CARTESIAN_POINT('Ctrl Pts',(23.003602741494,51.3012147603989,-30.6409228646142));
#19890=CARTESIAN_POINT('Ctrl Pts',(21.5394357280369,53.2835156991,-30.5281983117364));
#19891=CARTESIAN_POINT('Ctrl Pts',(18.0920999054453,53.0840322527814,-30.370249788544));
#19892=CARTESIAN_POINT('Ctrl Pts',(16.3745990724293,50.0883505594653,-30.2123012653514));
#19893=CARTESIAN_POINT('Ctrl Pts',(17.9441389988542,47.012564100946,-30.054352742159));
#19894=CARTESIAN_POINT('Ctrl Pts',(21.3776655688371,46.6453949133369,-29.8964042189665));
#19895=CARTESIAN_POINT('Ctrl Pts',(22.9724076658296,48.597794174159,-29.7810944539727));
#19896=CARTESIAN_POINT('Ctrl Pts',(23.0765730195789,49.8043451827873,-29.7184341967097));
#19897=CARTESIAN_POINT('Ctrl Pts',(23.07484016668,49.9974042568772,-29.7084234471775));
#19898=CARTESIAN_POINT('Ctrl Pts',(23.071599139613,49.9974440494104,-30.7915765528225));
#19899=CARTESIAN_POINT('Ctrl Pts',(23.0659001976564,50.7099535886278,-30.7547300790965));
#19900=CARTESIAN_POINT('Ctrl Pts',(22.4655605708053,52.449224872192,-30.6652340976396));
#19901=CARTESIAN_POINT('Ctrl Pts',(19.5796836281861,53.602037241767,-30.5230886084519));
#19902=CARTESIAN_POINT('Ctrl Pts',(16.7540571997694,51.6171559854022,-30.3651400852594));
#19903=CARTESIAN_POINT('Ctrl Pts',(16.8714283874341,48.1660485806496,-30.207191562067));
#19904=CARTESIAN_POINT('Ctrl Pts',(19.825380305008,46.3777291507101,-30.0492430388745));
#19905=CARTESIAN_POINT('Ctrl Pts',(22.5551893154724,47.6897844401465,-29.9107047024597));
#19906=CARTESIAN_POINT('Ctrl Pts',(23.0662108558178,49.3583277363963,-29.8248158737757));
#19907=CARTESIAN_POINT('Ctrl Pts',(23.0699776589026,50.0019420177659,-29.7915765528226));
#19908=CARTESIAN_POINT('Origin',(20.,50.,-42.2084234471774));
#19909=CARTESIAN_POINT('',(23.0783411161508,50.0005689006785,-31.7915765528225));
#19910=CARTESIAN_POINT('',(23.0686853624729,50.0004533262271,-31.7084234471775));
#19911=CARTESIAN_POINT('',(23.0735,50.0000000000002,-42.2084234471774));
#19912=CARTESIAN_POINT('Ctrl Pts',(23.0686853624729,50.0004533262271,-31.7084234471775));
#19913=CARTESIAN_POINT('Ctrl Pts',(23.0693265266791,50.4823621207053,-31.6835616228129));
#19914=CARTESIAN_POINT('Ctrl Pts',(22.7361512606728,51.9839633167782,-31.6060502907174));
#19915=CARTESIAN_POINT('Ctrl Pts',(20.397179025119,53.6046617773376,-31.4758894508912));
#19916=CARTESIAN_POINT('Ctrl Pts',(17.1987558318052,52.3031215376416,-31.3179409276987));
#19917=CARTESIAN_POINT('Ctrl Pts',(16.5401355298036,48.913411046041,-31.1599924045062));
#19918=CARTESIAN_POINT('Ctrl Pts',(19.0184691159077,46.508877711886,-31.0020438813138));
#19919=CARTESIAN_POINT('Ctrl Pts',(22.2283770573404,47.2338735834618,-30.8515208955375));
#19920=CARTESIAN_POINT('Ctrl Pts',(23.0691768887455,49.1310847567491,-30.7536474174921));
#19921=CARTESIAN_POINT('Ctrl Pts',(23.0762467922506,50.0022022521905,-30.7084234471775));
#19922=CARTESIAN_POINT('Ctrl Pts',(23.0783411161508,50.0005689006785,-31.7915765528225));
#19923=CARTESIAN_POINT('Ctrl Pts',(23.0784217978569,50.0319726308292,-31.7899432998789));
#19924=CARTESIAN_POINT('Ctrl Pts',(23.0638169133829,51.0756294932629,-31.7356605392045));
#19925=CARTESIAN_POINT('Ctrl Pts',(21.8880582287126,53.0962193508344,-31.6287282707992));
#19926=CARTESIAN_POINT('Ctrl Pts',(18.4395125322199,53.2735633499893,-31.4707797476067));
#19927=CARTESIAN_POINT('Ctrl Pts',(16.4058133626825,50.4828670206375,-31.3128312244142));
#19928=CARTESIAN_POINT('Ctrl Pts',(17.6308539049556,47.2543698494103,-31.1548827012218));
#19929=CARTESIAN_POINT('Ctrl Pts',(21.0039271572841,46.5152520311566,-30.9969341780293));
#19930=CARTESIAN_POINT('Ctrl Pts',(22.8922343895822,48.371015245975,-30.8758321285629));
#19931=CARTESIAN_POINT('Ctrl Pts',(23.0740433510782,49.6918568021561,-30.8073795868273));
#19932=CARTESIAN_POINT('Ctrl Pts',(23.071599139613,49.9974440494104,-30.7915765528225));
#19933=CARTESIAN_POINT('Origin',(20.,50.,-42.2084234471774));
#19934=CARTESIAN_POINT('',(23.0701085584971,50.0020159667116,-32.7915765528225));
#19935=CARTESIAN_POINT('',(23.0746459871597,49.9973711112026,-32.7084234471775));
#19936=CARTESIAN_POINT('',(23.0735,50.0000000000002,-42.2084234471774));
#19937=CARTESIAN_POINT('Ctrl Pts',(23.0746459871597,49.9973711112026,-32.7084234471775));
#19938=CARTESIAN_POINT('Ctrl Pts',(23.0672842995498,50.8132306194428,-32.6661253358645));
#19939=CARTESIAN_POINT('Ctrl Pts',(22.3159442955655,52.6565958105203,-32.5711777168206));
#19940=CARTESIAN_POINT('Ctrl Pts',(19.2124032663222,53.5399193623716,-32.423580590046));
#19941=CARTESIAN_POINT('Ctrl Pts',(16.6052922900793,51.2756556240609,-32.2656320668535));
#19942=CARTESIAN_POINT('Ctrl Pts',(17.0760595490536,47.8547937287262,-32.1076835436611));
#19943=CARTESIAN_POINT('Ctrl Pts',(20.197874687272,46.378925116056,-31.9497350204686));
#19944=CARTESIAN_POINT('Ctrl Pts',(22.6771342777603,47.9017055273113,-31.8166483216407));
#19945=CARTESIAN_POINT('Ctrl Pts',(23.0679687429807,49.4618311882865,-31.7362111305437));
#19946=CARTESIAN_POINT('Ctrl Pts',(23.0686853624729,50.0004533262271,-31.7084234471775));
#19947=CARTESIAN_POINT('Ctrl Pts',(23.0701085584971,50.0020159667116,-32.7915765528225));
#19948=CARTESIAN_POINT('Ctrl Pts',(23.0723580174886,50.3712206283648,-32.7725070129305));
#19949=CARTESIAN_POINT('Ctrl Pts',(22.840434117996,51.7570397268036,-32.7007879653077));
#19950=CARTESIAN_POINT('Ctrl Pts',(20.7875967467482,53.5399194211172,-32.5764194099539));
#19951=CARTESIAN_POINT('Ctrl Pts',(17.4663957106355,52.5946459196594,-32.4184708867616));
#19952=CARTESIAN_POINT('Ctrl Pts',(16.4423366275984,49.2968858754349,-32.260522363569));
#19953=CARTESIAN_POINT('Ctrl Pts',(18.6439027228774,46.6366180237041,-32.1025738403766));
#19954=CARTESIAN_POINT('Ctrl Pts',(22.0395220029246,47.0218017427905,-31.9462585701277));
#19955=CARTESIAN_POINT('Ctrl Pts',(23.0758209440669,49.0196426425154,-31.8425928076097));
#19956=CARTESIAN_POINT('Ctrl Pts',(23.0783411161508,50.0005689006785,-31.7915765528225));
#19957=CARTESIAN_POINT('Origin',(20.,50.,-42.2084234471774));
#19958=CARTESIAN_POINT('',(23.0714263576006,49.9974846737907,-33.7915765528225));
#19959=CARTESIAN_POINT('',(23.0764186910915,50.0021324681425,-33.7084234471775));
#19960=CARTESIAN_POINT('',(23.0735,50.0000000000002,-42.2084234471774));
#19961=CARTESIAN_POINT('Ctrl Pts',(23.0764186910915,50.0021324681425,-33.7084234471775));
#19962=CARTESIAN_POINT('Ctrl Pts',(23.0775012055128,50.1385838083694,-33.7013385566469));
#19963=CARTESIAN_POINT('Ctrl Pts',(23.0075098506611,51.2879204901039,-33.6416041583855));
#19964=CARTESIAN_POINT('Ctrl Pts',(21.5604874418836,53.2735632956638,-33.5292202523933));
#19965=CARTESIAN_POINT('Ctrl Pts',(18.1119418026202,53.0962192994522,-33.3712717292008));
#19966=CARTESIAN_POINT('Ctrl Pts',(16.3752411082267,50.1116274316806,-33.2133232060084));
#19967=CARTESIAN_POINT('Ctrl Pts',(17.9249990589457,47.0258263665991,-33.0553746828159));
#19968=CARTESIAN_POINT('Ctrl Pts',(21.3560972546178,46.63661807952,-32.8974261596234));
#19969=CARTESIAN_POINT('Ctrl Pts',(22.9680909366565,48.584474643407,-32.7817757477439));
#19970=CARTESIAN_POINT('Ctrl Pts',(23.0764475746156,49.7977100641984,-32.7187748435953));
#19971=CARTESIAN_POINT('Ctrl Pts',(23.0746459871597,49.9973711112026,-32.7084234471775));
#19972=CARTESIAN_POINT('Ctrl Pts',(23.0714263576006,49.9974846737907,-33.7915765528225));
#19973=CARTESIAN_POINT('Ctrl Pts',(23.0658928724823,50.7035076271574,-33.7550707259821));
#19974=CARTESIAN_POINT('Ctrl Pts',(22.4743381873349,52.4361500475419,-33.6659153914109));
#19975=CARTESIAN_POINT('Ctrl Pts',(19.6028209682899,53.6046618371577,-33.5241105491088));
#19976=CARTESIAN_POINT('Ctrl Pts',(16.7645078702952,51.6379648415364,-33.3661620259164));
#19977=CARTESIAN_POINT('Ctrl Pts',(16.8597170832589,48.1861749405428,-33.2082135027238));
#19978=CARTESIAN_POINT('Ctrl Pts',(19.8021253094441,46.3789250559636,-33.0502649795314));
#19979=CARTESIAN_POINT('Ctrl Pts',(22.5470355553875,47.6766081977323,-32.9113859962309));
#19980=CARTESIAN_POINT('Ctrl Pts',(23.0661474372001,49.3518754423758,-32.8251565206613));
#19981=CARTESIAN_POINT('Ctrl Pts',(23.0701085584971,50.0020159667116,-32.7915765528225));
#19982=CARTESIAN_POINT('Origin',(20.,50.,-42.2084234471774));
#19983=CARTESIAN_POINT('',(23.0783900204597,50.0004517332443,-34.7915765528225));
#19984=CARTESIAN_POINT('',(23.06871800645,50.0005575827461,-34.7084234471775));
#19985=CARTESIAN_POINT('',(23.0735,50.0000000000002,-42.2084234471774));
#19986=CARTESIAN_POINT('Ctrl Pts',(23.06871800645,50.0005575827462,-34.7084234471775));
#19987=CARTESIAN_POINT('Ctrl Pts',(23.0694962958913,50.4758508150922,-34.6839022696985));
#19988=CARTESIAN_POINT('Ctrl Pts',(22.7427398646814,51.9706343794756,-34.6067315844887));
#19989=CARTESIAN_POINT('Ctrl Pts',(20.4203163648388,53.6020371819906,-34.4769113915481));
#19990=CARTESIAN_POINT('Ctrl Pts',(17.2136019186591,52.3210608435138,-34.3189628683557));
#19991=CARTESIAN_POINT('Ctrl Pts',(16.5332298683643,48.9356492300977,-34.1610143451631));
#19992=CARTESIAN_POINT('Ctrl Pts',(18.9960728593762,46.5152520889867,-34.0030658219707));
#19993=CARTESIAN_POINT('Ctrl Pts',(22.2178445185897,47.2212162532767,-33.8522021893088));
#19994=CARTESIAN_POINT('Ctrl Pts',(23.0694567832106,49.1245814238351,-33.7539880643777));
#19995=CARTESIAN_POINT('Ctrl Pts',(23.0764186910915,50.0021324681425,-33.7084234471775));
#19996=CARTESIAN_POINT('Ctrl Pts',(23.0783900204597,50.0004517332443,-34.7915765528225));
#19997=CARTESIAN_POINT('Ctrl Pts',(23.0784415067144,50.0253045395665,-34.7902839467645));
#19998=CARTESIAN_POINT('Ctrl Pts',(23.0669562420345,51.062395329507,-34.7363418329757));
#19999=CARTESIAN_POINT('Ctrl Pts',(21.9079001262167,53.0840323039615,-34.6297502114561));
#20000=CARTESIAN_POINT('Ctrl Pts',(18.4605642464159,53.2835157535905,-34.4718016882636));
#20001=CARTESIAN_POINT('Ctrl Pts',(16.4089879445684,50.5059353330574,-34.3138531650712));
#20002=CARTESIAN_POINT('Ctrl Pts',(17.6132730576857,47.2696387333682,-34.1559046418787));
#20003=CARTESIAN_POINT('Ctrl Pts',(20.9815309003809,46.5088776539501,-33.9979561186862));
#20004=CARTESIAN_POINT('Ctrl Pts',(22.8870600694274,48.3576636413843,-33.8765134223341));
#20005=CARTESIAN_POINT('Ctrl Pts',(23.0738733866284,49.6852657693877,-33.8077202337129));
#20006=CARTESIAN_POINT('Ctrl Pts',(23.0714263576006,49.9974846737907,-33.7915765528225));
#20007=CARTESIAN_POINT('Origin',(20.,50.,-42.2084234471774));
#20008=CARTESIAN_POINT('',(23.0702445934797,50.0020868945689,-35.7915765528225));
#20009=CARTESIAN_POINT('',(23.0744507878878,49.9973424352097,-35.7084234471775));
#20010=CARTESIAN_POINT('',(23.0735,50.0000000000002,-42.2084234471774));
#20011=CARTESIAN_POINT('Ctrl Pts',(23.0744507878878,49.9973424352097,-35.7084234471775));
#20012=CARTESIAN_POINT('Ctrl Pts',(23.0671205125675,50.8067638727642,-35.6664659827501));
#20013=CARTESIAN_POINT('Ctrl Pts',(22.3258049686087,52.643754988248,-35.5718590105919));
#20014=CARTESIAN_POINT('Ctrl Pts',(19.2351493190419,53.5449035449308,-35.4246025307029));
#20015=CARTESIAN_POINT('Ctrl Pts',(16.6135532540943,51.2974267394088,-35.2666540075105));
#20016=CARTESIAN_POINT('Ctrl Pts',(17.0623454595379,47.8736125687236,-35.108705484318));
#20017=CARTESIAN_POINT('Ctrl Pts',(20.1746196920941,46.3777292108223,-34.9507569611255));
#20018=CARTESIAN_POINT('Ctrl Pts',(22.6699767186751,47.8884157689623,-34.817329615412));
#20019=CARTESIAN_POINT('Ctrl Pts',(23.0678252278526,49.4553470186378,-34.7365517774293));
#20020=CARTESIAN_POINT('Ctrl Pts',(23.06871800645,50.0005575827462,-34.7084234471775));
#20021=CARTESIAN_POINT('Ctrl Pts',(23.0702445934797,50.0020868945688,-35.7915765528225));
#20022=CARTESIAN_POINT('Ctrl Pts',(23.0725381809387,50.3646558763446,-35.7728476598162));
#20023=CARTESIAN_POINT('Ctrl Pts',(22.8460662390664,51.7436844134824,-35.7014692590789));
#20024=CARTESIAN_POINT('Ctrl Pts',(20.8103103275328,53.5347892888857,-35.5774413506109));
#20025=CARTESIAN_POINT('Ctrl Pts',(17.4831081577191,52.610860700561,-35.4194928274184));
#20026=CARTESIAN_POINT('Ctrl Pts',(16.4378952735367,49.3197441208273,-35.2615443042259));
#20027=CARTESIAN_POINT('Ctrl Pts',(18.6223344083003,46.6453948576666,-35.1035957810335));
#20028=CARTESIAN_POINT('Ctrl Pts',(22.0277620240878,47.0095592424952,-34.946939863899));
#20029=CARTESIAN_POINT('Ctrl Pts',(23.0763444053201,49.0130177639543,-34.8429334544954));
#20030=CARTESIAN_POINT('Ctrl Pts',(23.0783900204597,50.0004517332443,-34.7915765528225));
#20031=CARTESIAN_POINT('Origin',(20.,50.,-42.2084234471774));
#20032=CARTESIAN_POINT('',(23.0712571035372,49.9975291849918,-36.7915765528226));
#20033=CARTESIAN_POINT('',(23.0765863475585,50.0020587540993,-36.7084234471774));
#20034=CARTESIAN_POINT('',(23.0735,50.0000000000002,-42.2084234471774));
#20035=CARTESIAN_POINT('Ctrl Pts',(23.0765863475585,50.0020587540993,-36.7084234471774));
#20036=CARTESIAN_POINT('Ctrl Pts',(23.077590763035,50.1319308950101,-36.7016792035325));
#20037=CARTESIAN_POINT('Ctrl Pts',(23.011370253205,51.2746294458356,-36.6422854521568));
#20038=CARTESIAN_POINT('Ctrl Pts',(21.5814748173496,53.2634759238072,-36.5302421930502));
#20039=CARTESIAN_POINT('Ctrl Pts',(18.1318615437831,53.1082786903842,-36.3722936698577));
#20040=CARTESIAN_POINT('Ctrl Pts',(16.3760325915391,50.1348997013926,-36.2143451466653));
#20041=CARTESIAN_POINT('Ctrl Pts',(17.9059446705936,47.0392112564499,-36.0563966234728));
#20042=CARTESIAN_POINT('Ctrl Pts',(21.3344730289901,46.6279799167075,-35.8984481002803));
#20043=CARTESIAN_POINT('Ctrl Pts',(22.9637255136602,48.5711524990857,-35.7824570415152));
#20044=CARTESIAN_POINT('Ctrl Pts',(23.0763187659037,49.7910771334522,-35.7191154904809));
#20045=CARTESIAN_POINT('Ctrl Pts',(23.0744507878878,49.9973424352097,-35.7084234471775));
#20046=CARTESIAN_POINT('Ctrl Pts',(23.0712571035372,49.9975291849917,-36.7915765528226));
#20047=CARTESIAN_POINT('Ctrl Pts',(23.0658937343458,50.6970615757762,-36.7554113728678));
#20048=CARTESIAN_POINT('Ctrl Pts',(22.4830498332644,52.4230633627457,-36.6665966851821));
#20049=CARTESIAN_POINT('Ctrl Pts',(19.6259746853353,53.6071378153842,-36.5251324897657));
#20050=CARTESIAN_POINT('Ctrl Pts',(16.7750919383154,51.6587061640742,-36.3671839665732));
#20051=CARTESIAN_POINT('Ctrl Pts',(16.8481352521856,48.2063760842456,-36.2092354433807));
#20052=CARTESIAN_POINT('Ctrl Pts',(19.7788784720074,46.3802702566287,-36.0512869201883));
#20053=CARTESIAN_POINT('Ctrl Pts',(22.538817658055,47.6634412853501,-35.9120672900022));
#20054=CARTESIAN_POINT('Ctrl Pts',(23.0660905894759,49.3454243391448,-35.825497167547));
#20055=CARTESIAN_POINT('Ctrl Pts',(23.0702445934797,50.0020868945688,-35.7915765528225));
#20056=CARTESIAN_POINT('Origin',(20.,50.,-42.2084234471774));
#20057=CARTESIAN_POINT('',(23.0784282759302,50.0003336412877,-37.7915765528226));
#20058=CARTESIAN_POINT('',(23.0687573797509,50.0006610025294,-37.7084234471775));
#20059=CARTESIAN_POINT('',(23.0735,50.0000000000002,-42.2084234471774));
#20060=CARTESIAN_POINT('Ctrl Pts',(23.0687573797509,50.0006610025294,-37.7084234471775));
#20061=CARTESIAN_POINT('Ctrl Pts',(23.0696679145195,50.4693364673409,-37.6842429165841));
#20062=CARTESIAN_POINT('Ctrl Pts',(22.7492703636569,51.9573025041246,-37.60741287826));
#20063=CARTESIAN_POINT('Ctrl Pts',(20.4434363727656,53.5992640406764,-37.477933332205));
#20064=CARTESIAN_POINT('Ctrl Pts',(17.2285628888723,52.338904470578,-37.3199848090125));
#20065=CARTESIAN_POINT('Ctrl Pts',(16.5264671400482,48.9579312880643,-37.1620362858201));
#20066=CARTESIAN_POINT('Ctrl Pts',(18.9737179946959,46.5217701454759,-37.0040877626275));
#20067=CARTESIAN_POINT('Ctrl Pts',(22.2072410095807,47.2085800678294,-36.8528834830801));
#20068=CARTESIAN_POINT('Ctrl Pts',(23.0697497087703,49.1180730561048,-36.7543287112633));
#20069=CARTESIAN_POINT('Ctrl Pts',(23.0765863475585,50.0020587540993,-36.7084234471774));
#20070=CARTESIAN_POINT('Ctrl Pts',(23.0784282759302,50.0003336412877,-37.7915765528226));
#20071=CARTESIAN_POINT('Ctrl Pts',(23.0784567206548,50.0186362554802,-37.7906245936502));
#20072=CARTESIAN_POINT('Ctrl Pts',(23.0700522648677,51.0491651533383,-37.737023126747));
#20073=CARTESIAN_POINT('Ctrl Pts',(21.9276631892634,53.0717178847477,-37.6307721521129));
#20074=CARTESIAN_POINT('Ctrl Pts',(18.4816795176051,53.2933328888968,-37.4728236289205));
#20075=CARTESIAN_POINT('Ctrl Pts',(16.4123105391071,50.5289827307422,-37.314875105728));
#20076=CARTESIAN_POINT('Ctrl Pts',(17.595790636172,47.2850202168804,-37.1569265825356));
#20077=CARTESIAN_POINT('Ctrl Pts',(20.959094164331,46.5026472005525,-36.9989780593431));
#20078=CARTESIAN_POINT('Ctrl Pts',(22.8818333151723,48.3443111113272,-36.8771947161054));
#20079=CARTESIAN_POINT('Ctrl Pts',(23.0737017626221,49.6786777031506,-36.8080608805986));
#20080=CARTESIAN_POINT('Ctrl Pts',(23.0712571035372,49.9975291849917,-36.7915765528226));
#20081=CARTESIAN_POINT('Origin',(20.,50.,-42.2084234471774));
#20082=CARTESIAN_POINT('',(23.0703815974152,50.0021496035415,-38.7915765528225));
#20083=CARTESIAN_POINT('',(23.074254699799,49.9973154728993,-38.7084234471774));
#20084=CARTESIAN_POINT('',(23.0735,50.0000000000002,-42.2084234471774));
#20085=CARTESIAN_POINT('Ctrl Pts',(23.074254699799,49.9973154728993,-38.7084234471775));
#20086=CARTESIAN_POINT('Ctrl Pts',(23.0669677154469,50.8002971404021,-38.6668066296357));
#20087=CARTESIAN_POINT('Ctrl Pts',(22.3355967751289,52.6309008896528,-38.5725403043632));
#20088=CARTESIAN_POINT('Ctrl Pts',(19.257926763209,53.5497393781131,-38.4256244713598));
#20089=CARTESIAN_POINT('Ctrl Pts',(16.6219539119773,51.3191454645357,-38.2676759481674));
#20090=CARTESIAN_POINT('Ctrl Pts',(17.0487524523756,47.8925185252508,-38.1097274249749));
#20091=CARTESIAN_POINT('Ctrl Pts',(20.1513575155428,46.3766829286487,-37.9517789017824));
#20092=CARTESIAN_POINT('Ctrl Pts',(22.6627586022493,47.87513118127,-37.8180109091833));
#20093=CARTESIAN_POINT('Ctrl Pts',(23.0676853605324,49.4488653733505,-37.736892424315));
#20094=CARTESIAN_POINT('Ctrl Pts',(23.0687573797509,50.0006610025294,-37.7084234471775));
#20095=CARTESIAN_POINT('Ctrl Pts',(23.0703815974152,50.0021496035415,-38.7915765528225));
#20096=CARTESIAN_POINT('Ctrl Pts',(23.0727173594958,50.3580876206747,-38.7731883067018));
#20097=CARTESIAN_POINT('Ctrl Pts',(22.8516585980335,51.7303472925322,-38.7021505528502));
#20098=CARTESIAN_POINT('Ctrl Pts',(20.8329797652707,53.529499797304,-38.5784632912678));
#20099=CARTESIAN_POINT('Ctrl Pts',(17.4999297672036,52.6269746785947,-38.4205147680753));
#20100=CARTESIAN_POINT('Ctrl Pts',(16.4335980754498,49.3426269761734,-38.2625662448828));
#20101=CARTESIAN_POINT('Ctrl Pts',(18.6008242547947,46.6543117271026,-38.1046177216904));
#20102=CARTESIAN_POINT('Ctrl Pts',(22.0159279395425,46.9973440896119,-37.9476211576703));
#20103=CARTESIAN_POINT('Ctrl Pts',(23.0768835431613,49.0063831511548,-37.843274101381));
#20104=CARTESIAN_POINT('Ctrl Pts',(23.0784282759302,50.0003336412877,-37.7915765528226));
#20105=CARTESIAN_POINT('Origin',(20.,50.,-42.2084234471774));
#20106=CARTESIAN_POINT('',(23.0703066071761,49.9966560053347,-39.7915765528225));
#20107=CARTESIAN_POINT('',(23.0767446582541,50.0019103494728,-39.7084234471775));
#20108=CARTESIAN_POINT('',(23.0735,50.0000000000002,-42.2084234471774));
#20109=CARTESIAN_POINT('',(20.7937992825328,47.0307770462543,-40.));
#20110=CARTESIAN_POINT('Ctrl Pts',(20.7937992825328,47.0307770462543,-40.));
#20111=CARTESIAN_POINT('Ctrl Pts',(21.7760378723045,47.2933710986319,-39.9473504922692));
#20112=CARTESIAN_POINT('Ctrl Pts',(22.8758107695838,48.3306052064221,-39.8778760098767));
#20113=CARTESIAN_POINT('Ctrl Pts',(23.0726593916611,49.6711328391077,-39.8084015274842));
#20114=CARTESIAN_POINT('Ctrl Pts',(23.0703066071761,49.9966560053347,-39.7915765528225));
#20115=CARTESIAN_POINT('',(19.2043380770546,47.0257135261044,-40.));
#20116=CARTESIAN_POINT('Origin',(20.,50.,-40.));
#20117=CARTESIAN_POINT('Ctrl Pts',(19.2043342004084,47.0257029875827,-40.));
#20118=CARTESIAN_POINT('Ctrl Pts',(20.1513502732183,46.7747743426961,-39.9490537266973));
#20119=CARTESIAN_POINT('Ctrl Pts',(22.2116706660287,47.2298902467823,-39.8518615424231));
#20120=CARTESIAN_POINT('Ctrl Pts',(23.0700633101723,49.111677598951,-39.754669358149));
#20121=CARTESIAN_POINT('Ctrl Pts',(23.0767446582541,50.0019103494728,-39.7084234471775));
#20122=CARTESIAN_POINT('Origin',(-20.,50.,-32.));
#20123=CARTESIAN_POINT('',(-17.486538471654,50.0002728803002,-25.387416697508));
#20124=CARTESIAN_POINT('',(-17.4842348936637,49.9966178726365,-25.112583302492));
#20125=CARTESIAN_POINT('',(-17.4825,50.,-32.));
#20126=CARTESIAN_POINT('',(-18.0865340033349,51.6359872033749,-25.));
#20127=CARTESIAN_POINT('Ctrl Pts',(-17.4842348936637,49.9966178726365,-25.112583302492));
#20128=CARTESIAN_POINT('Ctrl Pts',(-17.4894449388897,50.5891792000144,-25.0750555349946));
#20129=CARTESIAN_POINT('Ctrl Pts',(-17.7007781719159,51.1848035603044,-25.0375277674973));
#20130=CARTESIAN_POINT('Ctrl Pts',(-18.0865340033349,51.6359872033749,-25.));
#20131=CARTESIAN_POINT('',(-17.4825,50.,-25.));
#20132=CARTESIAN_POINT('Origin',(-20.,50.,-25.));
#20133=CARTESIAN_POINT('',(-17.4825,50.,-24.));
#20134=CARTESIAN_POINT('',(-17.4825,50.,-32.));
#20135=CARTESIAN_POINT('Origin',(-20.,50.,-24.));
#20136=CARTESIAN_POINT('',(-21.9170729057076,51.63854067126,-25.));
#20137=CARTESIAN_POINT('Origin',(-20.,50.,-25.));
#20138=CARTESIAN_POINT('Ctrl Pts',(-21.9170804273993,51.6385459961512,-25.));
#20139=CARTESIAN_POINT('Ctrl Pts',(-21.3942486355313,52.2473162151012,-25.0509462733027));
#20140=CARTESIAN_POINT('Ctrl Pts',(-20.5545527314147,52.587362362996,-25.1018925466053));
#20141=CARTESIAN_POINT('Ctrl Pts',(-19.7559044795804,52.5095736846299,-25.152838819908));
#20142=CARTESIAN_POINT('Ctrl Pts',(-18.9305558410379,52.4291843772771,-25.2054883276388));
#20143=CARTESIAN_POINT('Ctrl Pts',(-18.1490453416046,51.902555145838,-25.2581378353696));
#20144=CARTESIAN_POINT('Ctrl Pts',(-17.7651664494765,51.1677990620503,-25.3107873431005));
#20145=CARTESIAN_POINT('Ctrl Pts',(-17.5789260777408,50.8113292248548,-25.3363304612363));
#20146=CARTESIAN_POINT('Ctrl Pts',(-17.4862780001353,50.4058716582546,-25.3618735793722));
#20147=CARTESIAN_POINT('Ctrl Pts',(-17.486538471654,50.0002728803002,-25.387416697508));
#20148=CARTESIAN_POINT('Origin',(-20.,50.,-32.));
#20149=CARTESIAN_POINT('',(-17.4812439066724,49.9979044740549,-26.387416697508));
#20150=CARTESIAN_POINT('',(-17.4786409565,50.0006703257771,-26.112583302492));
#20151=CARTESIAN_POINT('',(-17.4825,50.,-32.));
#20152=CARTESIAN_POINT('Ctrl Pts',(-17.4786409565,50.0006703257771,-26.112583302492));
#20153=CARTESIAN_POINT('Ctrl Pts',(-17.4785131615273,50.0371266681365,-26.1102687557771));
#20154=CARTESIAN_POINT('Ctrl Pts',(-17.4792361426369,50.0735777564612,-26.1079542090622));
#20155=CARTESIAN_POINT('Ctrl Pts',(-17.480825778613,50.1099909286062,-26.1056396623473));
#20156=CARTESIAN_POINT('Ctrl Pts',(-17.516985580908,50.9382894356126,-26.0529901546164));
#20157=CARTESIAN_POINT('Ctrl Pts',(-18.0015839011493,51.7469687422497,-26.0003406468856));
#20158=CARTESIAN_POINT('Ctrl Pts',(-18.7149419927441,52.1695268891006,-25.9476911391548));
#20159=CARTESIAN_POINT('Ctrl Pts',(-19.428300084339,52.5920850359516,-25.895041631424));
#20160=CARTESIAN_POINT('Ctrl Pts',(-20.3704179472873,52.6285220230163,-25.8423921236931));
#20161=CARTESIAN_POINT('Ctrl Pts',(-21.1141877771953,52.2621196062368,-25.7897426159623));
#20162=CARTESIAN_POINT('Ctrl Pts',(-21.8579576071032,51.8957171894573,-25.7370931082315));
#20163=CARTESIAN_POINT('Ctrl Pts',(-22.4033794039707,51.1264753688335,-25.6844436005007));
#20164=CARTESIAN_POINT('Ctrl Pts',(-22.503220283497,50.3035167497657,-25.6317940927699));
#20165=CARTESIAN_POINT('Ctrl Pts',(-22.6030611630233,49.4805581306978,-25.5791445850391));
#20166=CARTESIAN_POINT('Ctrl Pts',(-22.2573211252084,48.603882713186,-25.5264950773082));
#20167=CARTESIAN_POINT('Ctrl Pts',(-21.62268585804,48.0701218881779,-25.4738455695774));
#20168=CARTESIAN_POINT('Ctrl Pts',(-20.9880505908716,47.5363610631698,-25.4211960618466));
#20169=CARTESIAN_POINT('Ctrl Pts',(-20.0645200943497,47.3455148306655,-25.3685465541157));
#20170=CARTESIAN_POINT('Ctrl Pts',(-19.2708510806944,47.5857187630522,-25.3158970463849));
#20171=CARTESIAN_POINT('Ctrl Pts',(-18.4771820670391,47.8259226954389,-25.2632475386541));
#20172=CARTESIAN_POINT('Ctrl Pts',(-17.8133745362502,48.4971767927166,-25.2105980309233));
#20173=CARTESIAN_POINT('Ctrl Pts',(-17.5804136737438,49.2914461181452,-25.1579485231925));
#20174=CARTESIAN_POINT('Ctrl Pts',(-17.5135037670946,49.5195723615276,-25.142826782959));
#20175=CARTESIAN_POINT('Ctrl Pts',(-17.4821355161689,49.7578464491655,-25.1277050427255));
#20176=CARTESIAN_POINT('Ctrl Pts',(-17.4842348936637,49.9966178726365,-25.112583302492));
#20177=CARTESIAN_POINT('Ctrl Pts',(-17.486538471654,50.0002728803002,-25.387416697508));
#20178=CARTESIAN_POINT('Ctrl Pts',(-17.4868148843623,49.5698509390166,-25.414523087103));
#20179=CARTESIAN_POINT('Ctrl Pts',(-17.5917200878965,49.1392699728275,-25.4416294766979));
#20180=CARTESIAN_POINT('Ctrl Pts',(-17.8004369592101,48.7669049830551,-25.4687358662929));
#20181=CARTESIAN_POINT('Ctrl Pts',(-18.2058336458947,48.0436499239839,-25.5213853740237));
#20182=CARTESIAN_POINT('Ctrl Pts',(-19.0028743040869,47.5400227419779,-25.5740348817546));
#20183=CARTESIAN_POINT('Ctrl Pts',(-19.8301086827711,47.4841780405205,-25.6266843894854));
#20184=CARTESIAN_POINT('Ctrl Pts',(-20.6573430614552,47.428333339063,-25.6793338972162));
#20185=CARTESIAN_POINT('Ctrl Pts',(-21.5147711606312,47.8202711181543,-25.731983404947));
#20186=CARTESIAN_POINT('Ctrl Pts',(-22.0137532550528,48.4823912426514,-25.7846329126778));
#20187=CARTESIAN_POINT('Ctrl Pts',(-22.5127353494744,49.1445113671485,-25.8372824204087));
#20188=CARTESIAN_POINT('Ctrl Pts',(-22.6532714391415,50.0768138370515,-25.8899319281395));
#20189=CARTESIAN_POINT('Ctrl Pts',(-22.371620355899,50.8566138838869,-25.9425814358703));
#20190=CARTESIAN_POINT('Ctrl Pts',(-22.0899692726565,51.6364139307222,-25.9952309436011));
#20191=CARTESIAN_POINT('Ctrl Pts',(-21.3861310165042,52.2637115544899,-26.047880451332));
#20192=CARTESIAN_POINT('Ctrl Pts',(-20.5791956609239,52.4541508141935,-26.1005299590628));
#20193=CARTESIAN_POINT('Ctrl Pts',(-19.7722603053436,52.6445900738971,-26.1531794667936));
#20194=CARTESIAN_POINT('Ctrl Pts',(-18.8622278503352,52.3981709695366,-26.2058289745244));
#20195=CARTESIAN_POINT('Ctrl Pts',(-18.2616397845884,51.8265938623424,-26.2584784822552));
#20196=CARTESIAN_POINT('Ctrl Pts',(-17.7713613588437,51.3599979702671,-26.3014578873395));
#20197=CARTESIAN_POINT('Ctrl Pts',(-17.487295335698,50.6767181914727,-26.3444372924237));
#20198=CARTESIAN_POINT('Ctrl Pts',(-17.4812439066724,49.9979044740549,-26.387416697508));
#20199=CARTESIAN_POINT('Origin',(-20.,50.,-32.));
#20200=CARTESIAN_POINT('',(-17.4803937907486,50.0018577149014,-27.387416697508));
#20201=CARTESIAN_POINT('',(-17.4854881593906,50.0015280028117,-27.112583302492));
#20202=CARTESIAN_POINT('',(-17.4825,50.,-32.));
#20203=CARTESIAN_POINT('Ctrl Pts',(-17.4854881593906,50.0015280028117,-27.112583302492));
#20204=CARTESIAN_POINT('Ctrl Pts',(-17.4837319359023,50.314813245317,-27.0928324688287));
#20205=CARTESIAN_POINT('Ctrl Pts',(-17.5380280717696,50.627511664655,-27.0730816351654));
#20206=CARTESIAN_POINT('Ctrl Pts',(-17.651165447386,50.9172321802462,-27.0533308015021));
#20207=CARTESIAN_POINT('Ctrl Pts',(-17.9527540908682,51.6895359110876,-27.0006812937713));
#20208=CARTESIAN_POINT('Ctrl Pts',(-18.6724614246153,52.2985614536939,-26.9480317860404));
#20209=CARTESIAN_POINT('Ctrl Pts',(-19.4840191783241,52.46821795488,-26.8953822783096));
#20210=CARTESIAN_POINT('Ctrl Pts',(-20.2955769320328,52.6378744560661,-26.8427327705788));
#20211=CARTESIAN_POINT('Ctrl Pts',(-21.1989851057032,52.368161915832,-26.790083262848));
#20212=CARTESIAN_POINT('Ctrl Pts',(-21.7846971327504,51.7813471975056,-26.7374337551172));
#20213=CARTESIAN_POINT('Ctrl Pts',(-22.3704091597975,51.1945324791791,-26.6847842473863));
#20214=CARTESIAN_POINT('Ctrl Pts',(-22.6384250402214,50.2906155827604,-26.6321347396555));
#20215=CARTESIAN_POINT('Ctrl Pts',(-22.4672442663634,49.4793798880915,-26.5794852319247));
#20216=CARTESIAN_POINT('Ctrl Pts',(-22.2960634925054,48.6681441934227,-26.5268357241938));
#20217=CARTESIAN_POINT('Ctrl Pts',(-21.6856860643655,47.9495897005038,-26.474186216463));
#20218=CARTESIAN_POINT('Ctrl Pts',(-20.9128164788615,47.6494494205881,-26.4215367087322));
#20219=CARTESIAN_POINT('Ctrl Pts',(-20.1399468933575,47.3493091406725,-26.3688872010014));
#20220=CARTESIAN_POINT('Ctrl Pts',(-19.2045851504892,47.4675830737602,-26.3162376932706));
#20221=CARTESIAN_POINT('Ctrl Pts',(-18.5307649212294,47.950678893992,-26.2635881855397));
#20222=CARTESIAN_POINT('Ctrl Pts',(-17.8865667808605,48.4125371397071,-26.2132532245238));
#20223=CARTESIAN_POINT('Ctrl Pts',(-17.4814201421296,49.2078461586818,-26.1629182635079));
#20224=CARTESIAN_POINT('Ctrl Pts',(-17.4786409565,50.0006703257771,-26.112583302492));
#20225=CARTESIAN_POINT('Ctrl Pts',(-17.4812439066724,49.9979044740549,-26.387416697508));
#20226=CARTESIAN_POINT('Ctrl Pts',(-17.4798823722417,49.8451755492952,-26.3970868001546));
#20227=CARTESIAN_POINT('Ctrl Pts',(-17.4925945596475,49.6926727065716,-26.4067569028011));
#20228=CARTESIAN_POINT('Ctrl Pts',(-17.5201982738737,49.5429147761019,-26.4164270054477));
#20229=CARTESIAN_POINT('Ctrl Pts',(-17.6704885053911,48.7275479070835,-26.4690765131785));
#20230=CARTESIAN_POINT('Ctrl Pts',(-18.2622126449111,47.9935492790746,-26.5217260209094));
#20231=CARTESIAN_POINT('Ctrl Pts',(-19.0271195631323,47.6736634881809,-26.5743755286402));
#20232=CARTESIAN_POINT('Ctrl Pts',(-19.7920264813536,47.3537776972871,-26.627025036371));
#20233=CARTESIAN_POINT('Ctrl Pts',(-20.7301161782762,47.4480047435085,-26.6796745441018));
#20234=CARTESIAN_POINT('Ctrl Pts',(-21.4161209539682,47.9136294939318,-26.7323240518326));
#20235=CARTESIAN_POINT('Ctrl Pts',(-22.1021257296601,48.379254244355,-26.7849735595635));
#20236=CARTESIAN_POINT('Ctrl Pts',(-22.5360455841214,49.21627669898,-26.8376230672943));
#20237=CARTESIAN_POINT('Ctrl Pts',(-22.5211690482687,50.0452448208666,-26.8902725750251));
#20238=CARTESIAN_POINT('Ctrl Pts',(-22.5062925124159,50.8742129427532,-26.9429220827559));
#20239=CARTESIAN_POINT('Ctrl Pts',(-22.0426195862492,51.6951267319013,-26.9955715904868));
#20240=CARTESIAN_POINT('Ctrl Pts',(-21.3403495917614,52.1358377246691,-27.0482210982176));
#20241=CARTESIAN_POINT('Ctrl Pts',(-20.6380795972737,52.5765487174368,-27.1008706059484));
#20242=CARTESIAN_POINT('Ctrl Pts',(-19.6972125344649,52.6370569138241,-27.1535201136792));
#20243=CARTESIAN_POINT('Ctrl Pts',(-18.9442760521657,52.2899316828412,-27.2061696214101));
#20244=CARTESIAN_POINT('Ctrl Pts',(-18.1913395698665,51.9428064518583,-27.2588191291409));
#20245=CARTESIAN_POINT('Ctrl Pts',(-17.6263336680768,51.1880477935053,-27.3114686368717));
#20246=CARTESIAN_POINT('Ctrl Pts',(-17.5053952439644,50.3678141485724,-27.3641181446025));
#20247=CARTESIAN_POINT('Ctrl Pts',(-17.4875559491389,50.2468237360945,-27.3718843289044));
#20248=CARTESIAN_POINT('Ctrl Pts',(-17.4793788476514,50.1244086933274,-27.3796505132062));
#20249=CARTESIAN_POINT('Ctrl Pts',(-17.4803937907486,50.0018577149014,-27.387416697508));
#20250=CARTESIAN_POINT('Origin',(-20.,50.,-32.));
#20251=CARTESIAN_POINT('',(-17.4864645688206,50.0002853817988,-28.387416697508));
#20252=CARTESIAN_POINT('',(-17.4839128694198,49.9978763966856,-28.112583302492));
#20253=CARTESIAN_POINT('',(-17.4825,50.,-32.));
#20254=CARTESIAN_POINT('Ctrl Pts',(-17.4839128694198,49.9978763966856,-28.112583302492));
#20255=CARTESIAN_POINT('Ctrl Pts',(-17.4887122405414,50.5868019954094,-28.0753961818803));
#20256=CARTESIAN_POINT('Ctrl Pts',(-17.6952667199242,51.1787611136952,-28.0382090612686));
#20257=CARTESIAN_POINT('Ctrl Pts',(-18.0729549030142,51.6262950181732,-28.0010219406569));
#20258=CARTESIAN_POINT('Ctrl Pts',(-18.607685653563,52.2599133079476,-27.9483724329261));
#20259=CARTESIAN_POINT('Ctrl Pts',(-19.4854519104968,52.6040329467834,-27.8957229251952));
#20260=CARTESIAN_POINT('Ctrl Pts',(-20.3083316909491,52.5026525553353,-27.8430734174644));
#20261=CARTESIAN_POINT('Ctrl Pts',(-21.1312114714014,52.4012721638872,-27.7904239097336));
#20262=CARTESIAN_POINT('Ctrl Pts',(-21.8992047753722,51.8543917421554,-27.7377744020028));
#20263=CARTESIAN_POINT('Ctrl Pts',(-22.2641535138776,51.1099311613503,-27.685124894272));
#20264=CARTESIAN_POINT('Ctrl Pts',(-22.6291022523829,50.3654705805453,-27.6324753865411));
#20265=CARTESIAN_POINT('Ctrl Pts',(-22.5910064254228,49.4234298406672,-27.5798258788103));
#20266=CARTESIAN_POINT('Ctrl Pts',(-22.1671362035201,48.7108688885658,-27.5271763710795));
#20267=CARTESIAN_POINT('Ctrl Pts',(-21.7432659816174,47.9983079364644,-27.4745268633487));
#20268=CARTESIAN_POINT('Ctrl Pts',(-20.9336213647721,47.5152267721397,-27.4218773556178));
#20269=CARTESIAN_POINT('Ctrl Pts',(-20.1052424146065,47.4806226905502,-27.369227847887));
#20270=CARTESIAN_POINT('Ctrl Pts',(-19.2768634644409,47.4460186089606,-27.3165783401562));
#20271=CARTESIAN_POINT('Ctrl Pts',(-18.429750180955,47.8598916101062,-27.2639288324254));
#20272=CARTESIAN_POINT('Ctrl Pts',(-17.9479285158207,48.5346190702172,-27.2112793246946));
#20273=CARTESIAN_POINT('Ctrl Pts',(-17.6468564905899,48.9562305866647,-27.178380650627));
#20274=CARTESIAN_POINT('Ctrl Pts',(-17.488413475107,49.4796933674211,-27.1454819765595));
#20275=CARTESIAN_POINT('Ctrl Pts',(-17.4854881593906,50.0015280028117,-27.112583302492));
#20276=CARTESIAN_POINT('Ctrl Pts',(-17.4803937907486,50.0018577149014,-27.387416697508));
#20277=CARTESIAN_POINT('Ctrl Pts',(-17.4862594794222,49.2935954605613,-27.432300020937));
#20278=CARTESIAN_POINT('Ctrl Pts',(-17.7991452273176,48.5807928698821,-27.477183344366));
#20279=CARTESIAN_POINT('Ctrl Pts',(-18.3282967300838,48.1122107528984,-27.522066667795));
#20280=CARTESIAN_POINT('Ctrl Pts',(-18.9490075867506,47.5625496336702,-27.5747161755258));
#20281=CARTESIAN_POINT('Ctrl Pts',(-19.8673002465193,47.3489360267268,-27.6273656832566));
#20282=CARTESIAN_POINT('Ctrl Pts',(-20.6668807124105,47.5682084326959,-27.6800151909875));
#20283=CARTESIAN_POINT('Ctrl Pts',(-21.4664611783018,47.7874808386649,-27.7326646987183));
#20284=CARTESIAN_POINT('Ctrl Pts',(-22.1473294503157,48.4396392575466,-27.7853142064491));
#20285=CARTESIAN_POINT('Ctrl Pts',(-22.4008242431245,49.2290375771959,-27.8379637141799));
#20286=CARTESIAN_POINT('Ctrl Pts',(-22.6543190359332,50.0184358968453,-27.8906132219108));
#20287=CARTESIAN_POINT('Ctrl Pts',(-22.4804403495369,50.9450741172625,-27.9432627296416));
#20288=CARTESIAN_POINT('Ctrl Pts',(-21.9580134463135,51.5888748975553,-27.9959122373724));
#20289=CARTESIAN_POINT('Ctrl Pts',(-21.4355865430901,52.232675677848,-28.0485617451032));
#20290=CARTESIAN_POINT('Ctrl Pts',(-20.5646114230397,52.5936390180164,-28.1012112528341));
#20291=CARTESIAN_POINT('Ctrl Pts',(-19.7399314100524,52.5081276743256,-28.1538607605649));
#20292=CARTESIAN_POINT('Ctrl Pts',(-18.915251397065,52.4226163306348,-28.2065102682957));
#20293=CARTESIAN_POINT('Ctrl Pts',(-18.1368664911408,51.8906303030848,-28.2591597760265));
#20294=CARTESIAN_POINT('Ctrl Pts',(-17.7576456536461,51.153337368745,-28.3118092837573));
#20295=CARTESIAN_POINT('Ctrl Pts',(-17.5761187473869,50.8004071177026,-28.3370117550076));
#20296=CARTESIAN_POINT('Ctrl Pts',(-17.4860556044377,50.4004331976185,-28.3622142262578));
#20297=CARTESIAN_POINT('Ctrl Pts',(-17.4864645688206,50.0002853817988,-28.387416697508));
#20298=CARTESIAN_POINT('Origin',(-20.,50.,-32.));
#20299=CARTESIAN_POINT('',(-17.4814019803852,49.9978738298142,-29.387416697508));
#20300=CARTESIAN_POINT('',(-17.4785832788205,50.0005609135351,-29.112583302492));
#20301=CARTESIAN_POINT('',(-17.4825,50.,-32.));
#20302=CARTESIAN_POINT('Ctrl Pts',(-17.4785832788205,50.0005609135351,-29.112583302492));
#20303=CARTESIAN_POINT('Ctrl Pts',(-17.4784885568277,50.0316502572541,-29.1106094026627));
#20304=CARTESIAN_POINT('Ctrl Pts',(-17.4790143481923,50.0627363235243,-29.1086355028334));
#20305=CARTESIAN_POINT('Ctrl Pts',(-17.4801706320494,50.093798920144,-29.1066616030042));
#20306=CARTESIAN_POINT('Ctrl Pts',(-17.5110120025032,50.9223264860409,-29.0540120952733));
#20307=CARTESIAN_POINT('Ctrl Pts',(-17.9904110877069,51.734156798706,-29.0013625875425));
#20308=CARTESIAN_POINT('Ctrl Pts',(-18.7010396025018,52.1612589310346,-28.9487130798117));
#20309=CARTESIAN_POINT('Ctrl Pts',(-19.4116681172968,52.5883610633633,-28.8960635720809));
#20310=CARTESIAN_POINT('Ctrl Pts',(-20.3535260616831,52.6307350153553,-28.84341406435));
#20311=CARTESIAN_POINT('Ctrl Pts',(-21.0996364592575,52.269171200665,-28.7907645566192));
#20312=CARTESIAN_POINT('Ctrl Pts',(-21.8457468568319,51.9076073859748,-28.7381150488884));
#20313=CARTESIAN_POINT('Ctrl Pts',(-22.3961097075944,51.1421058046023,-28.6854655411576));
#20314=CARTESIAN_POINT('Ctrl Pts',(-22.5012263823627,50.3196949567933,-28.6328160334268));
#20315=CARTESIAN_POINT('Ctrl Pts',(-22.606343057131,49.4972841089843,-28.580166525696));
#20316=CARTESIAN_POINT('Ctrl Pts',(-22.2662135559049,48.6179639947387,-28.5275170179651));
#20317=CARTESIAN_POINT('Ctrl Pts',(-21.6350304158872,48.0803610178466,-28.4748675102343));
#20318=CARTESIAN_POINT('Ctrl Pts',(-21.0038472758696,47.5427580409546,-28.4222180025035));
#20319=CARTESIAN_POINT('Ctrl Pts',(-20.0816104970603,47.3468722014163,-28.3695684947726));
#20320=CARTESIAN_POINT('Ctrl Pts',(-19.2864020986368,47.5815053624962,-28.3169189870418));
#20321=CARTESIAN_POINT('Ctrl Pts',(-18.4911937002134,47.8161385235761,-28.264269479311));
#20322=CARTESIAN_POINT('Ctrl Pts',(-17.8230136821757,48.4812906852744,-28.2116199715802));
#20323=CARTESIAN_POINT('Ctrl Pts',(-17.5847712952388,49.27542523648,-28.1589704638494));
#20324=CARTESIAN_POINT('Ctrl Pts',(-17.5148030054337,49.5086508901404,-28.1435080767302));
#20325=CARTESIAN_POINT('Ctrl Pts',(-17.4819172931829,49.7530014119585,-28.1280456896111));
#20326=CARTESIAN_POINT('Ctrl Pts',(-17.4839128694198,49.9978763966856,-28.112583302492));
#20327=CARTESIAN_POINT('Ctrl Pts',(-17.4864645688206,50.0002853817988,-28.387416697508));
#20328=CARTESIAN_POINT('Ctrl Pts',(-17.4869099561092,49.5644998753144,-28.4148637339886));
#20329=CARTESIAN_POINT('Ctrl Pts',(-17.5946601977475,49.1285081190019,-28.4423107704692));
#20330=CARTESIAN_POINT('Ctrl Pts',(-17.8084343854675,48.752851148744,-28.4697578069498));
#20331=CARTESIAN_POINT('Ctrl Pts',(-18.2185007238488,48.0322577042129,-28.5224073146806));
#20332=CARTESIAN_POINT('Ctrl Pts',(-19.0186901696765,47.5336706562804,-28.5750568224115));
#20333=CARTESIAN_POINT('Ctrl Pts',(-19.8462490062726,47.4831168615326,-28.6277063301423));
#20334=CARTESIAN_POINT('Ctrl Pts',(-20.6738078428688,47.4325630667848,-28.6803558378731));
#20335=CARTESIAN_POINT('Ctrl Pts',(-21.5287360702333,47.8300425252218,-28.7330053456039));
#20336=CARTESIAN_POINT('Ctrl Pts',(-22.0234649770947,48.4953639685932,-28.7856548533347));
#20337=CARTESIAN_POINT('Ctrl Pts',(-22.5181938839562,49.1606854119646,-28.8383043610656));
#20338=CARTESIAN_POINT('Ctrl Pts',(-22.6527234703146,50.0938488402703,-28.8909538687964));
#20339=CARTESIAN_POINT('Ctrl Pts',(-22.3660667940254,50.8718188038116,-28.9436033765272));
#20340=CARTESIAN_POINT('Ctrl Pts',(-22.0794101177362,51.6497887673529,-28.996252884258));
#20341=CARTESIAN_POINT('Ctrl Pts',(-21.3715671787995,52.2725652661297,-29.0489023919889));
#20342=CARTESIAN_POINT('Ctrl Pts',(-20.5634278095146,52.4578220448258,-29.1015518997197));
#20343=CARTESIAN_POINT('Ctrl Pts',(-19.7552884402297,52.6430788235219,-29.1542014074505));
#20344=CARTESIAN_POINT('Ctrl Pts',(-18.8468526405967,52.3908158821372,-29.2068509151813));
#20345=CARTESIAN_POINT('Ctrl Pts',(-18.2499459659827,51.8153927890541,-29.2595004229121));
#20346=CARTESIAN_POINT('Ctrl Pts',(-17.766534810533,51.3493803383144,-29.3021391811108));
#20347=CARTESIAN_POINT('Ctrl Pts',(-17.4874475323917,50.6714155213793,-29.3447779393094));
#20348=CARTESIAN_POINT('Ctrl Pts',(-17.4814019803852,49.9978738298142,-29.387416697508));
#20349=CARTESIAN_POINT('Origin',(-20.,50.,-32.));
#20350=CARTESIAN_POINT('',(-17.4802498150093,50.0018038622189,-30.387416697508));
#20351=CARTESIAN_POINT('',(-17.4853852564016,50.0015907042489,-30.112583302492));
#20352=CARTESIAN_POINT('',(-17.4825,50.,-32.));
#20353=CARTESIAN_POINT('Ctrl Pts',(-17.4853852564016,50.0015907042489,-30.112583302492));
#20354=CARTESIAN_POINT('Ctrl Pts',(-17.483583538758,50.3094409370048,-30.0931731157143));
#20355=CARTESIAN_POINT('Ctrl Pts',(-17.5359687349261,50.6166993996009,-30.0737629289367));
#20356=CARTESIAN_POINT('Ctrl Pts',(-17.6453243085392,50.9021311817274,-30.054352742159));
#20357=CARTESIAN_POINT('Ctrl Pts',(-17.9419477869372,51.6763557160829,-30.0017032344282));
#20358=CARTESIAN_POINT('Ctrl Pts',(-18.6577297847812,52.2899908444972,-29.9490537266973));
#20359=CARTESIAN_POINT('Ctrl Pts',(-19.468181418111,52.4648544129348,-29.8964042189665));
#20360=CARTESIAN_POINT('Ctrl Pts',(-20.2786330514408,52.6397179813725,-29.8437547112357));
#20361=CARTESIAN_POINT('Ctrl Pts',(-21.1837543202565,52.3758099898334,-29.7911052035049));
#20362=CARTESIAN_POINT('Ctrl Pts',(-21.7732222613504,51.7927691130892,-29.738455695774));
#20363=CARTESIAN_POINT('Ctrl Pts',(-22.3626902024443,51.2097282363449,-29.6858061880432));
#20364=CARTESIAN_POINT('Ctrl Pts',(-22.6365048158163,50.3075544743955,-29.6331566803124));
#20365=CARTESIAN_POINT('Ctrl Pts',(-22.470536410341,49.4952345830201,-29.5805071725816));
#20366=CARTESIAN_POINT('Ctrl Pts',(-22.3045680048657,48.6829146916447,-29.5278576648507));
#20367=CARTESIAN_POINT('Ctrl Pts',(-21.698816580543,47.9604486708432,-29.4752081571199));
#20368=CARTESIAN_POINT('Ctrl Pts',(-20.927890334043,47.6553555047671,-29.4225586493891));
#20369=CARTESIAN_POINT('Ctrl Pts',(-20.156964087543,47.3502623386911,-29.3699091416583));
#20370=CARTESIAN_POINT('Ctrl Pts',(-19.2208630188656,47.4625420273406,-29.3172596339275));
#20371=CARTESIAN_POINT('Ctrl Pts',(-18.5439543123787,47.9412942812296,-29.2646101261966));
#20372=CARTESIAN_POINT('Ctrl Pts',(-17.8924238105087,48.4020974785568,-29.2139345182951));
#20373=CARTESIAN_POINT('Ctrl Pts',(-17.4810150610682,49.2024092703463,-29.1632589103935));
#20374=CARTESIAN_POINT('Ctrl Pts',(-17.4785832788205,50.0005609135351,-29.112583302492));
#20375=CARTESIAN_POINT('Ctrl Pts',(-17.4814019803852,49.9978738298142,-29.387416697508));
#20376=CARTESIAN_POINT('Ctrl Pts',(-17.4799826025825,49.8397393658052,-29.3974274470402));
#20377=CARTESIAN_POINT('Ctrl Pts',(-17.4936138006039,49.6818487128234,-29.4074381965724));
#20378=CARTESIAN_POINT('Ctrl Pts',(-17.5231848896151,49.5270021041333,-29.4174489461046));
#20379=CARTESIAN_POINT('Ctrl Pts',(-17.6787080374567,48.7126177570775,-29.4700984538354));
#20380=CARTESIAN_POINT('Ctrl Pts',(-18.275131882735,47.9824323077474,-29.5227479615663));
#20381=CARTESIAN_POINT('Ctrl Pts',(-19.0420767449029,47.6674642258089,-29.5753974692971));
#20382=CARTESIAN_POINT('Ctrl Pts',(-19.8090216070708,47.3524961438704,-29.6280469770279));
#20383=CARTESIAN_POINT('Ctrl Pts',(-20.7464874861283,47.4527454293235,-29.6806964847587));
#20384=CARTESIAN_POINT('Ctrl Pts',(-21.4294884816705,47.9227655930774,-29.7333459924895));
#20385=CARTESIAN_POINT('Ctrl Pts',(-22.1124894772127,48.3927857568314,-29.7859955002204));
#20386=CARTESIAN_POINT('Ctrl Pts',(-22.5410255892397,49.2325767988862,-29.8386450079512));
#20387=CARTESIAN_POINT('Ctrl Pts',(-22.5208264880333,50.0614322208726,-29.891294515682));
#20388=CARTESIAN_POINT('Ctrl Pts',(-22.5006273868269,50.8902876428591,-29.9439440234128));
#20389=CARTESIAN_POINT('Ctrl Pts',(-22.0316930723873,51.7082074447772,-29.9965935311437));
#20390=CARTESIAN_POINT('Ctrl Pts',(-21.3266077851688,52.1444001223798,-30.0492430388745));
#20391=CARTESIAN_POINT('Ctrl Pts',(-20.6215224979503,52.5805927999825,-30.1018925466053));
#20392=CARTESIAN_POINT('Ctrl Pts',(-19.680286237953,52.6350583532697,-30.1545420543361));
#20393=CARTESIAN_POINT('Ctrl Pts',(-18.9295941504434,52.2831056519065,-30.207191562067));
#20394=CARTESIAN_POINT('Ctrl Pts',(-18.1789020629339,51.9311529505433,-30.2598410697978));
#20395=CARTESIAN_POINT('Ctrl Pts',(-17.6187541479122,51.1727819945297,-30.3124905775286));
#20396=CARTESIAN_POINT('Ctrl Pts',(-17.5030849445888,50.3517887243693,-30.3651400852594));
#20397=CARTESIAN_POINT('Ctrl Pts',(-17.4867712878388,50.2359981593902,-30.3725656226756));
#20398=CARTESIAN_POINT('Ctrl Pts',(-17.4792989715977,50.1189619437461,-30.3799911600918));
#20399=CARTESIAN_POINT('Ctrl Pts',(-17.4802498150093,50.0018038622189,-30.387416697508));
#20400=CARTESIAN_POINT('Origin',(-20.,50.,-32.));
#20401=CARTESIAN_POINT('',(-17.4864433733835,50.0003713189876,-31.387416697508));
#20402=CARTESIAN_POINT('',(-17.4840571036416,49.9979064241661,-31.112583302492));
#20403=CARTESIAN_POINT('',(-17.4825,50.,-32.));
#20404=CARTESIAN_POINT('Ctrl Pts',(-17.4840571036416,49.9979064241661,-31.112583302492));
#20405=CARTESIAN_POINT('Ctrl Pts',(-17.488725099653,50.5815220694055,-31.0757368287659));
#20406=CARTESIAN_POINT('Ctrl Pts',(-17.6911787677614,51.1680598147817,-31.0388903550398));
#20407=CARTESIAN_POINT('Ctrl Pts',(-18.0625521907884,51.6138879352617,-31.0020438813138));
#20408=CARTESIAN_POINT('Ctrl Pts',(-18.5932034561454,52.2509266720031,-30.949394373583));
#20409=CARTESIAN_POINT('Ctrl Pts',(-19.4687420272821,52.6006753670845,-30.8967448658522));
#20410=CARTESIAN_POINT('Ctrl Pts',(-20.2922558071245,52.5045807681535,-30.8440953581213));
#20411=CARTESIAN_POINT('Ctrl Pts',(-21.115769586967,52.4084861692224,-30.7914458503905));
#20412=CARTESIAN_POINT('Ctrl Pts',(-21.8872585755153,51.866548276279,-30.7387963426597));
#20413=CARTESIAN_POINT('Ctrl Pts',(-22.2569799716995,51.1244463919412,-30.6861468349288));
#20414=CARTESIAN_POINT('Ctrl Pts',(-22.6267013678837,50.3823445076034,-30.633497327198));
#20415=CARTESIAN_POINT('Ctrl Pts',(-22.5946551717038,49.4400786318712,-30.5808478194672));
#20416=CARTESIAN_POINT('Ctrl Pts',(-22.1753690388774,48.7248106706471,-30.5281983117364));
#20417=CARTESIAN_POINT('Ctrl Pts',(-21.7560829060511,48.0095427094229,-30.4755488040056));
#20418=CARTESIAN_POINT('Ctrl Pts',(-20.9495568365783,47.5212726627068,-30.4228992962747));
#20419=CARTESIAN_POINT('Ctrl Pts',(-20.1214171593638,47.4813503311467,-30.3702497885439));
#20420=CARTESIAN_POINT('Ctrl Pts',(-19.2932774821493,47.4414279995867,-30.3176002808131));
#20421=CARTESIAN_POINT('Ctrl Pts',(-18.4435241971931,47.8498533831827,-30.2649507730823));
#20422=CARTESIAN_POINT('Ctrl Pts',(-17.957380034191,48.521473045129,-30.2123012653514));
#20423=CARTESIAN_POINT('Ctrl Pts',(-17.6504616495758,48.9454880542725,-30.1790619443983));
#20424=CARTESIAN_POINT('Ctrl Pts',(-17.4884706399535,49.4744070759156,-30.1458226234451));
#20425=CARTESIAN_POINT('Ctrl Pts',(-17.4853852564016,50.0015907042489,-30.112583302492));
#20426=CARTESIAN_POINT('Ctrl Pts',(-17.4802498150093,50.0018038622189,-30.387416697508));
#20427=CARTESIAN_POINT('Ctrl Pts',(-17.4860407647828,49.2882725305271,-30.4326406678226));
#20428=CARTESIAN_POINT('Ctrl Pts',(-17.804264517897,48.5702209355301,-30.4778646381373));
#20429=CARTESIAN_POINT('Ctrl Pts',(-18.3404526792369,48.1015156596168,-30.5230886084519));
#20430=CARTESIAN_POINT('Ctrl Pts',(-18.9646801088331,47.5558514493319,-30.5757381161827));
#20431=CARTESIAN_POINT('Ctrl Pts',(-19.8843254596506,47.3481386130694,-30.6283876239135));
#20432=CARTESIAN_POINT('Ctrl Pts',(-20.6824814967706,47.5725406064986,-30.6810371316444));
#20433=CARTESIAN_POINT('Ctrl Pts',(-21.4806375338907,47.7969425999279,-30.7336866393752));
#20434=CARTESIAN_POINT('Ctrl Pts',(-22.1573042573133,48.4534594230489,-30.786336147106));
#20435=CARTESIAN_POINT('Ctrl Pts',(-22.4057250979189,49.244469157628,-30.8389856548368));
#20436=CARTESIAN_POINT('Ctrl Pts',(-22.6541459385245,50.0354788922071,-30.8916351625677));
#20437=CARTESIAN_POINT('Ctrl Pts',(-22.4743208963131,50.9609815382444,-30.9442846702985));
#20438=CARTESIAN_POINT('Ctrl Pts',(-21.9477709196056,51.6014145451042,-30.9969341780293));
#20439=CARTESIAN_POINT('Ctrl Pts',(-21.421220942898,52.2418475519639,-31.0495836857601));
#20440=CARTESIAN_POINT('Ctrl Pts',(-20.5479460316942,52.5972109196462,-31.1022331934909));
#20441=CARTESIAN_POINT('Ctrl Pts',(-19.7238320872605,52.5064060693562,-31.1548827012218));
#20442=CARTESIAN_POINT('Ctrl Pts',(-18.8997181428269,52.4156012190662,-31.2075322089526));
#20443=CARTESIAN_POINT('Ctrl Pts',(-18.1247651651633,51.8786281508041,-31.2601817166834));
#20444=CARTESIAN_POINT('Ctrl Pts',(-17.750286302129,51.1389154394177,-31.3128312244142));
#20445=CARTESIAN_POINT('Ctrl Pts',(-17.5734522134114,50.7896128855406,-31.3376930487788));
#20446=CARTESIAN_POINT('Ctrl Pts',(-17.4859181965247,50.3951022544555,-31.3625548731434));
#20447=CARTESIAN_POINT('Ctrl Pts',(-17.4864433733835,50.0003713189876,-31.387416697508));
#20448=CARTESIAN_POINT('Origin',(-20.,50.,-32.));
#20449=CARTESIAN_POINT('',(-17.4815610326054,49.9978466802305,-32.387416697508));
#20450=CARTESIAN_POINT('',(-17.478534759349,50.0004659858125,-32.112583302492));
#20451=CARTESIAN_POINT('',(-17.4825,50.,-32.));
#20452=CARTESIAN_POINT('Ctrl Pts',(-17.478534759349,50.0004659858125,-32.112583302492));
#20453=CARTESIAN_POINT('Ctrl Pts',(-17.4784686730675,50.0261887407035,-32.1109500495484));
#20454=CARTESIAN_POINT('Ctrl Pts',(-17.4788286095695,50.0519096014822,-32.1093167966047));
#20455=CARTESIAN_POINT('Ctrl Pts',(-17.4796202951709,50.0776171661923,-32.1076835436611));
#20456=CARTESIAN_POINT('Ctrl Pts',(-17.5051410556608,50.9063256845015,-32.0550340359303));
#20457=CARTESIAN_POINT('Ctrl Pts',(-17.979317496994,51.7212174820695,-32.0023845281994));
#20458=CARTESIAN_POINT('Ctrl Pts',(-18.6871889402044,52.1528737543759,-31.9497350204686));
#20459=CARTESIAN_POINT('Ctrl Pts',(-19.3950603834147,52.5845300266822,-31.8970855127378));
#20460=CARTESIAN_POINT('Ctrl Pts',(-20.3366268285023,52.6329507737268,-31.844436005007));
#20461=CARTESIAN_POINT('Ctrl Pts',(-21.085043445811,52.2761851861623,-31.7917864972761));
#20462=CARTESIAN_POINT('Ctrl Pts',(-21.8334600631198,51.9194195985978,-31.7391369895453));
#20463=CARTESIAN_POINT('Ctrl Pts',(-22.3887268526497,51.1574676764241,-31.6864874818145));
#20464=CARTESIAN_POINT('Ctrl Pts',(-22.4991220592055,50.3357487366985,-31.6338379740837));
#20465=CARTESIAN_POINT('Ctrl Pts',(-22.6095172657613,49.514029796973,-31.5811884663529));
#20466=CARTESIAN_POINT('Ctrl Pts',(-22.2750408893429,48.6325438396956,-31.528538958622));
#20467=CARTESIAN_POINT('Ctrl Pts',(-21.64732270888,48.0908991190064,-31.4758894508912));
#20468=CARTESIAN_POINT('Ctrl Pts',(-21.0196045284171,47.5492543983172,-31.4232399431604));
#20469=CARTESIAN_POINT('Ctrl Pts',(-20.0986445439097,47.3474509142161,-31.3705904354296));
#20470=CARTESIAN_POINT('Ctrl Pts',(-19.3019459594684,47.5769732074326,-31.3179409276987));
#20471=CARTESIAN_POINT('Ctrl Pts',(-18.5052473750271,47.8064955006491,-31.2652914199679));
#20472=CARTESIAN_POINT('Ctrl Pts',(-17.8328101906518,48.4673435711831,-31.2126419122371));
#20473=CARTESIAN_POINT('Ctrl Pts',(-17.5894735782529,49.2599319956509,-31.1599924045063));
#20474=CARTESIAN_POINT('Ctrl Pts',(-17.5164347802454,49.49783169051,-31.1441893705015));
#20475=CARTESIAN_POINT('Ctrl Pts',(-17.4820550531808,49.7476003038031,-31.1283863364967));
#20476=CARTESIAN_POINT('Ctrl Pts',(-17.4840571036416,49.9979064241661,-31.112583302492));
#20477=CARTESIAN_POINT('Ctrl Pts',(-17.4864433733835,50.0003713189876,-31.387416697508));
#20478=CARTESIAN_POINT('Ctrl Pts',(-17.4870303555796,49.5591865495684,-31.4152043808743));
#20479=CARTESIAN_POINT('Ctrl Pts',(-17.59762258459,49.1177265716563,-31.4429920642405));
#20480=CARTESIAN_POINT('Ctrl Pts',(-17.8164875049079,48.7388048191065,-31.4707797476067));
#20481=CARTESIAN_POINT('Ctrl Pts',(-18.2311723191263,48.0208592646925,-31.5234292553375));
#20482=CARTESIAN_POINT('Ctrl Pts',(-19.0345466959683,47.5274205103753,-31.5760787630684));
#20483=CARTESIAN_POINT('Ctrl Pts',(-19.8624130784562,47.4821815117939,-31.6287282707992));
#20484=CARTESIAN_POINT('Ctrl Pts',(-20.690279460944,47.4369425132125,-31.68137777853));
#20485=CARTESIAN_POINT('Ctrl Pts',(-21.5426378490777,47.839903270367,-31.7340272862608));
#20486=CARTESIAN_POINT('Ctrl Pts',(-22.0330845292512,48.50838765175,-31.7866767939916));
#20487=CARTESIAN_POINT('Ctrl Pts',(-22.5235312094246,49.176872033133,-31.8393263017225));
#20488=CARTESIAN_POINT('Ctrl Pts',(-22.6520661816377,50.1108800387446,-31.8919758094533));
#20489=CARTESIAN_POINT('Ctrl Pts',(-22.360420070845,50.8869933425255,-31.9446253171841));
#20490=CARTESIAN_POINT('Ctrl Pts',(-22.0687739600522,51.6631066463064,-31.9972748249149));
#20491=CARTESIAN_POINT('Ctrl Pts',(-21.3569467662536,52.2813252482565,-32.0499243326458));
#20492=CARTESIAN_POINT('Ctrl Pts',(-20.547634523135,52.4613891463162,-32.1025738403766));
#20493=CARTESIAN_POINT('Ctrl Pts',(-19.7383222800163,52.6414530443759,-32.1552233481074));
#20494=CARTESIAN_POINT('Ctrl Pts',(-18.8315249875777,52.3833622385452,-32.2078728558382));
#20495=CARTESIAN_POINT('Ctrl Pts',(-18.2383254088496,51.8041182709089,-32.2605223635691));
#20496=CARTESIAN_POINT('Ctrl Pts',(-17.7617545368076,51.3387592034373,-32.302820474882));
#20497=CARTESIAN_POINT('Ctrl Pts',(-17.4875909824012,50.6661162585989,-32.345118586195));
#20498=CARTESIAN_POINT('Ctrl Pts',(-17.4815610326054,49.9978466802305,-32.387416697508));
#20499=CARTESIAN_POINT('Origin',(-20.,50.,-32.));
#20500=CARTESIAN_POINT('',(-17.4801090128678,50.0017467021859,-33.387416697508));
#20501=CARTESIAN_POINT('',(-17.4852780367125,50.001651275735,-33.112583302492));
#20502=CARTESIAN_POINT('',(-17.4825,50.,-32.));
#20503=CARTESIAN_POINT('Ctrl Pts',(-17.4852780367125,50.001651275735,-33.112583302492));
#20504=CARTESIAN_POINT('Ctrl Pts',(-17.4834355077518,50.3040663382375,-33.0935137626));
#20505=CARTESIAN_POINT('Ctrl Pts',(-17.5339466800226,50.6058866653819,-33.0744442227079));
#20506=CARTESIAN_POINT('Ctrl Pts',(-17.639580266889,50.8869932156125,-33.0553746828159));
#20507=CARTESIAN_POINT('Ctrl Pts',(-17.9312263359524,51.6631064083454,-33.0027251750851));
#20508=CARTESIAN_POINT('Ctrl Pts',(-18.6430534279012,52.2813249218394,-32.9500756673542));
#20509=CARTESIAN_POINT('Ctrl Pts',(-19.4523655552217,52.4613887941352,-32.8974261596234));
#20510=CARTESIAN_POINT('Ctrl Pts',(-20.2616776825422,52.641452666431,-32.8447766518926));
#20511=CARTESIAN_POINT('Ctrl Pts',(-21.1684748452343,52.3833618975286,-32.7921271441618));
#20512=CARTESIAN_POINT('Ctrl Pts',(-21.7616743390861,51.8041180127718,-32.739477636431));
#20513=CARTESIAN_POINT('Ctrl Pts',(-22.3548738329379,51.224874128015,-32.6868281287001));
#20514=CARTESIAN_POINT('Ctrl Pts',(-22.6344756579494,50.3244771274039,-32.6341786209693));
#20515=CARTESIAN_POINT('Ctrl Pts',(-22.4737265786042,49.5111082989972,-32.5815291132385));
#20516=CARTESIAN_POINT('Ctrl Pts',(-22.312977499259,48.6977394705904,-32.5288796055076));
#20517=CARTESIAN_POINT('Ctrl Pts',(-21.711877515557,47.9713988143879,-32.4762300977768));
#20518=CARTESIAN_POINT('Ctrl Pts',(-20.9429261642948,47.6613618215529,-32.423580590046));
#20519=CARTESIAN_POINT('Ctrl Pts',(-20.1739748130326,47.3513248287178,-32.3709310823152));
#20520=CARTESIAN_POINT('Ctrl Pts',(-19.2371720942102,47.4575914992502,-32.3182815745843));
#20521=CARTESIAN_POINT('Ctrl Pts',(-18.5572032746223,47.9319874540416,-32.2656320668535));
#20522=CARTESIAN_POINT('Ctrl Pts',(-17.8983279300551,48.3916670587091,-32.2146158120663));
#20523=CARTESIAN_POINT('Ctrl Pts',(-17.4805990290548,49.1969905520396,-32.1635995572792));
#20524=CARTESIAN_POINT('Ctrl Pts',(-17.478534759349,50.0004659858125,-32.112583302492));
#20525=CARTESIAN_POINT('Ctrl Pts',(-17.4815610326054,49.9978466802305,-32.387416697508));
#20526=CARTESIAN_POINT('Ctrl Pts',(-17.4800853544066,49.8343045478529,-32.3977680939258));
#20527=CARTESIAN_POINT('Ctrl Pts',(-17.494668257568,49.6710243373683,-32.4081194903437));
#20528=CARTESIAN_POINT('Ctrl Pts',(-17.5262730674496,49.5111082290455,-32.4184708867615));
#20529=CARTESIAN_POINT('Ctrl Pts',(-17.6870221697952,48.6977392842601,-32.4711203944923));
#20530=CARTESIAN_POINT('Ctrl Pts',(-18.2881222395038,47.9713985241312,-32.5237699022232));
#20531=CARTESIAN_POINT('Ctrl Pts',(-19.0570737007893,47.6613614869354,-32.576419409954));
#20532=CARTESIAN_POINT('Ctrl Pts',(-19.8260251620747,47.3513244497396,-32.6290689176848));
#20533=CARTESIAN_POINT('Ctrl Pts',(-20.762828014937,47.4575911354768,-32.6817184254156));
#20534=CARTESIAN_POINT('Ctrl Pts',(-21.4427969318163,47.9319871581458,-32.7343679331465));
#20535=CARTESIAN_POINT('Ctrl Pts',(-22.1227658486956,48.4063831808148,-32.7870174408773));
#20536=CARTESIAN_POINT('Ctrl Pts',(-22.5459008295921,49.2489085404154,-32.8396669486081));
#20537=CARTESIAN_POINT('Ctrl Pts',(-22.5203800654506,50.077617177298,-32.8923164563389));
#20538=CARTESIAN_POINT('Ctrl Pts',(-22.4948593013091,50.9063258141806,-32.9449659640697));
#20539=CARTESIAN_POINT('Ctrl Pts',(-22.0206827921297,51.7212177283451,-32.9976154718006));
#20540=CARTESIAN_POINT('Ctrl Pts',(-21.3128112476355,52.1528740624138,-33.0502649795314));
#20541=CARTESIAN_POINT('Ctrl Pts',(-20.6049397031413,52.5845303964825,-33.1029144872622));
#20542=CARTESIAN_POINT('Ctrl Pts',(-19.6633731233323,52.6329511504552,-33.155563994993));
#20543=CARTESIAN_POINT('Ctrl Pts',(-18.9149563989385,52.2761855118439,-33.2082135027239));
#20544=CARTESIAN_POINT('Ctrl Pts',(-18.1665396745447,51.9194198732325,-33.2608630104547));
#20545=CARTESIAN_POINT('Ctrl Pts',(-17.6112728055659,51.157467842037,-33.3135125181855));
#20546=CARTESIAN_POINT('Ctrl Pts',(-17.5008775832146,50.3357487847381,-33.3661620259163));
#20547=CARTESIAN_POINT('Ctrl Pts',(-17.4860220204721,50.225172450433,-33.3732469164469));
#20548=CARTESIAN_POINT('Ctrl Pts',(-17.479222326559,50.1135138369441,-33.3803318069775));
#20549=CARTESIAN_POINT('Ctrl Pts',(-17.4801090128678,50.0017467021859,-33.387416697508));
#20550=CARTESIAN_POINT('Origin',(-20.,50.,-32.));
#20551=CARTESIAN_POINT('',(-17.4864166347396,50.0004567153817,-34.387416697508));
#20552=CARTESIAN_POINT('',(-17.4841986291653,49.9979396995438,-34.112583302492));
#20553=CARTESIAN_POINT('',(-17.4825,50.,-32.));
#20554=CARTESIAN_POINT('Ctrl Pts',(-17.4841986291653,49.9979396995438,-34.112583302492));
#20555=CARTESIAN_POINT('Ctrl Pts',(-17.4887310996937,50.5762421906731,-34.0760774756515));
#20556=CARTESIAN_POINT('Ctrl Pts',(-17.6871330770759,51.1573544545628,-34.0395716488111));
#20557=CARTESIAN_POINT('Ctrl Pts',(-18.0522293590857,51.6014143159703,-34.0030658219707));
#20558=CARTESIAN_POINT('Ctrl Pts',(-18.5787792604534,52.2418472311955,-33.9504163142398));
#20559=CARTESIAN_POINT('Ctrl Pts',(-19.4520540467071,52.5972105480315,-33.897766806509));
#20560=CARTESIAN_POINT('Ctrl Pts',(-20.2761678732247,52.5064057107341,-33.8451172987782));
#20561=CARTESIAN_POINT('Ctrl Pts',(-21.1002816997423,52.4156008734368,-33.7924677910474));
#20562=CARTESIAN_POINT('Ctrl Pts',(-21.8752345665239,51.878627882006,-33.7398182833166));
#20563=CARTESIAN_POINT('Ctrl Pts',(-22.249713375977,51.1389152764592,-33.6871687755858));
#20564=CARTESIAN_POINT('Ctrl Pts',(-22.6241921854301,50.3992026709125,-33.6345192678549));
#20565=CARTESIAN_POINT('Ctrl Pts',(-22.5981969375548,49.4567504512499,-33.5818697601241));
#20566=CARTESIAN_POINT('Ctrl Pts',(-22.1835121826704,48.7388049995611,-33.5292202523933));
#20567=CARTESIAN_POINT('Ctrl Pts',(-21.768827427786,48.0208595478723,-33.4765707446624));
#20568=CARTESIAN_POINT('Ctrl Pts',(-20.9654531658926,47.5274208641573,-33.4239212369316));
#20569=CARTESIAN_POINT('Ctrl Pts',(-20.1375869018576,47.4821818720488,-33.3712717292008));
#20570=CARTESIAN_POINT('Ctrl Pts',(-19.3097206378227,47.4369428799404,-33.31862222147));
#20571=CARTESIAN_POINT('Ctrl Pts',(-18.4573623716463,47.8399035794383,-33.2659727137392));
#20572=CARTESIAN_POINT('Ctrl Pts',(-17.966915761647,48.5083878651731,-33.2133232060083));
#20573=CARTESIAN_POINT('Ctrl Pts',(-17.6541078722624,48.934748562228,-33.1797432381695));
#20574=CARTESIAN_POINT('Ctrl Pts',(-17.4885225860615,49.4691220101996,-33.1461632703308));
#20575=CARTESIAN_POINT('Ctrl Pts',(-17.4852780367125,50.001651275735,-33.112583302492));
#20576=CARTESIAN_POINT('Ctrl Pts',(-17.4801090128678,50.0017467021859,-33.387416697508));
#20577=CARTESIAN_POINT('Ctrl Pts',(-17.4858115035506,49.2829456580686,-33.4329813147083));
#20578=CARTESIAN_POINT('Ctrl Pts',(-17.8094289999739,48.5596560850262,-33.4785459319085));
#20579=CARTESIAN_POINT('Ctrl Pts',(-18.3526770554175,48.090898845848,-33.5241105491088));
#20580=CARTESIAN_POINT('Ctrl Pts',(-18.9803953256957,47.5492540476591,-33.5767600568396));
#20581=CARTESIAN_POINT('Ctrl Pts',(-19.9013554419761,47.3474505346835,-33.6294095645704));
#20582=CARTESIAN_POINT('Ctrl Pts',(-20.6980541404108,47.5769728607406,-33.6820590723013));
#20583=CARTESIAN_POINT('Ctrl Pts',(-21.4947528388455,47.8064951867976,-33.7347085800321));
#20584=CARTESIAN_POINT('Ctrl Pts',(-22.1671901194345,48.4673433518873,-33.7873580877629));
#20585=CARTESIAN_POINT('Ctrl Pts',(-22.4105267666506,49.2599318897604,-33.8400075954937));
#20586=CARTESIAN_POINT('Ctrl Pts',(-22.6538634138666,50.0525204276335,-33.8926571032246));
#20587=CARTESIAN_POINT('Ctrl Pts',(-22.4680994277097,50.97684933829,-33.9453066109554));
#20588=CARTESIAN_POINT('Ctrl Pts',(-21.9374480864259,51.6138881661804,-33.9979561186862));
#20589=CARTESIAN_POINT('Ctrl Pts',(-21.4067967451421,52.2509269940707,-34.050605626417));
#20590=CARTESIAN_POINT('Ctrl Pts',(-20.5312580487314,52.6006757391949,-34.1032551341478));
#20591=CARTESIAN_POINT('Ctrl Pts',(-19.7077441510588,52.5045811265144,-34.1559046418787));
#20592=CARTESIAN_POINT('Ctrl Pts',(-18.8842302533861,52.4084865138339,-34.2085541496095));
#20593=CARTESIAN_POINT('Ctrl Pts',(-18.1127411544516,51.8665485433488,-34.2612036573403));
#20594=CARTESIAN_POINT('Ctrl Pts',(-17.7430197053668,51.1244465528294,-34.3138531650711));
#20595=CARTESIAN_POINT('Ctrl Pts',(-17.5708242630631,50.7788172126644,-34.3383743425501));
#20596=CARTESIAN_POINT('Ctrl Pts',(-17.4857791387596,50.3897688515684,-34.3628955200291));
#20597=CARTESIAN_POINT('Ctrl Pts',(-17.4864166347396,50.0004567153817,-34.387416697508));
#20598=CARTESIAN_POINT('Origin',(-20.,50.,-32.));
#20599=CARTESIAN_POINT('',(-17.481720920103,49.9978231917579,-35.387416697508));
#20600=CARTESIAN_POINT('',(-17.4784947018927,50.0003700141181,-35.112583302492));
#20601=CARTESIAN_POINT('',(-17.4825,50.,-32.));
#20602=CARTESIAN_POINT('Ctrl Pts',(-17.4784947018927,50.0003700141181,-35.112583302492));
#20603=CARTESIAN_POINT('Ctrl Pts',(-17.4784525295678,50.0207269157445,-35.111290696434));
#20604=CARTESIAN_POINT('Ctrl Pts',(-17.4786779615225,50.0410828596851,-35.109998090376));
#20605=CARTESIAN_POINT('Ctrl Pts',(-17.4791738726521,50.0614322120827,-35.108705484318));
#20606=CARTESIAN_POINT('Ctrl Pts',(-17.4993729709683,50.8902875154747,-35.0560559765872));
#20607=CARTESIAN_POINT('Ctrl Pts',(-17.9683072183117,51.708207200363,-35.0034064688563));
#20608=CARTESIAN_POINT('Ctrl Pts',(-18.6733924046451,52.1443998155543,-34.9507569611255));
#20609=CARTESIAN_POINT('Ctrl Pts',(-19.3784775909784,52.5805924307456,-34.8981074533947));
#20610=CARTESIAN_POINT('Ctrl Pts',(-20.3197137163016,52.6350579762398,-34.8454579456639));
#20611=CARTESIAN_POINT('Ctrl Pts',(-21.0704056964005,52.2831053252348,-34.792808437933));
#20612=CARTESIAN_POINT('Ctrl Pts',(-21.8210976764994,51.9311526742298,-34.7401589302022));
#20613=CARTESIAN_POINT('Ctrl Pts',(-22.381245511374,51.1727818267255,-34.6875094224714));
#20614=CARTESIAN_POINT('Ctrl Pts',(-22.4969146981471,50.3517886740346,-34.6348599147406));
#20615=CARTESIAN_POINT('Ctrl Pts',(-22.6125838849203,49.5307955213437,-34.5822104070097));
#20616=CARTESIAN_POINT('Ctrl Pts',(-22.283774423592,48.6471800634662,-34.5295608992789));
#20617=CARTESIAN_POINT('Ctrl Pts',(-21.6595470833116,48.1015159312561,-34.4769113915481));
#20618=CARTESIAN_POINT('Ctrl Pts',(-21.0353197430311,47.5558517990461,-34.4242618838173));
#20619=CARTESIAN_POINT('Ctrl Pts',(-20.1156745237985,47.3481389925035,-34.3716123760864));
#20620=CARTESIAN_POINT('Ctrl Pts',(-19.3175186008803,47.5725409538248,-34.3189628683556));
#20621=CARTESIAN_POINT('Ctrl Pts',(-18.5193626779622,47.7969429151461,-34.2663133606248));
#20622=CARTESIAN_POINT('Ctrl Pts',(-17.8426960513585,48.4534596443312,-34.213663852894));
#20623=CARTESIAN_POINT('Ctrl Pts',(-17.5942752462975,49.2444692657309,-34.1610143451631));
#20624=CARTESIAN_POINT('Ctrl Pts',(-17.5181030962378,49.4870129752447,-34.1448706642728));
#20625=CARTESIAN_POINT('Ctrl Pts',(-17.4821942708426,49.7422015973575,-34.1287269833824));
#20626=CARTESIAN_POINT('Ctrl Pts',(-17.4841986291653,49.9979396995438,-34.112583302492));
#20627=CARTESIAN_POINT('Ctrl Pts',(-17.4864166347396,50.0004567153817,-34.387416697508));
#20628=CARTESIAN_POINT('Ctrl Pts',(-17.4871479086549,49.5538753737183,-34.4155450277599));
#20629=CARTESIAN_POINT('Ctrl Pts',(-17.6006243673771,49.1069469444978,-34.4436733580117));
#20630=CARTESIAN_POINT('Ctrl Pts',(-17.824630649866,48.7248104881901,-34.4718016882636));
#20631=CARTESIAN_POINT('Ctrl Pts',(-18.2439168426848,48.0095424246239,-34.5244511959944));
#20632=CARTESIAN_POINT('Ctrl Pts',(-19.0504430275571,47.521272308045,-34.5771007037253));
#20633=CARTESIAN_POINT('Ctrl Pts',(-19.8785828232637,47.4813499707728,-34.6297502114561));
#20634=CARTESIAN_POINT('Ctrl Pts',(-20.7067226189702,47.4414276335006,-34.6823997191869));
#20635=CARTESIAN_POINT('Ctrl Pts',(-21.556476025511,47.8498530755351,-34.7350492269177));
#20636=CARTESIAN_POINT('Ctrl Pts',(-22.0426202580716,48.5214728335782,-34.7876987346486));
#20637=CARTESIAN_POINT('Ctrl Pts',(-22.5287644906322,49.1930925916214,-34.8403482423794));
#20638=CARTESIAN_POINT('Ctrl Pts',(-22.6512995492126,50.1279066656732,-34.8929977501102));
#20639=CARTESIAN_POINT('Ctrl Pts',(-22.354676028373,50.9021313108064,-34.945647257841));
#20640=CARTESIAN_POINT('Ctrl Pts',(-22.0580525075334,51.6763559559396,-34.9982967655718));
#20641=CARTESIAN_POINT('Ctrl Pts',(-21.3422704072737,52.2899911721542,-35.0509462733027));
#20642=CARTESIAN_POINT('Ctrl Pts',(-20.5318186579827,52.4648547656116,-35.1035957810335));
#20643=CARTESIAN_POINT('Ctrl Pts',(-19.7213669086916,52.6397183590691,-35.1562452887643));
#20644=CARTESIAN_POINT('Ctrl Pts',(-18.8162455103692,52.3758103297695,-35.2088947964951));
#20645=CARTESIAN_POINT('Ctrl Pts',(-18.226777484933,51.7927693696024,-35.2615443042259));
#20646=CARTESIAN_POINT('Ctrl Pts',(-17.7570184164389,51.3281321602486,-35.3035017686533));
#20647=CARTESIAN_POINT('Ctrl Pts',(-17.4877251401288,50.6608193538835,-35.3454592330807));
#20648=CARTESIAN_POINT('Ctrl Pts',(-17.481720920103,49.9978231917579,-35.387416697508));
#20649=CARTESIAN_POINT('Origin',(-20.,50.,-32.));
#20650=CARTESIAN_POINT('',(-17.4799716856498,50.0016863230979,-36.387416697508));
#20651=CARTESIAN_POINT('',(-17.4851666106336,50.0017093726515,-36.112583302492));
#20652=CARTESIAN_POINT('',(-17.4825,50.,-32.));
#20653=CARTESIAN_POINT('Ctrl Pts',(-17.4851666106336,50.0017093726515,-36.112583302492));
#20654=CARTESIAN_POINT('Ctrl Pts',(-17.483287936102,50.298689158319,-36.0938544094856));
#20655=CARTESIAN_POINT('Ctrl Pts',(-17.5319618132886,50.5950731831941,-36.0751255164792));
#20656=CARTESIAN_POINT('Ctrl Pts',(-17.6339335445166,50.8718186790697,-36.0563966234728));
#20657=CARTESIAN_POINT('Ctrl Pts',(-17.9205901797904,51.6497885312973,-36.003747115742));
#20658=CARTESIAN_POINT('Ctrl Pts',(-18.6284330174474,52.2725649409661,-35.9510976080111));
#20659=CARTESIAN_POINT('Ctrl Pts',(-19.4365722711018,52.4578216931553,-35.8984481002803));
#20660=CARTESIAN_POINT('Ctrl Pts',(-20.2447115247563,52.6430784453445,-35.8457985925495));
#20661=CARTESIAN_POINT('Ctrl Pts',(-21.1531471944084,52.3908155400541,-35.7931490848187));
#20662=CARTESIAN_POINT('Ctrl Pts',(-21.7500537836158,51.8153925293037,-35.7404995770878));
#20663=CARTESIAN_POINT('Ctrl Pts',(-22.3469603728231,51.2399695185533,-35.687850069357));
#20664=CARTESIAN_POINT('Ctrl Pts',(-22.6323378815858,50.3413864023429,-35.6352005616262));
#20665=CARTESIAN_POINT('Ctrl Pts',(-22.4768147559968,49.5270021718109,-35.5825510538954));
#20666=CARTESIAN_POINT('Ctrl Pts',(-22.3212916304078,48.712617941279,-35.5299015461646));
#20667=CARTESIAN_POINT('Ctrl Pts',(-21.7248678704671,47.9824325964254,-35.4772520384337));
#20668=CARTESIAN_POINT('Ctrl Pts',(-20.9579231180354,47.6674645595532,-35.4246025307029));
#20669=CARTESIAN_POINT('Ctrl Pts',(-20.1909783656036,47.3524965226811,-35.3719530229721));
#20670=CARTESIAN_POINT('Ctrl Pts',(-19.2535126206808,47.4527457937902,-35.3193035152412));
#20671=CARTESIAN_POINT('Ctrl Pts',(-18.5705117228638,47.9227658902926,-35.2666540075104));
#20672=CARTESIAN_POINT('Ctrl Pts',(-17.9042792837883,48.3812464520433,-35.2152971058376));
#20673=CARTESIAN_POINT('Ctrl Pts',(-17.480170262617,49.1915641225488,-35.1639402041648));
#20674=CARTESIAN_POINT('Ctrl Pts',(-17.4784947018927,50.0003700141181,-35.112583302492));
#20675=CARTESIAN_POINT('Ctrl Pts',(-17.481720920103,49.9978231917579,-35.387416697508));
#20676=CARTESIAN_POINT('Ctrl Pts',(-17.4801908614735,49.8288715219602,-35.3981087408115));
#20677=CARTESIAN_POINT('Ctrl Pts',(-17.4957584265948,49.6602001690132,-35.408800784115));
#20678=CARTESIAN_POINT('Ctrl Pts',(-17.5294632361692,49.4952345107971,-35.4194928274184));
#20679=CARTESIAN_POINT('Ctrl Pts',(-17.6954316653917,48.6829145031932,-35.4721423351493));
#20680=CARTESIAN_POINT('Ctrl Pts',(-18.3011831763866,47.9604483790198,-35.52479184288));
#20681=CARTESIAN_POINT('Ctrl Pts',(-19.0721095331925,47.6553551692903,-35.5774413506109));
#20682=CARTESIAN_POINT('Ctrl Pts',(-19.8430358899984,47.3502619595608,-35.6300908583417));
#20683=CARTESIAN_POINT('Ctrl Pts',(-20.7791370926151,47.4625416642753,-35.6827403660725));
#20684=CARTESIAN_POINT('Ctrl Pts',(-21.4560458959555,47.9412939866653,-35.7353898738034));
#20685=CARTESIAN_POINT('Ctrl Pts',(-22.1329546992959,48.4200463090554,-35.7880393815342));
#20686=CARTESIAN_POINT('Ctrl Pts',(-22.5506711033599,49.2652712491211,-35.840688889265));
#20687=CARTESIAN_POINT('Ctrl Pts',(-22.5198297284933,50.0937989335653,-35.8933383969958));
#20688=CARTESIAN_POINT('Ctrl Pts',(-22.4889883536267,50.9223266180095,-35.9459879047266));
#20689=CARTESIAN_POINT('Ctrl Pts',(-22.0095891998295,51.7341570468322,-35.9986374124575));
#20690=CARTESIAN_POINT('Ctrl Pts',(-21.2989605833562,52.1612592402719,-36.0512869201883));
#20691=CARTESIAN_POINT('Ctrl Pts',(-20.588331966883,52.5883614337116,-36.1039364279191));
#20692=CARTESIAN_POINT('Ctrl Pts',(-19.6464738877337,52.6307353917684,-36.1565859356499));
#20693=CARTESIAN_POINT('Ctrl Pts',(-18.9003633834041,52.2691715253439,-36.2092354433808));
#20694=CARTESIAN_POINT('Ctrl Pts',(-18.1542528790745,51.9076076589195,-36.2618849511116));
#20695=CARTESIAN_POINT('Ctrl Pts',(-17.6038899495646,51.1421059680139,-36.3145344588424));
#20696=CARTESIAN_POINT('Ctrl Pts',(-17.4987732597562,50.3196950025341,-36.3671839665732));
#20697=CARTESIAN_POINT('Ctrl Pts',(-17.4853081278343,50.2143466305072,-36.3739282102182));
#20698=CARTESIAN_POINT('Ctrl Pts',(-17.4791489700962,50.1080644433152,-36.3806724538631));
#20699=CARTESIAN_POINT('Ctrl Pts',(-17.4799716856498,50.0016863230979,-36.387416697508));
#20700=CARTESIAN_POINT('Origin',(-20.,50.,-32.));
#20701=CARTESIAN_POINT('',(-17.4863843841259,50.0005414264851,-37.387416697508));
#20702=CARTESIAN_POINT('',(-17.4843372649484,49.997976158615,-37.112583302492));
#20703=CARTESIAN_POINT('',(-17.4825,50.,-32.));
#20704=CARTESIAN_POINT('Ctrl Pts',(-17.4843372649484,49.997976158615,-37.112583302492));
#20705=CARTESIAN_POINT('Ctrl Pts',(-17.4887303937409,50.5709622382976,-37.0764181225372));
#20706=CARTESIAN_POINT('Ctrl Pts',(-17.6831295324326,51.1466451272143,-37.0402529425824));
#20707=CARTESIAN_POINT('Ctrl Pts',(-18.0419868338466,51.5888746702098,-37.0040877626276));
#20708=CARTESIAN_POINT('Ctrl Pts',(-18.5644136623227,52.2326753583812,-36.9514382548968));
#20709=CARTESIAN_POINT('Ctrl Pts',(-19.4353886577459,52.5936386469132,-36.8987887471659));
#20710=CARTESIAN_POINT('Ctrl Pts',(-20.2600685527347,52.5081273154602,-36.8461392394351));
#20711=CARTESIAN_POINT('Ctrl Pts',(-21.0847484477236,52.4226159840072,-36.7934897317043));
#20712=CARTESIAN_POINT('Ctrl Pts',(-21.8631332422781,51.8906300325692,-36.7408402239735));
#20713=CARTESIAN_POINT('Ctrl Pts',(-22.2423540255139,51.1533372037214,-36.6881907162427));
#20714=CARTESIAN_POINT('Ctrl Pts',(-22.6215748087496,50.4160443748736,-36.6355412085118));
#20715=CARTESIAN_POINT('Ctrl Pts',(-22.6016315806666,49.473444668616,-36.582891700781));
#20716=CARTESIAN_POINT('Ctrl Pts',(-22.1915653009581,48.7528513271896,-36.5302421930502));
#20717=CARTESIAN_POINT('Ctrl Pts',(-21.7814990212495,48.0322579857633,-36.4775926853194));
#20718=CARTESIAN_POINT('Ctrl Pts',(-20.9813096899156,47.5336710091681,-36.4249431775885));
#20719=CARTESIAN_POINT('Ctrl Pts',(-20.1537509717286,47.4831172216533,-36.3722936698577));
#20720=CARTESIAN_POINT('Ctrl Pts',(-19.3261922535416,47.4325634341385,-36.3196441621269));
#20721=CARTESIAN_POINT('Ctrl Pts',(-18.4712641485017,47.830042835704,-36.2669946543961));
#20722=CARTESIAN_POINT('Ctrl Pts',(-17.976535312427,48.4953641838799,-36.2143451466653));
#20723=CARTESIAN_POINT('Ctrl Pts',(-17.6577952716397,48.9240122395235,-36.1804245319408));
#20724=CARTESIAN_POINT('Ctrl Pts',(-17.4885691499591,49.4638379198578,-36.1465039172164));
#20725=CARTESIAN_POINT('Ctrl Pts',(-17.4851666106336,50.0017093726515,-36.112583302492));
#20726=CARTESIAN_POINT('Ctrl Pts',(-17.4799716856498,50.0016863230979,-36.387416697508));
#20727=CARTESIAN_POINT('Ctrl Pts',(-17.4855715685639,49.277614661599,-36.4333219615939));
#20728=CARTESIAN_POINT('Ctrl Pts',(-17.8146387939379,48.5490984621573,-36.4792272256798));
#20729=CARTESIAN_POINT('Ctrl Pts',(-18.3649693501693,48.0803607431838,-36.5251324897657));
#20730=CARTESIAN_POINT('Ctrl Pts',(-18.9961525804978,47.5427576893674,-36.5777819974965));
#20731=CARTESIAN_POINT('Ctrl Pts',(-19.9183894912617,47.3468718217887,-36.6304315052273));
#20732=CARTESIAN_POINT('Ctrl Pts',(-20.7135980034659,47.5815050164462,-36.6830810129582));
#20733=CARTESIAN_POINT('Ctrl Pts',(-21.5088065156701,47.8161382111036,-36.735730520689));
#20734=CARTESIAN_POINT('Ctrl Pts',(-22.1769866293146,48.4812904679973,-36.7883800284198));
#20735=CARTESIAN_POINT('Ctrl Pts',(-22.4152290503386,49.2754251328188,-36.8410295361506));
#20736=CARTESIAN_POINT('Ctrl Pts',(-22.6534714713626,50.0695597976402,-36.8936790438815));
#20737=CARTESIAN_POINT('Ctrl Pts',(-22.4617761997662,50.9926768703893,-36.9463285516123));
#20738=CARTESIAN_POINT('Ctrl Pts',(-21.9270453727093,51.6262952508436,-36.9989780593431));
#20739=CARTESIAN_POINT('Ctrl Pts',(-21.3923145456525,52.2599136312978,-37.0516275670739));
#20740=CARTESIAN_POINT('Ctrl Pts',(-20.5145481631352,52.6040333194572,-37.1042770748047));
#20741=CARTESIAN_POINT('Ctrl Pts',(-19.6916682649385,52.502652913465,-37.1569265825356));
#20742=CARTESIAN_POINT('Ctrl Pts',(-18.8687883667419,52.4012725074729,-37.2095760902664));
#20743=CARTESIAN_POINT('Ctrl Pts',(-18.100794952866,51.8543920073292,-37.2622255979972));
#20744=CARTESIAN_POINT('Ctrl Pts',(-17.735846162153,51.1099313200771,-37.314875105728));
#20745=CARTESIAN_POINT('Ctrl Pts',(-17.5682348058617,50.768020157001,-37.3390556363214));
#20746=CARTESIAN_POINT('Ctrl Pts',(-17.4856385661448,50.3844329568945,-37.3632361669147));
#20747=CARTESIAN_POINT('Ctrl Pts',(-17.4863843841259,50.0005414264851,-37.387416697508));
#20748=CARTESIAN_POINT('Origin',(-20.,50.,-32.));
#20749=CARTESIAN_POINT('',(-17.4818815371047,49.9978011132584,-38.387416697508));
#20750=CARTESIAN_POINT('',(-17.4784633668112,50.000273285299,-38.112583302492));
#20751=CARTESIAN_POINT('',(-17.4825,50.,-32.));
#20752=CARTESIAN_POINT('Ctrl Pts',(-17.4784633668112,50.000273285299,-38.112583302492));
#20753=CARTESIAN_POINT('Ctrl Pts',(-17.4784400677728,50.0152649329971,-38.1116313433196));
#20754=CARTESIAN_POINT('Ctrl Pts',(-17.4785623286431,50.0302561905308,-38.1106793841472));
#20755=CARTESIAN_POINT('Ctrl Pts',(-17.4788313122131,50.0452448149025,-38.1097274249749));
#20756=CARTESIAN_POINT('Ctrl Pts',(-17.4937078457445,50.87421281861,-38.0570779172441));
#20757=CARTESIAN_POINT('Ctrl Pts',(-17.9573807060435,51.6951264893194,-38.0044284095132));
#20758=CARTESIAN_POINT('Ctrl Pts',(-18.6596506001565,52.1358374187989,-37.9517789017824));
#20759=CARTESIAN_POINT('Ctrl Pts',(-19.3619204942694,52.5765483482785,-37.8991293940516));
#20760=CARTESIAN_POINT('Ctrl Pts',(-20.3027874221963,52.6370565365281,-37.8464798863208));
#20761=CARTESIAN_POINT('Ctrl Pts',(-21.0557237967043,52.2899313553352,-37.7938303785899));
#20762=CARTESIAN_POINT('Ctrl Pts',(-21.8086601712123,51.9428061741423,-37.7411808708591));
#20763=CARTESIAN_POINT('Ctrl Pts',(-22.3736659923015,51.1880476235069,-37.6885313631283));
#20764=CARTESIAN_POINT('Ctrl Pts',(-22.4946043991423,50.3678140958698,-37.6358818553975));
#20765=CARTESIAN_POINT('Ctrl Pts',(-22.6155428059831,49.5475805682327,-37.5832323476666));
#20766=CARTESIAN_POINT('Ctrl Pts',(-22.2924137985756,48.661872063594,-37.5305828399358));
#20767=CARTESIAN_POINT('Ctrl Pts',(-21.6717030307037,48.1122110230468,-37.477933332205));
#20768=CARTESIAN_POINT('Ctrl Pts',(-21.0509922628319,47.5625499824997,-37.4252838244742));
#20769=CARTESIAN_POINT('Ctrl Pts',(-20.1326997344957,47.3489364060442,-37.3726343167433));
#20770=CARTESIAN_POINT('Ctrl Pts',(-19.3331193830197,47.5682087806212,-37.3199848090125));
#20771=CARTESIAN_POINT('Ctrl Pts',(-18.5335390315437,47.7874811551982,-37.2673353012817));
#20772=CARTESIAN_POINT('Ctrl Pts',(-17.8526708569279,48.4396394808077,-37.2146857935509));
#20773=CARTESIAN_POINT('Ctrl Pts',(-17.5991761003846,49.2290376875177,-37.1620362858201));
#20774=CARTESIAN_POINT('Ctrl Pts',(-17.519808014405,49.476194771146,-37.1455519580441));
#20775=CARTESIAN_POINT('Ctrl Pts',(-17.4823348478425,49.7368053207982,-37.129067630268));
#20776=CARTESIAN_POINT('Ctrl Pts',(-17.4843372649484,49.997976158615,-37.112583302492));
#20777=CARTESIAN_POINT('Ctrl Pts',(-17.4863843841259,50.0005414264851,-37.387416697508));
#20778=CARTESIAN_POINT('Ctrl Pts',(-17.4872624738341,49.5485662657117,-37.4158856746455));
#20779=CARTESIAN_POINT('Ctrl Pts',(-17.6036656476806,49.0961692556964,-37.444354651783));
#20780=CARTESIAN_POINT('Ctrl Pts',(-17.8328634864205,48.7108687042736,-37.4728236289205));
#20781=CARTESIAN_POINT('Ctrl Pts',(-18.256733768951,47.9983076500828,-37.5254731366513));
#20782=CARTESIAN_POINT('Ctrl Pts',(-19.0663785015622,47.5152264160619,-37.5781226443822));
#20783=CARTESIAN_POINT('Ctrl Pts',(-19.894757570296,47.4806223297718,-37.630772152113));
#20784=CARTESIAN_POINT('Ctrl Pts',(-20.7231366390297,47.4460182434818,-37.6834216598438));
#20785=CARTESIAN_POINT('Ctrl Pts',(-21.5702500438859,47.8598913049226,-37.7360711675746));
#20786=CARTESIAN_POINT('Ctrl Pts',(-22.0520717778747,48.5346188611104,-37.7887206753054));
#20787=CARTESIAN_POINT('Ctrl Pts',(-22.5338935118636,49.2093464172982,-37.8413701830363));
#20788=CARTESIAN_POINT('Ctrl Pts',(-22.6504235749849,50.144928468233,-37.8940196907671));
#20789=CARTESIAN_POINT('Ctrl Pts',(-22.3488348885255,50.9172323104341,-37.9466691984979));
#20790=CARTESIAN_POINT('Ctrl Pts',(-22.0472462020662,51.6895361526352,-37.9993187062287));
#20791=CARTESIAN_POINT('Ctrl Pts',(-21.327538766026,52.2985617861026,-38.0519682139595));
#20792=CARTESIAN_POINT('Ctrl Pts',(-20.5159808958408,52.468218309994,-38.1046177216904));
#20793=CARTESIAN_POINT('Ctrl Pts',(-19.7044230256556,52.6378748338855,-38.1572672294212));
#20794=CARTESIAN_POINT('Ctrl Pts',(-18.8010147213253,52.3681622482009,-38.209916737152));
#20795=CARTESIAN_POINT('Ctrl Pts',(-18.2153026112017,51.781347448765,-38.2625662448829));
#20796=CARTESIAN_POINT('Ctrl Pts',(-17.7523263162739,51.3174995327738,-38.3041830624246));
#20797=CARTESIAN_POINT('Ctrl Pts',(-17.4878502975171,50.6555224665065,-38.3457998799663));
#20798=CARTESIAN_POINT('Ctrl Pts',(-17.4818815371047,49.9978011132584,-38.387416697508));
#20799=CARTESIAN_POINT('Origin',(-20.,50.,-32.));
#20800=CARTESIAN_POINT('',(-17.4798420534852,50.0015648820515,-39.387416697508));
#20801=CARTESIAN_POINT('',(-17.4850543912228,50.0017607343381,-39.112583302492));
#20802=CARTESIAN_POINT('',(-17.4825,50.,-32.));
#20803=CARTESIAN_POINT('',(-21.913465996665,51.635987203375,-40.));
#20804=CARTESIAN_POINT('Ctrl Pts',(-17.4798420534852,50.0015648820515,-39.387416697508));
#20805=CARTESIAN_POINT('Ctrl Pts',(-17.4853146187272,49.2723761097304,-39.4336626084795));
#20806=CARTESIAN_POINT('Ctrl Pts',(-17.8198668900926,48.5389623205324,-39.4799085194511));
#20807=CARTESIAN_POINT('Ctrl Pts',(-18.3773137076179,48.0701212737088,-39.5261544304226));
#20808=CARTESIAN_POINT('Ctrl Pts',(-19.0119492875483,47.5363605627465,-39.5788039381534));
#20809=CARTESIAN_POINT('Ctrl Pts',(-19.9354807781592,47.345515300665,-39.6314534458843));
#20810=CARTESIAN_POINT('Ctrl Pts',(-20.7291493676954,47.5857188348087,-39.6841029536151));
#20811=CARTESIAN_POINT('Ctrl Pts',(-21.5228179572316,47.8259223689524,-39.7367524613459));
#20812=CARTESIAN_POINT('Ctrl Pts',(-22.186623645693,48.4971746993212,-39.7894019690767));
#20813=CARTESIAN_POINT('Ctrl Pts',(-22.4195845021318,49.2914441063715,-39.8420514768075));
#20814=CARTESIAN_POINT('Ctrl Pts',(-22.6525453585705,50.0857135134218,-39.8947009845384));
#20815=CARTESIAN_POINT('Ctrl Pts',(-22.4546613829867,51.0029999971535,-39.9473504922692));
#20816=CARTESIAN_POINT('Ctrl Pts',(-21.913465996665,51.635987203375,-40.));
#20817=CARTESIAN_POINT('',(-18.0829274149968,51.6385410457703,-40.));
#20818=CARTESIAN_POINT('Origin',(-20.,50.,-40.));
#20819=CARTESIAN_POINT('Ctrl Pts',(-18.0829199122823,51.6385463584782,-40.));
#20820=CARTESIAN_POINT('Ctrl Pts',(-18.6057517999179,52.2473170096207,-39.9490537266974));
#20821=CARTESIAN_POINT('Ctrl Pts',(-19.4454474456028,52.5873618729563,-39.8981074533947));
#20822=CARTESIAN_POINT('Ctrl Pts',(-20.2440955105381,52.5095729322154,-39.847161180092));
#20823=CARTESIAN_POINT('Ctrl Pts',(-21.0694439559331,52.429183353716,-39.7945116723612));
#20824=CARTESIAN_POINT('Ctrl Pts',(-21.8509543386143,51.9025549428044,-39.7418621646304));
#20825=CARTESIAN_POINT('Ctrl Pts',(-22.23483319536,51.1677991240005,-39.6892126568996));
#20826=CARTESIAN_POINT('Ctrl Pts',(-22.6187120521057,50.4330433051966,-39.6365631491688));
#20827=CARTESIAN_POINT('Ctrl Pts',(-22.6049593829159,49.4901600785004,-39.5839136414379));
#20828=CARTESIAN_POINT('Ctrl Pts',(-22.1995627546363,48.7669050303447,-39.5312641337071));
#20829=CARTESIAN_POINT('Ctrl Pts',(-21.7941661263566,48.0436499821891,-39.4786146259763));
#20830=CARTESIAN_POINT('Ctrl Pts',(-20.9971255389871,47.5400231125739,-39.4259651182454));
#20831=CARTESIAN_POINT('Ctrl Pts',(-20.1698912732234,47.4841784721833,-39.3733156105146));
#20832=CARTESIAN_POINT('Ctrl Pts',(-19.3426570074598,47.4283338317928,-39.3206661027838));
#20833=CARTESIAN_POINT('Ctrl Pts',(-18.4852290633019,47.8202714206268,-39.268016595053));
#20834=CARTESIAN_POINT('Ctrl Pts',(-17.9862470456528,48.4823914203806,-39.2153670873221));
#20835=CARTESIAN_POINT('Ctrl Pts',(-17.6615383411993,48.9132609100784,-39.1811058257121));
#20836=CARTESIAN_POINT('Ctrl Pts',(-17.4886191336564,49.4585433396218,-39.146844564102));
#20837=CARTESIAN_POINT('Ctrl Pts',(-17.4850543912228,50.0017607343381,-39.112583302492));
#20838=CARTESIAN_POINT('Origin',(-20.,50.,-42.2084234471774));
#20839=CARTESIAN_POINT('',(-16.9217886712226,50.0008183699211,-25.7915765528226));
#20840=CARTESIAN_POINT('',(-16.9314303843609,50.000333147012,-25.7084234471775));
#20841=CARTESIAN_POINT('',(-16.9265,50.0000000000002,-42.2084234471774));
#20842=CARTESIAN_POINT('',(-20.7937992825328,47.0307770462543,-25.));
#20843=CARTESIAN_POINT('Ctrl Pts',(-16.9314303843609,50.000333147012,-25.7084234471775));
#20844=CARTESIAN_POINT('Ctrl Pts',(-16.9311123866597,50.4955100463338,-25.6828803290416));
#20845=CARTESIAN_POINT('Ctrl Pts',(-17.2773641840547,52.0108184567304,-25.6046877031749));
#20846=CARTESIAN_POINT('Ctrl Pts',(-19.6484750337391,53.6086169320315,-25.4738455695774));
#20847=CARTESIAN_POINT('Ctrl Pts',(-22.8319255534364,52.2686663415281,-25.315897046385));
#20848=CARTESIAN_POINT('Ctrl Pts',(-23.4429082212044,48.865459646895,-25.1579485231924));
#20849=CARTESIAN_POINT('Ctrl Pts',(-21.7760378723045,47.2933710986319,-25.0526495077308));
#20850=CARTESIAN_POINT('Ctrl Pts',(-20.7937992825328,47.0307770462543,-25.));
#20851=CARTESIAN_POINT('',(-19.2062007174672,47.0307770462543,-25.));
#20852=CARTESIAN_POINT('Origin',(-20.,50.,-25.));
#20853=CARTESIAN_POINT('Ctrl Pts',(-16.9217886712226,50.0008183699211,-25.7915765528226));
#20854=CARTESIAN_POINT('Ctrl Pts',(-16.9216326522162,50.0453262421124,-25.7892620061077));
#20855=CARTESIAN_POINT('Ctrl Pts',(-16.9425932420072,51.1021122351085,-25.7342979516619));
#20856=CARTESIAN_POINT('Ctrl Pts',(-18.1518494766411,53.1200731989091,-25.6266843894854));
#20857=CARTESIAN_POINT('Ctrl Pts',(-21.6024146227446,53.2535259255151,-25.4687358662929));
#20858=CARTESIAN_POINT('Ctrl Pts',(-23.6000558056709,50.4361300140704,-25.3107873431005));
#20859=CARTESIAN_POINT('Ctrl Pts',(-22.3474165158894,47.2598763198176,-25.1545420543361));
#20860=CARTESIAN_POINT('Ctrl Pts',(-20.1513504643245,46.7747742461176,-25.0509462733027));
#20861=CARTESIAN_POINT('Ctrl Pts',(-19.2043343151472,47.0257029622097,-25.));
#20862=CARTESIAN_POINT('Origin',(-20.,50.,-42.2084234471774));
#20863=CARTESIAN_POINT('',(-16.9301481064099,50.0018654683783,-26.7915765528225));
#20864=CARTESIAN_POINT('',(-16.9249664934092,49.9974416687219,-26.7084234471774));
#20865=CARTESIAN_POINT('',(-16.9265,50.0000000000002,-42.2084234471774));
#20866=CARTESIAN_POINT('Ctrl Pts',(-16.9249664934092,49.9974416687219,-26.7084234471774));
#20867=CARTESIAN_POINT('Ctrl Pts',(-16.932354404873,50.8261741257165,-26.6654440420932));
#20868=CARTESIAN_POINT('Ctrl Pts',(-17.7039892803895,52.6822303383337,-26.5698151292781));
#20869=CARTESIAN_POINT('Ctrl Pts',(-20.8329798605529,53.5295001824726,-26.4215367087322));
#20870=CARTESIAN_POINT('Ctrl Pts',(-23.4108311578128,51.2319837018569,-26.2635881855397));
#20871=CARTESIAN_POINT('Ctrl Pts',(-22.8961090069582,47.8173680419797,-26.1056396623473));
#20872=CARTESIAN_POINT('Ctrl Pts',(-19.7557253769871,46.3818716002278,-25.9476911391548));
#20873=CARTESIAN_POINT('Ctrl Pts',(-17.3086034215628,47.9281379315223,-25.8152857340982));
#20874=CARTESIAN_POINT('Ctrl Pts',(-16.9317678439275,49.4748507889046,-25.7355298367724));
#20875=CARTESIAN_POINT('Ctrl Pts',(-16.9314303843609,50.000333147012,-25.7084234471775));
#20876=CARTESIAN_POINT('Ctrl Pts',(-16.9301481064099,50.0018654683783,-26.7915765528225));
#20877=CARTESIAN_POINT('Ctrl Pts',(-16.9280040139011,50.3843410166761,-26.7718257191592));
#20878=CARTESIAN_POINT('Ctrl Pts',(-17.1709937020916,51.7837498364551,-26.6994253777651));
#20879=CARTESIAN_POINT('Ctrl Pts',(-19.2579267840424,53.5497392783032,-26.5743755286402));
#20880=CARTESIAN_POINT('Ctrl Pts',(-22.5667152906276,52.5619003598412,-26.4164270054477));
#20881=CARTESIAN_POINT('Ctrl Pts',(-23.5483400872305,49.251248624616,-26.2584784822553));
#20882=CARTESIAN_POINT('Ctrl Pts',(-21.3127948732631,46.619498196827,-26.1005299590628));
#20883=CARTESIAN_POINT('Ctrl Pts',(-17.9371757378006,47.0463360002771,-25.9448959825852));
#20884=CARTESIAN_POINT('Ctrl Pts',(-16.9251816511758,49.0328957969052,-25.8419115138385));
#20885=CARTESIAN_POINT('Ctrl Pts',(-16.9217886712226,50.0008183699211,-25.7915765528226));
#20886=CARTESIAN_POINT('Origin',(-20.,50.,-42.2084234471774));
#20887=CARTESIAN_POINT('',(-16.9282249073135,49.997407390353,-27.7915765528225));
#20888=CARTESIAN_POINT('',(-16.9239286259646,50.0022679987088,-27.7084234471775));
#20889=CARTESIAN_POINT('',(-16.9265,50.0000000000002,-42.2084234471774));
#20890=CARTESIAN_POINT('Ctrl Pts',(-16.9239286259646,50.0022679987088,-27.7084234471775));
#20891=CARTESIAN_POINT('Ctrl Pts',(-16.9226895286024,50.1518848536015,-27.7006572628756));
#20892=CARTESIAN_POINT('Ctrl Pts',(-17.0003509237025,51.314512346611,-27.640241570843));
#20893=CARTESIAN_POINT('Ctrl Pts',(-18.4816793672832,53.2933332139959,-27.5271763710795));
#20894=CARTESIAN_POINT('Ctrl Pts',(-21.9276633802435,53.0717181892534,-27.369227847887));
#20895=CARTESIAN_POINT('Ctrl Pts',(-23.6258942504405,50.0650704860399,-27.2112793246945));
#20896=CARTESIAN_POINT('Ctrl Pts',(-22.0366358520053,46.9994237957239,-27.0533308015021));
#20897=CARTESIAN_POINT('Ctrl Pts',(-18.6008241139817,46.6543113906855,-26.8953822783096));
#20898=CARTESIAN_POINT('Ctrl Pts',(-17.0233221444774,48.6111088305139,-26.7804131602014));
#20899=CARTESIAN_POINT('Ctrl Pts',(-16.9233042586235,49.8109819466767,-26.718093549824));
#20900=CARTESIAN_POINT('Ctrl Pts',(-16.9249664934092,49.9974416687219,-26.7084234471774));
#20901=CARTESIAN_POINT('Ctrl Pts',(-16.9282249073135,49.997407390353,-27.7915765528225));
#20902=CARTESIAN_POINT('Ctrl Pts',(-16.9340842388497,50.7163995761236,-27.7543894322109));
#20903=CARTESIAN_POINT('Ctrl Pts',(-17.5432833311101,52.462287433857,-27.6645528038683));
#20904=CARTESIAN_POINT('Ctrl Pts',(-20.4434363605156,53.599263941172,-27.522066667795));
#20905=CARTESIAN_POINT('Ctrl Pts',(-23.2562595022286,51.5962804541496,-27.3641181446025));
#20906=CARTESIAN_POINT('Ctrl Pts',(-23.1167311715492,48.1459977760775,-27.2061696214101));
#20907=CARTESIAN_POINT('Ctrl Pts',(-20.151357511322,46.3766830290446,-27.0482210982176));
#20908=CARTESIAN_POINT('Ctrl Pts',(-17.4367209277074,47.7029693850521,-26.9100234086884));
#20909=CARTESIAN_POINT('Ctrl Pts',(-16.9337194898675,49.3647815550225,-26.8244752268901));
#20910=CARTESIAN_POINT('Ctrl Pts',(-16.9301481064099,50.0018654683783,-26.7915765528225));
#20911=CARTESIAN_POINT('Origin',(-20.,50.,-42.2084234471774));
#20912=CARTESIAN_POINT('',(-16.9217182551955,50.0006847935455,-28.7915765528225));
#20913=CARTESIAN_POINT('',(-16.9313401597895,50.0003484095168,-28.7084234471775));
#20914=CARTESIAN_POINT('',(-16.9265,50.0000000000002,-42.2084234471774));
#20915=CARTESIAN_POINT('Ctrl Pts',(-16.9313401597895,50.0003484095168,-28.7084234471775));
#20916=CARTESIAN_POINT('Ctrl Pts',(-16.9308408739778,50.4888704797936,-28.6832209759272));
#20917=CARTESIAN_POINT('Ctrl Pts',(-17.2704953682473,51.9972892968429,-28.6053689969462));
#20918=CARTESIAN_POINT('Ctrl Pts',(-19.6259746483565,53.6071381719488,-28.4748675102343));
#20919=CARTESIAN_POINT('Ctrl Pts',(-22.8159750830834,52.2850875351969,-28.3169189870418));
#20920=CARTESIAN_POINT('Ctrl Pts',(-23.4528165638848,48.8912175406165,-28.1589704638494));
#20921=CARTESIAN_POINT('Ctrl Pts',(-20.9590942591762,46.5026468548974,-28.0010219406569));
#20922=CARTESIAN_POINT('Ctrl Pts',(-17.7611609705603,47.2465513795375,-27.8508396017663));
#20923=CARTESIAN_POINT('Ctrl Pts',(-16.9310897755726,49.1375831769752,-27.7533067706065));
#20924=CARTESIAN_POINT('Ctrl Pts',(-16.9239286259646,50.0022679987088,-27.7084234471775));
#20925=CARTESIAN_POINT('Ctrl Pts',(-16.9217182551955,50.0006847935455,-28.7915765528225));
#20926=CARTESIAN_POINT('Ctrl Pts',(-16.9216026134698,50.0386403438613,-28.7896026529933));
#20927=CARTESIAN_POINT('Ctrl Pts',(-16.9393662086373,51.0888673611757,-28.7349792454332));
#20928=CARTESIAN_POINT('Ctrl Pts',(-18.1318615954084,53.1082786044884,-28.6277063301423));
#20929=CARTESIAN_POINT('Ctrl Pts',(-21.5814747736461,53.2634758336214,-28.4697578069498));
#20930=CARTESIAN_POINT('Ctrl Pts',(-23.5972128731322,50.4597787805748,-28.3118092837574));
#20931=CARTESIAN_POINT('Ctrl Pts',(-22.3514674645701,47.2392142866714,-28.1538607605649));
#20932=CARTESIAN_POINT('Ctrl Pts',(-18.9737180230564,46.5217702416014,-27.9959122373724));
#20933=CARTESIAN_POINT('Ctrl Pts',(-17.1026436278435,48.3843658671474,-27.8751508347916));
#20934=CARTESIAN_POINT('Ctrl Pts',(-16.9257886000388,49.6984507803992,-27.8070389399417));
#20935=CARTESIAN_POINT('Ctrl Pts',(-16.9282249073135,49.997407390353,-27.7915765528225));
#20936=CARTESIAN_POINT('Origin',(-20.,50.,-42.2084234471774));
#20937=CARTESIAN_POINT('',(-16.930022476882,50.0019420176801,-29.7915765528225));
#20938=CARTESIAN_POINT('',(-16.9251594783372,49.9974042565776,-29.7084234471774));
#20939=CARTESIAN_POINT('',(-16.9265,50.0000000000002,-42.2084234471774));
#20940=CARTESIAN_POINT('Ctrl Pts',(-16.9251594783372,49.9974042565776,-29.7084234471775));
#20941=CARTESIAN_POINT('Ctrl Pts',(-16.9325402148186,50.8197003396064,-29.6657846889788));
#20942=CARTESIAN_POINT('Ctrl Pts',(-17.6939854162501,52.6694193953535,-29.5704964230494));
#20943=CARTESIAN_POINT('Ctrl Pts',(-20.8103104076337,53.5347896383079,-29.4225586493891));
#20944=CARTESIAN_POINT('Ctrl Pts',(-23.4028291041448,51.2538320585774,-29.2646101261967));
#20945=CARTESIAN_POINT('Ctrl Pts',(-22.9101061444555,47.8360630851142,-29.1066616030042));
#20946=CARTESIAN_POINT('Ctrl Pts',(-19.7788784501499,46.3802698988112,-28.9487130798117));
#20947=CARTESIAN_POINT('Ctrl Pts',(-17.3157681767346,47.9150000634711,-28.8159670278695));
#20948=CARTESIAN_POINT('Ctrl Pts',(-16.9318839126521,49.4683179212627,-28.735870483658));
#20949=CARTESIAN_POINT('Ctrl Pts',(-16.9313401597895,50.0003484095168,-28.7084234471775));
#20950=CARTESIAN_POINT('Ctrl Pts',(-16.930022476882,50.0019420176801,-29.7915765528225));
#20951=CARTESIAN_POINT('Ctrl Pts',(-16.9278228426505,50.3777822124665,-29.7721663660449));
#20952=CARTESIAN_POINT('Ctrl Pts',(-17.1652525268972,51.7703947269283,-29.7001066715364));
#20953=CARTESIAN_POINT('Ctrl Pts',(-19.2351493401782,53.5449034469686,-29.5753974692971));
#20954=CARTESIAN_POINT('Ctrl Pts',(-22.5502121640569,52.5783240483645,-29.4174489461047));
#20955=CARTESIAN_POINT('Ctrl Pts',(-23.5530751799844,49.274056651322,-29.2595004229121));
#20956=CARTESIAN_POINT('Ctrl Pts',(-21.3344729921125,46.627980009892,-29.1015518997197));
#20957=CARTESIAN_POINT('Ctrl Pts',(-17.9487914181142,47.0340721357474,-28.9455772763565));
#20958=CARTESIAN_POINT('Ctrl Pts',(-16.9246871063329,49.0262581499145,-28.8422521607241));
#20959=CARTESIAN_POINT('Ctrl Pts',(-16.9217182551955,50.0006847935455,-28.7915765528225));
#20960=CARTESIAN_POINT('Origin',(-20.,50.,-42.2084234471774));
#20961=CARTESIAN_POINT('',(-16.9284009962433,49.9974440495234,-30.7915765528225));
#20962=CARTESIAN_POINT('',(-16.9237528526042,50.0022022524448,-30.7084234471775));
#20963=CARTESIAN_POINT('',(-16.9265,50.0000000000002,-42.2084234471774));
#20964=CARTESIAN_POINT('Ctrl Pts',(-16.9237528526042,50.0022022524448,-30.7084234471775));
#20965=CARTESIAN_POINT('Ctrl Pts',(-16.922592011601,50.1452351674692,-30.7009979097613));
#20966=CARTESIAN_POINT('Ctrl Pts',(-16.9963969117474,51.301214910621,-30.6409228646143));
#20967=CARTESIAN_POINT('Ctrl Pts',(-18.460564094239,53.2835160781738,-30.5281983117364));
#20968=CARTESIAN_POINT('Ctrl Pts',(-21.9079003148171,53.0840326088254,-30.3702497885439));
#20969=CARTESIAN_POINT('Ctrl Pts',(-23.6254013461144,50.0883505696652,-30.2123012653514));
#20970=CARTESIAN_POINT('Ctrl Pts',(-22.05586123849,47.0125637560539,-30.054352742159));
#20971=CARTESIAN_POINT('Ctrl Pts',(-18.6223342721148,46.6453945260559,-29.8964042189665));
#20972=CARTESIAN_POINT('Ctrl Pts',(-17.0275919910131,48.5977940122777,-29.7810944539727));
#20973=CARTESIAN_POINT('Ctrl Pts',(-16.9234266252383,49.8043451601994,-29.7184341967097));
#20974=CARTESIAN_POINT('Ctrl Pts',(-16.9251594783372,49.9974042565776,-29.7084234471775));
#20975=CARTESIAN_POINT('Ctrl Pts',(-16.9284009962433,49.9974440495234,-30.7915765528225));
#20976=CARTESIAN_POINT('Ctrl Pts',(-16.9340999379478,50.7099535572267,-30.7547300790965));
#20977=CARTESIAN_POINT('Ctrl Pts',(-17.534439538246,52.4492247638631,-30.6652340976396));
#20978=CARTESIAN_POINT('Ctrl Pts',(-20.4203163532235,53.6020370824496,-30.5230886084519));
#20979=CARTESIAN_POINT('Ctrl Pts',(-23.2459426566631,51.6171559138756,-30.3651400852594));
#20980=CARTESIAN_POINT('Ctrl Pts',(-23.1285714741897,48.166048661765,-30.207191562067));
#20981=CARTESIAN_POINT('Ctrl Pts',(-20.1746196872686,46.3777293109224,-30.0492430388745));
#20982=CARTESIAN_POINT('Ctrl Pts',(-17.4448107975432,47.689784542327,-29.9107047024597));
#20983=CARTESIAN_POINT('Ctrl Pts',(-16.9337892798002,49.3583277647774,-29.8248158737757));
#20984=CARTESIAN_POINT('Ctrl Pts',(-16.930022476882,50.0019420176801,-29.7915765528225));
#20985=CARTESIAN_POINT('Origin',(-20.,50.,-42.2084234471774));
#20986=CARTESIAN_POINT('',(-16.9216590200037,50.0005689006534,-31.7915765528225));
#20987=CARTESIAN_POINT('',(-16.9313142832549,50.0004533262794,-31.7084234471775));
#20988=CARTESIAN_POINT('',(-16.9265,50.0000000000002,-42.2084234471774));
#20989=CARTESIAN_POINT('Ctrl Pts',(-16.9313142832549,50.0004533262794,-31.7084234471775));
#20990=CARTESIAN_POINT('Ctrl Pts',(-16.9306731189746,50.4823621763928,-31.6835616228129));
#20991=CARTESIAN_POINT('Ctrl Pts',(-17.2638484234452,51.9839635458219,-31.6060502907175));
#20992=CARTESIAN_POINT('Ctrl Pts',(-19.6028209290277,53.604662193487,-31.4758894508912));
#20993=CARTESIAN_POINT('Ctrl Pts',(-22.8012444915916,52.3031218035313,-31.3179409276987));
#20994=CARTESIAN_POINT('Ctrl Pts',(-23.4598648696293,48.913410920597,-31.1599924045063));
#20995=CARTESIAN_POINT('Ctrl Pts',(-20.9815309974076,46.5088773088445,-31.0020438813138));
#20996=CARTESIAN_POINT('Ctrl Pts',(-17.7716226853989,47.2338732641192,-30.8515208955375));
#20997=CARTESIAN_POINT('Ctrl Pts',(-16.9308227569255,49.131084656435,-30.7536474174921));
#20998=CARTESIAN_POINT('Ctrl Pts',(-16.9237528526042,50.0022022524448,-30.7084234471775));
#20999=CARTESIAN_POINT('Ctrl Pts',(-16.9216590200037,50.0005689006534,-31.7915765528225));
#21000=CARTESIAN_POINT('Ctrl Pts',(-16.9215783383011,50.031972629415,-31.7899432998789));
#21001=CARTESIAN_POINT('Ctrl Pts',(-16.9361832221292,51.075629445688,-31.7356605392045));
#21002=CARTESIAN_POINT('Ctrl Pts',(-18.1119418547959,53.0962192138892,-31.6287282707992));
#21003=CARTESIAN_POINT('Ctrl Pts',(-21.56048739876,53.2735632052001,-31.4707797476067));
#21004=CARTESIAN_POINT('Ctrl Pts',(-23.5941864783473,50.4828669992804,-31.3128312244143));
#21005=CARTESIAN_POINT('Ctrl Pts',(-22.3691459902575,47.2543699708491,-31.1548827012218));
#21006=CARTESIAN_POINT('Ctrl Pts',(-18.9960728871194,46.5152521852863,-30.9969341780293));
#21007=CARTESIAN_POINT('Ctrl Pts',(-17.1077657383409,48.3710153180247,-30.8758321285629));
#21008=CARTESIAN_POINT('Ctrl Pts',(-16.9259567848863,49.6918568157852,-30.8073795868273));
#21009=CARTESIAN_POINT('Ctrl Pts',(-16.9284009962433,49.9974440495234,-30.7915765528225));
#21010=CARTESIAN_POINT('Origin',(-20.,50.,-42.2084234471774));
#21011=CARTESIAN_POINT('',(-16.9298915772933,50.0020159666225,-32.7915765528225));
#21012=CARTESIAN_POINT('',(-16.92535365788,49.9973711108991,-32.7084234471774));
#21013=CARTESIAN_POINT('',(-16.9265,50.0000000000002,-42.2084234471774));
#21014=CARTESIAN_POINT('Ctrl Pts',(-16.92535365788,49.9973711108991,-32.7084234471774));
#21015=CARTESIAN_POINT('Ctrl Pts',(-16.9327153463397,50.8132307133283,-32.6661253358645));
#21016=CARTESIAN_POINT('Ctrl Pts',(-17.6840554370644,52.6565961172178,-32.5711777168207));
#21017=CARTESIAN_POINT('Ctrl Pts',(-20.7875968246039,53.5399197710466,-32.423580590046));
#21018=CARTESIAN_POINT('Ctrl Pts',(-23.3947081018314,51.2756557713323,-32.2656320668536));
#21019=CARTESIAN_POINT('Ctrl Pts',(-22.9239407885082,47.8547934810673,-32.107683543661));
#21020=CARTESIAN_POINT('Ctrl Pts',(-19.8021252898838,46.3789246980118,-31.9497350204686));
#21021=CARTESIAN_POINT('Ctrl Pts',(-17.3228654131711,47.9017052850683,-31.8166483216407));
#21022=CARTESIAN_POINT('Ctrl Pts',(-16.9320309028298,49.4618311261562,-31.7362111305437));
#21023=CARTESIAN_POINT('Ctrl Pts',(-16.9313142832549,50.0004533262794,-31.7084234471775));
#21024=CARTESIAN_POINT('Ctrl Pts',(-16.9298915772933,50.0020159666225,-32.7915765528225));
#21025=CARTESIAN_POINT('Ctrl Pts',(-16.9276421184013,50.3712206119457,-32.7725070129305));
#21026=CARTESIAN_POINT('Ctrl Pts',(-17.1595660076359,51.75703964909,-32.7007879653076));
#21027=CARTESIAN_POINT('Ctrl Pts',(-19.2124032880871,53.5399192645472,-32.576419409954));
#21028=CARTESIAN_POINT('Ctrl Pts',(-22.5336041773036,52.5946458048986,-32.4184708867615));
#21029=CARTESIAN_POINT('Ctrl Pts',(-23.5576632150468,49.2968859065335,-32.260522363569));
#21030=CARTESIAN_POINT('Ctrl Pts',(-21.3560972171426,46.6366181724659,-32.1025738403766));
#21031=CARTESIAN_POINT('Ctrl Pts',(-17.9604780872831,47.0218018745157,-31.9462585701278));
#21032=CARTESIAN_POINT('Ctrl Pts',(-16.9241791919761,49.0196426858764,-31.8425928076097));
#21033=CARTESIAN_POINT('Ctrl Pts',(-16.9216590200037,50.0005689006534,-31.7915765528225));
#21034=CARTESIAN_POINT('Origin',(-20.,50.,-42.2084234471774));
#21035=CARTESIAN_POINT('',(-16.9285737782481,49.997484673902,-33.7915765528225));
#21036=CARTESIAN_POINT('',(-16.9235809537435,50.0021324683887,-33.7084234471775));
#21037=CARTESIAN_POINT('',(-16.9265,50.0000000000002,-42.2084234471774));
#21038=CARTESIAN_POINT('Ctrl Pts',(-16.9235809537435,50.0021324683887,-33.7084234471775));
#21039=CARTESIAN_POINT('Ctrl Pts',(-16.9224984391972,50.1385838243685,-33.7013385566469));
#21040=CARTESIAN_POINT('Ctrl Pts',(-16.9924898021293,51.2879206387911,-33.6416041583855));
#21041=CARTESIAN_POINT('Ctrl Pts',(-18.4395123779619,53.2735636735887,-33.5292202523933));
#21042=CARTESIAN_POINT('Ctrl Pts',(-21.8880584153516,53.0962196569031,-33.3712717292008));
#21043=CARTESIAN_POINT('Ctrl Pts',(-23.6247593102429,50.1116274445677,-33.2133232060084));
#21044=CARTESIAN_POINT('Ctrl Pts',(-22.0750011806081,47.025826023238,-33.0553746828159));
#21045=CARTESIAN_POINT('Ctrl Pts',(-18.6439025888241,46.6366176912258,-32.8974261596234));
#21046=CARTESIAN_POINT('Ctrl Pts',(-17.0319087206847,48.584474479988,-32.7817757477439));
#21047=CARTESIAN_POINT('Ctrl Pts',(-16.923552070216,49.7977100408445,-32.7187748435953));
#21048=CARTESIAN_POINT('Ctrl Pts',(-16.92535365788,49.9973711108991,-32.7084234471774));
#21049=CARTESIAN_POINT('Ctrl Pts',(-16.9285737782481,49.997484673902,-33.7915765528225));
#21050=CARTESIAN_POINT('Ctrl Pts',(-16.9341072631217,50.7035075960413,-33.7550707259821));
#21051=CARTESIAN_POINT('Ctrl Pts',(-17.5256619221046,52.4361499397914,-33.6659153914109));
#21052=CARTESIAN_POINT('Ctrl Pts',(-20.3971790141429,53.6046616777241,-33.5241105491088));
#21053=CARTESIAN_POINT('Ctrl Pts',(-23.2354919865996,51.6379647690895,-33.3661620259163));
#21054=CARTESIAN_POINT('Ctrl Pts',(-23.140282777847,48.1861750207679,-33.2082135027238));
#21055=CARTESIAN_POINT('Ctrl Pts',(-20.1978746818039,46.3789252161231,-33.0502649795314));
#21056=CARTESIAN_POINT('Ctrl Pts',(-17.4529645572674,47.6766083004955,-32.911385996231));
#21057=CARTESIAN_POINT('Ctrl Pts',(-16.9338526984151,49.3518754710422,-32.8251565206613));
#21058=CARTESIAN_POINT('Ctrl Pts',(-16.9298915772933,50.0020159666225,-32.7915765528225));
#21059=CARTESIAN_POINT('Origin',(-20.,50.,-42.2084234471774));
#21060=CARTESIAN_POINT('',(-16.921610115697,50.0004517332244,-34.7915765528225));
#21061=CARTESIAN_POINT('',(-16.931281639274,50.0005575828105,-34.7084234471775));
#21062=CARTESIAN_POINT('',(-16.9265,50.0000000000002,-42.2084234471774));
#21063=CARTESIAN_POINT('Ctrl Pts',(-16.931281639274,50.0005575828105,-34.7084234471775));
#21064=CARTESIAN_POINT('Ctrl Pts',(-16.9305033497428,50.4758508700281,-34.6839022696985));
#21065=CARTESIAN_POINT('Ctrl Pts',(-17.257259818676,51.9706346069805,-34.6067315844887));
#21066=CARTESIAN_POINT('Ctrl Pts',(-19.5796835866367,53.602037597837,-34.4769113915481));
#21067=CARTESIAN_POINT('Ctrl Pts',(-22.7863984030238,52.3210611114746,-34.3189628683556));
#21068=CARTESIAN_POINT('Ctrl Pts',(-23.4667705318659,48.935649107221,-34.1610143451632));
#21069=CARTESIAN_POINT('Ctrl Pts',(-21.0039272565248,46.515251686681,-34.0030658219707));
#21070=CARTESIAN_POINT('Ctrl Pts',(-17.7821552253656,47.2212159324729,-33.8522021893088));
#21071=CARTESIAN_POINT('Ctrl Pts',(-16.9305428624281,49.1245813227702,-33.7539880643777));
#21072=CARTESIAN_POINT('Ctrl Pts',(-16.9235809537435,50.0021324683887,-33.7084234471775));
#21073=CARTESIAN_POINT('Ctrl Pts',(-16.921610115697,50.0004517332244,-34.7915765528225));
#21074=CARTESIAN_POINT('Ctrl Pts',(-16.9215586294445,50.0253045384473,-34.7902839467645));
#21075=CARTESIAN_POINT('Ctrl Pts',(-16.9330438936165,51.0623952825175,-34.7363418329757));
#21076=CARTESIAN_POINT('Ctrl Pts',(-18.0920999581694,53.0840321675552,-34.6297502114561));
#21077=CARTESIAN_POINT('Ctrl Pts',(-21.5394356854951,53.2835156083612,-34.4718016882636));
#21078=CARTESIAN_POINT('Ctrl Pts',(-23.5910118966017,50.50593531068,-34.3138531650712));
#21079=CARTESIAN_POINT('Ctrl Pts',(-22.3867268367498,47.2696388541317,-34.1559046418787));
#21080=CARTESIAN_POINT('Ctrl Pts',(-19.0184691430321,46.5088778083619,-33.9979561186862));
#21081=CARTESIAN_POINT('Ctrl Pts',(-17.1129400582668,48.3576637140246,-33.8765134223342));
#21082=CARTESIAN_POINT('Ctrl Pts',(-16.9261267493285,49.6852657833083,-33.8077202337129));
#21083=CARTESIAN_POINT('Ctrl Pts',(-16.9285737782481,49.997484673902,-33.7915765528225));
#21084=CARTESIAN_POINT('Origin',(-20.,50.,-42.2084234471774));
#21085=CARTESIAN_POINT('',(-16.9297555423167,50.0020868944765,-35.7915765528225));
#21086=CARTESIAN_POINT('',(-16.9255488571744,49.9973424349028,-35.7084234471775));
#21087=CARTESIAN_POINT('',(-16.9265,50.0000000000002,-42.2084234471774));
#21088=CARTESIAN_POINT('Ctrl Pts',(-16.9255488571744,49.9973424349028,-35.7084234471775));
#21089=CARTESIAN_POINT('Ctrl Pts',(-16.9328791333409,50.8067639659031,-35.6664659827501));
#21090=CARTESIAN_POINT('Ctrl Pts',(-17.6741947628828,52.6437552934631,-35.5718590105919));
#21091=CARTESIAN_POINT('Ctrl Pts',(-20.7648507692583,53.5449039541813,-35.4246025307029));
#21092=CARTESIAN_POINT('Ctrl Pts',(-23.3864471368627,51.2974268891935,-35.2666540075105));
#21093=CARTESIAN_POINT('Ctrl Pts',(-22.9376548796072,47.8736123232374,-35.108705484318));
#21094=CARTESIAN_POINT('Ctrl Pts',(-19.8253802877465,46.3777287926399,-34.9507569611255));
#21095=CARTESIAN_POINT('Ctrl Pts',(-17.3300229730827,47.8884155251851,-34.817329615412));
#21096=CARTESIAN_POINT('Ctrl Pts',(-16.9321744179745,49.455346955759,-34.7365517774293));
#21097=CARTESIAN_POINT('Ctrl Pts',(-16.931281639274,50.0005575828105,-34.7084234471775));
#21098=CARTESIAN_POINT('Ctrl Pts',(-16.9297555423167,50.0020868944766,-35.7915765528225));
#21099=CARTESIAN_POINT('Ctrl Pts',(-16.9274619549591,50.3646558602159,-35.7728476598162));
#21100=CARTESIAN_POINT('Ctrl Pts',(-17.1539338868147,51.7436843363594,-35.7014692590789));
#21101=CARTESIAN_POINT('Ctrl Pts',(-19.1896897083071,53.5347891325428,-35.5774413506109));
#21102=CARTESIAN_POINT('Ctrl Pts',(-22.5168917309592,52.6108605850829,-35.4194928274184));
#21103=CARTESIAN_POINT('Ctrl Pts',(-23.562104568912,49.319744150915,-35.261544304226));
#21104=CARTESIAN_POINT('Ctrl Pts',(-21.3776655307659,46.6453950060402,-35.1035957810335));
#21105=CARTESIAN_POINT('Ctrl Pts',(-17.9722380655997,47.0095593747619,-34.946939863899));
#21106=CARTESIAN_POINT('Ctrl Pts',(-16.9236557307461,49.0130178076084,-34.8429334544954));
#21107=CARTESIAN_POINT('Ctrl Pts',(-16.921610115697,50.0004517332244,-34.7915765528225));
#21108=CARTESIAN_POINT('Origin',(-20.,50.,-42.2084234471774));
#21109=CARTESIAN_POINT('',(-16.9287430323014,49.9975291851057,-36.7915765528226));
#21110=CARTESIAN_POINT('',(-16.9234132972571,50.0020587543361,-36.7084234471775));
#21111=CARTESIAN_POINT('',(-16.9265,50.0000000000002,-42.2084234471774));
#21112=CARTESIAN_POINT('Ctrl Pts',(-16.9234132972571,50.0020587543361,-36.7084234471775));
#21113=CARTESIAN_POINT('Ctrl Pts',(-16.9224088816646,50.13193091024,-36.7016792035325));
#21114=CARTESIAN_POINT('Ctrl Pts',(-16.9886293991394,51.2746295929847,-36.6422854521568));
#21115=CARTESIAN_POINT('Ctrl Pts',(-18.4185250000732,53.263476300571,-36.5302421930502));
#21116=CARTESIAN_POINT('Ctrl Pts',(-21.8681386718888,53.1082790492255,-36.3722936698577));
#21117=CARTESIAN_POINT('Ctrl Pts',(-23.6239678268391,50.1348997169674,-36.2143451466652));
#21118=CARTESIAN_POINT('Ctrl Pts',(-22.09405557116,47.0392109146336,-36.0563966234728));
#21119=CARTESIAN_POINT('Ctrl Pts',(-18.6655268169483,46.6279795274162,-35.8984481002803));
#21120=CARTESIAN_POINT('Ctrl Pts',(-17.036274144185,48.5711523341288,-35.7824570415152));
#21121=CARTESIAN_POINT('Ctrl Pts',(-16.9236808789428,49.7910771093326,-35.7191154904809));
#21122=CARTESIAN_POINT('Ctrl Pts',(-16.9255488571744,49.9973424349028,-35.7084234471775));
#21123=CARTESIAN_POINT('Ctrl Pts',(-16.9287430323014,49.9975291851057,-36.7915765528226));
#21124=CARTESIAN_POINT('Ctrl Pts',(-16.9341064012563,50.6970615449486,-36.7554113728678));
#21125=CARTESIAN_POINT('Ctrl Pts',(-17.5169502765644,52.4230632555672,-36.6665966851821));
#21126=CARTESIAN_POINT('Ctrl Pts',(-20.3740252981191,53.6071376558454,-36.5251324897657));
#21127=CARTESIAN_POINT('Ctrl Pts',(-23.2249079190488,51.6587060907077,-36.3671839665732));
#21128=CARTESIAN_POINT('Ctrl Pts',(-23.1518646084073,48.2063761635784,-36.2092354433808));
#21129=CARTESIAN_POINT('Ctrl Pts',(-20.2211215182128,46.3802704167281,-36.0512869201883));
#21130=CARTESIAN_POINT('Ctrl Pts',(-17.4611824542364,47.6634413886959,-35.9120672900023));
#21131=CARTESIAN_POINT('Ctrl Pts',(-16.9339095461368,49.3454243680967,-35.825497167547));
#21132=CARTESIAN_POINT('Ctrl Pts',(-16.9297555423167,50.0020868944766,-35.7915765528225));
#21133=CARTESIAN_POINT('Origin',(-20.,50.,-42.2084234471774));
#21134=CARTESIAN_POINT('',(-16.9215718601367,50.0003336414566,-37.7915765528225));
#21135=CARTESIAN_POINT('',(-16.9312422659825,50.0006610027018,-37.7084234471775));
#21136=CARTESIAN_POINT('',(-16.9265,50.0000000000002,-42.2084234471774));
#21137=CARTESIAN_POINT('Ctrl Pts',(-16.9312422659825,50.0006610027018,-37.7084234471775));
#21138=CARTESIAN_POINT('Ctrl Pts',(-16.9303317311006,50.4693365215552,-37.6842429165841));
#21139=CARTESIAN_POINT('Ctrl Pts',(-17.250729318919,51.9573027298628,-37.60741287826));
#21140=CARTESIAN_POINT('Ctrl Pts',(-19.5565635760592,53.5992644563693,-37.477933332205));
#21141=CARTESIAN_POINT('Ctrl Pts',(-22.7714374310744,52.3389047405107,-37.3199848090126));
#21142=CARTESIAN_POINT('Ctrl Pts',(-23.4735332609671,48.9579311678064,-37.16203628582));
#21143=CARTESIAN_POINT('Ctrl Pts',(-21.0262821237837,46.5217697438983,-37.0040877626276));
#21144=CARTESIAN_POINT('Ctrl Pts',(-17.7927587355996,47.2085797455779,-36.85288348308));
#21145=CARTESIAN_POINT('Ctrl Pts',(-16.9302499368347,49.1180729542898,-36.7543287112633));
#21146=CARTESIAN_POINT('Ctrl Pts',(-16.9234132972571,50.0020587543361,-36.7084234471775));
#21147=CARTESIAN_POINT('Ctrl Pts',(-16.9215718601367,50.0003336414566,-37.7915765528225));
#21148=CARTESIAN_POINT('Ctrl Pts',(-16.921543415412,50.0186362548428,-37.7906245936502));
#21149=CARTESIAN_POINT('Ctrl Pts',(-16.9299478707484,51.0491651072969,-37.737023126747));
#21150=CARTESIAN_POINT('Ctrl Pts',(-18.0723368961882,53.0717177485,-37.630772152113));
#21151=CARTESIAN_POINT('Ctrl Pts',(-21.5183204151355,53.2933327434377,-37.4728236289205));
#21152=CARTESIAN_POINT('Ctrl Pts',(-23.5876893022666,50.5289827072374,-37.314875105728));
#21153=CARTESIAN_POINT('Ctrl Pts',(-22.4042092574597,47.2850203370204,-37.1569265825356));
#21154=CARTESIAN_POINT('Ctrl Pts',(-19.0409058781059,46.5026473552099,-36.9989780593431));
#21155=CARTESIAN_POINT('Ctrl Pts',(-17.1181668122877,48.3443111845633,-36.8771947161054));
#21156=CARTESIAN_POINT('Ctrl Pts',(-16.9262983733243,49.6786777173678,-36.8080608805986));
#21157=CARTESIAN_POINT('Ctrl Pts',(-16.9287430323014,49.9975291851057,-36.7915765528226));
#21158=CARTESIAN_POINT('Origin',(-20.,50.,-42.2084234471774));
#21159=CARTESIAN_POINT('',(-16.9296185387977,50.0021495995983,-38.7915765528225));
#21160=CARTESIAN_POINT('',(-16.9257449470869,49.9973154802779,-38.7084234471774));
#21161=CARTESIAN_POINT('',(-16.9265,50.0000000000002,-42.2084234471774));
#21162=CARTESIAN_POINT('Ctrl Pts',(-16.9257449470869,49.9973154802779,-38.7084234471774));
#21163=CARTESIAN_POINT('Ctrl Pts',(-16.9330319322419,50.8002972396456,-38.6668066296357));
#21164=CARTESIAN_POINT('Ctrl Pts',(-17.6644029527493,52.6309011816754,-38.5725403043632));
#21165=CARTESIAN_POINT('Ctrl Pts',(-20.7420733238179,53.5497397950539,-38.4256244713598));
#21166=CARTESIAN_POINT('Ctrl Pts',(-23.3780464773465,51.3191456129741,-38.2676759481674));
#21167=CARTESIAN_POINT('Ctrl Pts',(-22.951247888663,47.8925182840191,-38.1097274249748));
#21168=CARTESIAN_POINT('Ctrl Pts',(-19.8486424668251,46.3766825092365,-37.9517789017824));
#21169=CARTESIAN_POINT('Ctrl Pts',(-17.3372410903829,47.8751309362902,-37.8180109091832));
#21170=CARTESIAN_POINT('Ctrl Pts',(-16.9323142853343,49.4488653098967,-37.736892424315));
#21171=CARTESIAN_POINT('Ctrl Pts',(-16.9312422659825,50.0006610027018,-37.7084234471775));
#21172=CARTESIAN_POINT('Ctrl Pts',(-16.9296185387977,50.0021495995983,-38.7915765528225));
#21173=CARTESIAN_POINT('Ctrl Pts',(-16.9272827753867,50.3580876058963,-38.7731883067018));
#21174=CARTESIAN_POINT('Ctrl Pts',(-17.1483415218904,51.7303472358439,-38.7021505528502));
#21175=CARTESIAN_POINT('Ctrl Pts',(-19.167020277377,53.5294996249073,-38.5784632912678));
#21176=CARTESIAN_POINT('Ctrl Pts',(-22.5000701187915,52.6269745712345,-38.4205147680753));
#21177=CARTESIAN_POINT('Ctrl Pts',(-23.5664017687871,49.3426270004872,-38.2625662448828));
#21178=CARTESIAN_POINT('Ctrl Pts',(-21.3991756821973,46.6543118776375,-38.1046177216904));
#21179=CARTESIAN_POINT('Ctrl Pts',(-17.9840721502399,46.9973442210765,-37.9476211576703));
#21180=CARTESIAN_POINT('Ctrl Pts',(-16.9231165929177,49.0063831951071,-37.843274101381));
#21181=CARTESIAN_POINT('Ctrl Pts',(-16.9215718601367,50.0003336414566,-37.7915765528225));
#21182=CARTESIAN_POINT('Origin',(-20.,50.,-42.2084234471774));
#21183=CARTESIAN_POINT('',(-16.9296933173407,49.9966552073599,-39.7915765528226));
#21184=CARTESIAN_POINT('',(-16.9232550353076,50.0019104925463,-39.7084234471775));
#21185=CARTESIAN_POINT('',(-16.9265,50.0000000000002,-42.2084234471774));
#21186=CARTESIAN_POINT('',(-19.2062007174672,47.0307770462543,-40.));
#21187=CARTESIAN_POINT('Ctrl Pts',(-19.2062007174672,47.0307770462543,-40.));
#21188=CARTESIAN_POINT('Ctrl Pts',(-18.2239621276955,47.2933710986319,-39.9473504922692));
#21189=CARTESIAN_POINT('Ctrl Pts',(-17.1241890235734,48.3306038970069,-39.8778760098767));
#21190=CARTESIAN_POINT('Ctrl Pts',(-16.9273405012997,49.6711319064253,-39.8084015274842));
#21191=CARTESIAN_POINT('Ctrl Pts',(-16.9296933173407,49.9966552073599,-39.7915765528225));
#21192=CARTESIAN_POINT('',(-20.7956623919264,47.025713650831,-40.));
#21193=CARTESIAN_POINT('Origin',(-20.,50.,-40.));
#21194=CARTESIAN_POINT('Ctrl Pts',(-20.7956662771739,47.0257030918457,-40.));
#21195=CARTESIAN_POINT('Ctrl Pts',(-19.8486505232287,46.7747747443585,-39.9490537266973));
#21196=CARTESIAN_POINT('Ctrl Pts',(-17.7883283635535,47.2298889349752,-39.8518615424232));
#21197=CARTESIAN_POINT('Ctrl Pts',(-16.929936238593,49.1116774471724,-39.754669358149));
#21198=CARTESIAN_POINT('Ctrl Pts',(-16.9232550353076,50.0019104925463,-39.7084234471775));
#21199=CARTESIAN_POINT('Origin',(-20.,-50.,-32.));
#21200=CARTESIAN_POINT('',(-17.4865385565584,-49.9997270833425,-25.387416697508));
#21201=CARTESIAN_POINT('',(-17.4842343961705,-50.0033815919295,-25.112583302492));
#21202=CARTESIAN_POINT('',(-17.4825,-50.,-32.));
#21203=CARTESIAN_POINT('',(-18.0865340033349,-48.3640127966251,-25.));
#21204=CARTESIAN_POINT('Ctrl Pts',(-17.4842343961705,-50.0033815919295,
-25.112583302492));
#21205=CARTESIAN_POINT('Ctrl Pts',(-17.4894446223952,-49.4108204662451,
-25.0750555349947));
#21206=CARTESIAN_POINT('Ctrl Pts',(-17.7007781719159,-48.8151964396956,
-25.0375277674973));
#21207=CARTESIAN_POINT('Ctrl Pts',(-18.0865340033349,-48.3640127966251,
-25.));
#21208=CARTESIAN_POINT('',(-17.4825,-50.,-25.));
#21209=CARTESIAN_POINT('Origin',(-20.,-50.,-25.));
#21210=CARTESIAN_POINT('',(-17.4825,-50.,-24.));
#21211=CARTESIAN_POINT('',(-17.4825,-50.,-32.));
#21212=CARTESIAN_POINT('Origin',(-20.,-50.,-24.));
#21213=CARTESIAN_POINT('',(-21.9170728295299,-48.3614592401522,-25.));
#21214=CARTESIAN_POINT('Origin',(-20.,-50.,-25.));
#21215=CARTESIAN_POINT('Ctrl Pts',(-21.9170803467229,-48.3614539181488,
-25.));
#21216=CARTESIAN_POINT('Ctrl Pts',(-21.3942485321037,-47.7526835964708,
-25.0509462733027));
#21217=CARTESIAN_POINT('Ctrl Pts',(-20.5545526893521,-47.4126377534433,
-25.1018925466053));
#21218=CARTESIAN_POINT('Ctrl Pts',(-19.7559044819232,-47.4904264940795,
-25.152838819908));
#21219=CARTESIAN_POINT('Ctrl Pts',(-18.9305558892707,-47.5708158657842,
-25.2054883276388));
#21220=CARTESIAN_POINT('Ctrl Pts',(-18.1490454176151,-48.0974449024861,
-25.2581378353696));
#21221=CARTESIAN_POINT('Ctrl Pts',(-17.7651665339121,-48.8322009233391,
-25.3107873431004));
#21222=CARTESIAN_POINT('Ctrl Pts',(-17.5789261662639,-49.1886707300015,
-25.3363304612363));
#21223=CARTESIAN_POINT('Ctrl Pts',(-17.4862780881908,-49.5941282970916,
-25.3618735793722));
#21224=CARTESIAN_POINT('Ctrl Pts',(-17.4865385565584,-49.9997270833425,
-25.387416697508));
#21225=CARTESIAN_POINT('Origin',(-20.,-50.,-32.));
#21226=CARTESIAN_POINT('',(-17.4812439922137,-50.0020955261299,-26.387416697508));
#21227=CARTESIAN_POINT('',(-17.478641074515,-49.9993296596843,-26.112583302492));
#21228=CARTESIAN_POINT('',(-17.4825,-50.,-32.));
#21229=CARTESIAN_POINT('Ctrl Pts',(-17.478641074515,-49.9993296596843,-26.112583302492));
#21230=CARTESIAN_POINT('Ctrl Pts',(-17.4785132796901,-49.9628733193853,
-26.1102687557771));
#21231=CARTESIAN_POINT('Ctrl Pts',(-17.4792362609288,-49.9264222331827,
-26.1079542090622));
#21232=CARTESIAN_POINT('Ctrl Pts',(-17.4808258970162,-49.8900090632248,
-26.1056396623473));
#21233=CARTESIAN_POINT('Ctrl Pts',(-17.516985701843,-49.0617106059675,-26.0529901546164));
#21234=CARTESIAN_POINT('Ctrl Pts',(-18.0015840153798,-48.2530313826314,
-26.0003406468856));
#21235=CARTESIAN_POINT('Ctrl Pts',(-18.7149420635586,-47.8304732403596,
-25.9476911391548));
#21236=CARTESIAN_POINT('Ctrl Pts',(-19.4283001117373,-47.4079150980878,
-25.895041631424));
#21237=CARTESIAN_POINT('Ctrl Pts',(-20.3704178945579,-47.3714780368803,
-25.8423921236932));
#21238=CARTESIAN_POINT('Ctrl Pts',(-21.1141877060749,-47.7378804619289,
-25.7897426159623));
#21239=CARTESIAN_POINT('Ctrl Pts',(-21.8579575175919,-48.1042828869776,
-25.7370931082315));
#21240=CARTESIAN_POINT('Ctrl Pts',(-22.4033793578053,-48.8735247982823,
-25.6844436005007));
#21241=CARTESIAN_POINT('Ctrl Pts',(-22.5032201961104,-49.6964833362074,
-25.6317940927699));
#21242=CARTESIAN_POINT('Ctrl Pts',(-22.6030610344155,-50.5194418741325,
-25.5791445850391));
#21243=CARTESIAN_POINT('Ctrl Pts',(-22.2573208708123,-51.396117038678,-25.5264950773082));
#21244=CARTESIAN_POINT('Ctrl Pts',(-21.6226857101616,-51.9298779026354,
-25.4738455695774));
#21245=CARTESIAN_POINT('Ctrl Pts',(-20.988050549511,-52.4636387665928,-25.4211960618466));
#21246=CARTESIAN_POINT('Ctrl Pts',(-20.0645203918128,-52.654485329962,-25.3685465541158));
#21247=CARTESIAN_POINT('Ctrl Pts',(-19.2708512338734,-52.4142812621293,
-25.3158970463849));
#21248=CARTESIAN_POINT('Ctrl Pts',(-18.477182075934,-52.1740771942966,-25.2632475386541));
#21249=CARTESIAN_POINT('Ctrl Pts',(-17.8133739177533,-51.5028224952619,
-25.2105980309233));
#21250=CARTESIAN_POINT('Ctrl Pts',(-17.5804130530232,-50.7085531973994,
-25.1579485231925));
#21251=CARTESIAN_POINT('Ctrl Pts',(-17.5135031457353,-50.4804269619344,
-25.142826782959));
#21252=CARTESIAN_POINT('Ctrl Pts',(-17.4821349457426,-50.2421529341285,
-25.1277050427255));
#21253=CARTESIAN_POINT('Ctrl Pts',(-17.4842343961705,-50.0033815919295,
-25.112583302492));
#21254=CARTESIAN_POINT('Ctrl Pts',(-17.4865385565584,-49.9997270833425,
-25.387416697508));
#21255=CARTESIAN_POINT('Ctrl Pts',(-17.4868149659228,-50.4301490334305,
-25.414523087103));
#21256=CARTESIAN_POINT('Ctrl Pts',(-17.5917201630912,-50.8607300172153,
-25.4416294766979));
#21257=CARTESIAN_POINT('Ctrl Pts',(-17.800437027254,-51.2330950056298,-25.4687358662929));
#21258=CARTESIAN_POINT('Ctrl Pts',(-18.2058337000493,-51.9563500620634,
-25.5213853740237));
#21259=CARTESIAN_POINT('Ctrl Pts',(-19.0028743413902,-52.4599771699264,
-25.5740348817546));
#21260=CARTESIAN_POINT('Ctrl Pts',(-19.8301086932262,-52.5158218568911,
-25.6266843894854));
#21261=CARTESIAN_POINT('Ctrl Pts',(-20.6573430450623,-52.5716665438558,
-25.6793338972162));
#21262=CARTESIAN_POINT('Ctrl Pts',(-21.5147711073935,-52.1797288099222,
-25.731983404947));
#21263=CARTESIAN_POINT('Ctrl Pts',(-22.0137531835634,-51.5176087150676,
-25.7846329126778));
#21264=CARTESIAN_POINT('Ctrl Pts',(-22.5127352597332,-50.855488620213,-25.8372824204087));
#21265=CARTESIAN_POINT('Ctrl Pts',(-22.6532713497417,-49.9231861644375,
-25.8899319281395));
#21266=CARTESIAN_POINT('Ctrl Pts',(-22.3716202770373,-49.1433861401557,
-25.9425814358703));
#21267=CARTESIAN_POINT('Ctrl Pts',(-22.0899692043328,-48.3635861158738,
-25.9952309436012));
#21268=CARTESIAN_POINT('Ctrl Pts',(-21.3861309689154,-47.7362885230857,
-26.0478804513319));
#21269=CARTESIAN_POINT('Ctrl Pts',(-20.5791956401472,-47.5458492720573,
-26.1005299590628));
#21270=CARTESIAN_POINT('Ctrl Pts',(-19.7722603113789,-47.355410021029,-26.1531794667936));
#21271=CARTESIAN_POINT('Ctrl Pts',(-18.8622278892599,-47.6018291117603,
-26.2058289745244));
#21272=CARTESIAN_POINT('Ctrl Pts',(-18.2616398443447,-48.1734061983061,
-26.2584784822553));
#21273=CARTESIAN_POINT('Ctrl Pts',(-17.7713614356055,-48.6400020735255,
-26.3014578873395));
#21274=CARTESIAN_POINT('Ctrl Pts',(-17.4872954214302,-49.3232818307864,
-26.3444372924238));
#21275=CARTESIAN_POINT('Ctrl Pts',(-17.4812439922137,-50.0020955261299,
-26.387416697508));
#21276=CARTESIAN_POINT('Origin',(-20.,-50.,-32.));
#21277=CARTESIAN_POINT('',(-17.4803938764511,-49.9981422851833,-27.387416697508));
#21278=CARTESIAN_POINT('',(-17.4854882815929,-49.9984719969074,-27.112583302492));
#21279=CARTESIAN_POINT('',(-17.4825,-50.,-32.));
#21280=CARTESIAN_POINT('Ctrl Pts',(-17.4854882815929,-49.9984719969074,
-27.112583302492));
#21281=CARTESIAN_POINT('Ctrl Pts',(-17.4837320581771,-49.6851867695493,
-27.0928324688287));
#21282=CARTESIAN_POINT('Ctrl Pts',(-17.5380281914022,-49.372488365388,-27.0730816351654));
#21283=CARTESIAN_POINT('Ctrl Pts',(-17.6511655615397,-49.0827678639941,
-27.0533308015021));
#21284=CARTESIAN_POINT('Ctrl Pts',(-17.9527541904173,-48.3104641709981,
-27.0006812937713));
#21285=CARTESIAN_POINT('Ctrl Pts',(-18.6724614894036,-47.7014386592764,
-26.9480317860404));
#21286=CARTESIAN_POINT('Ctrl Pts',(-19.4840192035288,-47.5317821658037,
-26.8953822783096));
#21287=CARTESIAN_POINT('Ctrl Pts',(-20.295576917654,-47.362125672331,-26.8427327705788));
#21288=CARTESIAN_POINT('Ctrl Pts',(-21.1989850469181,-47.6318381971073,
-26.790083262848));
#21289=CARTESIAN_POINT('Ctrl Pts',(-21.7846970457346,-48.2186528878745,
-26.7374337551172));
#21290=CARTESIAN_POINT('Ctrl Pts',(-22.3704090445512,-48.8054675786417,
-26.6847842473863));
#21291=CARTESIAN_POINT('Ctrl Pts',(-22.6384249129202,-49.7093844353998,
-26.6321347396555));
#21292=CARTESIAN_POINT('Ctrl Pts',(-22.4672441468777,-50.5206200888683,
-26.5794852319247));
#21293=CARTESIAN_POINT('Ctrl Pts',(-22.2960633808352,-51.3318557423367,
-26.5268357241939));
#21294=CARTESIAN_POINT('Ctrl Pts',(-21.6856859803813,-52.0504101925156,
-26.474186216463));
#21295=CARTESIAN_POINT('Ctrl Pts',(-20.9128164334925,-52.3505504609625,
-26.4215367087322));
#21296=CARTESIAN_POINT('Ctrl Pts',(-20.1399468866037,-52.6506907294095,
-26.3688872010014));
#21297=CARTESIAN_POINT('Ctrl Pts',(-19.2045851932801,-52.5324168161245,
-26.3162376932706));
#21298=CARTESIAN_POINT('Ctrl Pts',(-18.5307649946765,-52.0493210138927,
-26.2635881855398));
#21299=CARTESIAN_POINT('Ctrl Pts',(-17.8865668836162,-51.5874627853863,
-26.2132532245238));
#21300=CARTESIAN_POINT('Ctrl Pts',(-17.4814202569298,-50.7921537819725,
-26.1629182635079));
#21301=CARTESIAN_POINT('Ctrl Pts',(-17.478641074515,-49.9993296596843,-26.112583302492));
#21302=CARTESIAN_POINT('Ctrl Pts',(-17.4812439922137,-50.0020955261299,
-26.387416697508));
#21303=CARTESIAN_POINT('Ctrl Pts',(-17.4798824577399,-50.154824445923,-26.3970868001546));
#21304=CARTESIAN_POINT('Ctrl Pts',(-17.4925946446391,-50.3073272836526,
-26.4067569028011));
#21305=CARTESIAN_POINT('Ctrl Pts',(-17.5201983578819,-50.4570852091481,
-26.4164270054477));
#21306=CARTESIAN_POINT('Ctrl Pts',(-17.6704885840456,-51.2724520510841,
-26.4690765131785));
#21307=CARTESIAN_POINT('Ctrl Pts',(-18.2622127040842,-52.0064506525957,
-26.5217260209094));
#21308=CARTESIAN_POINT('Ctrl Pts',(-19.0271195964254,-52.3263364322528,
-26.5743755286402));
#21309=CARTESIAN_POINT('Ctrl Pts',(-19.7920264887666,-52.6462222119098,
-26.627025036371));
#21310=CARTESIAN_POINT('Ctrl Pts',(-20.7301161534105,-52.5519951697124,
-26.6796745441018));
#21311=CARTESIAN_POINT('Ctrl Pts',(-21.4161209056844,-52.08637043532,-26.7323240518326));
#21312=CARTESIAN_POINT('Ctrl Pts',(-22.1021256579584,-51.6207457009276,
-26.7849735595635));
#21313=CARTESIAN_POINT('Ctrl Pts',(-22.5360454978625,-50.7837232743402,
-26.8376230672943));
#21314=CARTESIAN_POINT('Ctrl Pts',(-22.5211689625615,-49.9547551805518,
-26.8902725750251));
#21315=CARTESIAN_POINT('Ctrl Pts',(-22.5062924272606,-49.1257870867634,
-26.942922082756));
#21316=CARTESIAN_POINT('Ctrl Pts',(-22.0426195167546,-48.3048733257741,
-26.9955715904868));
#21317=CARTESIAN_POINT('Ctrl Pts',(-21.3403495461317,-47.8641623480534,
-27.0482210982176));
#21318=CARTESIAN_POINT('Ctrl Pts',(-20.6380795755089,-47.4234513703327,
-27.1008706059484));
#21319=CARTESIAN_POINT('Ctrl Pts',(-19.697212544769,-47.3629431758806,-27.1535201136792));
#21320=CARTESIAN_POINT('Ctrl Pts',(-18.9442760880979,-47.7100683950257,
-27.2061696214101));
#21321=CARTESIAN_POINT('Ctrl Pts',(-18.1913396314267,-48.0571936141707,
-27.2588191291409));
#21322=CARTESIAN_POINT('Ctrl Pts',(-17.6263337488242,-48.811952246913,-27.3114686368717));
#21323=CARTESIAN_POINT('Ctrl Pts',(-17.5053953288183,-49.632185863958,-27.3641181446025));
#21324=CARTESIAN_POINT('Ctrl Pts',(-17.4875560345985,-49.7531762723222,
-27.3718843289044));
#21325=CARTESIAN_POINT('Ctrl Pts',(-17.4793789333885,-49.875591310926,-27.3796505132062));
#21326=CARTESIAN_POINT('Ctrl Pts',(-17.4803938764511,-49.9981422851833,
-27.387416697508));
#21327=CARTESIAN_POINT('Origin',(-20.,-50.,-32.));
#21328=CARTESIAN_POINT('',(-17.4864646543277,-49.9997146182113,-28.387416697508));
#21329=CARTESIAN_POINT('',(-17.4839129917625,-50.00212360321,-28.112583302492));
#21330=CARTESIAN_POINT('',(-17.4825,-50.,-32.));
#21331=CARTESIAN_POINT('Ctrl Pts',(-17.4839129917625,-50.00212360321,-28.112583302492));
#21332=CARTESIAN_POINT('Ctrl Pts',(-17.4887123626501,-49.4131980331168,
-28.0753961818803));
#21333=CARTESIAN_POINT('Ctrl Pts',(-17.6952668319888,-48.8212389436082,
-28.0382090612686));
#21334=CARTESIAN_POINT('Ctrl Pts',(-18.0729549967146,-48.3737050608961,
-28.0010219406569));
#21335=CARTESIAN_POINT('Ctrl Pts',(-18.6076857212633,-47.7400868019379,
-27.9483724329261));
#21336=CARTESIAN_POINT('Ctrl Pts',(-19.4854519355195,-47.3959671798642,
-27.8957229251952));
#21337=CARTESIAN_POINT('Ctrl Pts',(-20.3083316759583,-47.4973475663696,
-27.8430734174644));
#21338=CARTESIAN_POINT('Ctrl Pts',(-21.131211416397,-47.598727952875,-27.7904239097336));
#21339=CARTESIAN_POINT('Ctrl Pts',(-21.8992046830182,-48.1456083479595,
-27.7377744020028));
#21340=CARTESIAN_POINT('Ctrl Pts',(-22.2641534037816,-48.8900688925903,
-27.685124894272));
#21341=CARTESIAN_POINT('Ctrl Pts',(-22.629102124545,-49.6345294372211,-27.6324753865412));
#21342=CARTESIAN_POINT('Ctrl Pts',(-22.5910062994507,-50.5765701313981,
-27.5798258788103));
#21343=CARTESIAN_POINT('Ctrl Pts',(-22.1671360981513,-51.2891310488058,
-27.5271763710795));
#21344=CARTESIAN_POINT('Ctrl Pts',(-21.743265896852,-52.0016919662134,-27.4745268633487));
#21345=CARTESIAN_POINT('Ctrl Pts',(-20.9336213193477,-52.4847731068517,
-27.4218773556179));
#21346=CARTESIAN_POINT('Ctrl Pts',(-20.1052424094757,-52.5193771868443,
-27.369227847887));
#21347=CARTESIAN_POINT('Ctrl Pts',(-19.2768634996038,-52.5539812668369,
-27.3165783401562));
#21348=CARTESIAN_POINT('Ctrl Pts',(-18.4297502573642,-52.1401082861839,
-27.2639288324254));
#21349=CARTESIAN_POINT('Ctrl Pts',(-17.9479286156288,-51.4653808587222,
-27.2112793246945));
#21350=CARTESIAN_POINT('Ctrl Pts',(-17.646856605019,-51.0437693626761,-27.178380650627));
#21351=CARTESIAN_POINT('Ctrl Pts',(-17.4884135971887,-50.5203066070677,
-27.1454819765595));
#21352=CARTESIAN_POINT('Ctrl Pts',(-17.4854882815929,-49.9984719969074,
-27.112583302492));
#21353=CARTESIAN_POINT('Ctrl Pts',(-17.4803938764511,-49.9981422851833,
-27.387416697508));
#21354=CARTESIAN_POINT('Ctrl Pts',(-17.4862595649243,-50.7064045154313,
-27.432300020937));
#21355=CARTESIAN_POINT('Ctrl Pts',(-17.7991453021895,-51.4192070818358,
-27.477183344366));
#21356=CARTESIAN_POINT('Ctrl Pts',(-18.3282967869582,-51.887789182872,-27.522066667795));
#21357=CARTESIAN_POINT('Ctrl Pts',(-18.9490076225134,-52.4374502833933,
-27.5747161755258));
#21358=CARTESIAN_POINT('Ctrl Pts',(-19.8673002510331,-52.6510638830879,
-27.6273656832566));
#21359=CARTESIAN_POINT('Ctrl Pts',(-20.6668806897214,-52.4317914845825,
-27.6800151909875));
#21360=CARTESIAN_POINT('Ctrl Pts',(-21.4664611284097,-52.2125190860771,
-27.7326646987183));
#21361=CARTESIAN_POINT('Ctrl Pts',(-22.1473293772665,-51.5603606893716,
-27.7853142064491));
#21362=CARTESIAN_POINT('Ctrl Pts',(-22.4008241614529,-50.7709623965743,
-27.8379637141799));
#21363=CARTESIAN_POINT('Ctrl Pts',(-22.6543189456393,-49.981564103777,-27.8906132219107));
#21364=CARTESIAN_POINT('Ctrl Pts',(-22.4804402651553,-49.0549259148879,
-27.9432627296416));
#21365=CARTESIAN_POINT('Ctrl Pts',(-21.9580133797035,-48.4111251564977,
-27.9959122373724));
#21366=CARTESIAN_POINT('Ctrl Pts',(-21.4355864942518,-47.7673243981074,
-28.0485617451032));
#21367=CARTESIAN_POINT('Ctrl Pts',(-20.5646114038323,-47.4063610702159,
-28.1012112528341));
#21368=CARTESIAN_POINT('Ctrl Pts',(-19.7399314188999,-47.4918724109971,
-28.1538607605649));
#21369=CARTESIAN_POINT('Ctrl Pts',(-18.9152514339676,-47.5773837517783,
-28.2065102682957));
#21370=CARTESIAN_POINT('Ctrl Pts',(-18.1368665545222,-48.1093697612321,
-28.2591597760265));
#21371=CARTESIAN_POINT('Ctrl Pts',(-17.757645729928,-48.8466626704905,-28.3118092837573));
#21372=CARTESIAN_POINT('Ctrl Pts',(-17.576118829844,-49.1995929095268,-28.3370117550076));
#21373=CARTESIAN_POINT('Ctrl Pts',(-17.4860556899587,-49.5995668160042,
-28.3622142262578));
#21374=CARTESIAN_POINT('Ctrl Pts',(-17.4864646543277,-49.9997146182113,
-28.387416697508));
#21375=CARTESIAN_POINT('Origin',(-20.,-50.,-32.));
#21376=CARTESIAN_POINT('',(-17.4814020660648,-50.0021261701134,-29.387416697508));
#21377=CARTESIAN_POINT('',(-17.4785834014225,-49.9994390864922,-29.112583302492));
#21378=CARTESIAN_POINT('',(-17.4825,-50.,-32.));
#21379=CARTESIAN_POINT('Ctrl Pts',(-17.4785834014225,-49.9994390864922,
-29.112583302492));
#21380=CARTESIAN_POINT('Ctrl Pts',(-17.4784886794343,-49.968349744285,-29.1106094026627));
#21381=CARTESIAN_POINT('Ctrl Pts',(-17.4790144707734,-49.9372636795263,
-29.1086355028335));
#21382=CARTESIAN_POINT('Ctrl Pts',(-17.4801707545743,-49.906201084417,-29.1066616030042));
#21383=CARTESIAN_POINT('Ctrl Pts',(-17.5110121235283,-49.0776735588066,
-29.0540120952734));
#21384=CARTESIAN_POINT('Ctrl Pts',(-17.9904111854216,-48.2658432856158,
-29.0013625875425));
#21385=CARTESIAN_POINT('Ctrl Pts',(-18.7010396656628,-47.8387411740548,
-28.9487130798117));
#21386=CARTESIAN_POINT('Ctrl Pts',(-19.411668145904,-47.4116390624939,-28.8960635720809));
#21387=CARTESIAN_POINT('Ctrl Pts',(-20.3535260444932,-47.3692651125628,
-28.8434140643501));
#21388=CARTESIAN_POINT('Ctrl Pts',(-21.0996364057885,-47.730828909672,-28.7907645566192));
#21389=CARTESIAN_POINT('Ctrl Pts',(-21.8457467670838,-48.0923927067812,
-28.7381150488884));
#21390=CARTESIAN_POINT('Ctrl Pts',(-22.3961095910853,-48.8578942509305,
-28.6854655411576));
#21391=CARTESIAN_POINT('Ctrl Pts',(-22.5012262607424,-49.680305058751,-28.6328160334268));
#21392=CARTESIAN_POINT('Ctrl Pts',(-22.6063429303995,-50.5027158665715,
-28.580166525696));
#21393=CARTESIAN_POINT('Ctrl Pts',(-22.2662134457122,-51.3820359380631,
-28.5275170179651));
#21394=CARTESIAN_POINT('Ctrl Pts',(-21.6350303363852,-51.9196388888135,
-28.4748675102343));
#21395=CARTESIAN_POINT('Ctrl Pts',(-21.0038472270583,-52.457241839564,-28.4222180025035));
#21396=CARTESIAN_POINT('Ctrl Pts',(-20.0816104930917,-52.6531276695732,
-28.3695684947727));
#21397=CARTESIAN_POINT('Ctrl Pts',(-19.2864021333348,-52.4184945199041,
-28.3169189870418));
#21398=CARTESIAN_POINT('Ctrl Pts',(-18.491193773578,-52.183861370235,-28.264269479311));
#21399=CARTESIAN_POINT('Ctrl Pts',(-17.8230137880308,-51.5187092408875,
-28.2116199715802));
#21400=CARTESIAN_POINT('Ctrl Pts',(-17.5847714126778,-50.7245747282924,
-28.1589704638494));
#21401=CARTESIAN_POINT('Ctrl Pts',(-17.5148031262748,-50.4913490859714,
-28.1435080767302));
#21402=CARTESIAN_POINT('Ctrl Pts',(-17.4819174156229,-50.2469985760325,
-28.1280456896111));
#21403=CARTESIAN_POINT('Ctrl Pts',(-17.4839129917625,-50.00212360321,-28.112583302492));
#21404=CARTESIAN_POINT('Ctrl Pts',(-17.4864646543277,-49.9997146182113,
-28.387416697508));
#21405=CARTESIAN_POINT('Ctrl Pts',(-17.4869100416013,-50.4355001098706,
-28.4148637339886));
#21406=CARTESIAN_POINT('Ctrl Pts',(-17.5946602795742,-50.871491851351,-28.4423107704692));
#21407=CARTESIAN_POINT('Ctrl Pts',(-17.808434460022,-51.2471488088293,-28.4697578069498));
#21408=CARTESIAN_POINT('Ctrl Pts',(-18.2185007844534,-51.9677422288466,
-28.5224073146806));
#21409=CARTESIAN_POINT('Ctrl Pts',(-19.0186902030594,-52.4663292598182,
-28.5750568224114));
#21410=CARTESIAN_POINT('Ctrl Pts',(-19.846249011503,-52.5168830528463,-28.6277063301423));
#21411=CARTESIAN_POINT('Ctrl Pts',(-20.6738078199465,-52.5674368458744,
-28.6803558378731));
#21412=CARTESIAN_POINT('Ctrl Pts',(-21.5287360182276,-52.169957400959,-28.7330053456039));
#21413=CARTESIAN_POINT('Ctrl Pts',(-22.023464908259,-51.5046359802209,-28.7856548533348));
#21414=CARTESIAN_POINT('Ctrl Pts',(-22.5181937982904,-50.8393145594829,
-28.8383043610656));
#21415=CARTESIAN_POINT('Ctrl Pts',(-22.6527233800722,-49.9061511629222,
-28.8909538687964));
#21416=CARTESIAN_POINT('Ctrl Pts',(-22.3660667135347,-49.1281812258465,
-28.9436033765272));
#21417=CARTESIAN_POINT('Ctrl Pts',(-22.0794100469972,-48.3502112887709,
-28.996252884258));
#21418=CARTESIAN_POINT('Ctrl Pts',(-21.3715671321404,-47.7274348111802,
-29.0489023919889));
#21419=CARTESIAN_POINT('Ctrl Pts',(-20.5634277903475,-47.5421780387863,
-29.1015518997197));
#21420=CARTESIAN_POINT('Ctrl Pts',(-19.7552884485545,-47.3569212663924,
-29.1542014074505));
#21421=CARTESIAN_POINT('Ctrl Pts',(-18.8468526798254,-47.6091841991953,
-29.2068509151813));
#21422=CARTESIAN_POINT('Ctrl Pts',(-18.2499460255173,-48.1846072727033,
-29.2595004229121));
#21423=CARTESIAN_POINT('Ctrl Pts',(-17.7665348865127,-48.6506197075898,
-29.3021391811108));
#21424=CARTESIAN_POINT('Ctrl Pts',(-17.4874476178656,-49.3285845014614,
-29.3447779393094));
#21425=CARTESIAN_POINT('Ctrl Pts',(-17.4814020660648,-50.0021261701134,
-29.387416697508));
#21426=CARTESIAN_POINT('Origin',(-20.,-50.,-32.));
#21427=CARTESIAN_POINT('',(-17.4802499007281,-49.9981961378425,-30.387416697508));
#21428=CARTESIAN_POINT('',(-17.4853853786729,-49.9984092958285,-30.112583302492));
#21429=CARTESIAN_POINT('',(-17.4825,-50.,-32.));
#21430=CARTESIAN_POINT('Ctrl Pts',(-17.4853853786729,-49.9984092958285,
-30.112583302492));
#21431=CARTESIAN_POINT('Ctrl Pts',(-17.4835836611168,-49.6905590780416,
-30.0931731157143));
#21432=CARTESIAN_POINT('Ctrl Pts',(-17.5359688547378,-49.3833006303856,
-30.0737629289367));
#21433=CARTESIAN_POINT('Ctrl Pts',(-17.6453244230335,-49.0978688621381,
-30.054352742159));
#21434=CARTESIAN_POINT('Ctrl Pts',(-17.9419478870084,-48.3236443654287,
-30.0017032344282));
#21435=CARTESIAN_POINT('Ctrl Pts',(-18.657729850048,-47.7100092668519,-29.9490537266973));
#21436=CARTESIAN_POINT('Ctrl Pts',(-19.4681814439702,-47.5351457069169,
-29.8964042189665));
#21437=CARTESIAN_POINT('Ctrl Pts',(-20.2786330378925,-47.3602821469818,
-29.8437547112357));
#21438=CARTESIAN_POINT('Ctrl Pts',(-21.1837542626973,-47.6241901256886,
-29.7911052035049));
#21439=CARTESIAN_POINT('Ctrl Pts',(-21.7732221751288,-48.2072309740829,
-29.7384556957741));
#21440=CARTESIAN_POINT('Ctrl Pts',(-22.3626900875602,-48.7902718224772,
-29.6858061880432));
#21441=CARTESIAN_POINT('Ctrl Pts',(-22.6365046876183,-49.6924455405591,
-29.6331566803124));
#21442=CARTESIAN_POINT('Ctrl Pts',(-22.470536290213,-50.5047653924361,-29.5805071725816));
#21443=CARTESIAN_POINT('Ctrl Pts',(-22.3045678928078,-51.317085244313,-29.5278576648508));
#21444=CARTESIAN_POINT('Ctrl Pts',(-21.6988164979394,-52.0395512299852,
-29.4752081571199));
#21445=CARTESIAN_POINT('Ctrl Pts',(-20.9278902889251,-52.3446443812263,
-29.4225586493891));
#21446=CARTESIAN_POINT('Ctrl Pts',(-20.1569640799107,-52.6497375324674,
-29.3699091416583));
#21447=CARTESIAN_POINT('Ctrl Pts',(-19.2208630567505,-52.5374578492774,
-29.3172596339275));
#21448=CARTESIAN_POINT('Ctrl Pts',(-18.5439543831779,-52.0587056186674,
-29.2646101261966));
#21449=CARTESIAN_POINT('Ctrl Pts',(-17.892423912988,-51.5979024437465,-29.2139345182951));
#21450=CARTESIAN_POINT('Ctrl Pts',(-17.481015183552,-50.7975906908716,-29.1632589103935));
#21451=CARTESIAN_POINT('Ctrl Pts',(-17.4785834014225,-49.9994390864922,
-29.112583302492));
#21452=CARTESIAN_POINT('Ctrl Pts',(-17.4814020660648,-50.0021261701134,
-29.387416697508));
#21453=CARTESIAN_POINT('Ctrl Pts',(-17.4799826883104,-50.160260628743,-29.3974274470402));
#21454=CARTESIAN_POINT('Ctrl Pts',(-17.4936138858681,-50.3181512763535,
-29.4074381965724));
#21455=CARTESIAN_POINT('Ctrl Pts',(-17.5231849738733,-50.4729978797759,
-29.4174489461046));
#21456=CARTESIAN_POINT('Ctrl Pts',(-17.6787081164242,-51.2873821991274,
-29.4700984538354));
#21457=CARTESIAN_POINT('Ctrl Pts',(-18.2751319414129,-52.0175676236174,
-29.5227479615662));
#21458=CARTESIAN_POINT('Ctrl Pts',(-19.0420767774903,-52.3325356948411,
-29.5753974692971));
#21459=CARTESIAN_POINT('Ctrl Pts',(-19.8090216135677,-52.6475037660647,
-29.6280469770279));
#21460=CARTESIAN_POINT('Ctrl Pts',(-20.7464874607337,-52.5472544840221,
-29.6806964847587));
#21461=CARTESIAN_POINT('Ctrl Pts',(-21.4294884330411,-52.0772343362577,
-29.7333459924896));
#21462=CARTESIAN_POINT('Ctrl Pts',(-22.1124894053484,-51.6072141884932,
-29.7859955002204));
#21463=CARTESIAN_POINT('Ctrl Pts',(-22.5410255027971,-50.767423175007,-29.8386450079512));
#21464=CARTESIAN_POINT('Ctrl Pts',(-22.5208264022779,-49.9385677812172,
-29.891294515682));
#21465=CARTESIAN_POINT('Ctrl Pts',(-22.5006273017587,-49.1097123874274,
-29.9439440234128));
#21466=CARTESIAN_POINT('Ctrl Pts',(-22.0316930032716,-48.2917926133339,
-29.9965935311437));
#21467=CARTESIAN_POINT('Ctrl Pts',(-21.3266077400392,-47.85559995057,-30.0492430388745));
#21468=CARTESIAN_POINT('Ctrl Pts',(-20.6215224768069,-47.4194072878061,
-30.1018925466053));
#21469=CARTESIAN_POINT('Ctrl Pts',(-19.6802862488292,-47.3649417363718,
-30.1545420543361));
#21470=CARTESIAN_POINT('Ctrl Pts',(-18.9295941868573,-47.716894425762,-30.207191562067));
#21471=CARTESIAN_POINT('Ctrl Pts',(-18.1789021248854,-48.0688471151522,
-30.2598410697978));
#21472=CARTESIAN_POINT('Ctrl Pts',(-17.6187542289192,-48.8272180453669,
-30.3124905775286));
#21473=CARTESIAN_POINT('Ctrl Pts',(-17.5030850295308,-49.6482112875982,
-30.3651400852594));
#21474=CARTESIAN_POINT('Ctrl Pts',(-17.4867713733357,-49.7640018486382,
-30.3725656226756));
#21475=CARTESIAN_POINT('Ctrl Pts',(-17.4792990573488,-49.8810380603009,
-30.3799911600918));
#21476=CARTESIAN_POINT('Ctrl Pts',(-17.4802499007281,-49.9981961378425,
-30.387416697508));
#21477=CARTESIAN_POINT('Origin',(-20.,-50.,-32.));
#21478=CARTESIAN_POINT('',(-17.4864434588916,-49.999628681025,-31.387416697508));
#21479=CARTESIAN_POINT('',(-17.4840572259774,-50.0020935757321,-31.112583302492));
#21480=CARTESIAN_POINT('',(-17.4825,-50.,-32.));
#21481=CARTESIAN_POINT('Ctrl Pts',(-17.4840572259774,-50.0020935757321,
-31.112583302492));
#21482=CARTESIAN_POINT('Ctrl Pts',(-17.4887252217618,-49.4184779588706,
-31.0757368287659));
#21483=CARTESIAN_POINT('Ctrl Pts',(-17.6911788800261,-48.8319402420143,
-31.0388903550399));
#21484=CARTESIAN_POINT('Ctrl Pts',(-18.0625522849953,-48.3861121432124,
-31.0020438813138));
#21485=CARTESIAN_POINT('Ctrl Pts',(-18.5932035245498,-47.7490734374465,
-30.949394373583));
#21486=CARTESIAN_POINT('Ctrl Pts',(-19.468742053114,-47.3993247593714,-30.8967448658521));
#21487=CARTESIAN_POINT('Ctrl Pts',(-20.2922557929138,-47.4954193536299,
-30.8440953581213));
#21488=CARTESIAN_POINT('Ctrl Pts',(-21.1157695327135,-47.5915139478884,
-30.7914458503905));
#21489=CARTESIAN_POINT('Ctrl Pts',(-21.8872584837488,-48.1334518144805,
-30.7387963426597));
#21490=CARTESIAN_POINT('Ctrl Pts',(-22.2569798619555,-48.8755536627342,
-30.6861468349289));
#21491=CARTESIAN_POINT('Ctrl Pts',(-22.6267012401623,-49.6176555109878,
-30.6334973271981));
#21492=CARTESIAN_POINT('Ctrl Pts',(-22.5946550455406,-50.559921340903,-30.5808478194672));
#21493=CARTESIAN_POINT('Ctrl Pts',(-22.1753689331017,-51.2751892673478,
-30.5281983117364));
#21494=CARTESIAN_POINT('Ctrl Pts',(-21.7560828206629,-51.9904571937926,
-30.4755488040056));
#21495=CARTESIAN_POINT('Ctrl Pts',(-20.9495567904068,-52.478727216767,-30.4228992962747));
#21496=CARTESIAN_POINT('Ctrl Pts',(-20.12141715346,-52.5186495463858,-30.3702497885439));
#21497=CARTESIAN_POINT('Ctrl Pts',(-19.2932775165132,-52.5585718760047,
-30.3176002808131));
#21498=CARTESIAN_POINT('Ctrl Pts',(-18.4435242728756,-52.150146512268,-30.2649507730823));
#21499=CARTESIAN_POINT('Ctrl Pts',(-17.9573801335119,-51.4785268829787,
-30.2123012653515));
#21500=CARTESIAN_POINT('Ctrl Pts',(-17.6504617638204,-51.0545118944526,
-30.1790619443983));
#21501=CARTESIAN_POINT('Ctrl Pts',(-17.4884707620747,-50.5255928985278,
-30.1458226234451));
#21502=CARTESIAN_POINT('Ctrl Pts',(-17.4853853786729,-49.9984092958285,
-30.112583302492));
#21503=CARTESIAN_POINT('Ctrl Pts',(-17.4802499007281,-49.9981961378425,
-30.387416697508));
#21504=CARTESIAN_POINT('Ctrl Pts',(-17.4860408503046,-50.7117274452609,
-30.4326406678226));
#21505=CARTESIAN_POINT('Ctrl Pts',(-17.8042645925932,-51.4297790158306,
-30.4778646381373));
#21506=CARTESIAN_POINT('Ctrl Pts',(-18.3404527356926,-51.8984842757991,
-30.5230886084519));
#21507=CARTESIAN_POINT('Ctrl Pts',(-18.9646801440534,-52.4441484675212,
-30.5757381161827));
#21508=CARTESIAN_POINT('Ctrl Pts',(-19.8843254635857,-52.6518612967176,
-30.6283876239135));
#21509=CARTESIAN_POINT('Ctrl Pts',(-20.6824814735535,-52.4274593109222,
-30.6810371316444));
#21510=CARTESIAN_POINT('Ctrl Pts',(-21.4806374835213,-52.2030573251268,
-30.7336866393752));
#21511=CARTESIAN_POINT('Ctrl Pts',(-22.1573041839245,-51.5465405243398,
-30.786336147106));
#21512=CARTESIAN_POINT('Ctrl Pts',(-22.4057250160791,-50.7555308166698,
-30.8389856548368));
#21513=CARTESIAN_POINT('Ctrl Pts',(-22.6541458482338,-49.9645211089998,
-30.8916351625677));
#21514=CARTESIAN_POINT('Ctrl Pts',(-22.4743208121398,-49.0390184944469,
-30.9442846702985));
#21515=CARTESIAN_POINT('Ctrl Pts',(-21.9477708533448,-48.3985855093739,
-30.9969341780293));
#21516=CARTESIAN_POINT('Ctrl Pts',(-21.4212208945498,-47.7581525243009,
-31.0495836857601));
#21517=CARTESIAN_POINT('Ctrl Pts',(-20.5479460130537,-47.4027891687077,
-31.1022331934909));
#21518=CARTESIAN_POINT('Ctrl Pts',(-19.7238320966554,-47.4935940159087,
-31.1548827012218));
#21519=CARTESIAN_POINT('Ctrl Pts',(-18.8997181802571,-47.5843988631096,
-31.2075322089526));
#21520=CARTESIAN_POINT('Ctrl Pts',(-18.1247652289565,-48.1213719131045,
-31.2601817166834));
#21521=CARTESIAN_POINT('Ctrl Pts',(-17.7502863786615,-48.8610845993269,
-31.3128312244143));
#21522=CARTESIAN_POINT('Ctrl Pts',(-17.5734522959595,-49.2103871413211,
-31.3376930487788));
#21523=CARTESIAN_POINT('Ctrl Pts',(-17.4859182820506,-49.6048977589854,
-31.3625548731434));
#21524=CARTESIAN_POINT('Ctrl Pts',(-17.4864434588916,-49.999628681025,-31.387416697508));
#21525=CARTESIAN_POINT('Origin',(-20.,-50.,-32.));
#21526=CARTESIAN_POINT('',(-17.4815611182796,-50.0021533196962,-32.387416697508));
#21527=CARTESIAN_POINT('',(-17.4785348819534,-49.9995340142102,-32.112583302492));
#21528=CARTESIAN_POINT('',(-17.4825,-50.,-32.));
#21529=CARTESIAN_POINT('Ctrl Pts',(-17.4785348819534,-49.9995340142102,
-32.112583302492));
#21530=CARTESIAN_POINT('Ctrl Pts',(-17.4784687956751,-49.97381126057,-32.1109500495483));
#21531=CARTESIAN_POINT('Ctrl Pts',(-17.4788287321595,-49.9480904010419,
-32.1093167966047));
#21532=CARTESIAN_POINT('Ctrl Pts',(-17.4796204177225,-49.9223828375818,
-32.1076835436611));
#21533=CARTESIAN_POINT('Ctrl Pts',(-17.5051411769714,-49.093674359568,-32.0550340359302));
#21534=CARTESIAN_POINT('Ctrl Pts',(-17.9793175952482,-48.2787826016234,
-32.0023845281994));
#21535=CARTESIAN_POINT('Ctrl Pts',(-18.6871890040388,-47.847126350306,-31.9497350204686));
#21536=CARTESIAN_POINT('Ctrl Pts',(-19.3950604128295,-47.4154700989886,
-31.8970855127378));
#21537=CARTESIAN_POINT('Ctrl Pts',(-20.336626812134,-47.3670493542984,-31.844436005007));
#21538=CARTESIAN_POINT('Ctrl Pts',(-21.0850433930516,-47.7238149245155,
-31.7917864972761));
#21539=CARTESIAN_POINT('Ctrl Pts',(-21.8334599739691,-48.0805804947325,
-31.7391369895453));
#21540=CARTESIAN_POINT('Ctrl Pts',(-22.3887267364997,-48.8425323798569,
-31.6864874818145));
#21541=CARTESIAN_POINT('Ctrl Pts',(-22.4991219376876,-49.664251279627,-31.6338379740837));
#21542=CARTESIAN_POINT('Ctrl Pts',(-22.6095171388755,-50.4859701793971,
-31.5811884663529));
#21543=CARTESIAN_POINT('Ctrl Pts',(-22.2750407787207,-51.3674560938129,
-31.5285389586221));
#21544=CARTESIAN_POINT('Ctrl Pts',(-21.6473226287802,-51.909100788165,-31.4758894508912));
#21545=CARTESIAN_POINT('Ctrl Pts',(-21.0196044788396,-52.4507454825172,
-31.4232399431604));
#21546=CARTESIAN_POINT('Ctrl Pts',(-20.0986445391132,-52.6525489568057,
-31.3705904354295));
#21547=CARTESIAN_POINT('Ctrl Pts',(-19.3019459934108,-52.4230266747496,
-31.3179409276987));
#21548=CARTESIAN_POINT('Ctrl Pts',(-18.5052474477083,-52.1935043926934,
-31.2652914199679));
#21549=CARTESIAN_POINT('Ctrl Pts',(-17.8328102960298,-51.5326563542926,
-31.2126419122371));
#21550=CARTESIAN_POINT('Ctrl Pts',(-17.5894736954629,-50.7400679683638,
-31.1599924045063));
#21551=CARTESIAN_POINT('Ctrl Pts',(-17.5164349010069,-50.5021682850724,
-31.1441893705015));
#21552=CARTESIAN_POINT('Ctrl Pts',(-17.482055175614,-50.2523996839241,-31.1283863364968));
#21553=CARTESIAN_POINT('Ctrl Pts',(-17.4840572259774,-50.0020935757321,
-31.112583302492));
#21554=CARTESIAN_POINT('Ctrl Pts',(-17.4864434588916,-49.999628681025,-31.387416697508));
#21555=CARTESIAN_POINT('Ctrl Pts',(-17.4870304410677,-50.4408134354357,
-31.4152043808742));
#21556=CARTESIAN_POINT('Ctrl Pts',(-17.5976226663159,-50.8822733983299,
-31.4429920642405));
#21557=CARTESIAN_POINT('Ctrl Pts',(-17.8164875791883,-51.2611951379893,
-31.4707797476067));
#21558=CARTESIAN_POINT('Ctrl Pts',(-18.2311723792997,-51.9791406679796,
-31.5234292553375));
#21559=CARTESIAN_POINT('Ctrl Pts',(-19.0345467288119,-52.4725794055107,
-31.5760787630683));
#21560=CARTESIAN_POINT('Ctrl Pts',(-19.8624130831367,-52.5178184025531,
-31.6287282707992));
#21561=CARTESIAN_POINT('Ctrl Pts',(-20.6902794374616,-52.5630573995955,
-31.68137777853));
#21562=CARTESIAN_POINT('Ctrl Pts',(-21.5426377965991,-52.1600966561492,
-31.7340272862608));
#21563=CARTESIAN_POINT('Ctrl Pts',(-22.0330844600882,-51.4916122975072,
-31.7866767939917));
#21564=CARTESIAN_POINT('Ctrl Pts',(-22.5235311235772,-50.8231279388651,
-31.8393263017225));
#21565=CARTESIAN_POINT('Ctrl Pts',(-22.6520660914177,-49.8891199650273,
-31.8919758094533));
#21566=CARTESIAN_POINT('Ctrl Pts',(-22.3604199905464,-49.1130066876489,
-31.9446253171841));
#21567=CARTESIAN_POINT('Ctrl Pts',(-22.0687738896751,-48.3368934102704,
-31.9972748249149));
#21568=CARTESIAN_POINT('Ctrl Pts',(-21.3569467200919,-47.7186748293514,
-32.0499243326458));
#21569=CARTESIAN_POINT('Ctrl Pts',(-20.5476345045051,-47.5386109374172,
-32.1025738403766));
#21570=CARTESIAN_POINT('Ctrl Pts',(-19.7383222889183,-47.3585470454831,
-32.1552233481074));
#21571=CARTESIAN_POINT('Ctrl Pts',(-18.8315250273277,-47.6166378425338,
-32.2078728558382));
#21572=CARTESIAN_POINT('Ctrl Pts',(-18.2383254687796,-48.1958817904649,
-32.2605223635691));
#21573=CARTESIAN_POINT('Ctrl Pts',(-17.76175461295,-48.6612408421056,-32.302820474882));
#21574=CARTESIAN_POINT('Ctrl Pts',(-17.4875910678703,-49.3338837640615,
-32.345118586195));
#21575=CARTESIAN_POINT('Ctrl Pts',(-17.4815611182796,-50.0021533196962,
-32.387416697508));
#21576=CARTESIAN_POINT('Origin',(-20.,-50.,-32.));
#21577=CARTESIAN_POINT('',(-17.4801090985914,-49.9982532978734,-33.387416697508));
#21578=CARTESIAN_POINT('',(-17.485278158989,-49.9983487243454,-33.112583302492));
#21579=CARTESIAN_POINT('',(-17.4825,-50.,-32.));
#21580=CARTESIAN_POINT('Ctrl Pts',(-17.485278158989,-49.9983487243454,-33.112583302492));
#21581=CARTESIAN_POINT('Ctrl Pts',(-17.4834356301179,-49.6959336765475,
-33.0935137626));
#21582=CARTESIAN_POINT('Ctrl Pts',(-17.5339467999326,-49.3941133640789,
-33.0744442227079));
#21583=CARTESIAN_POINT('Ctrl Pts',(-17.6395803816627,-49.1130068275169,
-33.0553746828159));
#21584=CARTESIAN_POINT('Ctrl Pts',(-17.931226436545,-48.3368936725219,-33.0027251750851));
#21585=CARTESIAN_POINT('Ctrl Pts',(-18.6430534938817,-47.7186751890883,
-32.9500756673542));
#21586=CARTESIAN_POINT('Ctrl Pts',(-19.45236558185,-47.5386113255479,-32.8974261596234));
#21587=CARTESIAN_POINT('Ctrl Pts',(-20.2616776698183,-47.3585474620076,
-32.8447766518926));
#21588=CARTESIAN_POINT('Ctrl Pts',(-21.1684747884181,-47.6166382183606,
-32.7921271441618));
#21589=CARTESIAN_POINT('Ctrl Pts',(-21.761674253426,-48.1958820749521,-32.7394776364309));
#21590=CARTESIAN_POINT('Ctrl Pts',(-22.3548737184339,-48.7751259315435,
-32.6868281287001));
#21591=CARTESIAN_POINT('Ctrl Pts',(-22.63447552985,-49.6755228883735,-32.6341786209693));
#21592=CARTESIAN_POINT('Ctrl Pts',(-22.4737264583211,-50.4888916772308,
-32.5815291132385));
#21593=CARTESIAN_POINT('Ctrl Pts',(-22.3129773867922,-51.3022604660881,
-32.5288796055077));
#21594=CARTESIAN_POINT('Ctrl Pts',(-21.7118774323183,-52.0286010869729,
-32.4762300977768));
#21595=CARTESIAN_POINT('Ctrl Pts',(-20.9429261184457,-52.3386380647326,
-32.423580590046));
#21596=CARTESIAN_POINT('Ctrl Pts',(-20.1739748045732,-52.6486750424923,
-32.3709310823152));
#21597=CARTESIAN_POINT('Ctrl Pts',(-19.2371721313021,-52.5424083771271,
-32.3182815745844));
#21598=CARTESIAN_POINT('Ctrl Pts',(-18.5572033447772,-52.0680124454029,
-32.2656320668536));
#21599=CARTESIAN_POINT('Ctrl Pts',(-17.8983280322473,-51.6083328630869,
-32.2146158120664));
#21600=CARTESIAN_POINT('Ctrl Pts',(-17.4805991515588,-50.8030094089147,
-32.1635995572792));
#21601=CARTESIAN_POINT('Ctrl Pts',(-17.4785348819534,-49.9995340142102,
-32.112583302492));
#21602=CARTESIAN_POINT('Ctrl Pts',(-17.4815611182796,-50.0021533196962,
-32.387416697508));
#21603=CARTESIAN_POINT('Ctrl Pts',(-17.480085440131,-50.1656954465103,-32.3977680939259));
#21604=CARTESIAN_POINT('Ctrl Pts',(-17.4946683427963,-50.3289756514404,
-32.4081194903437));
#21605=CARTESIAN_POINT('Ctrl Pts',(-17.5262731516027,-50.4888917543231,
-32.4184708867615));
#21606=CARTESIAN_POINT('Ctrl Pts',(-17.6870222484798,-51.3022606714387,
-32.4711203944923));
#21607=CARTESIAN_POINT('Ctrl Pts',(-18.2881222977398,-52.0286014068583,
-32.5237699022232));
#21608=CARTESIAN_POINT('Ctrl Pts',(-19.0570737328665,-52.3386384335071,
-32.576419409954));
#21609=CARTESIAN_POINT('Ctrl Pts',(-19.8260251679932,-52.6486754601558,
-32.6290689176848));
#21610=CARTESIAN_POINT('Ctrl Pts',(-20.7628279889865,-52.5424087780336,
-32.6817184254156));
#21611=CARTESIAN_POINT('Ctrl Pts',(-21.4427968827342,-52.068012771503,-32.7343679331465));
#21612=CARTESIAN_POINT('Ctrl Pts',(-22.1227657764818,-51.5936167649724,
-32.7870174408773));
#21613=CARTESIAN_POINT('Ctrl Pts',(-22.5459007429837,-50.7510914340334,
-32.8396669486081));
#21614=CARTESIAN_POINT('Ctrl Pts',(-22.5203799797104,-49.9223828253425,
-32.8923164563389));
#21615=CARTESIAN_POINT('Ctrl Pts',(-22.4948592164371,-49.0936742166515,
-32.9449659640698));
#21616=CARTESIAN_POINT('Ctrl Pts',(-22.0206827233885,-48.2787823302085,
-32.9976154718006));
#21617=CARTESIAN_POINT('Ctrl Pts',(-21.3128112029753,-47.8471260108243,
-33.0502649795314));
#21618=CARTESIAN_POINT('Ctrl Pts',(-20.604939682562,-47.41546969144,-33.1029144872622));
#21619=CARTESIAN_POINT('Ctrl Pts',(-19.663373134784,-47.3670489391145,-33.155563994993));
#21620=CARTESIAN_POINT('Ctrl Pts',(-18.9149564358503,-47.7238145655892,
-33.2082135027239));
#21621=CARTESIAN_POINT('Ctrl Pts',(-18.1665397369167,-48.0805801920638,
-33.2608630104547));
#21622=CARTESIAN_POINT('Ctrl Pts',(-17.6112728868275,-48.8425321973387,
-33.3135125181855));
#21623=CARTESIAN_POINT('Ctrl Pts',(-17.5008776682317,-49.6642512266837,
-33.3661620259163));
#21624=CARTESIAN_POINT('Ctrl Pts',(-17.4860221059945,-49.7748275572271,
-33.3732469164469));
#21625=CARTESIAN_POINT('Ctrl Pts',(-17.4792224123127,-49.8864861669174,
-33.3803318069775));
#21626=CARTESIAN_POINT('Ctrl Pts',(-17.4801090985914,-49.9982532978734,
-33.387416697508));
#21627=CARTESIAN_POINT('Origin',(-20.,-50.,-32.));
#21628=CARTESIAN_POINT('',(-17.4864167202486,-49.9995432846338,-34.387416697508));
#21629=CARTESIAN_POINT('',(-17.4841987514942,-50.0020603003561,-34.112583302492));
#21630=CARTESIAN_POINT('',(-17.4825,-50.,-32.));
#21631=CARTESIAN_POINT('Ctrl Pts',(-17.4841987514942,-50.0020603003561,
-34.112583302492));
#21632=CARTESIAN_POINT('Ctrl Pts',(-17.4887312218023,-49.4237578373463,
-34.0760774756515));
#21633=CARTESIAN_POINT('Ctrl Pts',(-17.6871331895373,-48.8426456017127,
-34.0395716488111));
#21634=CARTESIAN_POINT('Ctrl Pts',(-18.0522294537946,-48.3985857618973,
-34.0030658219707));
#21635=CARTESIAN_POINT('Ctrl Pts',(-18.5787793295592,-47.7581528778126,
-33.9504163142399));
#21636=CARTESIAN_POINT('Ctrl Pts',(-19.4520540733505,-47.4027895782559,
-33.8977668065091));
#21637=CARTESIAN_POINT('Ctrl Pts',(-20.2761678597962,-47.493594411138,-33.8451172987782));
#21638=CARTESIAN_POINT('Ctrl Pts',(-21.1002816462419,-47.58439924402,-33.7924677910474));
#21639=CARTESIAN_POINT('Ctrl Pts',(-21.875234475342,-48.1213722093409,-33.7398182833166));
#21640=CARTESIAN_POINT('Ctrl Pts',(-22.2497132665864,-48.8610847789196,
-33.6871687755858));
#21641=CARTESIAN_POINT('Ctrl Pts',(-22.6241920578308,-49.6007973484984,
-33.6345192678549));
#21642=CARTESIAN_POINT('Ctrl Pts',(-22.5981968112194,-50.543249522335,-33.5818697601241));
#21643=CARTESIAN_POINT('Ctrl Pts',(-22.1835120764988,-51.2611949391142,
-33.5292202523933));
#21644=CARTESIAN_POINT('Ctrl Pts',(-21.7688273417781,-51.9791403558935,
-33.4765707446625));
#21645=CARTESIAN_POINT('Ctrl Pts',(-20.9654531189481,-52.4725790156154,
-33.4239212369317));
#21646=CARTESIAN_POINT('Ctrl Pts',(-20.1375868951676,-52.5178180055241,
-33.3712717292008));
#21647=CARTESIAN_POINT('Ctrl Pts',(-19.309720671387,-52.5630569954329,-33.31862222147));
#21648=CARTESIAN_POINT('Ctrl Pts',(-18.4573624466559,-52.1600963155286,
-33.2659727137392));
#21649=CARTESIAN_POINT('Ctrl Pts',(-17.9669158605042,-51.4916120622984,
-33.2133232060083));
#21650=CARTESIAN_POINT('Ctrl Pts',(-17.6541079863296,-51.0652513859749,
-33.1797432381696));
#21651=CARTESIAN_POINT('Ctrl Pts',(-17.4885227081802,-50.5308779639869,
-33.1461632703308));
#21652=CARTESIAN_POINT('Ctrl Pts',(-17.485278158989,-49.9983487243454,-33.112583302492));
#21653=CARTESIAN_POINT('Ctrl Pts',(-17.4801090985914,-49.9982532978734,
-33.387416697508));
#21654=CARTESIAN_POINT('Ctrl Pts',(-17.4858115890802,-50.7170543175381,
-33.4329813147083));
#21655=CARTESIAN_POINT('Ctrl Pts',(-17.8094290744944,-51.4403438659751,
-33.4785459319085));
#21656=CARTESIAN_POINT('Ctrl Pts',(-18.3526771114574,-51.9091010892068,
-33.5241105491088));
#21657=CARTESIAN_POINT('Ctrl Pts',(-18.9803953603814,-52.4507458689696,
-33.5767600568396));
#21658=CARTESIAN_POINT('Ctrl Pts',(-19.9013554453319,-52.65254937508,-33.6294095645704));
#21659=CARTESIAN_POINT('Ctrl Pts',(-20.6980541166638,-52.4230270568311,
-33.6820590723013));
#21660=CARTESIAN_POINT('Ctrl Pts',(-21.4947527879958,-52.1935047385821,
-33.7347085800321));
#21661=CARTESIAN_POINT('Ctrl Pts',(-22.1671900457094,-51.5326565959736,
-33.7873580877629));
#21662=CARTESIAN_POINT('Ctrl Pts',(-22.4105266846474,-50.7400680850634,
-33.8400075954937));
#21663=CARTESIAN_POINT('Ctrl Pts',(-22.6538633235855,-49.9474795741532,
-33.8926571032246));
#21664=CARTESIAN_POINT('Ctrl Pts',(-22.468099343748,-49.0231506949411,-33.9453066109554));
#21665=CARTESIAN_POINT('Ctrl Pts',(-21.9374480205163,-48.3861118887221,
-33.9979561186862));
#21666=CARTESIAN_POINT('Ctrl Pts',(-21.4067966972846,-47.749073082503,-34.050605626417));
#21667=CARTESIAN_POINT('Ctrl Pts',(-20.5312580306586,-47.3993243492769,
-34.1032551341478));
#21668=CARTESIAN_POINT('Ctrl Pts',(-19.7077441610009,-47.4954189586884,
-34.1559046418787));
#21669=CARTESIAN_POINT('Ctrl Pts',(-18.8842302913432,-47.5915135680998,
-34.2085541496095));
#21670=CARTESIAN_POINT('Ctrl Pts',(-18.1127412186538,-48.1334515201489,
-34.2612036573403));
#21671=CARTESIAN_POINT('Ctrl Pts',(-17.7430197821465,-48.8755534854229,
-34.3138531650712));
#21672=CARTESIAN_POINT('Ctrl Pts',(-17.5708243457006,-49.22118281383,-34.3383743425501));
#21673=CARTESIAN_POINT('Ctrl Pts',(-17.4857792242903,-49.610231161691,-34.3628955200291));
#21674=CARTESIAN_POINT('Ctrl Pts',(-17.4864167202486,-49.9995432846338,
-34.387416697508));
#21675=CARTESIAN_POINT('Origin',(-20.,-50.,-32.));
#21676=CARTESIAN_POINT('',(-17.4817210057717,-50.002176808168,-35.387416697508));
#21677=CARTESIAN_POINT('',(-17.478494824499,-49.9996299858999,-35.112583302492));
#21678=CARTESIAN_POINT('',(-17.4825,-50.,-32.));
#21679=CARTESIAN_POINT('Ctrl Pts',(-17.478494824499,-49.9996299858999,-35.112583302492));
#21680=CARTESIAN_POINT('Ctrl Pts',(-17.4784526521761,-49.9792730852633,
-35.111290696434));
#21681=CARTESIAN_POINT('Ctrl Pts',(-17.4786780841199,-49.9589171423125,
-35.109998090376));
#21682=CARTESIAN_POINT('Ctrl Pts',(-17.4791739952253,-49.9385677909044,
-35.108705484318));
#21683=CARTESIAN_POINT('Ctrl Pts',(-17.4993730925594,-49.1097125278149,
-35.0560559765871));
#21684=CARTESIAN_POINT('Ctrl Pts',(-17.9683073171013,-48.2917928826973,
-35.0034064688563));
#21685=CARTESIAN_POINT('Ctrl Pts',(-18.6733924691504,-47.8556002887155,
-34.9507569611255));
#21686=CARTESIAN_POINT('Ctrl Pts',(-19.3784776211995,-47.4194076947338,
-34.8981074533947));
#21687=CARTESIAN_POINT('Ctrl Pts',(-20.3197137007558,-47.3649421518879,
-34.8454579456639));
#21688=CARTESIAN_POINT('Ctrl Pts',(-21.0704056443528,-47.7168947857795,
-34.792808437933));
#21689=CARTESIAN_POINT('Ctrl Pts',(-21.8210975879499,-48.0688474196711,
-34.7401589302022));
#21690=CARTESIAN_POINT('Ctrl Pts',(-22.3812453955877,-48.8272182303001,
-34.6875094224714));
#21691=CARTESIAN_POINT('Ctrl Pts',(-22.4969145767365,-49.6482113430708,
-34.6348599147406));
#21692=CARTESIAN_POINT('Ctrl Pts',(-22.6125837578853,-50.4692044558415,
-34.5822104070098));
#21693=CARTESIAN_POINT('Ctrl Pts',(-22.2837743125452,-51.352819870754,-34.5295608992789));
#21694=CARTESIAN_POINT('Ctrl Pts',(-21.6595470026173,-51.8984839764315,
-34.4769113915481));
#21695=CARTESIAN_POINT('Ctrl Pts',(-21.0353196926895,-52.4441480821091,
-34.4242618838173));
#21696=CARTESIAN_POINT('Ctrl Pts',(-20.1156745181739,-52.6518608785517,
-34.3716123760864));
#21697=CARTESIAN_POINT('Ctrl Pts',(-19.3175186340655,-52.4274589281418,
-34.3189628683556));
#21698=CARTESIAN_POINT('Ctrl Pts',(-18.5193627499571,-52.2030569777319,
-34.2663133606248));
#21699=CARTESIAN_POINT('Ctrl Pts',(-17.8426961562558,-51.5465402804695,
-34.213663852894));
#21700=CARTESIAN_POINT('Ctrl Pts',(-17.5942753632741,-50.755530697532,-34.1610143451632));
#21701=CARTESIAN_POINT('Ctrl Pts',(-17.5181032169182,-50.5129869998117,
-34.1448706642728));
#21702=CARTESIAN_POINT('Ctrl Pts',(-17.482194393269,-50.2577983901072,-34.1287269833824));
#21703=CARTESIAN_POINT('Ctrl Pts',(-17.4841987514942,-50.0020603003561,
-34.112583302492));
#21704=CARTESIAN_POINT('Ctrl Pts',(-17.4864167202486,-49.9995432846338,
-34.387416697508));
#21705=CARTESIAN_POINT('Ctrl Pts',(-17.487147994139,-50.446124611105,-34.4155450277599));
#21706=CARTESIAN_POINT('Ctrl Pts',(-17.6006244490009,-50.8930530251216,
-34.4436733580117));
#21707=CARTESIAN_POINT('Ctrl Pts',(-17.8246307238694,-51.2751894684295,
-34.4718016882636));
#21708=CARTESIAN_POINT('Ctrl Pts',(-18.2439169024245,-51.9904575076633,
-34.5244511959944));
#21709=CARTESIAN_POINT('Ctrl Pts',(-19.0504430598599,-52.4787276076318,
-34.5771007037253));
#21710=CARTESIAN_POINT('Ctrl Pts',(-19.8785828273941,-52.5186499435459,
-34.6297502114561));
#21711=CARTESIAN_POINT('Ctrl Pts',(-20.7067225949284,-52.5585722794599,
-34.6823997191869));
#21712=CARTESIAN_POINT('Ctrl Pts',(-21.5564759725616,-52.1501468513196,
-34.7350492269177));
#21713=CARTESIAN_POINT('Ctrl Pts',(-22.0426201885842,-51.4785271161241,
-34.7876987346485));
#21714=CARTESIAN_POINT('Ctrl Pts',(-22.5287644046068,-50.8069073809286,
-34.8403482423794));
#21715=CARTESIAN_POINT('Ctrl Pts',(-22.6512994590187,-49.872093338678,-34.8929977501102));
#21716=CARTESIAN_POINT('Ctrl Pts',(-22.3546759482698,-49.097868719883,-34.945647257841));
#21717=CARTESIAN_POINT('Ctrl Pts',(-22.058052437521,-48.323644101088,-34.9982967655718));
#21718=CARTESIAN_POINT('Ctrl Pts',(-21.3422703616113,-47.7100089057485,
-35.0509462733027));
#21719=CARTESIAN_POINT('Ctrl Pts',(-20.5318186398909,-47.5351453182397,
-35.1035957810335));
#21720=CARTESIAN_POINT('Ctrl Pts',(-19.7213669181704,-47.3602817307308,
-35.1562452887643));
#21721=CARTESIAN_POINT('Ctrl Pts',(-18.8162455506391,-47.6241897510527,
-35.2088947964951));
#21722=CARTESIAN_POINT('Ctrl Pts',(-18.2267775452558,-48.2072306913854,
-35.261544304226));
#21723=CARTESIAN_POINT('Ctrl Pts',(-17.7570184927424,-48.6718678849328,
-35.3035017686533));
#21724=CARTESIAN_POINT('Ctrl Pts',(-17.4877252255933,-49.3391806685967,
-35.3454592330807));
#21725=CARTESIAN_POINT('Ctrl Pts',(-17.4817210057717,-50.002176808168,-35.387416697508));
#21726=CARTESIAN_POINT('Origin',(-20.,-50.,-32.));
#21727=CARTESIAN_POINT('',(-17.4799717713781,-49.9983136769593,-36.387416697508));
#21728=CARTESIAN_POINT('',(-17.4851667329155,-49.9982906274316,-36.112583302492));
#21729=CARTESIAN_POINT('',(-17.4825,-50.,-32.));
#21730=CARTESIAN_POINT('Ctrl Pts',(-17.4851667329155,-49.9982906274316,
-36.112583302492));
#21731=CARTESIAN_POINT('Ctrl Pts',(-17.4832880584752,-49.7013108562046,
-36.0938544094856));
#21732=CARTESIAN_POINT('Ctrl Pts',(-17.5319619332951,-49.4049268457409,
-36.0751255164792));
#21733=CARTESIAN_POINT('Ctrl Pts',(-17.6339336595649,-49.1281813633219,
-36.0563966234728));
#21734=CARTESIAN_POINT('Ctrl Pts',(-17.9205902809002,-48.3502115489225,
-36.003747115742));
#21735=CARTESIAN_POINT('Ctrl Pts',(-18.6284330841387,-47.7274351695357,
-35.9510976080112));
#21736=CARTESIAN_POINT('Ctrl Pts',(-19.436572298498,-47.5421784263544,-35.8984481002803));
#21737=CARTESIAN_POINT('Ctrl Pts',(-20.2447115128574,-47.3569216831732,
-35.8457985925495));
#21738=CARTESIAN_POINT('Ctrl Pts',(-21.1531471383375,-47.6091845761975,
-35.7931490848186));
#21739=CARTESIAN_POINT('Ctrl Pts',(-21.7500536985207,-48.1846075589684,
-35.7404995770878));
#21740=CARTESIAN_POINT('Ctrl Pts',(-22.346960258704,-48.7600305417393,-35.687850069357));
#21741=CARTESIAN_POINT('Ctrl Pts',(-22.6323377535904,-49.6586136142567,
-35.6352005616262));
#21742=CARTESIAN_POINT('Ctrl Pts',(-22.4768146355635,-50.4729978051899,
-35.5825510538954));
#21743=CARTESIAN_POINT('Ctrl Pts',(-22.3212915175367,-51.287381996123,-35.5299015461646));
#21744=CARTESIAN_POINT('Ctrl Pts',(-21.7248677865967,-52.0175673054719,
-35.4772520384337));
#21745=CARTESIAN_POINT('Ctrl Pts',(-20.9579230714571,-52.332535327029,-35.4246025307029));
#21746=CARTESIAN_POINT('Ctrl Pts',(-20.1909783563175,-52.6475033485861,
-35.3719530229721));
#21747=CARTESIAN_POINT('Ctrl Pts',(-19.2535126569782,-52.5472540823515,
-35.3193035152413));
#21748=CARTESIAN_POINT('Ctrl Pts',(-18.5705117923717,-52.0772340087034,
-35.2666540075105));
#21749=CARTESIAN_POINT('Ctrl Pts',(-17.9042793856912,-51.618753469246,-35.2152971058376));
#21750=CARTESIAN_POINT('Ctrl Pts',(-17.4801703851418,-50.8084358381416,
-35.1639402041648));
#21751=CARTESIAN_POINT('Ctrl Pts',(-17.478494824499,-49.9996299858999,-35.112583302492));
#21752=CARTESIAN_POINT('Ctrl Pts',(-17.4817210057717,-50.002176808168,-35.387416697508));
#21753=CARTESIAN_POINT('Ctrl Pts',(-17.4801909471942,-50.1711284722182,
-35.3981087408115));
#21754=CARTESIAN_POINT('Ctrl Pts',(-17.495758511786,-50.3397998194272,-35.4088007841149));
#21755=CARTESIAN_POINT('Ctrl Pts',(-17.5294633202138,-50.5047654720315,
-35.4194928274184));
#21756=CARTESIAN_POINT('Ctrl Pts',(-17.6954317437902,-51.3170854520013,
-35.4721423351492));
#21757=CARTESIAN_POINT('Ctrl Pts',(-18.3011832341783,-52.0395515515973,
-35.5247918428801));
#21758=CARTESIAN_POINT('Ctrl Pts',(-19.0721095647582,-52.3446447509478,
-35.5774413506109));
#21759=CARTESIAN_POINT('Ctrl Pts',(-19.8430358953381,-52.6497379502984,
-35.6300908583417));
#21760=CARTESIAN_POINT('Ctrl Pts',(-20.7791370661099,-52.5374582494034,
-35.6827403660725));
#21761=CARTESIAN_POINT('Ctrl Pts',(-21.4560458464227,-52.0587059433,-35.7353898738033));
#21762=CARTESIAN_POINT('Ctrl Pts',(-22.1329546267354,-51.5799536371965,
-35.7880393815342));
#21763=CARTESIAN_POINT('Ctrl Pts',(-22.5506710165893,-50.7347287258845,
-35.840688889265));
#21764=CARTESIAN_POINT('Ctrl Pts',(-22.5198296427718,-49.9062010696257,
-35.8933383969958));
#21765=CARTESIAN_POINT('Ctrl Pts',(-22.4889882689544,-49.077673413367,-35.9459879047267));
#21766=CARTESIAN_POINT('Ctrl Pts',(-22.0095891314657,-48.2658430121615,
-35.9986374124575));
#21767=CARTESIAN_POINT('Ctrl Pts',(-21.2989605391671,-47.8387408332513,
-36.0512869201883));
#21768=CARTESIAN_POINT('Ctrl Pts',(-20.5883319468686,-47.4116386543412,
-36.1039364279191));
#21769=CARTESIAN_POINT('Ctrl Pts',(-19.6464738997602,-47.3692646977264,
-36.1565859356499));
#21770=CARTESIAN_POINT('Ctrl Pts',(-18.9003634208124,-47.7308285518507,
-36.2092354433807));
#21771=CARTESIAN_POINT('Ctrl Pts',(-18.1542529418645,-48.092392405975,-36.2618849511116));
#21772=CARTESIAN_POINT('Ctrl Pts',(-17.6038900310774,-48.8578940708383,
-36.3145344588424));
#21773=CARTESIAN_POINT('Ctrl Pts',(-17.4987733448449,-49.6803050083411,
-36.3671839665732));
#21774=CARTESIAN_POINT('Ctrl Pts',(-17.4853082133811,-49.7856533767842,
-36.3739282102182));
#21775=CARTESIAN_POINT('Ctrl Pts',(-17.4791490558524,-49.8919355603607,
-36.3806724538631));
#21776=CARTESIAN_POINT('Ctrl Pts',(-17.4799717713781,-49.9983136769593,
-36.387416697508));
#21777=CARTESIAN_POINT('Origin',(-20.,-50.,-32.));
#21778=CARTESIAN_POINT('',(-17.4863844696326,-49.9994585735565,-37.387416697508));
#21779=CARTESIAN_POINT('',(-17.4843373872682,-50.0020238412825,-37.112583302492));
#21780=CARTESIAN_POINT('',(-17.4825,-50.,-32.));
#21781=CARTESIAN_POINT('Ctrl Pts',(-17.4843373872682,-50.0020238412825,
-37.112583302492));
#21782=CARTESIAN_POINT('Ctrl Pts',(-17.4887305158478,-49.429037789462,-37.0764181225372));
#21783=CARTESIAN_POINT('Ctrl Pts',(-17.6831296450892,-48.8533549285412,
-37.0402529425824));
#21784=CARTESIAN_POINT('Ctrl Pts',(-18.0419869290546,-48.4111254070499,
-37.0040877626276));
#21785=CARTESIAN_POINT('Ctrl Pts',(-18.5644137321291,-47.7673247501846,
-36.9514382548968));
#21786=CARTESIAN_POINT('Ctrl Pts',(-19.4353886851995,-47.4063614792004,
-36.898788747166));
#21787=CARTESIAN_POINT('Ctrl Pts',(-20.2600685400885,-47.4918728064946,
-36.8461392394351));
#21788=CARTESIAN_POINT('Ctrl Pts',(-21.0847483949774,-47.5773841337888,
-36.7934897317043));
#21789=CARTESIAN_POINT('Ctrl Pts',(-21.8631331516847,-48.1093700593613,
-36.7408402239735));
#21790=CARTESIAN_POINT('Ctrl Pts',(-22.2423539164814,-48.8466628523593,
-36.6881907162427));
#21791=CARTESIAN_POINT('Ctrl Pts',(-22.6215746812781,-49.5839556453572,
-36.6355412085118));
#21792=CARTESIAN_POINT('Ctrl Pts',(-22.6016314541642,-50.5265553057806,
-36.582891700781));
#21793=CARTESIAN_POINT('Ctrl Pts',(-22.1915651943947,-51.2471486121684,
-36.5302421930502));
#21794=CARTESIAN_POINT('Ctrl Pts',(-21.7814989346252,-51.9677419185562,
-36.4775926853194));
#21795=CARTESIAN_POINT('Ctrl Pts',(-20.9813096422002,-52.4663288709085,
-36.4249431775885));
#21796=CARTESIAN_POINT('Ctrl Pts',(-20.1537509642527,-52.5168826559653,
-36.3722936698577));
#21797=CARTESIAN_POINT('Ctrl Pts',(-19.3261922863052,-52.5674364410221,
-36.3196441621269));
#21798=CARTESIAN_POINT('Ctrl Pts',(-18.4712642228353,-52.1699570587834,
-36.2669946543961));
#21799=CARTESIAN_POINT('Ctrl Pts',(-17.9765354108164,-51.5046357429582,
-36.2143451466653));
#21800=CARTESIAN_POINT('Ctrl Pts',(-17.6577953855276,-51.0759877081572,
-36.1804245319408));
#21801=CARTESIAN_POINT('Ctrl Pts',(-17.4885692720755,-50.5361620540716,
-36.1465039172164));
#21802=CARTESIAN_POINT('Ctrl Pts',(-17.4851667329155,-49.9982906274316,
-36.112583302492));
#21803=CARTESIAN_POINT('Ctrl Pts',(-17.4799717713781,-49.9983136769593,
-36.387416697508));
#21804=CARTESIAN_POINT('Ctrl Pts',(-17.4855716541017,-50.7223853138266,
-36.4333219615939));
#21805=CARTESIAN_POINT('Ctrl Pts',(-17.8146388682811,-51.4509014884862,
-36.4792272256798));
#21806=CARTESIAN_POINT('Ctrl Pts',(-18.364969405791,-51.9196391915133,-36.5251324897657));
#21807=CARTESIAN_POINT('Ctrl Pts',(-18.9961526146475,-52.4572422270403,
-36.5777819974965));
#21808=CARTESIAN_POINT('Ctrl Pts',(-19.9183894940382,-52.6531280879523,
-36.6304315052273));
#21809=CARTESIAN_POINT('Ctrl Pts',(-20.7135979791903,-52.4184949012781,
-36.6830810129582));
#21810=CARTESIAN_POINT('Ctrl Pts',(-21.5088064643423,-52.1838617146039,
-36.735730520689));
#21811=CARTESIAN_POINT('Ctrl Pts',(-22.1769865552557,-51.5187094803435,
-36.7883800284198));
#21812=CARTESIAN_POINT('Ctrl Pts',(-22.4152289681752,-50.724574842535,-36.8410295361506));
#21813=CARTESIAN_POINT('Ctrl Pts',(-22.6534713810948,-49.9304402047265,
-36.8936790438815));
#21814=CARTESIAN_POINT('Ctrl Pts',(-22.4617761160207,-49.0073231633699,
-36.9463285516123));
#21815=CARTESIAN_POINT('Ctrl Pts',(-21.9270453071541,-48.3737048044754,
-36.9989780593431));
#21816=CARTESIAN_POINT('Ctrl Pts',(-21.3923144982876,-47.7400864455809,
-37.0516275670739));
#21817=CARTESIAN_POINT('Ctrl Pts',(-20.5145481456286,-47.3959667691485,
-37.1042770748047));
#21818=CARTESIAN_POINT('Ctrl Pts',(-19.6916682754265,-47.4973471716827,
-37.1569265825355));
#21819=CARTESIAN_POINT('Ctrl Pts',(-18.8687884052244,-47.598727574217,-37.2095760902664));
#21820=CARTESIAN_POINT('Ctrl Pts',(-18.1007950174792,-48.1456080557178,
-37.2622255979972));
#21821=CARTESIAN_POINT('Ctrl Pts',(-17.7358462391789,-48.8900687176614,
-37.314875105728));
#21822=CARTESIAN_POINT('Ctrl Pts',(-17.5682348885884,-49.2319798691139,
-37.3390556363214));
#21823=CARTESIAN_POINT('Ctrl Pts',(-17.4856386516788,-49.6155670561907,
-37.3632361669147));
#21824=CARTESIAN_POINT('Ctrl Pts',(-17.4863844696326,-49.9994585735565,
-37.387416697508));
#21825=CARTESIAN_POINT('Origin',(-20.,-50.,-32.));
#21826=CARTESIAN_POINT('',(-17.4818816223345,-50.0021988885187,-38.387416697508));
#21827=CARTESIAN_POINT('',(-17.4784634893366,-49.9997267145485,-38.112583302492));
#21828=CARTESIAN_POINT('',(-17.4825,-50.,-32.));
#21829=CARTESIAN_POINT('Ctrl Pts',(-17.4784634893366,-49.9997267145485,
-38.112583302492));
#21830=CARTESIAN_POINT('Ctrl Pts',(-17.4784401902979,-49.9847350675764,
-38.1116313433196));
#21831=CARTESIAN_POINT('Ctrl Pts',(-17.478562451161,-49.9697438107687,-38.1106793841472));
#21832=CARTESIAN_POINT('Ctrl Pts',(-17.4788314347168,-49.9547551871231,
-38.1097274249749));
#21833=CARTESIAN_POINT('Ctrl Pts',(-17.493707967459,-49.1257872235762,-38.057077917244));
#21834=CARTESIAN_POINT('Ctrl Pts',(-17.9573808053747,-48.3048735931184,
-38.0044284095132));
#21835=CARTESIAN_POINT('Ctrl Pts',(-18.659650665377,-47.8641626851468,-37.9517789017824));
#21836=CARTESIAN_POINT('Ctrl Pts',(-19.3619205253793,-47.4234517771752,
-37.8991293940516));
#21837=CARTESIAN_POINT('Ctrl Pts',(-20.3027874074683,-47.3629435916899,
-37.8464798863208));
#21838=CARTESIAN_POINT('Ctrl Pts',(-21.055723745345,-47.7100687559622,-37.7938303785899));
#21839=CARTESIAN_POINT('Ctrl Pts',(-21.8086600832218,-48.0571939202345,
-37.7411808708591));
#21840=CARTESIAN_POINT('Ctrl Pts',(-22.3736658768864,-48.8119524342645,
-37.6885313631283));
#21841=CARTESIAN_POINT('Ctrl Pts',(-22.4946042778578,-49.6321859220406,
-37.6358818553975));
#21842=CARTESIAN_POINT('Ctrl Pts',(-22.6155426788291,-50.4524194098166,
-37.5832323476666));
#21843=CARTESIAN_POINT('Ctrl Pts',(-22.2924136871073,-51.3381278713388,
-37.5305828399358));
#21844=CARTESIAN_POINT('Ctrl Pts',(-21.6717029494111,-51.8877888851473,
-37.477933332205));
#21845=CARTESIAN_POINT('Ctrl Pts',(-21.0509922117148,-52.4374498989559,
-37.4252838244742));
#21846=CARTESIAN_POINT('Ctrl Pts',(-20.132699728044,-52.6510634650507,-37.3726343167434));
#21847=CARTESIAN_POINT('Ctrl Pts',(-19.3331194154503,-52.4317911011418,
-37.3199848090125));
#21848=CARTESIAN_POINT('Ctrl Pts',(-18.5335391028565,-52.212518737233,-37.2673353012817));
#21849=CARTESIAN_POINT('Ctrl Pts',(-17.8526709613398,-51.5603604433206,
-37.2146857935509));
#21850=CARTESIAN_POINT('Ctrl Pts',(-17.5991762171207,-50.7709622749911,
-37.1620362858201));
#21851=CARTESIAN_POINT('Ctrl Pts',(-17.5198081349998,-50.5238052033796,
-37.145551958044));
#21852=CARTESIAN_POINT('Ctrl Pts',(-17.4823349702594,-50.2631946663995,
-37.129067630268));
#21853=CARTESIAN_POINT('Ctrl Pts',(-17.4843373872682,-50.0020238412825,
-37.112583302492));
#21854=CARTESIAN_POINT('Ctrl Pts',(-17.4863844696326,-49.9994585735565,
-37.387416697508));
#21855=CARTESIAN_POINT('Ctrl Pts',(-17.4872625593087,-50.4514337189728,
-37.4158856746455));
#21856=CARTESIAN_POINT('Ctrl Pts',(-17.6036657291937,-50.9038307136114,
-37.444354651783));
#21857=CARTESIAN_POINT('Ctrl Pts',(-17.8328635601392,-51.2891312519096,
-37.4728236289205));
#21858=CARTESIAN_POINT('Ctrl Pts',(-18.2567338282551,-52.001692281828,-37.5254731366513));
#21859=CARTESIAN_POINT('Ctrl Pts',(-19.0663785333421,-52.4847734992787,
-37.5781226443822));
#21860=CARTESIAN_POINT('Ctrl Pts',(-19.8947575738855,-52.5193775844509,
-37.630772152113));
#21861=CARTESIAN_POINT('Ctrl Pts',(-20.7231366144289,-52.5539816696232,
-37.6834216598438));
#21862=CARTESIAN_POINT('Ctrl Pts',(-21.5702499904287,-52.1401086225171,
-37.7360711675746));
#21863=CARTESIAN_POINT('Ctrl Pts',(-22.0520717080468,-51.4653810891725,
-37.7887206753054));
#21864=CARTESIAN_POINT('Ctrl Pts',(-22.5338934256649,-50.7906535558279,
-37.8413701830363));
#21865=CARTESIAN_POINT('Ctrl Pts',(-22.6504234849012,-49.8550715362449,
-37.8940196907671));
#21866=CARTESIAN_POINT('Ctrl Pts',(-22.3488348086601,-49.0827677205198,
-37.9466691984979));
#21867=CARTESIAN_POINT('Ctrl Pts',(-22.047246132419,-48.3104639047946,-37.9993187062287));
#21868=CARTESIAN_POINT('Ctrl Pts',(-21.3275387207004,-47.7014382929273,
-38.0519682139596));
#21869=CARTESIAN_POINT('Ctrl Pts',(-20.5159808782079,-47.5317817744353,
-38.1046177216904));
#21870=CARTESIAN_POINT('Ctrl Pts',(-19.7044230357155,-47.3621252559433,
-38.1572672294212));
#21871=CARTESIAN_POINT('Ctrl Pts',(-18.801014762449,-47.6318378308265,-38.209916737152));
#21872=CARTESIAN_POINT('Ctrl Pts',(-18.2153026720781,-48.2186526109762,
-38.2625662448829));
#21873=CARTESIAN_POINT('Ctrl Pts',(-17.7523263927637,-48.6825005117228,
-38.3041830624246));
#21874=CARTESIAN_POINT('Ctrl Pts',(-17.4878503825531,-49.3444775574439,
-38.3457998799663));
#21875=CARTESIAN_POINT('Ctrl Pts',(-17.4818816223345,-50.0021988885187,
-38.387416697508));
#21876=CARTESIAN_POINT('Origin',(-20.,-50.,-32.));
#21877=CARTESIAN_POINT('',(-17.4798421274757,-49.9984351524252,-39.387416697508));
#21878=CARTESIAN_POINT('',(-17.4850545138796,-49.9982392692185,-39.112583302492));
#21879=CARTESIAN_POINT('',(-17.4825,-50.,-32.));
#21880=CARTESIAN_POINT('',(-21.913465996665,-48.364012796625,-40.));
#21881=CARTESIAN_POINT('Ctrl Pts',(-17.4798421274757,-49.9984351524252,
-39.387416697508));
#21882=CARTESIAN_POINT('Ctrl Pts',(-17.4853147276126,-50.7276238536423,
-39.4336626084795));
#21883=CARTESIAN_POINT('Ctrl Pts',(-17.8198670584883,-51.4610375097699,
-39.4799085194511));
#21884=CARTESIAN_POINT('Ctrl Pts',(-18.3773138107771,-51.9298785803434,
-39.5261544304226));
#21885=CARTESIAN_POINT('Ctrl Pts',(-19.0119493164378,-52.4636393183443,
-39.5788039381534));
#21886=CARTESIAN_POINT('Ctrl Pts',(-19.9354805710936,-52.6544848107208,
-39.6314534458842));
#21887=CARTESIAN_POINT('Ctrl Pts',(-20.7291492614058,-52.4142811819356,
-39.6841029536151));
#21888=CARTESIAN_POINT('Ctrl Pts',(-21.522817951718,-52.1740775531505,-39.7367524613459));
#21889=CARTESIAN_POINT('Ctrl Pts',(-22.1866240776865,-51.5028248032037,
-39.7894019690767));
#21890=CARTESIAN_POINT('Ctrl Pts',(-22.4195849355037,-50.7085554156277,
-39.8420514768075));
#21891=CARTESIAN_POINT('Ctrl Pts',(-22.6525457933209,-49.9142860280518,
-39.8947009845383));
#21892=CARTESIAN_POINT('Ctrl Pts',(-22.4546613829867,-48.9970000028465,
-39.9473504922692));
#21893=CARTESIAN_POINT('Ctrl Pts',(-21.913465996665,-48.364012796625,-40.));
#21894=CARTESIAN_POINT('',(-18.0829275241642,-48.361458825814,-40.));
#21895=CARTESIAN_POINT('Origin',(-20.,-50.,-40.));
#21896=CARTESIAN_POINT('Ctrl Pts',(-18.0829200279321,-48.3614535172687,
-40.));
#21897=CARTESIAN_POINT('Ctrl Pts',(-18.6057519481588,-47.7526827191803,
-39.9490537266973));
#21898=CARTESIAN_POINT('Ctrl Pts',(-19.4454475058209,-47.4126382937553,
-39.8981074533947));
#21899=CARTESIAN_POINT('Ctrl Pts',(-20.2440955071633,-47.4904273239402,
-39.847161180092));
#21900=CARTESIAN_POINT('Ctrl Pts',(-21.0694438868393,-47.5708169948738,
-39.7945116723612));
#21901=CARTESIAN_POINT('Ctrl Pts',(-21.8509542298921,-48.0974451260636,
-39.7418621646304));
#21902=CARTESIAN_POINT('Ctrl Pts',(-22.2348330746457,-48.8322008546483,
-39.6892126568995));
#21903=CARTESIAN_POINT('Ctrl Pts',(-22.6187119193993,-49.566956583233,-39.6365631491687));
#21904=CARTESIAN_POINT('Ctrl Pts',(-22.6049592658536,-50.5098399092124,
-39.5839136414379));
#21905=CARTESIAN_POINT('Ctrl Pts',(-22.199562657414,-51.2330949537652,-39.5312641337071));
#21906=CARTESIAN_POINT('Ctrl Pts',(-21.7941660489743,-51.9563499983181,
-39.4786146259763));
#21907=CARTESIAN_POINT('Ctrl Pts',(-20.9971254856407,-52.4599767614444,
-39.4259651182454));
#21908=CARTESIAN_POINT('Ctrl Pts',(-20.1698912582501,-52.515821381016,-39.3733156105146));
#21909=CARTESIAN_POINT('Ctrl Pts',(-19.3426570308596,-52.5716660005875,
-39.3206661027838));
#21910=CARTESIAN_POINT('Ctrl Pts',(-18.485229139412,-52.1797284766043,-39.268016595053));
#21911=CARTESIAN_POINT('Ctrl Pts',(-17.9862471478564,-51.517608519283,-39.2153670873222));
#21912=CARTESIAN_POINT('Ctrl Pts',(-17.661538460383,-51.0867390571978,-39.1811058257121));
#21913=CARTESIAN_POINT('Ctrl Pts',(-17.488619258549,-50.5414566457736,-39.146844564102));
#21914=CARTESIAN_POINT('Ctrl Pts',(-17.4850545138796,-49.9982392692185,
-39.112583302492));
#21915=CARTESIAN_POINT('Origin',(-20.,-50.,-42.2084234471774));
#21916=CARTESIAN_POINT('',(-16.9217888153016,-49.9991816123293,-25.7915765528225));
#21917=CARTESIAN_POINT('',(-16.9314304880168,-49.9996668086012,-25.7084234471775));
#21918=CARTESIAN_POINT('',(-16.9265,-49.9999999999998,-42.2084234471774));
#21919=CARTESIAN_POINT('',(-20.7937992825329,-52.9692229537457,-25.));
#21920=CARTESIAN_POINT('Ctrl Pts',(-16.9314304880168,-49.9996668086012,
-25.7084234471775));
#21921=CARTESIAN_POINT('Ctrl Pts',(-16.9311124941626,-49.5044898991504,
-25.6828803290416));
#21922=CARTESIAN_POINT('Ctrl Pts',(-17.2773642933051,-47.9891814869228,
-25.6046877031749));
#21923=CARTESIAN_POINT('Ctrl Pts',(-19.6484750587118,-46.3913836024568,
-25.4738455695774));
#21924=CARTESIAN_POINT('Ctrl Pts',(-22.8319253439964,-47.7313330083366,
-25.3158970463849));
#21925=CARTESIAN_POINT('Ctrl Pts',(-23.4429084618352,-51.1345418770559,
-25.1579485231925));
#21926=CARTESIAN_POINT('Ctrl Pts',(-21.7760378723045,-52.706628901368,-25.0526495077308));
#21927=CARTESIAN_POINT('Ctrl Pts',(-20.7937992825329,-52.9692229537457,
-25.));
#21928=CARTESIAN_POINT('',(-19.2062007174672,-52.9692229537457,-25.));
#21929=CARTESIAN_POINT('Origin',(-20.,-50.,-25.));
#21930=CARTESIAN_POINT('Ctrl Pts',(-16.9217888153016,-49.9991816123293,
-25.7915765528225));
#21931=CARTESIAN_POINT('Ctrl Pts',(-16.9216327964757,-49.9546737426535,
-25.7892620061076));
#21932=CARTESIAN_POINT('Ctrl Pts',(-16.942593390011,-48.897887811184,-25.7342979516619));
#21933=CARTESIAN_POINT('Ctrl Pts',(-18.1518496079148,-46.8799270552508,
-25.6266843894854));
#21934=CARTESIAN_POINT('Ctrl Pts',(-21.6024144605454,-46.7464740570925,
-25.468735866293));
#21935=CARTESIAN_POINT('Ctrl Pts',(-23.6000558022285,-49.5638703006617,
-25.3107873431004));
#21936=CARTESIAN_POINT('Ctrl Pts',(-22.3474160567079,-52.7401230784006,
-25.1545420543362));
#21937=CARTESIAN_POINT('Ctrl Pts',(-20.1513508010164,-53.2252259242231,
-25.0509462733027));
#21938=CARTESIAN_POINT('Ctrl Pts',(-19.2043345174297,-52.9742970828256,
-25.));
#21939=CARTESIAN_POINT('Origin',(-20.,-50.,-42.2084234471774));
#21940=CARTESIAN_POINT('',(-16.9301482556011,-49.9981345312788,-26.7915765528225));
#21941=CARTESIAN_POINT('',(-16.9249665978426,-50.0025583315037,-26.7084234471774));
#21942=CARTESIAN_POINT('',(-16.9265,-49.9999999999998,-42.2084234471774));
#21943=CARTESIAN_POINT('Ctrl Pts',(-16.9249665978426,-50.0025583315037,
-26.7084234471774));
#21944=CARTESIAN_POINT('Ctrl Pts',(-16.9323545095395,-49.1738259014586,
-26.6654440420932));
#21945=CARTESIAN_POINT('Ctrl Pts',(-17.703989360689,-47.3177697473349,-26.5698151292781));
#21946=CARTESIAN_POINT('Ctrl Pts',(-20.8329798277681,-46.4704999500574,
-26.4215367087322));
#21947=CARTESIAN_POINT('Ctrl Pts',(-23.4108310490853,-48.7680163172086,
-26.2635881855398));
#21948=CARTESIAN_POINT('Ctrl Pts',(-22.8961088969807,-52.1826319253429,
-26.1056396623473));
#21949=CARTESIAN_POINT('Ctrl Pts',(-19.7557254019559,-53.6181282017024,
-25.9476911391548));
#21950=CARTESIAN_POINT('Ctrl Pts',(-17.3086034982695,-52.0718620980463,
-25.8152857340982));
#21951=CARTESIAN_POINT('Ctrl Pts',(-16.931767943501,-50.5251491774573,-25.7355298367724));
#21952=CARTESIAN_POINT('Ctrl Pts',(-16.9314304880168,-49.9996668086012,
-25.7084234471775));
#21953=CARTESIAN_POINT('Ctrl Pts',(-16.9301482556011,-49.9981345312788,
-26.7915765528225));
#21954=CARTESIAN_POINT('Ctrl Pts',(-16.9280041631807,-49.6156590014734,
-26.7718257191592));
#21955=CARTESIAN_POINT('Ctrl Pts',(-17.1709938395466,-48.2162502496147,
-26.6994253777651));
#21956=CARTESIAN_POINT('Ctrl Pts',(-19.2579268207016,-46.4502608973225,
-26.5743755286402));
#21957=CARTESIAN_POINT('Ctrl Pts',(-22.5667151646459,-47.4380997591695,
-26.4164270054477));
#21958=CARTESIAN_POINT('Ctrl Pts',(-23.5483399170972,-50.748751349135,-26.2584784822553));
#21959=CARTESIAN_POINT('Ctrl Pts',(-21.312794804531,-53.3805016203859,-26.1005299590628));
#21960=CARTESIAN_POINT('Ctrl Pts',(-17.9371758478695,-52.9536638884015,
-25.9448959825852));
#21961=CARTESIAN_POINT('Ctrl Pts',(-16.9251817913301,-50.9671041306423,
-25.8419115138385));
#21962=CARTESIAN_POINT('Ctrl Pts',(-16.9217888153016,-49.9991816123293,
-25.7915765528225));
#21963=CARTESIAN_POINT('Origin',(-20.,-50.,-42.2084234471774));
#21964=CARTESIAN_POINT('',(-16.928225056676,-50.0025926095194,-27.7915765528225));
#21965=CARTESIAN_POINT('',(-16.9239287305948,-49.9977320013947,-27.7084234471775));
#21966=CARTESIAN_POINT('',(-16.9265,-49.9999999999998,-42.2084234471774));
#21967=CARTESIAN_POINT('Ctrl Pts',(-16.9239287305948,-49.9977320013947,
-27.7084234471775));
#21968=CARTESIAN_POINT('Ctrl Pts',(-16.9226896332749,-49.8481151515914,
-27.7006572628756));
#21969=CARTESIAN_POINT('Ctrl Pts',(-17.0003510257386,-48.6854876981218,
-27.640241570843));
#21970=CARTESIAN_POINT('Ctrl Pts',(-18.4816794190144,-46.7066668978831,
-27.5271763710795));
#21971=CARTESIAN_POINT('Ctrl Pts',(-21.9276633145204,-46.9282819155376,
-27.369227847887));
#21972=CARTESIAN_POINT('Ctrl Pts',(-23.6258941273587,-49.9349295156179,
-27.2112793246946));
#21973=CARTESIAN_POINT('Ctrl Pts',(-22.0366357822403,-53.0005761032442,
-27.0533308015021));
#21974=CARTESIAN_POINT('Ctrl Pts',(-18.6008241624394,-53.3456884935447,
-26.8953822783096));
#21975=CARTESIAN_POINT('Ctrl Pts',(-17.0233222448715,-51.3888911243564,
-26.7804131602014));
#21976=CARTESIAN_POINT('Ctrl Pts',(-16.9233043630045,-50.1890180474854,
-26.718093549824));
#21977=CARTESIAN_POINT('Ctrl Pts',(-16.9249665978426,-50.0025583315037,
-26.7084234471774));
#21978=CARTESIAN_POINT('Ctrl Pts',(-16.928225056676,-50.0025926095194,-27.7915765528225));
#21979=CARTESIAN_POINT('Ctrl Pts',(-16.9340843879266,-49.2836004587027,
-27.7543894322109));
#21980=CARTESIAN_POINT('Ctrl Pts',(-17.5432834505634,-47.5377126858431,
-27.6645528038683));
#21981=CARTESIAN_POINT('Ctrl Pts',(-20.4434363389617,-46.4007362339102,
-27.522066667795));
#21982=CARTESIAN_POINT('Ctrl Pts',(-23.2562593438794,-48.403719623335,-27.3641181446025));
#21983=CARTESIAN_POINT('Ctrl Pts',(-23.1167310200335,-51.8540021340239,
-27.2061696214101));
#21984=CARTESIAN_POINT('Ctrl Pts',(-20.1513575038949,-53.623316794304,-27.0482210982176));
#21985=CARTESIAN_POINT('Ctrl Pts',(-17.4367210524572,-52.2970305039663,
-26.9100234086884));
#21986=CARTESIAN_POINT('Ctrl Pts',(-16.9337196389114,-50.635218413832,-26.8244752268901));
#21987=CARTESIAN_POINT('Ctrl Pts',(-16.9301482556011,-49.9981345312788,
-26.7915765528225));
#21988=CARTESIAN_POINT('Origin',(-20.,-50.,-42.2084234471774));
#21989=CARTESIAN_POINT('',(-16.9217184048747,-49.9993152064879,-28.7915765528225));
#21990=CARTESIAN_POINT('',(-16.9313402641813,-49.9996515904955,-28.7084234471775));
#21991=CARTESIAN_POINT('',(-16.9265,-49.9999999999998,-42.2084234471774));
#21992=CARTESIAN_POINT('Ctrl Pts',(-16.9313402641813,-49.9996515904955,
-28.7084234471775));
#21993=CARTESIAN_POINT('Ctrl Pts',(-16.9308409783865,-49.5111295368377,
-28.6832209759272));
#21994=CARTESIAN_POINT('Ctrl Pts',(-17.2704954611012,-48.0027107711033,
-28.6053689969462));
#21995=CARTESIAN_POINT('Ctrl Pts',(-19.6259746610823,-46.3928619507583,
-28.4748675102343));
#21996=CARTESIAN_POINT('Ctrl Pts',(-22.8159749872838,-47.7149125425452,
-28.3169189870419));
#21997=CARTESIAN_POINT('Ctrl Pts',(-23.4528164464309,-51.1087824216521,
-28.1589704638493));
#21998=CARTESIAN_POINT('Ctrl Pts',(-20.9590942265365,-53.4973530261498,
-28.0010219406569));
#21999=CARTESIAN_POINT('Ctrl Pts',(-17.7611610467444,-52.7534485267535,
-27.8508396017662));
#22000=CARTESIAN_POINT('Ctrl Pts',(-16.9310898799582,-50.8624167937153,
-27.7533067706064));
#22001=CARTESIAN_POINT('Ctrl Pts',(-16.9239287305948,-49.9977320013947,
-27.7084234471775));
#22002=CARTESIAN_POINT('Ctrl Pts',(-16.9217184048747,-49.9993152064879,
-28.7915765528225));
#22003=CARTESIAN_POINT('Ctrl Pts',(-16.9216027631545,-49.9613596580176,
-28.7896026529933));
#22004=CARTESIAN_POINT('Ctrl Pts',(-16.9393663574583,-48.9111326917697,
-28.7349792454332));
#22005=CARTESIAN_POINT('Ctrl Pts',(-18.1318616862451,-46.8917215466485,
-28.6277063301423));
#22006=CARTESIAN_POINT('Ctrl Pts',(-21.5814746967481,-46.7365243250642,
-28.4697578069498));
#22007=CARTESIAN_POINT('Ctrl Pts',(-23.5972126982202,-49.5402212417787,
-28.3118092837573));
#22008=CARTESIAN_POINT('Ctrl Pts',(-22.3514673502323,-52.7607855790929,
-28.1538607605649));
#22009=CARTESIAN_POINT('Ctrl Pts',(-18.9737180729577,-53.4782295892619,
-27.9959122373724));
#22010=CARTESIAN_POINT('Ctrl Pts',(-17.1026437687264,-51.6156340543063,
-27.8751508347916));
#22011=CARTESIAN_POINT('Ctrl Pts',(-16.9257887495201,-50.3015492049395,
-27.8070389399417));
#22012=CARTESIAN_POINT('Ctrl Pts',(-16.928225056676,-50.0025926095194,-27.7915765528225));
#22013=CARTESIAN_POINT('Origin',(-20.,-50.,-42.2084234471774));
#22014=CARTESIAN_POINT('',(-16.9300226261573,-49.9980579824143,-29.7915765528225));
#22015=CARTESIAN_POINT('',(-16.9251595829395,-50.0025957433342,-29.7084234471775));
#22016=CARTESIAN_POINT('',(-16.9265,-49.9999999999998,-42.2084234471774));
#22017=CARTESIAN_POINT('Ctrl Pts',(-16.9251595829395,-50.0025957433342,
-29.7084234471775));
#22018=CARTESIAN_POINT('Ctrl Pts',(-16.9325403191697,-49.1802996882788,
-29.6657846889788));
#22019=CARTESIAN_POINT('Ctrl Pts',(-17.6939854946978,-47.3305806954569,
-29.5704964230493));
#22020=CARTESIAN_POINT('Ctrl Pts',(-20.810310380068,-46.4652104819412,-29.4225586493892));
#22021=CARTESIAN_POINT('Ctrl Pts',(-23.4028289883847,-48.7461679840765,
-29.2646101261966));
#22022=CARTESIAN_POINT('Ctrl Pts',(-22.9101060454574,-52.163936841271,-29.1066616030042));
#22023=CARTESIAN_POINT('Ctrl Pts',(-19.7788784576719,-53.6197299780505,
-28.9487130798117));
#22024=CARTESIAN_POINT('Ctrl Pts',(-17.3157682680493,-52.0849998655991,
-28.8159670278695));
#22025=CARTESIAN_POINT('Ctrl Pts',(-16.9318840170255,-50.5316820606504,
-28.7358704836581));
#22026=CARTESIAN_POINT('Ctrl Pts',(-16.9313402641813,-49.9996515904955,
-28.7084234471775));
#22027=CARTESIAN_POINT('Ctrl Pts',(-16.9300226261573,-49.9980579824143,
-29.7915765528225));
#22028=CARTESIAN_POINT('Ctrl Pts',(-16.9278229920328,-49.6222178059028,
-29.7721663660449));
#22029=CARTESIAN_POINT('Ctrl Pts',(-17.1652526647347,-48.2296053591559,
-29.7001066715364));
#22030=CARTESIAN_POINT('Ctrl Pts',(-19.2351493773684,-46.4550967253995,
-29.5753974692971));
#22031=CARTESIAN_POINT('Ctrl Pts',(-22.5502120400548,-47.4216760770047,
-29.4174489461046));
#22032=CARTESIAN_POINT('Ctrl Pts',(-23.5530750072187,-50.7259433133794,
-29.2595004229121));
#22033=CARTESIAN_POINT('Ctrl Pts',(-21.3344729272248,-53.3720198261462,
-29.1015518997197));
#22034=CARTESIAN_POINT('Ctrl Pts',(-17.9487915178527,-52.9659277200364,
-28.9455772763565));
#22035=CARTESIAN_POINT('Ctrl Pts',(-16.9246872558677,-50.9737418027382,
-28.8422521607241));
#22036=CARTESIAN_POINT('Ctrl Pts',(-16.9217184048747,-49.9993152064879,
-28.7915765528225));
#22037=CARTESIAN_POINT('Origin',(-20.,-50.,-42.2084234471774));
#22038=CARTESIAN_POINT('',(-16.9284011455975,-50.0025559503523,-30.7915765528225));
#22039=CARTESIAN_POINT('',(-16.9237529572543,-49.9977977476302,-30.7084234471775));
#22040=CARTESIAN_POINT('',(-16.9265,-49.9999999999998,-42.2084234471774));
#22041=CARTESIAN_POINT('Ctrl Pts',(-16.9237529572543,-49.9977977476302,
-30.7084234471775));
#22042=CARTESIAN_POINT('Ctrl Pts',(-16.9225921162906,-49.8547648374716,
-30.7009979097613));
#22043=CARTESIAN_POINT('Ctrl Pts',(-16.9963970139262,-48.6987851336448,
-30.6409228646142));
#22044=CARTESIAN_POINT('Ctrl Pts',(-18.4605641466087,-46.7164840335274,
-30.5281983117364));
#22045=CARTESIAN_POINT('Ctrl Pts',(-21.9079002499127,-46.9159674960896,
-30.370249788544));
#22046=CARTESIAN_POINT('Ctrl Pts',(-23.6254012227827,-49.9116494333404,
-30.2123012653514));
#22047=CARTESIAN_POINT('Ctrl Pts',(-22.0558611685522,-52.9874361423172,
-30.054352742159));
#22048=CARTESIAN_POINT('Ctrl Pts',(-18.6223343189813,-53.3546053598246,
-29.8964042189665));
#22049=CARTESIAN_POINT('Ctrl Pts',(-17.0275920921308,-51.402205940021,-29.7810944539727));
#22050=CARTESIAN_POINT('Ctrl Pts',(-16.9234267298995,-50.1956548331446,
-29.7184341967097));
#22051=CARTESIAN_POINT('Ctrl Pts',(-16.9251595829395,-50.0025957433342,
-29.7084234471775));
#22052=CARTESIAN_POINT('Ctrl Pts',(-16.9284011455975,-50.0025559503523,
-30.7915765528225));
#22053=CARTESIAN_POINT('Ctrl Pts',(-16.9341000870249,-49.2900464772943,
-30.7547300790965));
#22054=CARTESIAN_POINT('Ctrl Pts',(-17.534439658132,-47.5507753552286,-30.6652340976396));
#22055=CARTESIAN_POINT('Ctrl Pts',(-20.4203163327858,-46.3979630926968,
-30.5230886084519));
#22056=CARTESIAN_POINT('Ctrl Pts',(-23.2459424988316,-48.3828441647573,
-30.3651400852595));
#22057=CARTESIAN_POINT('Ctrl Pts',(-23.1285713220653,-51.8339512490605,
-30.207191562067));
#22058=CARTESIAN_POINT('Ctrl Pts',(-20.1746196787779,-53.6222705129474,
-30.0492430388745));
#22059=CARTESIAN_POINT('Ctrl Pts',(-17.4448109217873,-52.3102153453405,
-29.9107047024597));
#22060=CARTESIAN_POINT('Ctrl Pts',(-16.9337894288924,-50.6416722040218,
-29.8248158737757));
#22061=CARTESIAN_POINT('Ctrl Pts',(-16.9300226261573,-49.9980579824143,
-29.7915765528225));
#22062=CARTESIAN_POINT('Origin',(-20.,-50.,-42.2084234471774));
#22063=CARTESIAN_POINT('',(-16.9216591696857,-49.9994310993742,-31.7915765528225));
#22064=CARTESIAN_POINT('',(-16.9313143876478,-49.999546673736,-31.7084234471775));
#22065=CARTESIAN_POINT('',(-16.9265,-49.9999999999998,-42.2084234471774));
#22066=CARTESIAN_POINT('Ctrl Pts',(-16.9313143876478,-49.999546673736,-31.7084234471775));
#22067=CARTESIAN_POINT('Ctrl Pts',(-16.9306732233893,-49.5176378400166,
-31.6835616228129));
#22068=CARTESIAN_POINT('Ctrl Pts',(-17.2638485165257,-48.0160365216701,
-31.6060502907175));
#22069=CARTESIAN_POINT('Ctrl Pts',(-19.6028209425392,-46.3953379291391,
-31.4758894508912));
#22070=CARTESIAN_POINT('Ctrl Pts',(-22.8012443962967,-47.696878274818,-31.3179409276987));
#22071=CARTESIAN_POINT('Ctrl Pts',(-23.459864751929,-51.0865890424386,-31.1599924045063));
#22072=CARTESIAN_POINT('Ctrl Pts',(-20.9815309640172,-53.4911225723918,
-31.0020438813138));
#22073=CARTESIAN_POINT('Ctrl Pts',(-17.7716227612056,-52.7661266417806,
-30.8515208955375));
#22074=CARTESIAN_POINT('Ctrl Pts',(-16.9308228613352,-50.8689153140057,
-30.7536474174921));
#22075=CARTESIAN_POINT('Ctrl Pts',(-16.9237529572543,-49.9977977476302,
-30.7084234471775));
#22076=CARTESIAN_POINT('Ctrl Pts',(-16.9216591696857,-49.9994310993742,
-31.7915765528225));
#22077=CARTESIAN_POINT('Ctrl Pts',(-16.9215784879871,-49.9680273721396,
-31.7899432998789));
#22078=CARTESIAN_POINT('Ctrl Pts',(-16.936183371105,-48.9243706066136,-31.7356605392045));
#22079=CARTESIAN_POINT('Ctrl Pts',(-18.1119419466013,-46.9037809366621,
-31.6287282707992));
#22080=CARTESIAN_POINT('Ctrl Pts',(-21.5604873228824,-46.7264369539744,
-31.4707797476067));
#22081=CARTESIAN_POINT('Ctrl Pts',(-23.5941863035827,-49.5171330241987,
-31.3128312244142));
#22082=CARTESIAN_POINT('Ctrl Pts',(-22.3691458750596,-52.7456298956467,
-31.1548827012218));
#22083=CARTESIAN_POINT('Ctrl Pts',(-18.9960729359346,-53.4847476452704,
-30.9969341780293));
#22084=CARTESIAN_POINT('Ctrl Pts',(-17.1077658789735,-51.6289846027671,
-30.8758321285629));
#22085=CARTESIAN_POINT('Ctrl Pts',(-16.9259569343593,-50.3081431692316,
-30.8073795868273));
#22086=CARTESIAN_POINT('Ctrl Pts',(-16.9284011455975,-50.0025559503523,
-30.7915765528225));
#22087=CARTESIAN_POINT('Origin',(-20.,-50.,-42.2084234471774));
#22088=CARTESIAN_POINT('',(-16.929891726575,-49.9979840334756,-32.7915765528225));
#22089=CARTESIAN_POINT('',(-16.9253537624756,-50.0026288890115,-32.7084234471775));
#22090=CARTESIAN_POINT('',(-16.9265,-49.9999999999998,-42.2084234471774));
#22091=CARTESIAN_POINT('Ctrl Pts',(-16.9253537624756,-50.0026288890115,
-32.7084234471775));
#22092=CARTESIAN_POINT('Ctrl Pts',(-16.9327154506849,-49.1867693143368,
-32.6661253358645));
#22093=CARTESIAN_POINT('Ctrl Pts',(-17.6840555158499,-47.3434039731563,
-32.5711777168206));
#22094=CARTESIAN_POINT('Ctrl Pts',(-20.7875967978108,-46.460080349377,-32.423580590046));
#22095=CARTESIAN_POINT('Ctrl Pts',(-23.3947079863477,-48.724344272064,-32.2656320668535));
#22096=CARTESIAN_POINT('Ctrl Pts',(-22.9239406890394,-52.1452064459554,
-32.1076835436611));
#22097=CARTESIAN_POINT('Ctrl Pts',(-19.8021252966153,-53.6210751788038,
-31.9497350204686));
#22098=CARTESIAN_POINT('Ctrl Pts',(-17.3228655042439,-52.0982946435502,
-31.8166483216408));
#22099=CARTESIAN_POINT('Ctrl Pts',(-16.9320310071983,-50.5381688555359,
-31.7362111305437));
#22100=CARTESIAN_POINT('Ctrl Pts',(-16.9313143876478,-49.999546673736,-31.7084234471775));
#22101=CARTESIAN_POINT('Ctrl Pts',(-16.929891726575,-49.9979840334756,-32.7915765528225));
#22102=CARTESIAN_POINT('Ctrl Pts',(-16.9276422677924,-49.6287794061046,
-32.7725070129305));
#22103=CARTESIAN_POINT('Ctrl Pts',(-17.1595661457499,-48.2429604363447,
-32.7007879653077));
#22104=CARTESIAN_POINT('Ctrl Pts',(-19.2124033263834,-46.4600809075787,
-32.576419409954));
#22105=CARTESIAN_POINT('Ctrl Pts',(-22.533604054109,-47.405354321264,-32.4184708867615));
#22106=CARTESIAN_POINT('Ctrl Pts',(-23.5576630420582,-50.7031140592781,
-32.2605223635691));
#22107=CARTESIAN_POINT('Ctrl Pts',(-21.3560971512034,-53.3633816639922,
-32.1025738403766));
#22108=CARTESIAN_POINT('Ctrl Pts',(-17.9604781864533,-52.9781979806717,
-31.9462585701277));
#22109=CARTESIAN_POINT('Ctrl Pts',(-16.9241793415355,-50.9803572664544,
-31.8425928076097));
#22110=CARTESIAN_POINT('Ctrl Pts',(-16.9216591696857,-49.9994310993742,
-31.7915765528225));
#22111=CARTESIAN_POINT('Origin',(-20.,-50.,-42.2084234471774));
#22112=CARTESIAN_POINT('',(-16.9285739275939,-50.0025153259756,-33.7915765528225));
#22113=CARTESIAN_POINT('',(-16.9235810583994,-49.9978675316839,-33.7084234471775));
#22114=CARTESIAN_POINT('',(-16.9265,-49.9999999999998,-42.2084234471774));
#22115=CARTESIAN_POINT('Ctrl Pts',(-16.9235810583994,-49.9978675316839,
-33.7084234471775));
#22116=CARTESIAN_POINT('Ctrl Pts',(-16.92249854389,-49.861416180346,-33.7013385566469));
#22117=CARTESIAN_POINT('Ctrl Pts',(-16.992489904441,-48.7120794050224,-33.6416041583855));
#22118=CARTESIAN_POINT('Ctrl Pts',(-18.4395124310478,-46.7264364377739,
-33.5292202523933));
#22119=CARTESIAN_POINT('Ctrl Pts',(-21.8880583511222,-46.9037804484265,
-33.3712717292008));
#22120=CARTESIAN_POINT('Ctrl Pts',(-23.6247591869331,-49.8883725592297,
-33.2133232060084));
#22121=CARTESIAN_POINT('Ctrl Pts',(-22.0750011100191,-52.9741738755843,
-33.0553746828159));
#22122=CARTESIAN_POINT('Ctrl Pts',(-18.6439026349568,-53.3633821943561,
-32.8974261596234));
#22123=CARTESIAN_POINT('Ctrl Pts',(-17.0319088216555,-51.4155254718575,
-32.781775747744));
#22124=CARTESIAN_POINT('Ctrl Pts',(-16.9235521748729,-50.2022899522738,
-32.7187748435953));
#22125=CARTESIAN_POINT('Ctrl Pts',(-16.9253537624756,-50.0026288890115,
-32.7084234471775));
#22126=CARTESIAN_POINT('Ctrl Pts',(-16.9285739275939,-50.0025153259756,
-33.7915765528225));
#22127=CARTESIAN_POINT('Ctrl Pts',(-16.9341074121984,-49.2964924381661,
-33.7550707259821));
#22128=CARTESIAN_POINT('Ctrl Pts',(-17.5256620424174,-47.5638501786645,
-33.6659153914109));
#22129=CARTESIAN_POINT('Ctrl Pts',(-20.3971789948304,-46.3953384975499,
-33.5241105491088));
#22130=CARTESIAN_POINT('Ctrl Pts',(-23.2354918292762,-48.3620353105553,
-33.3661620259163));
#22131=CARTESIAN_POINT('Ctrl Pts',(-23.1402826251531,-51.8138248910362,
-33.2082135027239));
#22132=CARTESIAN_POINT('Ctrl Pts',(-20.1978746721824,-53.6210746078049,
-33.0502649795314));
#22133=CARTESIAN_POINT('Ctrl Pts',(-17.4529646811151,-52.3233915865314,
-32.9113859962309));
#22134=CARTESIAN_POINT('Ctrl Pts',(-16.9338528475042,-50.6481244974432,
-32.8251565206613));
#22135=CARTESIAN_POINT('Ctrl Pts',(-16.929891726575,-49.9979840334756,-32.7915765528225));
#22136=CARTESIAN_POINT('Origin',(-20.,-50.,-42.2084234471774));
#22137=CARTESIAN_POINT('',(-16.9216102653814,-49.9995482667975,-34.7915765528225));
#22138=CARTESIAN_POINT('',(-16.931281743668,-49.9994424172085,-34.7084234471775));
#22139=CARTESIAN_POINT('',(-16.9265,-49.9999999999998,-42.2084234471774));
#22140=CARTESIAN_POINT('Ctrl Pts',(-16.931281743668,-49.9994424172085,-34.7084234471775));
#22141=CARTESIAN_POINT('Ctrl Pts',(-16.9305034541633,-49.5241491461598,
-34.6839022696985));
#22142=CARTESIAN_POINT('Ctrl Pts',(-17.2572599119806,-48.029365460058,-34.6067315844887));
#22143=CARTESIAN_POINT('Ctrl Pts',(-19.5796836009353,-46.3979625246999,
-34.4769113915481));
#22144=CARTESIAN_POINT('Ctrl Pts',(-22.7863983082339,-47.678938967485,-34.3189628683557));
#22145=CARTESIAN_POINT('Ctrl Pts',(-23.4667704139307,-51.0643508565711,
-34.1610143451631));
#22146=CARTESIAN_POINT('Ctrl Pts',(-21.0039272223724,-53.4847481947722,
-34.0030658219707));
#22147=CARTESIAN_POINT('Ctrl Pts',(-17.7821553008139,-52.7787839729962,
-33.8522021893088));
#22148=CARTESIAN_POINT('Ctrl Pts',(-16.9305429668472,-50.8754186474492,
-33.7539880643777));
#22149=CARTESIAN_POINT('Ctrl Pts',(-16.9235810583994,-49.9978675316839,
-33.7084234471775));
#22150=CARTESIAN_POINT('Ctrl Pts',(-16.9216102653814,-49.9995482667975,
-34.7915765528225));
#22151=CARTESIAN_POINT('Ctrl Pts',(-16.9215587791314,-49.9746954627831,
-34.7902839467645));
#22152=CARTESIAN_POINT('Ctrl Pts',(-16.9330440427449,-48.9376047691407,
-34.7363418329757));
#22153=CARTESIAN_POINT('Ctrl Pts',(-18.0921000509396,-46.9159679824036,
-34.6297502114561));
#22154=CARTESIAN_POINT('Ctrl Pts',(-21.5394356106412,-46.7164845512972,
-34.4718016882636));
#22155=CARTESIAN_POINT('Ctrl Pts',(-23.5910117219915,-49.4940647139208,
-34.3138531650712));
#22156=CARTESIAN_POINT('Ctrl Pts',(-22.386726720697,-52.7303610131065,-34.1559046418786));
#22157=CARTESIAN_POINT('Ctrl Pts',(-19.0184691907583,-53.491122021885,-33.9979561186862));
#22158=CARTESIAN_POINT('Ctrl Pts',(-17.1129401986479,-51.642336206118,-33.8765134223342));
#22159=CARTESIAN_POINT('Ctrl Pts',(-16.9261268987933,-50.3147342013879,
-33.8077202337129));
#22160=CARTESIAN_POINT('Ctrl Pts',(-16.9285739275939,-50.0025153259756,
-33.7915765528225));
#22161=CARTESIAN_POINT('Origin',(-20.,-50.,-42.2084234471774));
#22162=CARTESIAN_POINT('',(-16.929755691605,-49.9979131056248,-35.7915765528225));
#22163=CARTESIAN_POINT('',(-16.9255489617634,-50.0026575650068,-35.7084234471774));
#22164=CARTESIAN_POINT('',(-16.9265,-49.9999999999998,-42.2084234471774));
#22165=CARTESIAN_POINT('Ctrl Pts',(-16.9255489617634,-50.0026575650068,
-35.7084234471774));
#22166=CARTESIAN_POINT('Ctrl Pts',(-16.9328792376806,-49.193236061542,-35.6664659827501));
#22167=CARTESIAN_POINT('Ctrl Pts',(-17.6741948420038,-47.3562447964742,
-35.5718590105919));
#22168=CARTESIAN_POINT('Ctrl Pts',(-20.764850743239,-46.4550961664119,-35.4246025307029));
#22169=CARTESIAN_POINT('Ctrl Pts',(-23.38644702166,-48.7025731549433,-35.2666540075105));
#22170=CARTESIAN_POINT('Ctrl Pts',(-22.9376547796718,-52.1263876044256,
-35.108705484318));
#22171=CARTESIAN_POINT('Ctrl Pts',(-19.8253802936868,-53.6222710841349,
-34.9507569611255));
#22172=CARTESIAN_POINT('Ctrl Pts',(-17.330023063912,-52.1115844029815,-34.817329615412));
#22173=CARTESIAN_POINT('Ctrl Pts',(-16.9321745223381,-50.5446530257126,
-34.7365517774293));
#22174=CARTESIAN_POINT('Ctrl Pts',(-16.931281743668,-49.9994424172085,-34.7084234471775));
#22175=CARTESIAN_POINT('Ctrl Pts',(-16.929755691605,-49.9979131056248,-35.7915765528225));
#22176=CARTESIAN_POINT('Ctrl Pts',(-16.927462104359,-49.6353441575151,-35.7728476598161));
#22177=CARTESIAN_POINT('Ctrl Pts',(-17.1539340252026,-48.2563157484261,
-35.7014692590789));
#22178=CARTESIAN_POINT('Ctrl Pts',(-19.1896897477077,-46.4652110393336,
-35.5774413506109));
#22179=CARTESIAN_POINT('Ctrl Pts',(-22.5168916085772,-47.3891395418682,
-35.4194928274184));
#22180=CARTESIAN_POINT('Ctrl Pts',(-23.5621043957074,-50.6802558160081,
-35.261544304226));
#22181=CARTESIAN_POINT('Ctrl Pts',(-21.3776654637779,-53.3546048308447,
-35.1035957810335));
#22182=CARTESIAN_POINT('Ctrl Pts',(-17.9722381641981,-52.9904404798302,
-34.946939863899));
#22183=CARTESIAN_POINT('Ctrl Pts',(-16.923655880331,-50.9869821444003,-34.8429334544954));
#22184=CARTESIAN_POINT('Ctrl Pts',(-16.9216102653814,-49.9995482667975,
-34.7915765528225));
#22185=CARTESIAN_POINT('Origin',(-20.,-50.,-42.2084234471774));
#22186=CARTESIAN_POINT('',(-16.9287431816361,-50.0024708147691,-36.7915765528225));
#22187=CARTESIAN_POINT('',(-16.9234134019188,-49.9979412457337,-36.7084234471775));
#22188=CARTESIAN_POINT('',(-16.9265,-49.9999999999998,-42.2084234471774));
#22189=CARTESIAN_POINT('Ctrl Pts',(-16.9234134019188,-49.9979412457337,
-36.7084234471775));
#22190=CARTESIAN_POINT('Ctrl Pts',(-16.9224089863605,-49.8680690942478,
-36.7016792035325));
#22191=CARTESIAN_POINT('Ctrl Pts',(-16.9886295015825,-48.7253704503755,
-36.6422854521568));
#22192=CARTESIAN_POINT('Ctrl Pts',(-18.4185250538729,-46.7365238104494,
-36.5302421930502));
#22193=CARTESIAN_POINT('Ctrl Pts',(-21.868138608337,-46.8917210565137,-36.3722936698577));
#22194=CARTESIAN_POINT('Ctrl Pts',(-23.6239677035562,-49.865100287622,-36.2143451466653));
#22195=CARTESIAN_POINT('Ctrl Pts',(-22.0940554999228,-52.9607889846439,
-36.0563966234728));
#22196=CARTESIAN_POINT('Ctrl Pts',(-18.6655268623454,-53.3720203578719,
-35.8984481002803));
#22197=CARTESIAN_POINT('Ctrl Pts',(-17.0362742450073,-51.4288476172636,
-35.7824570415152));
#22198=CARTESIAN_POINT('Ctrl Pts',(-16.9236809835954,-50.2089228835601,
-35.7191154904809));
#22199=CARTESIAN_POINT('Ctrl Pts',(-16.9255489617634,-50.0026575650068,
-35.7084234471774));
#22200=CARTESIAN_POINT('Ctrl Pts',(-16.9287431816361,-50.0024708147691,
-36.7915765528225));
#22201=CARTESIAN_POINT('Ctrl Pts',(-16.9341065503311,-49.3029384889418,
-36.7554113728678));
#22202=CARTESIAN_POINT('Ctrl Pts',(-17.5169503973051,-47.5769368622601,
-36.6665966851822));
#22203=CARTESIAN_POINT('Ctrl Pts',(-20.3740252799296,-46.3928625195443,
-36.5251324897657));
#22204=CARTESIAN_POINT('Ctrl Pts',(-23.2249077622416,-48.3412939899481,
-36.3671839665732));
#22205=CARTESIAN_POINT('Ctrl Pts',(-23.1518644551494,-51.7936237492067,
-36.2092354433807));
#22206=CARTESIAN_POINT('Ctrl Pts',(-20.2211215074614,-53.6197294072659,
-36.0512869201883));
#22207=CARTESIAN_POINT('Ctrl Pts',(-17.4611825776843,-52.3365584976905,
-35.9120672900022));
#22208=CARTESIAN_POINT('Ctrl Pts',(-16.933909695223,-50.654575600075,-35.825497167547));
#22209=CARTESIAN_POINT('Ctrl Pts',(-16.929755691605,-49.9979131056248,-35.7915765528225));
#22210=CARTESIAN_POINT('Origin',(-20.,-50.,-42.2084234471774));
#22211=CARTESIAN_POINT('',(-16.9215720097223,-49.9996663583571,-37.7915765528225));
#22212=CARTESIAN_POINT('',(-16.9312423703737,-49.999338997349,-37.7084234471775));
#22213=CARTESIAN_POINT('',(-16.9265,-49.9999999999998,-42.2084234471774));
#22214=CARTESIAN_POINT('Ctrl Pts',(-16.9312423703737,-49.999338997349,-37.7084234471775));
#22215=CARTESIAN_POINT('Ctrl Pts',(-16.9303318355252,-49.53066349442,-37.6842429165841));
#22216=CARTESIAN_POINT('Ctrl Pts',(-17.2507294124538,-48.0426973366553,
-37.60741287826));
#22217=CARTESIAN_POINT('Ctrl Pts',(-19.5565635911389,-46.4007356661223,
-37.477933332205));
#22218=CARTESIAN_POINT('Ctrl Pts',(-22.7714373367961,-47.6610953390299,
-37.3199848090126));
#22219=CARTESIAN_POINT('Ctrl Pts',(-23.4735331428005,-51.0420687967573,
-37.1620362858201));
#22220=CARTESIAN_POINT('Ctrl Pts',(-21.0262820888715,-53.4782301377694,
-37.0040877626276));
#22221=CARTESIAN_POINT('Ctrl Pts',(-17.792758810687,-52.7914201594648,-36.8528834830801));
#22222=CARTESIAN_POINT('Ctrl Pts',(-16.9302500412638,-50.8819270157086,
-36.7543287112634));
#22223=CARTESIAN_POINT('Ctrl Pts',(-16.9234134019188,-49.9979412457337,
-36.7084234471775));
#22224=CARTESIAN_POINT('Ctrl Pts',(-16.9215720097223,-49.9996663583571,
-37.7915765528225));
#22225=CARTESIAN_POINT('Ctrl Pts',(-16.9215435649973,-49.9813637458573,
-37.7906245936502));
#22226=CARTESIAN_POINT('Ctrl Pts',(-16.9299480198382,-48.9508349433177,
-37.737023126747));
#22227=CARTESIAN_POINT('Ctrl Pts',(-18.0723369901302,-46.9282824012858,
-37.630772152113));
#22228=CARTESIAN_POINT('Ctrl Pts',(-21.5183203411933,-46.7066674164727,
-37.4728236289205));
#22229=CARTESIAN_POINT('Ctrl Pts',(-23.5876891278802,-49.4710173186029,
-37.3148751057281));
#22230=CARTESIAN_POINT('Ctrl Pts',(-22.4042091405233,-52.7149795309031,
-37.1569265825355));
#22231=CARTESIAN_POINT('Ctrl Pts',(-19.0409059247592,-53.4973524747668,
-36.9989780593431));
#22232=CARTESIAN_POINT('Ctrl Pts',(-17.1181669524113,-51.6556887349243,
-36.8771947161054));
#22233=CARTESIAN_POINT('Ctrl Pts',(-16.9262985227775,-50.3213222670024,
-36.8080608805986));
#22234=CARTESIAN_POINT('Ctrl Pts',(-16.9287431816361,-50.0024708147691,
-36.7915765528225));
#22235=CARTESIAN_POINT('Origin',(-20.,-50.,-42.2084234471774));
#22236=CARTESIAN_POINT('',(-16.9296186885438,-49.9978504047438,-38.7915765528225));
#22237=CARTESIAN_POINT('',(-16.9257450511401,-50.0026845218917,-38.7084234471775));
#22238=CARTESIAN_POINT('',(-16.9265,-49.9999999999998,-42.2084234471774));
#22239=CARTESIAN_POINT('Ctrl Pts',(-16.9257450511401,-50.0026845218917,
-38.7084234471775));
#22240=CARTESIAN_POINT('Ctrl Pts',(-16.9330320360583,-49.1997027895944,
-38.6668066296358));
#22241=CARTESIAN_POINT('Ctrl Pts',(-17.6644030329328,-47.369098904382,-38.5725403043632));
#22242=CARTESIAN_POINT('Ctrl Pts',(-20.7420732981751,-46.4502603278007,
-38.4256244713598));
#22243=CARTESIAN_POINT('Ctrl Pts',(-23.3780463626243,-48.6808544307687,
-38.2676759481674));
#22244=CARTESIAN_POINT('Ctrl Pts',(-22.95124778817,-52.107481644896,-38.1097274249748));
#22245=CARTESIAN_POINT('Ctrl Pts',(-19.8486424720205,-53.6233173671768,
-37.9517789017825));
#22246=CARTESIAN_POINT('Ctrl Pts',(-17.3372411809546,-52.1248689915217,
-37.8180109091832));
#22247=CARTESIAN_POINT('Ctrl Pts',(-16.9323143896863,-50.5511346714054,
-37.7368924243149));
#22248=CARTESIAN_POINT('Ctrl Pts',(-16.9312423703737,-49.999338997349,-37.7084234471775));
#22249=CARTESIAN_POINT('Ctrl Pts',(-16.9296186885438,-49.9978504047438,
-38.7915765528226));
#22250=CARTESIAN_POINT('Ctrl Pts',(-16.9272829236679,-49.6419124103458,
-38.7731883067018));
#22251=CARTESIAN_POINT('Ctrl Pts',(-17.1483416537186,-48.2696528264275,
-38.7021505528502));
#22252=CARTESIAN_POINT('Ctrl Pts',(-19.1670203242729,-46.4705005646606,
-38.5784632912678));
#22253=CARTESIAN_POINT('Ctrl Pts',(-22.5000699934528,-47.373025546768,-38.4205147680754));
#22254=CARTESIAN_POINT('Ctrl Pts',(-23.5664015975527,-50.657372972797,-38.2625662448828));
#22255=CARTESIAN_POINT('Ctrl Pts',(-21.3991756129266,-53.3456879568638,
-38.1046177216904));
#22256=CARTESIAN_POINT('Ctrl Pts',(-17.9840722489439,-53.0026556344016,
-37.9476211576703));
#22257=CARTESIAN_POINT('Ctrl Pts',(-16.9231167425166,-50.9936167565737,
-37.843274101381));
#22258=CARTESIAN_POINT('Ctrl Pts',(-16.9215720097223,-49.9996663583571,
-37.7915765528225));
#22259=CARTESIAN_POINT('Origin',(-20.,-50.,-42.2084234471774));
#22260=CARTESIAN_POINT('',(-16.9296932342852,-50.0033456701988,-39.7915765528225));
#22261=CARTESIAN_POINT('',(-16.9232551256392,-49.9980895495447,-39.7084234471775));
#22262=CARTESIAN_POINT('',(-16.9265,-49.9999999999998,-42.2084234471774));
#22263=CARTESIAN_POINT('',(-19.2062007174672,-52.9692229537457,-40.));
#22264=CARTESIAN_POINT('Ctrl Pts',(-19.2062007174672,-52.9692229537457,
-40.));
#22265=CARTESIAN_POINT('Ctrl Pts',(-18.2239621276955,-52.7066289013681,
-39.9473504922692));
#22266=CARTESIAN_POINT('Ctrl Pts',(-17.1241887959713,-51.6693975435551,
-39.8778760098767));
#22267=CARTESIAN_POINT('Ctrl Pts',(-16.9273403835209,-50.3288691193977,
-39.8084015274842));
#22268=CARTESIAN_POINT('Ctrl Pts',(-16.9296932342852,-50.0033456701988,
-39.7915765528225));
#22269=CARTESIAN_POINT('',(-20.7956622540211,-52.9742863856178,-40.));
#22270=CARTESIAN_POINT('Origin',(-20.,-50.,-40.));
#22271=CARTESIAN_POINT('Ctrl Pts',(-20.7956661367394,-52.9742969385866,
-40.));
#22272=CARTESIAN_POINT('Ctrl Pts',(-19.8486502888634,-53.2252253736959,
-39.9490537266974));
#22273=CARTESIAN_POINT('Ctrl Pts',(-17.7883286491776,-52.7701106788771,
-39.8518615424231));
#22274=CARTESIAN_POINT('Ctrl Pts',(-16.9299363715263,-50.888322508111,-39.754669358149));
#22275=CARTESIAN_POINT('Ctrl Pts',(-16.9232551256392,-49.9980895495447,
-39.7084234471775));
#22276=CARTESIAN_POINT('Origin',(0.,0.,-48.));
#22277=CARTESIAN_POINT('',(-7.26252539463726,0.000110654559175658,-46.6717617050839));
#22278=CARTESIAN_POINT('',(-7.26321021083306,-0.000162629342338461,-47.0782382949161));
#22279=CARTESIAN_POINT('',(-7.263,-8.89460970220723E-16,-48.));
#22280=CARTESIAN_POINT('',(5.46288453460432,-4.78623668048091,-48.));
#22281=CARTESIAN_POINT('Ctrl Pts',(-7.26321021083306,-0.000162629342338461,
-47.0782382949161));
#22282=CARTESIAN_POINT('Ctrl Pts',(-7.26225254003205,0.986861826811056,
-47.1106847833874));
#22283=CARTESIAN_POINT('Ctrl Pts',(-7.05946423163692,1.97426720615771,-47.1431312718588));
#22284=CARTESIAN_POINT('Ctrl Pts',(-6.66813922368638,2.88023829893362,-47.1755777603301));
#22285=CARTESIAN_POINT('Ctrl Pts',(-6.19466067823692,3.97640610449594,-47.2148359622192));
#22286=CARTESIAN_POINT('Ctrl Pts',(-5.44517436528813,4.95335841680263,-47.2540941641082));
#22287=CARTESIAN_POINT('Ctrl Pts',(-4.50904795872082,5.694592197166,-47.2933523659972));
#22288=CARTESIAN_POINT('Ctrl Pts',(-3.5729215521535,6.43582597752937,-47.3326105678863));
#22289=CARTESIAN_POINT('Ctrl Pts',(-2.45015505196766,6.94134122594944,-47.3718687697753));
#22290=CARTESIAN_POINT('Ctrl Pts',(-1.27463114363028,7.15088143827442,-47.4111269716644));
#22291=CARTESIAN_POINT('Ctrl Pts',(-0.0991072352929019,7.36042165059941,
-47.4503851735534));
#22292=CARTESIAN_POINT('Ctrl Pts',(1.129174081196,7.27398682682932,-47.4896433754424));
#22293=CARTESIAN_POINT('Ctrl Pts',(2.26375827103325,6.90183984862936,-47.5289015773315));
#22294=CARTESIAN_POINT('Ctrl Pts',(3.3983424608705,6.52969287042939,-47.5681597792205));
#22295=CARTESIAN_POINT('Ctrl Pts',(4.4392295240561,5.87183373779956,-47.6074179811096));
#22296=CARTESIAN_POINT('Ctrl Pts',(5.26228985868794,5.00679499485275,-47.6466761829986));
#22297=CARTESIAN_POINT('Ctrl Pts',(6.08535019331978,4.14175625190593,-47.6859343848877));
#22298=CARTESIAN_POINT('Ctrl Pts',(6.69058379939787,3.06953789864212,-47.7251925867767));
#22299=CARTESIAN_POINT('Ctrl Pts',(7.00585036078105,1.91780922016447,-47.7644507886658));
#22300=CARTESIAN_POINT('Ctrl Pts',(7.32111692216422,0.766080541686827,-47.8037089905548));
#22301=CARTESIAN_POINT('Ctrl Pts',(7.3464164388525,-0.465158462004661,-47.8429671924438));
#22302=CARTESIAN_POINT('Ctrl Pts',(7.07862576269182,-1.62865261403763,-47.8822253943329));
#22303=CARTESIAN_POINT('Ctrl Pts',(6.81083508653114,-2.7921467660706,-47.9214835962219));
#22304=CARTESIAN_POINT('Ctrl Pts',(6.2499542175215,-3.88789606644505,-47.960741798111));
#22305=CARTESIAN_POINT('Ctrl Pts',(5.46288453460432,-4.78623668048091,-48.));
#22306=CARTESIAN_POINT('',(-5.46328272950459,-4.78643225728875,-48.));
#22307=CARTESIAN_POINT('Origin',(0.,0.,-48.));
#22308=CARTESIAN_POINT('Ctrl Pts',(-5.46328272950459,-4.78643225728875,
-48.));
#22309=CARTESIAN_POINT('Ctrl Pts',(-4.76265400353559,-5.58484241293595,
-47.9650783907933));
#22310=CARTESIAN_POINT('Ctrl Pts',(-3.88494971070624,-6.2285788144042,-47.9301567815866));
#22311=CARTESIAN_POINT('Ctrl Pts',(-2.91187904120844,-6.65437822564185,
-47.8952351723799));
#22312=CARTESIAN_POINT('Ctrl Pts',(-1.81797169663776,-7.1330537400391,-47.8559769704909));
#22313=CARTESIAN_POINT('Ctrl Pts',(-0.603542001115805,-7.33630431601018,
-47.8167187686018));
#22314=CARTESIAN_POINT('Ctrl Pts',(0.586609853467524,-7.23987447027158,
-47.7774605667127));
#22315=CARTESIAN_POINT('Ctrl Pts',(1.77676170805086,-7.14344462453298,-47.7382023648237));
#22316=CARTESIAN_POINT('Ctrl Pts',(2.94263572169557,-6.74733435708469,-47.6989441629347));
#22317=CARTESIAN_POINT('Ctrl Pts',(3.94520772278473,-6.09878584913582,-47.6596859610456));
#22318=CARTESIAN_POINT('Ctrl Pts',(4.94777972387388,-5.45023734118695,-47.6204277591566));
#22319=CARTESIAN_POINT('Ctrl Pts',(5.78704971240747,-4.54925059273749,-47.5811695572675));
#22320=CARTESIAN_POINT('Ctrl Pts',(6.36294479614214,-3.50325510007056,-47.5419113553785));
#22321=CARTESIAN_POINT('Ctrl Pts',(6.9388398798768,-2.45725960740365,-47.5026531534894));
#22322=CARTESIAN_POINT('Ctrl Pts',(7.25136005881256,-1.26625537051926,-47.4633949516004));
#22323=CARTESIAN_POINT('Ctrl Pts',(7.26323910849272,-0.0722609117331363,
-47.4241367497114));
#22324=CARTESIAN_POINT('Ctrl Pts',(7.27511815817288,1.12173354705299,-47.3848785478223));
#22325=CARTESIAN_POINT('Ctrl Pts',(6.98635607859744,2.31871822774086,-47.3456203459333));
#22326=CARTESIAN_POINT('Ctrl Pts',(6.43138560219337,3.37596501114632,-47.3063621440442));
#22327=CARTESIAN_POINT('Ctrl Pts',(5.87641512578929,4.43321179455178,-47.2671039421552));
#22328=CARTESIAN_POINT('Ctrl Pts',(5.05523625255658,5.35072068067483,-47.2278457402662));
#22329=CARTESIAN_POINT('Ctrl Pts',(4.06576665043739,6.01908670620214,-47.1885875383771));
#22330=CARTESIAN_POINT('Ctrl Pts',(3.07629704831819,6.68745273172946,-47.1493293364881));
#22331=CARTESIAN_POINT('Ctrl Pts',(1.91853671731251,7.10667589666103,-47.1100711345991));
#22332=CARTESIAN_POINT('Ctrl Pts',(0.730537929376382,7.22676802273927,-47.07081293271));
#22333=CARTESIAN_POINT('Ctrl Pts',(-0.45746085855973,7.3468601488175,-47.031554730821));
#22334=CARTESIAN_POINT('Ctrl Pts',(-1.67569810342629,7.16782123604241,-46.9922965289319));
#22335=CARTESIAN_POINT('Ctrl Pts',(-2.77891042070149,6.71099986948637,-46.9530383270428));
#22336=CARTESIAN_POINT('Ctrl Pts',(-3.8821227379767,6.25417850293032,-46.9137801251538));
#22337=CARTESIAN_POINT('Ctrl Pts',(-4.87031012766054,5.51957468259332,-46.8745219232648));
#22338=CARTESIAN_POINT('Ctrl Pts',(-5.62564041196335,4.59478314278975,-46.8352637213757));
#22339=CARTESIAN_POINT('Ctrl Pts',(-6.38097069626616,3.66999160298619,-46.7960055194867));
#22340=CARTESIAN_POINT('Ctrl Pts',(-6.90344387518794,2.55501234371607,-46.7567473175976));
#22341=CARTESIAN_POINT('Ctrl Pts',(-7.13075990222278,1.38279622732194,-46.7174891157086));
#22342=CARTESIAN_POINT('Ctrl Pts',(-7.21901809040275,0.927669187060691,
-46.7022466455004));
#22343=CARTESIAN_POINT('Ctrl Pts',(-7.26278209805939,0.463913837991132,
-46.6870041752921));
#22344=CARTESIAN_POINT('Ctrl Pts',(-7.26252539463726,0.000110654559175658,
-46.6717617050839));
#22345=CARTESIAN_POINT('Origin',(0.,0.,-48.));
#22346=CARTESIAN_POINT('',(-7.26337486577337,0.000131920041138065,-45.1717617050839));
#22347=CARTESIAN_POINT('',(-7.26244595120635,-6.5281985395238E-5,-45.5782382949161));
#22348=CARTESIAN_POINT('',(-7.263,-8.89460970220723E-16,-48.));
#22349=CARTESIAN_POINT('Ctrl Pts',(-7.26244595120635,-6.5281985395238E-5,
-45.5782382949161));
#22350=CARTESIAN_POINT('Ctrl Pts',(-7.26222960724132,0.672113855431829,
-45.6003281588299));
#22351=CARTESIAN_POINT('Ctrl Pts',(-7.1696578432929,1.34435139215194,-45.6224180227437));
#22352=CARTESIAN_POINT('Ctrl Pts',(-6.98553937325194,1.99050304088456,-45.6445078866575));
#22353=CARTESIAN_POINT('Ctrl Pts',(-6.65832323029251,3.13884655154996,-45.6837660885465));
#22354=CARTESIAN_POINT('Ctrl Pts',(-6.04196091327337,4.20479895246961,-45.7230242904355));
#22355=CARTESIAN_POINT('Ctrl Pts',(-5.20994789013978,5.06125534521791,-45.7622824923246));
#22356=CARTESIAN_POINT('Ctrl Pts',(-4.37793486700618,5.91771173796621,-45.8015406942136));
#22357=CARTESIAN_POINT('Ctrl Pts',(-3.33027113775813,6.56467212254317,-45.8407988961027));
#22358=CARTESIAN_POINT('Ctrl Pts',(-2.19188084772556,6.92499249435054,-45.8800570979917));
#22359=CARTESIAN_POINT('Ctrl Pts',(-1.05349055769298,7.28531286615791,-45.9193152998808));
#22360=CARTESIAN_POINT('Ctrl Pts',(0.175626293124121,7.35899322519568,-45.9585735017698));
#22361=CARTESIAN_POINT('Ctrl Pts',(1.34890896305861,7.13724787896668,-45.9978317036589));
#22362=CARTESIAN_POINT('Ctrl Pts',(2.52219163299309,6.91550253273769,-46.0370899055479));
#22363=CARTESIAN_POINT('Ctrl Pts',(3.63964012204496,6.39833148124193,-46.076348107437));
#22364=CARTESIAN_POINT('Ctrl Pts',(4.56800910299865,5.64740254855039,-46.115606309326));
#22365=CARTESIAN_POINT('Ctrl Pts',(5.49637808395232,4.89647361585885,-46.154864511215));
#22366=CARTESIAN_POINT('Ctrl Pts',(6.23566755680782,3.91178680197153,-46.194122713104));
#22367=CARTESIAN_POINT('Ctrl Pts',(6.69772413224052,2.8107568596051,-46.2333809149931));
#22368=CARTESIAN_POINT('Ctrl Pts',(7.15978070767323,1.70972691723866,-46.2726391168821));
#22369=CARTESIAN_POINT('Ctrl Pts',(7.34460438568313,0.492353846393101,-46.3118973187712));
#22370=CARTESIAN_POINT('Ctrl Pts',(7.23015666890219,-0.696201984692038,
-46.3511555206602));
#22371=CARTESIAN_POINT('Ctrl Pts',(7.11570895212125,-1.88475781577716,-46.3904137225493));
#22372=CARTESIAN_POINT('Ctrl Pts',(6.70198984054947,-3.04449640710186,-46.4296719244383));
#22373=CARTESIAN_POINT('Ctrl Pts',(6.03833147527558,-4.03712965529138,-46.4689301263274));
#22374=CARTESIAN_POINT('Ctrl Pts',(5.37467311000168,-5.02976290348091,-46.5081883282164));
#22375=CARTESIAN_POINT('Ctrl Pts',(4.46107549102567,-5.85529080853525,-46.5474465301055));
#22376=CARTESIAN_POINT('Ctrl Pts',(3.40647665113655,-6.41527700380401,-46.5867047319945));
#22377=CARTESIAN_POINT('Ctrl Pts',(2.35187781124742,-6.97526319907276,-46.6259629338835));
#22378=CARTESIAN_POINT('Ctrl Pts',(1.15627775044517,-7.26970768455593,-46.6652211357726));
#22379=CARTESIAN_POINT('Ctrl Pts',(-0.0377594013239463,-7.26350039167212,
-46.7044793376616));
#22380=CARTESIAN_POINT('Ctrl Pts',(-1.23179655309304,-7.25729309878831,
-46.7437375395507));
#22381=CARTESIAN_POINT('Ctrl Pts',(-2.42427079582901,-6.95043402753753,
-46.7829957414397));
#22382=CARTESIAN_POINT('Ctrl Pts',(-3.47299058508026,-6.37951388512164,
-46.8222539433288));
#22383=CARTESIAN_POINT('Ctrl Pts',(-4.52171037433153,-5.80859374270573,
-46.8615121452178));
#22384=CARTESIAN_POINT('Ctrl Pts',(-5.42667571009807,-4.9736125291247,-46.9007703471068));
#22385=CARTESIAN_POINT('Ctrl Pts',(-6.0799780911766,-3.97413272045434,-46.9400285489959));
#22386=CARTESIAN_POINT('Ctrl Pts',(-6.73328047225512,-2.97465291178399,
-46.9792867508849));
#22387=CARTESIAN_POINT('Ctrl Pts',(-7.13491989864563,-1.8106745080243,-47.018544952774));
#22388=CARTESIAN_POINT('Ctrl Pts',(-7.23700422286582,-0.620993656735478,
-47.057803154663));
#22389=CARTESIAN_POINT('Ctrl Pts',(-7.25471693326944,-0.414571441056566,
-47.0646148680807));
#22390=CARTESIAN_POINT('Ctrl Pts',(-7.26341126121947,-0.207375429504603,
-47.0714265814984));
#22391=CARTESIAN_POINT('Ctrl Pts',(-7.26321021083306,-0.000162629342338461,
-47.0782382949161));
#22392=CARTESIAN_POINT('Ctrl Pts',(-7.26252539463726,0.000110654559175658,
-46.6717617050839));
#22393=CARTESIAN_POINT('Ctrl Pts',(-7.26212093785149,-0.730648379498221,
-46.6477459734031));
#22394=CARTESIAN_POINT('Ctrl Pts',(-7.15243715971961,-1.46152616008496,
-46.6237302417223));
#22395=CARTESIAN_POINT('Ctrl Pts',(-6.93532594245516,-2.15896185620489,
-46.5997145100415));
#22396=CARTESIAN_POINT('Ctrl Pts',(-6.58041708050481,-3.29905084981948,
-46.5604563081524));
#22397=CARTESIAN_POINT('Ctrl Pts',(-5.93844048145624,-4.34977586353051,
-46.5211981062634));
#22398=CARTESIAN_POINT('Ctrl Pts',(-5.08594588155711,-5.18584773014426,
-46.4819399043743));
#22399=CARTESIAN_POINT('Ctrl Pts',(-4.23345128165796,-6.021919596758,-46.4426817024853));
#22400=CARTESIAN_POINT('Ctrl Pts',(-3.17043868090825,-6.64333831627446,
-46.4034235005962));
#22401=CARTESIAN_POINT('Ctrl Pts',(-2.02366243310959,-6.97600548798374,
-46.3641652987072));
#22402=CARTESIAN_POINT('Ctrl Pts',(-0.876886185310941,-7.30867265969301,
-46.3249070968182));
#22403=CARTESIAN_POINT('Ctrl Pts',(0.353653709536664,-7.35258828359512,
-46.2856488949291));
#22404=CARTESIAN_POINT('Ctrl Pts',(1.52122682474423,-7.10251583237715,-46.2463906930401));
#22405=CARTESIAN_POINT('Ctrl Pts',(2.68879993995179,-6.85244338115917,-46.2071324911511));
#22406=CARTESIAN_POINT('Ctrl Pts',(3.79340627551931,-6.30838285482113,-46.167874289262));
#22407=CARTESIAN_POINT('Ctrl Pts',(4.70333181059907,-5.53520840479315,-46.128616087373));
#22408=CARTESIAN_POINT('Ctrl Pts',(5.61325734567882,-4.76203395476518,-46.0893578854839));
#22409=CARTESIAN_POINT('Ctrl Pts',(6.3285020802708,-3.75974558104729,-46.0500996835949));
#22410=CARTESIAN_POINT('Ctrl Pts',(6.76377973869342,-2.64785684107879,-46.0108414817058));
#22411=CARTESIAN_POINT('Ctrl Pts',(7.19905739711604,-1.53596810111027,-45.9715832798168));
#22412=CARTESIAN_POINT('Ctrl Pts',(7.35436797936928,-0.314478994891145,
-45.9323250779277));
#22413=CARTESIAN_POINT('Ctrl Pts',(7.21119214461735,0.870959274325189,-45.8930668760387));
#22414=CARTESIAN_POINT('Ctrl Pts',(7.06801630986543,2.05639754354152,-45.8538086741497));
#22415=CARTESIAN_POINT('Ctrl Pts',(6.62635405810834,3.20578497575507,-45.8145504722606));
#22416=CARTESIAN_POINT('Ctrl Pts',(5.93886950080655,4.18206782069874,-45.7752922703716));
#22417=CARTESIAN_POINT('Ctrl Pts',(5.25138494350475,5.15835066564242,-45.7360340684826));
#22418=CARTESIAN_POINT('Ctrl Pts',(4.31807808065826,5.96152892331622,-45.6967758665935));
#22419=CARTESIAN_POINT('Ctrl Pts',(3.25023706632267,6.49583106437886,-45.6575176647045));
#22420=CARTESIAN_POINT('Ctrl Pts',(2.1823960519871,7.03013320544148,-45.6182594628154));
#22421=CARTESIAN_POINT('Ctrl Pts',(0.980020886162445,7.29555922989294,-45.5790012609263));
#22422=CARTESIAN_POINT('Ctrl Pts',(-0.213516387111539,7.26045955548486,
-45.5397430590373));
#22423=CARTESIAN_POINT('Ctrl Pts',(-1.40705366038551,7.22535988107679,-45.5004848571483));
#22424=CARTESIAN_POINT('Ctrl Pts',(-2.59175304110882,6.88973450780919,-45.4612266552593));
#22425=CARTESIAN_POINT('Ctrl Pts',(-3.62635015802862,6.29360363668561,-45.4219684533702));
#22426=CARTESIAN_POINT('Ctrl Pts',(-4.66094727494843,5.69747276556203,-45.3827102514812));
#22427=CARTESIAN_POINT('Ctrl Pts',(-5.54544212806474,4.84083639658247,-45.3434520495921));
#22428=CARTESIAN_POINT('Ctrl Pts',(-6.1743669410577,3.82584044120064,-45.3041938477031));
#22429=CARTESIAN_POINT('Ctrl Pts',(-6.80329175405065,2.81084448581881,-45.264935645814));
#22430=CARTESIAN_POINT('Ctrl Pts',(-7.17664652692027,1.63748894403472,-45.225677443925));
#22431=CARTESIAN_POINT('Ctrl Pts',(-7.24991217904467,0.44568553991911,-45.1864192420359));
#22432=CARTESIAN_POINT('Ctrl Pts',(-7.25903039257842,0.29736067534915,-45.1815333963853));
#22433=CARTESIAN_POINT('Ctrl Pts',(-7.26350057604359,0.148750074933102,
-45.1766475507346));
#22434=CARTESIAN_POINT('Ctrl Pts',(-7.26337486577337,0.000131920041138065,
-45.1717617050839));
#22435=CARTESIAN_POINT('Origin',(0.,0.,-48.));
#22436=CARTESIAN_POINT('',(-7.26332735433935,-0.000142917180729311,-43.6717617050839));
#22437=CARTESIAN_POINT('',(-7.26276508042368,0.000167022802991385,-44.0782382949161));
#22438=CARTESIAN_POINT('',(-7.263,-8.89460970220723E-16,-48.));
#22439=CARTESIAN_POINT('Ctrl Pts',(-7.26276508042368,0.000167022802991385,
-44.0782382949161));
#22440=CARTESIAN_POINT('Ctrl Pts',(-7.26307825553427,0.357156309383415,
-44.0899715342723));
#22441=CARTESIAN_POINT('Ctrl Pts',(-7.23721492674339,0.714100615384112,
-44.1017047736286));
#22442=CARTESIAN_POINT('Ctrl Pts',(-7.18478680450647,1.0670994630721,-44.1134380129848));
#22443=CARTESIAN_POINT('Ctrl Pts',(-7.00936774545981,2.24819699363302,-44.1526962148739));
#22444=CARTESIAN_POINT('Ctrl Pts',(-6.53655524196093,3.3851250319695,-44.1919544167629));
#22445=CARTESIAN_POINT('Ctrl Pts',(-5.82272778302649,4.34231549464923,-44.2312126186519));
#22446=CARTESIAN_POINT('Ctrl Pts',(-5.10890032409204,5.29950595732896,-44.270470820541));
#22447=CARTESIAN_POINT('Ctrl Pts',(-4.15405790972205,6.07695884435194,-44.30972902243));
#22448=CARTESIAN_POINT('Ctrl Pts',(-3.07205660796225,6.58197013725935,-44.3489872243191));
#22449=CARTESIAN_POINT('Ctrl Pts',(-1.99005530620244,7.08698143016676,-44.3882454262081));
#22450=CARTESIAN_POINT('Ctrl Pts',(-0.780895117052828,7.3195511289586,-44.4275036280971));
#22451=CARTESIAN_POINT('Ctrl Pts',(0.411242864572872,7.25194746234682,-44.4667618299862));
#22452=CARTESIAN_POINT('Ctrl Pts',(1.60338084619856,7.18434379573504,-44.5060200318752));
#22453=CARTESIAN_POINT('Ctrl Pts',(2.77849662030031,6.81656676371965,-44.5452782337643));
#22454=CARTESIAN_POINT('Ctrl Pts',(3.79646857149504,6.19247035325541,-44.5845364356533));
#22455=CARTESIAN_POINT('Ctrl Pts',(4.81444052268977,5.56837394279117,-44.6237946375423));
#22456=CARTESIAN_POINT('Ctrl Pts',(5.67526865097746,4.68795815387806,-44.6630528394314));
#22457=CARTESIAN_POINT('Ctrl Pts',(6.2763072166269,3.65620437240841,-44.7023110413205));
#22458=CARTESIAN_POINT('Ctrl Pts',(6.87734578227633,2.62445059093877,-44.7415692432095));
#22459=CARTESIAN_POINT('Ctrl Pts',(7.21859478528751,1.44135881691259,-44.7808274450985));
#22460=CARTESIAN_POINT('Ctrl Pts',(7.25936345918091,0.248001729448511,-44.8200856469876));
#22461=CARTESIAN_POINT('Ctrl Pts',(7.30013213307431,-0.945355358015584,
-44.8593438488766));
#22462=CARTESIAN_POINT('Ctrl Pts',(7.04042047784991,-2.14897775891758,-44.8986020507657));
#22463=CARTESIAN_POINT('Ctrl Pts',(6.51119669040129,-3.21934470804107,-44.9378602526547));
#22464=CARTESIAN_POINT('Ctrl Pts',(5.98197290295268,-4.28971165716457,-44.9771184545437));
#22465=CARTESIAN_POINT('Ctrl Pts',(5.18323698327985,-5.22682315450957,-45.0163766564328));
#22466=CARTESIAN_POINT('Ctrl Pts',(4.2102307533317,-5.91893737879056,-45.0556348583218));
#22467=CARTESIAN_POINT('Ctrl Pts',(3.23722452338356,-6.61105160307155,-45.0948930602109));
#22468=CARTESIAN_POINT('Ctrl Pts',(2.08994798316011,-7.05816855428853,-45.1341512620999));
#22469=CARTESIAN_POINT('Ctrl Pts',(0.905203178600487,-7.20697369883143,
-45.173409463989));
#22470=CARTESIAN_POINT('Ctrl Pts',(-0.279541625959134,-7.35577884337434,
-45.212667665878));
#22471=CARTESIAN_POINT('Ctrl Pts',(-1.50175469485492,-7.20627218124317,
-45.251925867767));
#22472=CARTESIAN_POINT('Ctrl Pts',(-2.61569849879883,-6.77628098988389,
-45.2911840696561));
#22473=CARTESIAN_POINT('Ctrl Pts',(-3.72964230274274,-6.34628979852462,
-45.3304422715451));
#22474=CARTESIAN_POINT('Ctrl Pts',(-4.73531684173477,-5.63581407793723,
-45.3697004734342));
#22475=CARTESIAN_POINT('Ctrl Pts',(-5.51280479011146,-4.72957144318576,
-45.4089586753232));
#22476=CARTESIAN_POINT('Ctrl Pts',(-6.29029273848814,-3.82332880843428,
-45.4482168772123));
#22477=CARTESIAN_POINT('Ctrl Pts',(-6.83959409624948,-2.72131925951872,
-45.4874750791013));
#22478=CARTESIAN_POINT('Ctrl Pts',(-7.09520979068029,-1.55494717485536,
-45.5267332809903));
#22479=CARTESIAN_POINT('Ctrl Pts',(-7.20699526282622,-1.04487108397895,
-45.5439016189656));
#22480=CARTESIAN_POINT('Ctrl Pts',(-7.26261409467365,-0.522485820931676,
-45.5610699569408));
#22481=CARTESIAN_POINT('Ctrl Pts',(-7.26244595120635,-6.5281985395238E-5,
-45.5782382949161));
#22482=CARTESIAN_POINT('Ctrl Pts',(-7.26337486577337,0.000131920041138065,
-45.1717617050839));
#22483=CARTESIAN_POINT('Ctrl Pts',(-7.26249048290506,-1.04540994285732,
-45.1373893488456));
#22484=CARTESIAN_POINT('Ctrl Pts',(-7.03414397040485,-2.09132569542317,
-45.1030169926072));
#22485=CARTESIAN_POINT('Ctrl Pts',(-6.5964883600218,-3.04075706370068,-45.0686446363688));
#22486=CARTESIAN_POINT('Ctrl Pts',(-6.09662235749536,-4.12514499675771,
-45.0293864344798));
#22487=CARTESIAN_POINT('Ctrl Pts',(-5.3237138210633,-5.08366959642465,-44.9901282325907));
#22488=CARTESIAN_POINT('Ctrl Pts',(-4.36992489768557,-5.80203572834054,
-44.9508700307017));
#22489=CARTESIAN_POINT('Ctrl Pts',(-3.41613597430784,-6.52040186025644,
-44.9116118288126));
#22490=CARTESIAN_POINT('Ctrl Pts',(-2.28146666398445,-6.9986095244213,-44.8723536269236));
#22491=CARTESIAN_POINT('Ctrl Pts',(-1.10121571786165,-7.17963690913996,
-44.8330954250346));
#22492=CARTESIAN_POINT('Ctrl Pts',(0.0790352282611506,-7.36066429385862,
-44.7938372231455));
#22493=CARTESIAN_POINT('Ctrl Pts',(1.30486781018336,-7.24451139913107,-44.7545790212565));
#22494=CARTESIAN_POINT('Ctrl Pts',(2.43011290537809,-6.84502837623527,-44.7153208193674));
#22495=CARTESIAN_POINT('Ctrl Pts',(3.55535800057282,-6.44554535333947,-44.6760626174784));
#22496=CARTESIAN_POINT('Ctrl Pts',(4.58001560904007,-5.76273220227542,-44.6368044155893));
#22497=CARTESIAN_POINT('Ctrl Pts',(5.38190485083829,-4.87800803411333,-44.5975462137003));
#22498=CARTESIAN_POINT('Ctrl Pts',(6.18379409263651,-3.99328386595124,-44.5582880118113));
#22499=CARTESIAN_POINT('Ctrl Pts',(6.7629149677657,-2.90664868069111,-44.5190298099222));
#22500=CARTESIAN_POINT('Ctrl Pts',(7.05021270365494,-1.74767360727724,-44.4797716080332));
#22501=CARTESIAN_POINT('Ctrl Pts',(7.33751043954418,-0.58869853386337,-44.4405134061441));
#22502=CARTESIAN_POINT('Ctrl Pts',(7.33298503619347,0.642616427704244,-44.4012552042551));
#22503=CARTESIAN_POINT('Ctrl Pts',(7.03717610581953,1.79944843216851,-44.361997002366));
#22504=CARTESIAN_POINT('Ctrl Pts',(6.74136717544558,2.95628043663279,-44.322738800477));
#22505=CARTESIAN_POINT('Ctrl Pts',(6.15427471804838,4.03862948399371,-44.283480598588));
#22506=CARTESIAN_POINT('Ctrl Pts',(5.34590404316654,4.91743552734621,-44.2442223966989));
#22507=CARTESIAN_POINT('Ctrl Pts',(4.53753336828468,5.79624157069871,-44.2049641948099));
#22508=CARTESIAN_POINT('Ctrl Pts',(3.50788447591818,6.47150461004279,-44.1657059929209));
#22509=CARTESIAN_POINT('Ctrl Pts',(2.37973341014317,6.86270581483713,-44.1264477910318));
#22510=CARTESIAN_POINT('Ctrl Pts',(1.25158234436817,7.25390701963147,-44.0871895891428));
#22511=CARTESIAN_POINT('Ctrl Pts',(0.0249291051846681,7.36104638987607,
-44.0479313872537));
#22512=CARTESIAN_POINT('Ctrl Pts',(-1.15395932914251,7.17134855316878,-44.0086731853647));
#22513=CARTESIAN_POINT('Ctrl Pts',(-2.33284776346969,6.98165071646149,-43.9694149834756));
#22514=CARTESIAN_POINT('Ctrl Pts',(-3.46397139294055,6.49511567280232,-43.9301567815866));
#22515=CARTESIAN_POINT('Ctrl Pts',(-4.41245425583934,5.76975819636112,-43.8908985796975));
#22516=CARTESIAN_POINT('Ctrl Pts',(-5.36093711873811,5.04440071991993,-43.8516403778085));
#22517=CARTESIAN_POINT('Ctrl Pts',(-6.12677921506481,4.08022081069672,-43.8123821759195));
#22518=CARTESIAN_POINT('Ctrl Pts',(-6.618661005051,2.9921879460636,-43.7731239740304));
#22519=CARTESIAN_POINT('Ctrl Pts',(-7.04199720731669,2.05577657603305,-43.7393365510482));
#22520=CARTESIAN_POINT('Ctrl Pts',(-7.26240774709746,1.02762584652013,-43.7055491280661));
#22521=CARTESIAN_POINT('Ctrl Pts',(-7.26332735433935,-0.000142917180729311,
-43.6717617050839));
#22522=CARTESIAN_POINT('Origin',(0.,0.,-48.));
#22523=CARTESIAN_POINT('',(-7.26249686403911,-9.76851341781633E-5,-42.1717617050839));
#22524=CARTESIAN_POINT('',(-7.26357703776439,4.20713134600785E-5,-42.5782382949161));
#22525=CARTESIAN_POINT('',(-7.263,-8.89460970220723E-16,-48.));
#22526=CARTESIAN_POINT('Ctrl Pts',(-7.26357703776439,4.20713134600785E-5,
-42.5782382949161));
#22527=CARTESIAN_POINT('Ctrl Pts',(-7.26359058067385,0.0419126988576804,
-42.5796149097148));
#22528=CARTESIAN_POINT('Ctrl Pts',(-7.26323593189466,0.0837830962705636,
-42.5809915245135));
#22529=CARTESIAN_POINT('Ctrl Pts',(-7.26251165209856,0.125647098779436,
-42.5823681393121));
#22530=CARTESIAN_POINT('Ctrl Pts',(-7.2418566929288,1.31952171348383,-42.6216263412012));
#22531=CARTESIAN_POINT('Ctrl Pts',(-6.92059109431216,2.50819553037637,-42.6608845430902));
#22532=CARTESIAN_POINT('Ctrl Pts',(-6.33702278780508,3.5499302637007,-42.7001427449793));
#22533=CARTESIAN_POINT('Ctrl Pts',(-5.75345448129799,4.59166499702504,-42.7394009468683));
#22534=CARTESIAN_POINT('Ctrl Pts',(-4.90758346690044,5.48646064678117,-42.7786591487574));
#22535=CARTESIAN_POINT('Ctrl Pts',(-3.90027198776768,6.12762116255026,-42.8179173506464));
#22536=CARTESIAN_POINT('Ctrl Pts',(-2.89296050863493,6.76878167831935,-42.8571755525354));
#22537=CARTESIAN_POINT('Ctrl Pts',(-1.72420856476698,7.1563070601014,-42.8964337544245));
#22538=CARTESIAN_POINT('Ctrl Pts',(-0.533378944040606,7.24398851409589,
-42.9356919563135));
#22539=CARTESIAN_POINT('Ctrl Pts',(0.657450676685749,7.33166996809038,-42.9749501582026));
#22540=CARTESIAN_POINT('Ctrl Pts',(1.87035797427052,7.11950749429731,-43.0142083600916));
#22541=CARTESIAN_POINT('Ctrl Pts',(2.96071504600573,6.63279949242055,-43.0534665619806));
#22542=CARTESIAN_POINT('Ctrl Pts',(4.05107211774098,6.14609149054378,-43.0927247638697));
#22543=CARTESIAN_POINT('Ctrl Pts',(5.01887896362666,5.38483796058329,-43.1319829657587));
#22544=CARTESIAN_POINT('Ctrl Pts',(5.74873362786153,4.43981129848928,-43.1712411676478));
#22545=CARTESIAN_POINT('Ctrl Pts',(6.47858829209638,3.49478463639531,-43.2104993695368));
#22546=CARTESIAN_POINT('Ctrl Pts',(6.97049077468044,2.3659848421678,-43.2497575714259));
#22547=CARTESIAN_POINT('Ctrl Pts',(7.16578628432451,1.18801078180539,-43.2890157733149));
#22548=CARTESIAN_POINT('Ctrl Pts',(7.36108179396858,0.0100367214429617,
-43.328273975204));
#22549=CARTESIAN_POINT('Ctrl Pts',(7.25977033067266,-1.21711160505437,-43.367532177093));
#22550=CARTESIAN_POINT('Ctrl Pts',(6.87393234319481,-2.34710818486907,-43.406790378982));
#22551=CARTESIAN_POINT('Ctrl Pts',(6.48809435571697,-3.47710476468377,-43.4460485808711));
#22552=CARTESIAN_POINT('Ctrl Pts',(5.8177298440572,-4.50994959781582,-43.4853067827601));
#22553=CARTESIAN_POINT('Ctrl Pts',(4.94277353493723,-5.32248555400794,-43.5245649846492));
#22554=CARTESIAN_POINT('Ctrl Pts',(4.06781722581725,-6.13502151020005,-43.5638231865382));
#22555=CARTESIAN_POINT('Ctrl Pts',(2.98826911923707,-6.72724858945223,-43.6030813884273));
#22556=CARTESIAN_POINT('Ctrl Pts',(1.83285527599125,-7.02854922637454,-43.6423395903163));
#22557=CARTESIAN_POINT('Ctrl Pts',(0.67744143274542,-7.32984986329684,-43.6815977922053));
#22558=CARTESIAN_POINT('Ctrl Pts',(-0.553838147166054,-7.34022405788928,
-43.7208559940944));
#22559=CARTESIAN_POINT('Ctrl Pts',(-1.71416483741916,-7.05843478403355,
-43.7601141959834));
#22560=CARTESIAN_POINT('Ctrl Pts',(-2.87449152767229,-6.77664551017782,
-43.7993723978725));
#22561=CARTESIAN_POINT('Ctrl Pts',(-3.96386532826705,-6.20269276787391,
-43.8386305997615));
#22562=CARTESIAN_POINT('Ctrl Pts',(-4.8523885558778,-5.40501507797021,-43.8778888016506));
#22563=CARTESIAN_POINT('Ctrl Pts',(-5.74091178348852,-4.60733738806652,
-43.9171470035396));
#22564=CARTESIAN_POINT('Ctrl Pts',(-6.42858443811523,-3.58593475056303,
-43.9564052054286));
#22565=CARTESIAN_POINT('Ctrl Pts',(-6.83340795813138,-2.46259992041862,
-43.9956634073177));
#22566=CARTESIAN_POINT('Ctrl Pts',(-7.11724042331498,-1.67500019287866,
-44.0231883698505));
#22567=CARTESIAN_POINT('Ctrl Pts',(-7.26203040409744,-0.837292815814653,
-44.0507133323833));
#22568=CARTESIAN_POINT('Ctrl Pts',(-7.26276508042368,0.000167022802991385,
-44.0782382949161));
#22569=CARTESIAN_POINT('Ctrl Pts',(-7.26332735433935,-0.000142917180729311,
-43.6717617050839));
#22570=CARTESIAN_POINT('Ctrl Pts',(-7.26347625494962,-0.166556782972505,
-43.666290926177));
#22571=CARTESIAN_POINT('Ctrl Pts',(-7.25787069293385,-0.332960634646776,
-43.6608201472702));
#22572=CARTESIAN_POINT('Ctrl Pts',(-7.24644034797737,-0.49896341304413,
-43.6553493683633));
#22573=CARTESIAN_POINT('Ctrl Pts',(-7.16441641727186,-1.69019608747572,
-43.6160911664742));
#22574=CARTESIAN_POINT('Ctrl Pts',(-6.78244707221516,-2.86077561629585,
-43.5768329645852));
#22575=CARTESIAN_POINT('Ctrl Pts',(-6.14607860095665,-3.87112128913753,
-43.5375747626962));
#22576=CARTESIAN_POINT('Ctrl Pts',(-5.50971012969813,-4.88146696197922,
-43.4983165608071));
#22577=CARTESIAN_POINT('Ctrl Pts',(-4.61894253223782,-5.73157877884247,
-43.4590583589181));
#22578=CARTESIAN_POINT('Ctrl Pts',(-3.5799915512606,-6.32008882036113,-43.419800157029));
#22579=CARTESIAN_POINT('Ctrl Pts',(-2.5410405702834,-6.90859886187978,-43.38054195514));
#22580=CARTESIAN_POINT('Ctrl Pts',(-1.3539062057893,-7.23550712805385,-43.3412837532509));
#22581=CARTESIAN_POINT('Ctrl Pts',(-0.160143178168928,-7.26183285175561,
-43.3020255513619));
#22582=CARTESIAN_POINT('Ctrl Pts',(1.03361984945147,-7.28815857545737,-43.2627673494729));
#22583=CARTESIAN_POINT('Ctrl Pts',(2.23401154019812,-7.01390175668682,-43.2235091475838));
#22584=CARTESIAN_POINT('Ctrl Pts',(3.29789636095449,-6.47176496766949,-43.1842509456948));
#22585=CARTESIAN_POINT('Ctrl Pts',(4.36178118171085,-5.92962817865217,-43.1449927438057));
#22586=CARTESIAN_POINT('Ctrl Pts',(5.28915913247692,-5.11961141938807,-43.1057345419167));
#22587=CARTESIAN_POINT('Ctrl Pts',(5.96944902678939,-4.13830164692163,-43.0664763400276));
#22588=CARTESIAN_POINT('Ctrl Pts',(6.64973892110183,-3.1569918744552,-43.0272181381386));
#22589=CARTESIAN_POINT('Ctrl Pts',(7.08294075896069,-2.00438908878645,-42.9879599362496));
#22590=CARTESIAN_POINT('Ctrl Pts',(7.21739925443971,-0.817930441030332,
-42.9487017343605));
#22591=CARTESIAN_POINT('Ctrl Pts',(7.35185774991875,0.368528206725825,-42.9094435324715));
#22592=CARTESIAN_POINT('Ctrl Pts',(7.18757290301792,1.58884271656934,-42.8701853305825));
#22593=CARTESIAN_POINT('Ctrl Pts',(6.7441341521892,2.6975019446937,-42.8309271286934));
#22594=CARTESIAN_POINT('Ctrl Pts',(6.30069540136048,3.80616117281805,-42.7916689268044));
#22595=CARTESIAN_POINT('Ctrl Pts',(5.57810274660387,4.80316511922327,-42.7524107249153));
#22596=CARTESIAN_POINT('Ctrl Pts',(4.66251863444579,5.56963034570489,-42.7131525230263));
#22597=CARTESIAN_POINT('Ctrl Pts',(3.74693452228772,6.33609557218649,-42.6738943211372));
#22598=CARTESIAN_POINT('Ctrl Pts',(2.63835895272819,6.87202207874449,-42.6346361192482));
#22599=CARTESIAN_POINT('Ctrl Pts',(1.46897924126767,7.11350561910762,-42.5953779173591));
#22600=CARTESIAN_POINT('Ctrl Pts',(0.299599529807162,7.35498915947074,-42.5561197154701));
#22601=CARTESIAN_POINT('Ctrl Pts',(-0.930584323554325,7.30202973363898,
-42.5168615135811));
#22602=CARTESIAN_POINT('Ctrl Pts',(-2.07488434768231,6.96094226007471,-42.477603311692));
#22603=CARTESIAN_POINT('Ctrl Pts',(-3.21918437181033,6.61985478651042,-42.438345109803));
#22604=CARTESIAN_POINT('Ctrl Pts',(-4.27760056670487,5.99063926521361,-42.3990869079139));
#22605=CARTESIAN_POINT('Ctrl Pts',(-5.12392665529544,5.14832378891459,-42.3598287060249));
#22606=CARTESIAN_POINT('Ctrl Pts',(-5.97025274388599,4.3060083126156,-42.3205705041358));
#22607=CARTESIAN_POINT('Ctrl Pts',(-6.60448872617259,3.25059288131442,-42.2813123022468));
#22608=CARTESIAN_POINT('Ctrl Pts',(-6.9510078661939,2.10792595896098,-42.2420541003578));
#22609=CARTESIAN_POINT('Ctrl Pts',(-7.15782376018353,1.4259385770681,-42.2186233019332));
#22610=CARTESIAN_POINT('Ctrl Pts',(-7.2621503245026,0.712870821985042,-42.1951925035086));
#22611=CARTESIAN_POINT('Ctrl Pts',(-7.26249686403911,-9.76851341781633E-5,
-42.1717617050839));
#22612=CARTESIAN_POINT('Origin',(0.,0.,-48.));
#22613=CARTESIAN_POINT('',(-7.26266111293989,0.000150415497278031,-40.6717617050839));
#22614=CARTESIAN_POINT('',(-7.26300930122575,-0.000177974604063658,-41.0782382949161));
#22615=CARTESIAN_POINT('',(-7.263,-8.89460970220723E-16,-48.));
#22616=CARTESIAN_POINT('Ctrl Pts',(-7.26300930122575,-0.000177974604063658,
-41.0782382949161));
#22617=CARTESIAN_POINT('Ctrl Pts',(-7.26209383406802,0.920961063102483,
-41.1085164870463));
#22618=CARTESIAN_POINT('Ctrl Pts',(-7.08613975434704,1.8424399406362,-41.1387946791764));
#22619=CARTESIAN_POINT('Ctrl Pts',(-6.74413418324784,2.69750195711643,-41.1690728713066));
#22620=CARTESIAN_POINT('Ctrl Pts',(-6.30069543037697,3.80616119034647,-41.2083310731957));
#22621=CARTESIAN_POINT('Ctrl Pts',(-5.57810277229263,4.80316514134317,-41.2475892750847));
#22622=CARTESIAN_POINT('Ctrl Pts',(-4.66251865591803,5.56963037135458,-41.2868474769738));
#22623=CARTESIAN_POINT('Ctrl Pts',(-3.74693453954343,6.33609560136598,-41.3261056788628));
#22624=CARTESIAN_POINT('Ctrl Pts',(-2.63835896487857,6.8720221103921,-41.3653638807518));
#22625=CARTESIAN_POINT('Ctrl Pts',(-1.46897924803272,7.11350565186732,-41.4046220826409));
#22626=CARTESIAN_POINT('Ctrl Pts',(-0.299599531186881,7.35498919334254,
-41.4438802845299));
#22627=CARTESIAN_POINT('Ctrl Pts',(0.930584327839943,7.30202976726688,-41.483138486419));
#22628=CARTESIAN_POINT('Ctrl Pts',(2.07488435723775,6.9609422921318,-41.522396688308));
#22629=CARTESIAN_POINT('Ctrl Pts',(3.21918438663557,6.61985481699672,-41.5616548901971));
#22630=CARTESIAN_POINT('Ctrl Pts',(4.27760058640437,5.99063929280222,-41.6009130920861));
#22631=CARTESIAN_POINT('Ctrl Pts',(5.1239266788925,5.14832381262414,-41.6401712939751));
#22632=CARTESIAN_POINT('Ctrl Pts',(5.97025277138064,4.30600833244604,-41.6794294958642));
#22633=CARTESIAN_POINT('Ctrl Pts',(6.6044887565881,3.25059289628436,-41.7186876977532));
#22634=CARTESIAN_POINT('Ctrl Pts',(6.95100789820523,2.10792596866861,-41.7579458996423));
#22635=CARTESIAN_POINT('Ctrl Pts',(7.29752703982237,0.965259041052854,-41.7972041015313));
#22636=CARTESIAN_POINT('Ctrl Pts',(7.35632933784919,-0.264659378016966,
-41.8364623034203));
#22637=CARTESIAN_POINT('Ctrl Pts',(7.12040316571293,-1.4351729679744,-41.8757205053094));
#22638=CARTESIAN_POINT('Ctrl Pts',(6.88447699357666,-2.60568655793184,-41.9149787071984));
#22639=CARTESIAN_POINT('Ctrl Pts',(6.35382235127733,-3.71679531877686,-41.9542369090875));
#22640=CARTESIAN_POINT('Ctrl Pts',(5.59171486435599,-4.63600987553299,-41.9934951109765));
#22641=CARTESIAN_POINT('Ctrl Pts',(4.82960737743465,-5.5552244322891,-42.0327533128656));
#22642=CARTESIAN_POINT('Ctrl Pts',(3.83604704589131,-6.28254478495629,-42.0720115147546));
#22643=CARTESIAN_POINT('Ctrl Pts',(2.72950668891924,-6.73124475304859,-42.1112697166436));
#22644=CARTESIAN_POINT('Ctrl Pts',(1.62296633194719,-7.17994472114088,-42.1505279185327));
#22645=CARTESIAN_POINT('Ctrl Pts',(0.403445949546412,-7.35002430465829,
-42.1897861204217));
#22646=CARTESIAN_POINT('Ctrl Pts',(-0.783638006780596,-7.22120309675805,
-42.2290443223108));
#22647=CARTESIAN_POINT('Ctrl Pts',(-1.9707219631076,-7.09238188885781,-42.2683025241998));
#22648=CARTESIAN_POINT('Ctrl Pts',(-3.12536949336084,-6.66465988953992,
-42.3075607260888));
#22649=CARTESIAN_POINT('Ctrl Pts',(-4.10989962967079,-5.98903896500356,
-42.3468189279779));
#22650=CARTESIAN_POINT('Ctrl Pts',(-5.09442976598076,-5.31341804046719,
-42.3860771298669));
#22651=CARTESIAN_POINT('Ctrl Pts',(-5.90884250834743,-4.38989819071233,
-42.425335331756));
#22652=CARTESIAN_POINT('Ctrl Pts',(-6.45602671966932,-3.32860055957678,
-42.4645935336451));
#22653=CARTESIAN_POINT('Ctrl Pts',(-6.98402355493559,-2.30451803138863,
-42.5024751207354));
#22654=CARTESIAN_POINT('Ctrl Pts',(-7.26320436495528,-1.15215084812863,
-42.5403567078257));
#22655=CARTESIAN_POINT('Ctrl Pts',(-7.26357703776439,4.20713134600785E-5,
-42.5782382949161));
#22656=CARTESIAN_POINT('Ctrl Pts',(-7.26249686403911,-9.76851341781633E-5,
-42.1717617050839));
#22657=CARTESIAN_POINT('Ctrl Pts',(-7.26273095000414,-0.481704842309011,
-42.1559343016195));
#22658=CARTESIAN_POINT('Ctrl Pts',(-7.2155195294283,-0.963266713190378,
-42.1401068981551));
#22659=CARTESIAN_POINT('Ctrl Pts',(-7.12040313292146,-1.43517296136506,
-42.1242794946906));
#22660=CARTESIAN_POINT('Ctrl Pts',(-6.88447696187169,-2.60568654593194,
-42.0850212928016));
#22661=CARTESIAN_POINT('Ctrl Pts',(-6.35382232201616,-3.71679530166001,
-42.0457630909126));
#22662=CARTESIAN_POINT('Ctrl Pts',(-5.59171483860454,-4.63600985418288,
-42.0065048890235));
#22663=CARTESIAN_POINT('Ctrl Pts',(-4.82960735519293,-5.55522440670574,
-41.9672466871345));
#22664=CARTESIAN_POINT('Ctrl Pts',(-3.83604702822523,-6.2825447560234,-41.9279884852454));
#22665=CARTESIAN_POINT('Ctrl Pts',(-2.72950667634911,-6.7312447220493,-41.8887302833564));
#22666=CARTESIAN_POINT('Ctrl Pts',(-1.62296632447299,-7.17994468807521,
-41.8494720814673));
#22667=CARTESIAN_POINT('Ctrl Pts',(-0.403445947688449,-7.35002427080935,
-41.8102138795783));
#22668=CARTESIAN_POINT('Ctrl Pts',(0.783638003171704,-7.22120306350237,
-41.7709556776892));
#22669=CARTESIAN_POINT('Ctrl Pts',(1.97072195403187,-7.09238185619539,-41.7316974758002));
#22670=CARTESIAN_POINT('Ctrl Pts',(3.12536947896766,-6.66465985884728,-41.6924392739112));
#22671=CARTESIAN_POINT('Ctrl Pts',(4.10989961074358,-5.98903893742233,-41.6531810720221));
#22672=CARTESIAN_POINT('Ctrl Pts',(5.0944297425195,-5.31341801599738,-41.6139228701331));
#22673=CARTESIAN_POINT('Ctrl Pts',(5.90884248113557,-4.38989817049558,-41.5746646682441));
#22674=CARTESIAN_POINT('Ctrl Pts',(6.45602668993751,-3.3286005442476,-41.535406466355));
#22675=CARTESIAN_POINT('Ctrl Pts',(7.00321089873946,-2.26730291799962,-41.496148264466));
#22676=CARTESIAN_POINT('Ctrl Pts',(7.28316657772729,-1.06822751100545,-41.4568900625769));
#22677=CARTESIAN_POINT('Ctrl Pts',(7.26251161865265,0.12564709820083,-41.4176318606879));
#22678=CARTESIAN_POINT('Ctrl Pts',(7.241856659578,1.31952170740711,-41.3783736587988));
#22679=CARTESIAN_POINT('Ctrl Pts',(6.92059106244087,2.50819551882549,-41.3391154569098));
#22680=CARTESIAN_POINT('Ctrl Pts',(6.33702275862127,3.54993024735234,-41.2998572550207));
#22681=CARTESIAN_POINT('Ctrl Pts',(5.75345445480167,4.59166497587919,-41.2605990531317));
#22682=CARTESIAN_POINT('Ctrl Pts',(4.90758344429959,5.48646062151451,-41.2213408512427));
#22683=CARTESIAN_POINT('Ctrl Pts',(3.9002719698058,6.12762113433086,-41.1820826493536));
#22684=CARTESIAN_POINT('Ctrl Pts',(2.89296049531201,6.76878164714721,-41.1428244474646));
#22685=CARTESIAN_POINT('Ctrl Pts',(1.72420855682651,7.15630702714459,-41.1035662455755));
#22686=CARTESIAN_POINT('Ctrl Pts',(0.533378941584264,7.24398848073528,-41.0643080436865));
#22687=CARTESIAN_POINT('Ctrl Pts',(-0.657450673658001,7.33166993432597,
-41.0250498417974));
#22688=CARTESIAN_POINT('Ctrl Pts',(-1.87035796565701,7.11950746150997,-40.9857916399084));
#22689=CARTESIAN_POINT('Ctrl Pts',(-2.96071503237084,6.63279946187463,-40.9465334380193));
#22690=CARTESIAN_POINT('Ctrl Pts',(-4.05107209908466,6.14609146223928,-40.9072752361303));
#22691=CARTESIAN_POINT('Ctrl Pts',(-5.0188789405133,5.38483793578459,-40.8680170342413));
#22692=CARTESIAN_POINT('Ctrl Pts',(-5.74873360138698,4.43981127804272,-40.8287588323522));
#22693=CARTESIAN_POINT('Ctrl Pts',(-6.47858826226065,3.49478462030085,-40.7895006304632));
#22694=CARTESIAN_POINT('Ctrl Pts',(-6.97049074257936,2.3659848312718,-40.7502424285742));
#22695=CARTESIAN_POINT('Ctrl Pts',(-7.16578625132404,1.18801077633428,-40.7109842266851));
#22696=CARTESIAN_POINT('Ctrl Pts',(-7.2308255886834,0.795709629973483,-40.697910052818));
#22697=CARTESIAN_POINT('Ctrl Pts',(-7.26296847415723,0.397954603469952,
-40.684835878951));
#22698=CARTESIAN_POINT('Ctrl Pts',(-7.26266111293989,0.000150415497278031,
-40.6717617050839));
#22699=CARTESIAN_POINT('Origin',(0.,0.,-48.));
#22700=CARTESIAN_POINT('',(-7.26352054254983,8.04286712641332E-5,-39.1717617050839));
#22701=CARTESIAN_POINT('',(-7.26240901964853,-7.93431878864936E-6,-39.5782382949161));
#22702=CARTESIAN_POINT('',(-7.263,-8.89460970220723E-16,-48.));
#22703=CARTESIAN_POINT('Ctrl Pts',(-7.26240901964853,-7.93431878864936E-6,
-39.5782382949161));
#22704=CARTESIAN_POINT('Ctrl Pts',(-7.26238545910871,0.606200286890817,
-39.5981598624887));
#22705=CARTESIAN_POINT('Ctrl Pts',(-7.18728432807362,1.2124142426494,-39.6180814300613));
#22706=CARTESIAN_POINT('Ctrl Pts',(-7.03717613822771,1.79944844045549,-39.638002997634));
#22707=CARTESIAN_POINT('Ctrl Pts',(-6.74136720649147,2.95628045024729,-39.677261199523));
#22708=CARTESIAN_POINT('Ctrl Pts',(-6.15427474639056,4.03862950259272,-39.716519401412));
#22709=CARTESIAN_POINT('Ctrl Pts',(-5.34590406778595,4.91743554999236,-39.7557776033011));
#22710=CARTESIAN_POINT('Ctrl Pts',(-4.53753338918133,5.79624159739201,-39.7950358051901));
#22711=CARTESIAN_POINT('Ctrl Pts',(-3.507884492073,6.47150463984588,-39.8342940070792));
#22712=CARTESIAN_POINT('Ctrl Pts',(-2.37973342110255,6.86270584644181,-39.8735522089682));
#22713=CARTESIAN_POINT('Ctrl Pts',(-1.2515823501321,7.25390705303775,-39.9128104108573));
#22714=CARTESIAN_POINT('Ctrl Pts',(-0.0249291052995126,7.36104642377576,
-39.9520686127463));
#22715=CARTESIAN_POINT('Ctrl Pts',(1.15395933445678,7.17134858619487,-39.9913268146353));
#22716=CARTESIAN_POINT('Ctrl Pts',(2.33284777421308,6.98165074861397,-40.0305850165244));
#22717=CARTESIAN_POINT('Ctrl Pts',(3.46397140889309,6.49511570271417,-40.0698432184134));
#22718=CARTESIAN_POINT('Ctrl Pts',(4.41245427615991,5.7697582229325,-40.1091014203025));
#22719=CARTESIAN_POINT('Ctrl Pts',(5.36093714342672,5.04440074315083,-40.1483596221915));
#22720=CARTESIAN_POINT('Ctrl Pts',(6.12677924328035,4.0802208294873,-40.1876178240806));
#22721=CARTESIAN_POINT('Ctrl Pts',(6.6186610355318,2.99218795984346,-40.2268760259696));
#22722=CARTESIAN_POINT('Ctrl Pts',(7.11054282778324,1.90415509019964,-40.2661342278586));
#22723=CARTESIAN_POINT('Ctrl Pts',(7.32846431243252,0.692269264575519,-40.3053924297477));
#22724=CARTESIAN_POINT('Ctrl Pts',(7.24644038134927,-0.498963415342015,
-40.3446506316367));
#22725=CARTESIAN_POINT('Ctrl Pts',(7.16441645026602,-1.69019609525955,-40.3839088335258));
#22726=CARTESIAN_POINT('Ctrl Pts',(6.78244710345024,-2.8607756294705,-40.4231670354148));
#22727=CARTESIAN_POINT('Ctrl Pts',(6.14607862926109,-3.8711213069651,-40.4624252373038));
#22728=CARTESIAN_POINT('Ctrl Pts',(5.50971015507191,-4.88146698445973,-40.5016834391929));
#22729=CARTESIAN_POINT('Ctrl Pts',(4.61894255350935,-5.73157880523801,-40.5409416410819));
#22730=CARTESIAN_POINT('Ctrl Pts',(3.57999156774745,-6.32008884946693,-40.580199842971));
#22731=CARTESIAN_POINT('Ctrl Pts',(2.54104058198559,-6.90859889369583,-40.61945804486));
#22732=CARTESIAN_POINT('Ctrl Pts',(1.3539062120244,-7.2355071613754,-40.6587162467491));
#22733=CARTESIAN_POINT('Ctrl Pts',(0.160143178906415,-7.26183288519839,
-40.6979744486381));
#22734=CARTESIAN_POINT('Ctrl Pts',(-1.03361985421157,-7.28815860902139,
-40.7372326505271));
#22735=CARTESIAN_POINT('Ctrl Pts',(-2.23401155048636,-7.01390178898781,
-40.7764908524162));
#22736=CARTESIAN_POINT('Ctrl Pts',(-3.2978963761422,-6.47176499747381,-40.8157490543052));
#22737=CARTESIAN_POINT('Ctrl Pts',(-4.36178120179806,-5.9296282059598,-40.8550072561943));
#22738=CARTESIAN_POINT('Ctrl Pts',(-5.28915915683497,-5.11961144296535,
-40.8942654580833));
#22739=CARTESIAN_POINT('Ctrl Pts',(-5.96944905428036,-4.1383016659797,-40.9335236599724));
#22740=CARTESIAN_POINT('Ctrl Pts',(-6.64973895172576,-3.15699188899405,
-40.9727818618614));
#22741=CARTESIAN_POINT('Ctrl Pts',(-7.08294079157965,-2.00438909801718,
-41.0120400637505));
#22742=CARTESIAN_POINT('Ctrl Pts',(-7.21739928767788,-0.817930444797065,
-41.0512982656395));
#22743=CARTESIAN_POINT('Ctrl Pts',(-7.24815562772976,-0.546537213020399,
-41.0602782753984));
#22744=CARTESIAN_POINT('Ctrl Pts',(-7.26328081360585,-0.273372540260897,
-41.0692582851572));
#22745=CARTESIAN_POINT('Ctrl Pts',(-7.26300930122575,-0.000177974604063658,
-41.0782382949161));
#22746=CARTESIAN_POINT('Ctrl Pts',(-7.26266111293989,0.000150415497278031,
-40.6717617050839));
#22747=CARTESIAN_POINT('Ctrl Pts',(-7.26204555169606,-0.796543594468861,
-40.6455776770619));
#22748=CARTESIAN_POINT('Ctrl Pts',(-7.13127452650012,-1.59343478733736,
-40.61939364904));
#22749=CARTESIAN_POINT('Ctrl Pts',(-6.8739323115384,-2.34710817406001,-40.593209621018));
#22750=CARTESIAN_POINT('Ctrl Pts',(-6.48809432583744,-3.47710474867077,
-40.5539514191289));
#22751=CARTESIAN_POINT('Ctrl Pts',(-5.81772981726488,-4.50994957704628,
-40.5146932172399));
#22752=CARTESIAN_POINT('Ctrl Pts',(-4.94277351217432,-5.32248552949644,
-40.4754350153508));
#22753=CARTESIAN_POINT('Ctrl Pts',(-4.06781720708377,-6.13502148194658,
-40.4361768134618));
#22754=CARTESIAN_POINT('Ctrl Pts',(-2.98826910547521,-6.72724855847138,
-40.3969186115728));
#22755=CARTESIAN_POINT('Ctrl Pts',(-1.8328552675504,-7.0285491940061,-40.3576604096837));
#22756=CARTESIAN_POINT('Ctrl Pts',(-0.677441429625552,-7.32984982954083,
-40.3184022077947));
#22757=CARTESIAN_POINT('Ctrl Pts',(0.55383814461556,-7.34022402408548,-40.2791440059056));
#22758=CARTESIAN_POINT('Ctrl Pts',(1.71416482952506,-7.05843475152745,-40.2398858040166));
#22759=CARTESIAN_POINT('Ctrl Pts',(2.87449151443453,-6.77664547896942,-40.2006276021276));
#22760=CARTESIAN_POINT('Ctrl Pts',(3.96386531001239,-6.20269273930873,-40.1613694002385));
#22761=CARTESIAN_POINT('Ctrl Pts',(4.85238853353121,-5.40501505307857,-40.1221111983495));
#22762=CARTESIAN_POINT('Ctrl Pts',(5.74091175705003,-4.6073373668484,-40.0828529964604));
#22763=CARTESIAN_POINT('Ctrl Pts',(6.42858440850981,-3.58593473404876,-40.0435947945714));
#22764=CARTESIAN_POINT('Ctrl Pts',(6.83340792666162,-2.46259990907762,-40.0043365926823));
#22765=CARTESIAN_POINT('Ctrl Pts',(7.23823144481344,-1.33926508410647,-39.9650783907933));
#22766=CARTESIAN_POINT('Ctrl Pts',(7.3602058296573,-0.11399806696383,-39.9258201889043));
#22767=CARTESIAN_POINT('Ctrl Pts',(7.1847867714185,1.06709945815779,-39.8865619870152));
#22768=CARTESIAN_POINT('Ctrl Pts',(7.0093677131797,2.24819698327945,-39.8473037851262));
#22769=CARTESIAN_POINT('Ctrl Pts',(6.53655521185824,3.38512501638008,-39.8080455832371));
#22770=CARTESIAN_POINT('Ctrl Pts',(5.82272775621115,4.34231547465169,-39.7687873813481));
#22771=CARTESIAN_POINT('Ctrl Pts',(5.10890030056408,5.29950593292327,-39.729529179459));
#22772=CARTESIAN_POINT('Ctrl Pts',(4.15405789059141,6.07695881636586,-39.69027097757));
#22773=CARTESIAN_POINT('Ctrl Pts',(3.07205659381453,6.58197010694754,-39.651012775681));
#22774=CARTESIAN_POINT('Ctrl Pts',(1.99005529703764,7.08698139752923,-39.6117545737919));
#22775=CARTESIAN_POINT('Ctrl Pts',(0.780895113456552,7.31955109525001,-39.5724963719029));
#22776=CARTESIAN_POINT('Ctrl Pts',(-0.411242862679016,7.25194742894955,
-39.5332381700138));
#22777=CARTESIAN_POINT('Ctrl Pts',(-1.60338083881458,7.1843437626491,-39.4939799681248));
#22778=CARTESIAN_POINT('Ctrl Pts',(-2.77849660750463,6.81656673232741,-39.4547217662357));
#22779=CARTESIAN_POINT('Ctrl Pts',(-3.79646855401131,6.1924703247373,-39.4154635643467));
#22780=CARTESIAN_POINT('Ctrl Pts',(-4.81444050051797,5.56837391714719,-39.3762053624577));
#22781=CARTESIAN_POINT('Ctrl Pts',(-5.67526862484128,4.68795813228867,-39.3369471605686));
#22782=CARTESIAN_POINT('Ctrl Pts',(-6.27630718772275,3.65620435557054,-39.2976889586796));
#22783=CARTESIAN_POINT('Ctrl Pts',(-6.87734575060422,2.62445057885241,-39.2584307567905));
#22784=CARTESIAN_POINT('Ctrl Pts',(-7.21859475204387,1.44135881027467,-39.2191725549015));
#22785=CARTESIAN_POINT('Ctrl Pts',(-7.2593634257495,0.248001728306349,-39.1799143530124));
#22786=CARTESIAN_POINT('Ctrl Pts',(-7.2621855336339,0.165394615447164,-39.1771968037029));
#22787=CARTESIAN_POINT('Ctrl Pts',(-7.26356781521829,0.0827383137831455,
-39.1744792543934));
#22788=CARTESIAN_POINT('Ctrl Pts',(-7.26352054254983,8.04286712641332E-5,
-39.1717617050839));
#22789=CARTESIAN_POINT('Origin',(0.,0.,-48.));
#22790=CARTESIAN_POINT('',(-7.26313420453275,-0.000171068891272981,-37.6717617050839));
#22791=CARTESIAN_POINT('',(-7.26295522622064,0.000178426625192518,-38.0782382949161));
#22792=CARTESIAN_POINT('',(-7.263,-8.89460970220723E-16,-48.));
#22793=CARTESIAN_POINT('Ctrl Pts',(-7.26295522622064,0.000178426625192518,
-38.0782382949161));
#22794=CARTESIAN_POINT('Ctrl Pts',(-7.26324087904769,0.291174376834878,
-38.0878032379312));
#22795=CARTESIAN_POINT('Ctrl Pts',(-7.24607581082464,0.582136841251713,
-38.0973681809462));
#22796=CARTESIAN_POINT('Ctrl Pts',(-7.21119217782702,0.870959278336532,
-38.1069331239613));
#22797=CARTESIAN_POINT('Ctrl Pts',(-7.06801634241581,2.05639755301244,-38.1461913258504));
#22798=CARTESIAN_POINT('Ctrl Pts',(-6.62635408862456,3.20578499051862,-38.1854495277394));
#22799=CARTESIAN_POINT('Ctrl Pts',(-5.93886952815666,4.1820678399582,-38.2247077296284));
#22800=CARTESIAN_POINT('Ctrl Pts',(-5.25138496768876,5.15835068939778,-38.2639659315175));
#22801=CARTESIAN_POINT('Ctrl Pts',(-4.31807810054421,5.96152895077076,-38.3032241334065));
#22802=CARTESIAN_POINT('Ctrl Pts',(-3.25023708129094,6.49583109429408,-38.3424823352956));
#22803=CARTESIAN_POINT('Ctrl Pts',(-2.18239606203769,7.03013323781739,-38.3817405371846));
#22804=CARTESIAN_POINT('Ctrl Pts',(-0.980020890675717,7.29555926349104,
-38.4209987390737));
#22805=CARTESIAN_POINT('Ctrl Pts',(0.213516388094846,7.26045958892129,-38.4602569409627));
#22806=CARTESIAN_POINT('Ctrl Pts',(1.40705366686543,7.22535991435153,-38.4995151428517));
#22807=CARTESIAN_POINT('Ctrl Pts',(2.5917530530446,6.88973453953835,-38.5387733447408));
#22808=CARTESIAN_POINT('Ctrl Pts',(3.62635017472901,6.29360366566943,-38.5780315466298));
#22809=CARTESIAN_POINT('Ctrl Pts',(4.66094729641343,5.69747279180051,-38.6172897485189));
#22810=CARTESIAN_POINT('Ctrl Pts',(5.54544215360309,4.84083641887585,-38.6565479504079));
#22811=CARTESIAN_POINT('Ctrl Pts',(6.17436696949242,3.82584045881966,-38.6958061522969));
#22812=CARTESIAN_POINT('Ctrl Pts',(6.80329178538175,2.81084449876349,-38.735064354186));
#22813=CARTESIAN_POINT('Ctrl Pts',(7.17664655997076,1.63748895157579,-38.774322556075));
#22814=CARTESIAN_POINT('Ctrl Pts',(7.24991221243256,0.445685541971607,-38.8135807579641));
#22815=CARTESIAN_POINT('Ctrl Pts',(7.32317786489436,-0.74611786763258,-38.8528389598531));
#22816=CARTESIAN_POINT('Ctrl Pts',(7.09635439522896,-1.95636913965326,-38.8920971617422));
#22817=CARTESIAN_POINT('Ctrl Pts',(6.5964883904005,-3.0407570777042,-38.9313553636312));
#22818=CARTESIAN_POINT('Ctrl Pts',(6.09662238557205,-4.12514501575514,-38.9706135655202));
#22819=CARTESIAN_POINT('Ctrl Pts',(5.32371384558054,-5.08366961983634,-39.0098717674093));
#22820=CARTESIAN_POINT('Ctrl Pts',(4.36992491781035,-5.80203575506052,-39.0491299692983));
#22821=CARTESIAN_POINT('Ctrl Pts',(3.41613599004017,-6.52040189028469,-39.0883881711874));
#22822=CARTESIAN_POINT('Ctrl Pts',(2.28146667449132,-6.99860955665184,-39.1276463730764));
#22823=CARTESIAN_POINT('Ctrl Pts',(1.10121572293315,-7.1796369422042,-39.1669045749655));
#22824=CARTESIAN_POINT('Ctrl Pts',(-0.0790352286250597,-7.36066432775656,
-39.2061627768545));
#22825=CARTESIAN_POINT('Ctrl Pts',(-1.30486781619259,-7.24451143249411,
-39.2454209787435));
#22826=CARTESIAN_POINT('Ctrl Pts',(-2.43011291656941,-6.84502840775857,
-39.2846791806326));
#22827=CARTESIAN_POINT('Ctrl Pts',(-3.55535801694622,-6.44554538302304,
-39.3239373825216));
#22828=CARTESIAN_POINT('Ctrl Pts',(-4.58001563013233,-5.76273222881443,
-39.3631955844107));
#22829=CARTESIAN_POINT('Ctrl Pts',(-5.38190487562348,-4.87800805657794,
-39.4024537862997));
#22830=CARTESIAN_POINT('Ctrl Pts',(-6.18379412111464,-3.99328388434143,
-39.4417119881888));
#22831=CARTESIAN_POINT('Ctrl Pts',(-6.76291499891085,-2.90664869407702,
-39.4809701900778));
#22832=CARTESIAN_POINT('Ctrl Pts',(-7.05021273612318,-1.74767361532571,
-39.5202283919668));
#22833=CARTESIAN_POINT('Ctrl Pts',(-7.19172128763834,-1.17682023434321,
-39.5395650262832));
#22834=CARTESIAN_POINT('Ctrl Pts',(-7.26243188840829,-0.588416785700682,
-39.5589016605997));
#22835=CARTESIAN_POINT('Ctrl Pts',(-7.26240901964853,-7.93431878864936E-6,
-39.5782382949161));
#22836=CARTESIAN_POINT('Ctrl Pts',(-7.26352054254983,8.04286712641332E-5,
-39.1717617050839));
#22837=CARTESIAN_POINT('Ctrl Pts',(-7.2628849058206,-1.11135223320081,-39.1352210525044));
#22838=CARTESIAN_POINT('Ctrl Pts',(-7.00378627314357,-2.22307118198899,
-39.0986803999249));
#22839=CARTESIAN_POINT('Ctrl Pts',(-6.51119666041538,-3.21934469321509,
-39.0621397473453));
#22840=CARTESIAN_POINT('Ctrl Pts',(-5.98197287540399,-4.28971163740927,
-39.0228815454563));
#22841=CARTESIAN_POINT('Ctrl Pts',(-5.18323695940958,-5.22682313043868,
-38.9836233435672));
#22842=CARTESIAN_POINT('Ctrl Pts',(-4.21023073394239,-5.91893735153225,
-38.9443651416782));
#22843=CARTESIAN_POINT('Ctrl Pts',(-3.23722450847519,-6.61105157262582,
-38.9051069397891));
#22844=CARTESIAN_POINT('Ctrl Pts',(-2.08994797353521,-7.05816852178353,
-38.8658487379001));
#22845=CARTESIAN_POINT('Ctrl Pts',(-0.90520317443169,-7.20697366564122,
-38.8265905360111));
#22846=CARTESIAN_POINT('Ctrl Pts',(0.279541624671835,-7.3557788094989,-38.787332334122));
#22847=CARTESIAN_POINT('Ctrl Pts',(1.5017546879389,-7.20627214805655,-38.748074132233));
#22848=CARTESIAN_POINT('Ctrl Pts',(2.61569848675283,-6.77628095867734,-38.7088159303439));
#22849=CARTESIAN_POINT('Ctrl Pts',(3.72964228556675,-6.34628976929814,-38.6695577284549));
#22850=CARTESIAN_POINT('Ctrl Pts',(4.73531681992753,-5.63581405198208,-38.6302995265658));
#22851=CARTESIAN_POINT('Ctrl Pts',(5.51280476472356,-4.72957142140441,-38.5910413246768));
#22852=CARTESIAN_POINT('Ctrl Pts',(6.29029270951958,-3.82332879082673,-38.5517831227878));
#22853=CARTESIAN_POINT('Ctrl Pts',(6.83959406475085,-2.72131924698744,-38.5125249208987));
#22854=CARTESIAN_POINT('Ctrl Pts',(7.09520975800467,-1.554947167695,-38.4732667190097));
#22855=CARTESIAN_POINT('Ctrl Pts',(7.35082545125849,-0.388575088402531,
-38.4340085171206));
#22856=CARTESIAN_POINT('Ctrl Pts',(7.31275548253484,0.842159526343091,-38.3947503152316));
#22857=CARTESIAN_POINT('Ctrl Pts',(6.98553934108194,1.99050303171896,-38.3554921133426));
#22858=CARTESIAN_POINT('Ctrl Pts',(6.65832319962904,3.13884653709483,-38.3162339114535));
#22859=CARTESIAN_POINT('Ctrl Pts',(6.04196088544689,4.20479893310094,-38.2769757095645));
#22860=CARTESIAN_POINT('Ctrl Pts',(5.20994786614568,5.06125532190715,-38.2377175076754));
#22861=CARTESIAN_POINT('Ctrl Pts',(4.37793484684449,5.91771171071335,-38.1984593057864));
#22862=CARTESIAN_POINT('Ctrl Pts',(3.33027112242425,6.56467209231964,-38.1592011038973));
#22863=CARTESIAN_POINT('Ctrl Pts',(2.1918808376328,6.92499246246351,-38.1199429020083));
#22864=CARTESIAN_POINT('Ctrl Pts',(1.05349055284132,7.28531283260738,-38.0806847001193));
#22865=CARTESIAN_POINT('Ctrl Pts',(-0.175626292321373,7.35899319128881,
-38.0414264982302));
#22866=CARTESIAN_POINT('Ctrl Pts',(-1.34890895684957,7.13724784608893,-38.0021682963412));
#22867=CARTESIAN_POINT('Ctrl Pts',(-2.52219162137778,6.91550250088904,-37.9629100944521));
#22868=CARTESIAN_POINT('Ctrl Pts',(-3.63964010527149,6.39833145180785,-37.9236518925631));
#22869=CARTESIAN_POINT('Ctrl Pts',(-4.56800908195572,5.64740252255931,-37.884393690674));
#22870=CARTESIAN_POINT('Ctrl Pts',(-5.4963780586399,4.89647359331081,-37.845135488785));
#22871=CARTESIAN_POINT('Ctrl Pts',(-6.23566752811461,3.911786783895,-37.805877286896));
#22872=CARTESIAN_POINT('Ctrl Pts',(-6.69772410140762,2.81075684662822,-37.7666190850069));
#22873=CARTESIAN_POINT('Ctrl Pts',(-7.06987118413825,1.92397132546851,-37.7349999583659));
#22874=CARTESIAN_POINT('Ctrl Pts',(-7.2621793435513,0.961714880272418,-37.7033808317249));
#22875=CARTESIAN_POINT('Ctrl Pts',(-7.26313420453275,-0.000171068891272981,
-37.6717617050839));
#22876=CARTESIAN_POINT('Origin',(0.,0.,-48.));
#22877=CARTESIAN_POINT('',(-7.26243100057087,-0.00011786593126363,-36.1717617050839));
#22878=CARTESIAN_POINT('',(-7.26359129981488,-2.41004779799603E-5,-36.5782382949161));
#22879=CARTESIAN_POINT('',(-7.263,-8.89460970220723E-16,-48.));
#22880=CARTESIAN_POINT('',(-5.46288453460435,-4.78623668048088,-36.));
#22881=CARTESIAN_POINT('Ctrl Pts',(-7.26243100057087,-0.00011786593126363,
-36.1717617050839));
#22882=CARTESIAN_POINT('Ctrl Pts',(-7.26254766902496,-0.547742115475237,
-36.1537660052783));
#22883=CARTESIAN_POINT('Ctrl Pts',(-7.2013797096861,-1.09531506383856,-36.1357703054727));
#22884=CARTESIAN_POINT('Ctrl Pts',(-7.07862623058799,-1.62865307118789,
-36.1177746056671));
#22885=CARTESIAN_POINT('Ctrl Pts',(-6.81083554075238,-2.79214720555352,
-36.0785164037781));
#22886=CARTESIAN_POINT('Ctrl Pts',(-6.24995421752147,-3.88789606644511,
-36.039258201889));
#22887=CARTESIAN_POINT('Ctrl Pts',(-5.46288453460428,-4.78623668048096,
-36.));
#22888=CARTESIAN_POINT('',(5.46288453460446,-4.78623668048075,-36.));
#22889=CARTESIAN_POINT('Origin',(0.,0.,-36.));
#22890=CARTESIAN_POINT('Ctrl Pts',(5.46328275624298,-4.78643223329959,-36.));
#22891=CARTESIAN_POINT('Ctrl Pts',(4.76265403019709,-5.58484238403501,-36.0349216092067));
#22892=CARTESIAN_POINT('Ctrl Pts',(3.88494973086336,-6.22857884933557,-36.0698432184135));
#22893=CARTESIAN_POINT('Ctrl Pts',(2.91187905542927,-6.65437827772981,-36.1047648276202));
#22894=CARTESIAN_POINT('Ctrl Pts',(1.81797170418512,-7.13305381141417,-36.1440230295092));
#22895=CARTESIAN_POINT('Ctrl Pts',(0.603542002707702,-7.33630434768437,
-36.1832812313982));
#22896=CARTESIAN_POINT('Ctrl Pts',(-0.586609857006575,-7.23987449212561,
-36.2225394332873));
#22897=CARTESIAN_POINT('Ctrl Pts',(-1.77676171672083,-7.14344463656685,
-36.2617976351763));
#22898=CARTESIAN_POINT('Ctrl Pts',(-2.94263573467192,-6.74733438917911,
-36.3010558370653));
#22899=CARTESIAN_POINT('Ctrl Pts',(-3.94520774032596,-6.0987858833362,-36.3403140389544));
#22900=CARTESIAN_POINT('Ctrl Pts',(-4.94777974598003,-5.45023737749328,
-36.3795722408435));
#22901=CARTESIAN_POINT('Ctrl Pts',(-5.78704973933708,-4.54925061319516,
-36.4188304427325));
#22902=CARTESIAN_POINT('Ctrl Pts',(-6.36294482586013,-3.50325511296896,
-36.4580886446215));
#22903=CARTESIAN_POINT('Ctrl Pts',(-6.93883991238317,-2.45725961274279,
-36.4973468465106));
#22904=CARTESIAN_POINT('Ctrl Pts',(-7.25136009207222,-1.26625537658855,
-36.5366050483996));
#22905=CARTESIAN_POINT('Ctrl Pts',(-7.26323914168565,-0.0722609137693696,
-36.5758632502886));
#22906=CARTESIAN_POINT('Ctrl Pts',(-7.26347869479477,-0.0481828018704033,
-36.5766549318311));
#22907=CARTESIAN_POINT('Ctrl Pts',(-7.26359598671164,-0.0241034739412912,
-36.5774466133736));
#22908=CARTESIAN_POINT('Ctrl Pts',(-7.26359129981488,-2.41004779799603E-5,
-36.5782382949161));
#22909=CARTESIAN_POINT('Origin',(0.,0.,-51.3123464956316));
#22910=CARTESIAN_POINT('',(-8.10164969819937,-0.000190818480503285,-37.1876535043684));
#22911=CARTESIAN_POINT('',(-8.10215956429164,-2.68828339804187E-5,-37.0623464956316));
#22912=CARTESIAN_POINT('',(-8.1015,-2.19835914433334E-13,-51.3123464956316));
#22913=CARTESIAN_POINT('',(2.10185380438477,7.82409821225381,-36.));
#22914=CARTESIAN_POINT('Ctrl Pts',(-8.10215956429164,-2.6882833979924E-5,
-37.0623464956316));
#22915=CARTESIAN_POINT('Ctrl Pts',(-8.10216479228202,-0.0268861757036945,
-37.0615548140891));
#22916=CARTESIAN_POINT('Ctrl Pts',(-8.09554616061823,-1.38565160926748,
-37.0215049306576));
#22917=CARTESIAN_POINT('Ctrl Pts',(-7.39131616610511,-4.06944920443886,
-36.942196845337));
#22918=CARTESIAN_POINT('Ctrl Pts',(-4.58282965177962,-7.08446129488128,
-36.8244222396699));
#22919=CARTESIAN_POINT('Ctrl Pts',(-0.681413560730255,-8.40998263697618,
-36.7066476340027));
#22920=CARTESIAN_POINT('Ctrl Pts',(3.38248657413956,-7.72983632570271,-36.5888730283357));
#22921=CARTESIAN_POINT('Ctrl Pts',(6.63976810478354,-5.20635617176029,-36.4710984226685));
#22922=CARTESIAN_POINT('Ctrl Pts',(8.31350431780115,-1.44107773576215,-36.3533238170014));
#22923=CARTESIAN_POINT('Ctrl Pts',(8.00479582109024,2.66750482517421,-36.2355492113343));
#22924=CARTESIAN_POINT('Ctrl Pts',(5.78674112666189,6.14069293294423,-36.1177746056671));
#22925=CARTESIAN_POINT('Ctrl Pts',(3.38848271769057,7.47846018434309,-36.039258201889));
#22926=CARTESIAN_POINT('Ctrl Pts',(2.10185380438477,7.82409821225381,-36.));
#22927=CARTESIAN_POINT('',(-2.10185380438507,7.82409821225373,-36.));
#22928=CARTESIAN_POINT('Origin',(0.,0.,-36.));
#22929=CARTESIAN_POINT('Ctrl Pts',(-8.10164969819937,-0.000190818480503216,
-37.1876535043684));
#22930=CARTESIAN_POINT('Ctrl Pts',(-8.10190702229628,-0.259408063727026,
-37.1800144291204));
#22931=CARTESIAN_POINT('Ctrl Pts',(-8.02700216464902,-1.85062837958727,
-37.1331171519833));
#22932=CARTESIAN_POINT('Ctrl Pts',(-7.01423999417884,-4.68960618017365,
-37.0469616729571));
#22933=CARTESIAN_POINT('Ctrl Pts',(-3.95702765317846,-7.45210691888099,
-36.92918706729));
#22934=CARTESIAN_POINT('Ctrl Pts',(0.0438619977836959,-8.43741959751058,
-36.8114124616229));
#22935=CARTESIAN_POINT('Ctrl Pts',(4.03429158844322,-7.41056343594989,-36.6936378559558));
#22936=CARTESIAN_POINT('Ctrl Pts',(7.06261733076329,-4.61642867900756,-36.5758632502887));
#22937=CARTESIAN_POINT('Ctrl Pts',(8.40664121397815,-0.721355965422936,
-36.4580886446215));
#22938=CARTESIAN_POINT('Ctrl Pts',(7.74583594905282,3.34573518158168,-36.3403140389544));
#22939=CARTESIAN_POINT('Ctrl Pts',(5.23779660784082,6.61495421252791,-36.2225394332873));
#22940=CARTESIAN_POINT('Ctrl Pts',(1.61897602708266,8.24429461880617,-36.1091014203025));
#22941=CARTESIAN_POINT('Ctrl Pts',(-0.957565004786227,8.13102710041623,
-36.0349216092067));
#22942=CARTESIAN_POINT('Ctrl Pts',(-2.10210198597168,7.82452632564983,-36.));
#22943=CARTESIAN_POINT('Origin',(0.,0.,-51.3123464956316));
#22944=CARTESIAN_POINT('',(-8.10208063823041,8.97140133537117E-5,-38.6876535043684));
#22945=CARTESIAN_POINT('',(-8.10145005717011,0.000199025651108617,-38.5623464956316));
#22946=CARTESIAN_POINT('',(-8.1015,-2.19835914433334E-13,-51.3123464956316));
#22947=CARTESIAN_POINT('Ctrl Pts',(-8.10145005717011,0.000199025651108561,
-38.5623464956316));
#22948=CARTESIAN_POINT('Ctrl Pts',(-8.10046090434358,-1.00745585958161,
-38.5326532367576));
#22949=CARTESIAN_POINT('Ctrl Pts',(-7.66255247376433,-3.34819241285004,
-38.4637017759946));
#22950=CARTESIAN_POINT('Ctrl Pts',(-5.46347918924325,-6.4298027756069,-38.3554921133425));
#22951=CARTESIAN_POINT('Ctrl Pts',(-1.76708585226559,-8.25041672623214,
-38.2377175076754));
#22952=CARTESIAN_POINT('Ctrl Pts',(2.35072455830847,-8.10345991964222,-38.1199429020083));
#22953=CARTESIAN_POINT('Ctrl Pts',(5.90793092950644,-6.02397880472869,-38.0021682963412));
#22954=CARTESIAN_POINT('Ctrl Pts',(8.05620579157874,-2.50789093275115,-37.8843936906741));
#22955=CARTESIAN_POINT('Ctrl Pts',(8.28322556673132,1.60628226439634,-37.7666190850069));
#22956=CARTESIAN_POINT('Ctrl Pts',(6.53485031734875,5.33738697798904,-37.6488444793398));
#22957=CARTESIAN_POINT('Ctrl Pts',(3.22803487993391,7.79562443188376,-37.5310698736727));
#22958=CARTESIAN_POINT('Ctrl Pts',(-0.848606625837317,8.39475031472183,
-37.4132952680055));
#22959=CARTESIAN_POINT('Ctrl Pts',(-4.72287154262983,6.99188517896739,-37.2955206623384));
#22960=CARTESIAN_POINT('Ctrl Pts',(-7.4523472329625,3.94222294771503,-37.1785377382137));
#22961=CARTESIAN_POINT('Ctrl Pts',(-8.10190554473014,1.30502253442654,-37.1008130159782));
#22962=CARTESIAN_POINT('Ctrl Pts',(-8.10215956429164,-2.6882833979924E-5,
-37.0623464956316));
#22963=CARTESIAN_POINT('Ctrl Pts',(-8.10208063823041,8.97140133539198E-5,
-38.6876535043684));
#22964=CARTESIAN_POINT('Ctrl Pts',(-8.10137161840911,-1.23965580576583,
-38.6511128517889));
#22965=CARTESIAN_POINT('Ctrl Pts',(-7.50185551031583,-3.81200985713521,
-38.5753139973203));
#22966=CARTESIAN_POINT('Ctrl Pts',(-4.89068362979871,-6.87554954592136,
-38.4602569409627));
#22967=CARTESIAN_POINT('Ctrl Pts',(-1.05150112347229,-8.3717568832205,-38.3424823352955));
#22968=CARTESIAN_POINT('Ctrl Pts',(3.03844482120267,-7.87145609112005,-38.2247077296284));
#22969=CARTESIAN_POINT('Ctrl Pts',(6.40377825371979,-5.49395959222041,-38.1069331239613));
#22970=CARTESIAN_POINT('Ctrl Pts',(8.24192981481277,-1.80625603195024,-37.9891585182942));
#22971=CARTESIAN_POINT('Ctrl Pts',(8.11453458490175,2.31220595952502,-37.871383912627));
#22972=CARTESIAN_POINT('Ctrl Pts',(6.05197395361438,5.87924988197173,-37.7536093069599));
#22973=CARTESIAN_POINT('Ctrl Pts',(2.54613022648071,8.0442021874585,-37.6358347012928));
#22974=CARTESIAN_POINT('Ctrl Pts',(-1.56691815067151,8.29076204944015,-37.5180600956257));
#22975=CARTESIAN_POINT('Ctrl Pts',(-5.30628572285852,6.56012956115795,-37.4002854899586));
#22976=CARTESIAN_POINT('Ctrl Pts',(-7.61974018825314,3.47875455134372,-37.2901499595394));
#22977=CARTESIAN_POINT('Ctrl Pts',(-8.10058460027276,1.07274309548756,-37.2192726310094));
#22978=CARTESIAN_POINT('Ctrl Pts',(-8.10164969819937,-0.000190818480503216,
-37.1876535043684));
#22979=CARTESIAN_POINT('Origin',(0.,0.,-51.3123464956316));
#22980=CARTESIAN_POINT('',(-8.1011219890517,0.00016778068961748,-40.1876535043684));
#22981=CARTESIAN_POINT('',(-8.10084079205323,-8.85032130801111E-6,-40.0623464956316));
#22982=CARTESIAN_POINT('',(-8.1015,-2.19835914433334E-13,-51.3123464956316));
#22983=CARTESIAN_POINT('Ctrl Pts',(-8.10084079205322,-8.85032130713836E-6,
-40.0623464956316));
#22984=CARTESIAN_POINT('Ctrl Pts',(-8.10086630096926,-0.656348422050696,
-40.0430098613152));
#22985=CARTESIAN_POINT('Ctrl Pts',(-7.86185833292864,-2.64520314986847,
-39.9844150251097));
#22986=CARTESIAN_POINT('Ctrl Pts',(-6.25172246740249,-5.66638639445397,
-39.8865619870152));
#22987=CARTESIAN_POINT('Ctrl Pts',(-2.82286511373573,-7.95131442783728,
-39.768787381348));
#22988=CARTESIAN_POINT('Ctrl Pts',(1.27919300612309,-8.34000202840266,-39.651012775681));
#22989=CARTESIAN_POINT('Ctrl Pts',(5.07618741335941,-6.73975444101172,-39.5332381700138));
#22990=CARTESIAN_POINT('Ctrl Pts',(7.66260564414886,-3.53220091768916,-39.4154635643467));
#22991=CARTESIAN_POINT('Ctrl Pts',(8.42163511110229,0.517716752808797,-39.2976889586796));
#22992=CARTESIAN_POINT('Ctrl Pts',(7.17226141992802,4.4441686179642,-39.1799143530125));
#22993=CARTESIAN_POINT('Ctrl Pts',(4.21243693189744,7.31076902079321,-39.0621397473453));
#22994=CARTESIAN_POINT('Ctrl Pts',(0.248024673685762,8.43388714307694,-38.9443651416782));
#22995=CARTESIAN_POINT('Ctrl Pts',(-3.77553685080373,7.54568022568945,-38.8265905360111));
#22996=CARTESIAN_POINT('Ctrl Pts',(-6.89870313918519,4.85796907966996,-38.7088159303439));
#22997=CARTESIAN_POINT('Ctrl Pts',(-8.0040363497543,1.98143594698576,-38.6207345835508));
#22998=CARTESIAN_POINT('Ctrl Pts',(-8.10176868809099,0.324789923437666,
-38.5719114386467));
#22999=CARTESIAN_POINT('Ctrl Pts',(-8.10145005717011,0.000199025651108561,
-38.5623464956316));
#23000=CARTESIAN_POINT('Ctrl Pts',(-8.1011219890517,0.000167780689617515,
-40.1876535043684));
#23001=CARTESIAN_POINT('Ctrl Pts',(-8.10043536239369,-0.888503088336933,
-40.1614694763464));
#23002=CARTESIAN_POINT('Ctrl Pts',(-7.73586399862886,-3.11012449507375,
-40.0960272464354));
#23003=CARTESIAN_POINT('Ctrl Pts',(-5.74161917229395,-6.18269983140913,
-39.9913268146354));
#23004=CARTESIAN_POINT('Ctrl Pts',(-2.12907933537458,-8.16449564324956,
-39.8735522089682));
#23005=CARTESIAN_POINT('Ctrl Pts',(1.9912062783033,-8.19921127195815,-39.7557776033011));
#23006=CARTESIAN_POINT('Ctrl Pts',(5.63662627205554,-6.27856768651366,-39.638002997634));
#23007=CARTESIAN_POINT('Ctrl Pts',(7.93781585726883,-2.86060261851435,-39.5202283919668));
#23008=CARTESIAN_POINT('Ctrl Pts',(8.3459841673938,1.23956290787192,-39.4024537862997));
#23009=CARTESIAN_POINT('Ctrl Pts',(6.76379066080322,5.0441157621324,-39.2846791806326));
#23010=CARTESIAN_POINT('Ctrl Pts',(3.56855902743119,7.64574093157071,-39.1669045749655));
#23011=CARTESIAN_POINT('Ctrl Pts',(-0.477707485283489,8.42399925709112,
-39.0491299692983));
#23012=CARTESIAN_POINT('Ctrl Pts',(-4.4100496579569,7.19329061968874,-38.9313553636312));
#23013=CARTESIAN_POINT('Ctrl Pts',(-7.29067710496446,4.24711611286043,-38.8135807579641));
#23014=CARTESIAN_POINT('Ctrl Pts',(-8.07831747062495,1.51640970996623,-38.7323468048765));
#23015=CARTESIAN_POINT('Ctrl Pts',(-8.10213336844155,0.09229030002937,-38.6903710536779));
#23016=CARTESIAN_POINT('Ctrl Pts',(-8.10208063823041,8.97140133539198E-5,
-38.6876535043684));
#23017=CARTESIAN_POINT('Origin',(0.,0.,-51.3123464956316));
#23018=CARTESIAN_POINT('',(-8.10093877791723,-0.000108962703712356,-41.6876535043684));
#23019=CARTESIAN_POINT('',(-8.10151037503517,-0.000198521445029568,-41.5623464956316));
#23020=CARTESIAN_POINT('',(-8.1015,-2.19835914433334E-13,-51.3123464956316));
#23021=CARTESIAN_POINT('Ctrl Pts',(-8.10151037503517,-0.000198521445028341,
-41.5623464956316));
#23022=CARTESIAN_POINT('Ctrl Pts',(-8.10181323302049,-0.304932897552518,
-41.5533664858727));
#23023=CARTESIAN_POINT('Ctrl Pts',(-8.01118479339215,-1.9417053813148,-41.5051282742248));
#23024=CARTESIAN_POINT('Ctrl Pts',(-6.93422489492358,-4.80712946437895,
-41.4176318606879));
#23025=CARTESIAN_POINT('Ctrl Pts',(-3.83089878888002,-7.51772459259022,
-41.2998572550207));
#23026=CARTESIAN_POINT('Ctrl Pts',(0.186025344688875,-8.43548238998882,
-41.1820826493536));
#23027=CARTESIAN_POINT('Ctrl Pts',(4.15858589745246,-7.3415347110933,-41.0643080436865));
#23028=CARTESIAN_POINT('Ctrl Pts',(7.13940114902576,-4.49676770736134,-40.9465334380193));
#23029=CARTESIAN_POINT('Ctrl Pts',(8.41760216646814,-0.579605337923066,
-40.8287588323522));
#23030=CARTESIAN_POINT('Ctrl Pts',(7.68836180798567,3.47578211201243,-40.7109842266851));
#23031=CARTESIAN_POINT('Ctrl Pts',(5.12559032018552,6.70226024937101,-40.593209621018));
#23032=CARTESIAN_POINT('Ctrl Pts',(1.34046098257293,8.33037411734177,-40.4754350153508));
#23033=CARTESIAN_POINT('Ctrl Pts',(-2.76434333919955,7.97184887486595,-40.3576604096838));
#23034=CARTESIAN_POINT('Ctrl Pts',(-6.20990324829623,5.71218611631991,-40.2398858040166));
#23035=CARTESIAN_POINT('Ctrl Pts',(-7.85195993614671,2.68493126162982,-40.1414478326659));
#23036=CARTESIAN_POINT('Ctrl Pts',(-8.10081451149239,0.676184995765657,
-40.0822680632042));
#23037=CARTESIAN_POINT('Ctrl Pts',(-8.10084079205322,-8.85032130713836E-6,
-40.0623464956316));
#23038=CARTESIAN_POINT('Ctrl Pts',(-8.10093877791723,-0.000108962703712148,
-41.6876535043684));
#23039=CARTESIAN_POINT('Ctrl Pts',(-8.10119988867663,-0.537316780940126,
-41.671826100904));
#23040=CARTESIAN_POINT('Ctrl Pts',(-7.9179157370419,-2.40683601775939,-41.6167404955505));
#23041=CARTESIAN_POINT('Ctrl Pts',(-6.49544168759803,-5.38527670672303,
-41.522396688308));
#23042=CARTESIAN_POINT('Ctrl Pts',(-3.17064656618999,-7.81914114703574,
-41.4046220826409));
#23043=CARTESIAN_POINT('Ctrl Pts',(0.910288721922364,-8.38828602085676,
-41.2868474769737));
#23044=CARTESIAN_POINT('Ctrl Pts',(4.77413709997572,-6.95698087359707,-41.1690728713066));
#23045=CARTESIAN_POINT('Ctrl Pts',(7.4994426769679,-3.86656533112174,-41.0512982656395));
#23046=CARTESIAN_POINT('Ctrl Pts',(8.43627081960314,0.145954045071271,-40.9335236599723));
#23047=CARTESIAN_POINT('Ctrl Pts',(7.36120546016224,4.12366609926623,-40.8157490543053));
#23048=CARTESIAN_POINT('Ctrl Pts',(4.53062966851309,7.11796057391082,-40.6979744486381));
#23049=CARTESIAN_POINT('Ctrl Pts',(0.619583063952851,8.41475399235312,-40.5801998429711));
#23050=CARTESIAN_POINT('Ctrl Pts',(-3.43922256435361,7.70478527136227,-40.4624252373038));
#23051=CARTESIAN_POINT('Ctrl Pts',(-6.67783765143915,5.15736873085314,-40.3446506316368));
#23052=CARTESIAN_POINT('Ctrl Pts',(-7.95795209728732,2.21980900261142,-40.2530600539916));
#23053=CARTESIAN_POINT('Ctrl Pts',(-8.10146483455665,0.443897730966563,
-40.2007276782355));
#23054=CARTESIAN_POINT('Ctrl Pts',(-8.1011219890517,0.000167780689617515,
-40.1876535043684));
#23055=CARTESIAN_POINT('Origin',(0.,0.,-51.3123464956316));
#23056=CARTESIAN_POINT('',(-8.10186514679612,-0.000159416706437265,-43.1876535043684));
#23057=CARTESIAN_POINT('',(-8.10214365571365,4.6928369269332E-5,-43.0623464956316));
#23058=CARTESIAN_POINT('',(-8.1015,-2.19835914433334E-13,-51.3123464956316));
#23059=CARTESIAN_POINT('Ctrl Pts',(-8.10214365571365,4.69283692696408E-5,
-43.0623464956316));
#23060=CARTESIAN_POINT('Ctrl Pts',(-8.10172795851372,-1.28516454579568,
-43.0244649085412));
#23061=CARTESIAN_POINT('Ctrl Pts',(-7.46758783086871,-3.90268783700937,
-42.9473251195619));
#23062=CARTESIAN_POINT('Ctrl Pts',(-4.77413712196194,-6.95698090563593,
-42.8309271286933));
#23063=CARTESIAN_POINT('Ctrl Pts',(-0.910288726114504,-8.38828605948718,
-42.7131525230263));
#23064=CARTESIAN_POINT('Ctrl Pts',(3.17064658079171,-7.8191411830451,-42.5953779173591));
#23065=CARTESIAN_POINT('Ctrl Pts',(6.49544171751139,-5.38527673152374,-42.477603311692));
#23066=CARTESIAN_POINT('Ctrl Pts',(8.27119495360724,-1.66712405660176,-42.3598287060249));
#23067=CARTESIAN_POINT('Ctrl Pts',(8.07442220785581,2.44860666297451,-42.2420541003577));
#23068=CARTESIAN_POINT('Ctrl Pts',(5.95205011609281,5.98039028794925,-42.1242794946906));
#23069=CARTESIAN_POINT('Ctrl Pts',(2.41022490236832,8.08596218768562,-42.0065048890235));
#23070=CARTESIAN_POINT('Ctrl Pts',(-1.70639407074438,8.26318267110237,-41.8887302833564));
#23071=CARTESIAN_POINT('Ctrl Pts',(-5.41606983206093,6.46978795285578,-41.7709556776892));
#23072=CARTESIAN_POINT('Ctrl Pts',(-7.64974417706006,3.38785496849908,-41.662161081781));
#23073=CARTESIAN_POINT('Ctrl Pts',(-8.10048921887679,1.02728432503435,-41.5926246877618));
#23074=CARTESIAN_POINT('Ctrl Pts',(-8.10151037503517,-0.000198521445028341,
-41.5623464956316));
#23075=CARTESIAN_POINT('Ctrl Pts',(-8.10186514679612,-0.000159416706436502,
-43.1876535043684));
#23076=CARTESIAN_POINT('Ctrl Pts',(-8.10203123770816,-0.185785457421342,
-43.1821827254615));
#23077=CARTESIAN_POINT('Ctrl Pts',(-8.05090917221341,-1.70336898962407,
-43.1374537446656));
#23078=CARTESIAN_POINT('Ctrl Pts',(-7.1394011161468,-4.49676768665247,-43.0534665619807));
#23079=CARTESIAN_POINT('Ctrl Pts',(-4.15858587830098,-7.34153467728348,
-42.9356919563136));
#23080=CARTESIAN_POINT('Ctrl Pts',(-0.186025343832157,-8.43548235114104,
-42.8179173506464));
#23081=CARTESIAN_POINT('Ctrl Pts',(3.83089877123767,-7.51772455796898,-42.7001427449793));
#23082=CARTESIAN_POINT('Ctrl Pts',(6.93422486298953,-4.80712944224074,-42.5823681393122));
#23083=CARTESIAN_POINT('Ctrl Pts',(8.38386744432517,-0.950123466158245,
-42.464593533645));
#23084=CARTESIAN_POINT('Ctrl Pts',(7.83411375280636,3.13346926473683,-42.3468189279779));
#23085=CARTESIAN_POINT('Ctrl Pts',(5.41606980711838,6.46978792306059,-42.2290443223107));
#23086=CARTESIAN_POINT('Ctrl Pts',(1.70639406288594,8.2631826330481,-42.1112697166436));
#23087=CARTESIAN_POINT('Ctrl Pts',(-2.4102248912686,8.08596215044749,-41.9934951109765));
#23088=CARTESIAN_POINT('Ctrl Pts',(-5.95205008868199,5.98039026040782,-41.8757205053094));
#23089=CARTESIAN_POINT('Ctrl Pts',(-7.78920245753314,2.92323328116088,-41.7737733031067));
#23090=CARTESIAN_POINT('Ctrl Pts',(-8.10055223102823,0.795170448066936,
-41.711084302793));
#23091=CARTESIAN_POINT('Ctrl Pts',(-8.10093877791723,-0.000108962703712148,
-41.6876535043684));
#23092=CARTESIAN_POINT('Origin',(0.,0.,-51.3123464956316));
#23093=CARTESIAN_POINT('',(-8.10191814333788,0.000147149967349575,-44.6876535043684));
#23094=CARTESIAN_POINT('',(-8.1012379593904,0.000186305278623682,-44.5623464956316));
#23095=CARTESIAN_POINT('',(-8.1015,-2.19835914433334E-13,-51.3123464956316));
#23096=CARTESIAN_POINT('Ctrl Pts',(-8.1012379593904,0.000186305278623185,
-44.5623464956316));
#23097=CARTESIAN_POINT('Ctrl Pts',(-8.10041846603269,-0.93395673238637,
-44.5348215330988));
#23098=CARTESIAN_POINT('Ctrl Pts',(-7.70856096931196,-3.20111578570497,
-44.4680383686769));
#23099=CARTESIAN_POINT('Ctrl Pts',(-5.63662629801377,-6.27856771542826,
-44.3619970023661));
#23100=CARTESIAN_POINT('Ctrl Pts',(-1.99120628747333,-8.19921130971783,
-44.2442223966989));
#23101=CARTESIAN_POINT('Ctrl Pts',(2.12907934517964,-8.16449568084935,-44.1264477910318));
#23102=CARTESIAN_POINT('Ctrl Pts',(5.74161919873576,-6.18269985988217,-44.0086731853647));
#23103=CARTESIAN_POINT('Ctrl Pts',(7.98488978577069,-2.72644524789567,-43.8908985796975));
#23104=CARTESIAN_POINT('Ctrl Pts',(8.32391284231425,1.38001578767571,-43.7731239740304));
#23105=CARTESIAN_POINT('Ctrl Pts',(6.67783768219246,5.1573687546043,-43.6553493683633));
#23106=CARTESIAN_POINT('Ctrl Pts',(3.43922258019218,7.70478530684499,-43.5375747626961));
#23107=CARTESIAN_POINT('Ctrl Pts',(-0.619583066806221,8.41475403110543,
-43.4198001570291));
#23108=CARTESIAN_POINT('Ctrl Pts',(-4.53062968937796,7.11796060669102,-43.3020255513619));
#23109=CARTESIAN_POINT('Ctrl Pts',(-7.36120549406269,4.12366611825681,-43.1842509456948));
#23110=CARTESIAN_POINT('Ctrl Pts',(-8.0904816961954,1.42536436889202,-43.104357927118));
#23111=CARTESIAN_POINT('Ctrl Pts',(-8.10215876212711,0.0467514429017632,
-43.0637231104303));
#23112=CARTESIAN_POINT('Ctrl Pts',(-8.10214365571365,4.69283692696408E-5,
-43.0623464956316));
#23113=CARTESIAN_POINT('Ctrl Pts',(-8.10191814333787,0.00014714996734987,
-44.6876535043684));
#23114=CARTESIAN_POINT('Ctrl Pts',(-8.10093166009298,-1.16610059920954,
-44.6532811481301));
#23115=CARTESIAN_POINT('Ctrl Pts',(-7.55530879276033,-3.66526533641054,
-44.5796505900026));
#23116=CARTESIAN_POINT('Ctrl Pts',(-5.0761873899821,-6.73975440997329,-44.4667618299862));
#23117=CARTESIAN_POINT('Ctrl Pts',(-1.27919300023199,-8.3400019899946,-44.3489872243191));
#23118=CARTESIAN_POINT('Ctrl Pts',(2.82286510073567,-7.95131439121922,-44.2312126186519));
#23119=CARTESIAN_POINT('Ctrl Pts',(6.25172243861154,-5.66638636835865,-44.1134380129848));
#23120=CARTESIAN_POINT('Ctrl Pts',(8.18966038568263,-2.03013070814185,-43.9956634073177));
#23121=CARTESIAN_POINT('Ctrl Pts',(8.17451682713419,2.09027332372109,-43.8778888016505));
#23122=CARTESIAN_POINT('Ctrl Pts',(6.20990321969786,5.71218609001371,-43.7601141959834));
#23123=CARTESIAN_POINT('Ctrl Pts',(2.76434332646893,7.97184883815334,-43.6423395903163));
#23124=CARTESIAN_POINT('Ctrl Pts',(-1.34046097639977,8.33037407897806,-43.5245649846492));
#23125=CARTESIAN_POINT('Ctrl Pts',(-5.12559029658075,6.70226021850519,-43.406790378982));
#23126=CARTESIAN_POINT('Ctrl Pts',(-7.569317806737,3.62565607228497,-43.2944865522218));
#23127=CARTESIAN_POINT('Ctrl Pts',(-8.10083937258845,1.1462633616389,-43.2214409273506));
#23128=CARTESIAN_POINT('Ctrl Pts',(-8.10186514679612,-0.000159416706436502,
-43.1876535043684));
#23129=CARTESIAN_POINT('Origin',(0.,0.,-51.3123464956316));
#23130=CARTESIAN_POINT('',(-8.10097060232049,0.000123429424611077,-46.1876535043684));
#23131=CARTESIAN_POINT('',(-8.10088198729152,-7.28186706448135E-5,-46.0623464956316));
#23132=CARTESIAN_POINT('',(-8.1015,-2.19835914433334E-13,-51.3123464956316));
#23133=CARTESIAN_POINT('Ctrl Pts',(-8.10088198729152,-7.28186706448752E-5,
-46.0623464956316));
#23134=CARTESIAN_POINT('Ctrl Pts',(-8.10106954261305,-0.582805848585725,
-46.0451781576563));
#23135=CARTESIAN_POINT('Ctrl Pts',(-7.8971652255018,-2.4979235666786,-45.988751617792));
#23136=CARTESIAN_POINT('Ctrl Pts',(-6.40377828321054,-5.49395961752304,
-45.8930668760387));
#23137=CARTESIAN_POINT('Ctrl Pts',(-3.03844483519571,-7.87145612736966,
-45.7752922703716));
#23138=CARTESIAN_POINT('Ctrl Pts',(1.05150112831493,-8.37175692177514,-45.6575176647045));
#23139=CARTESIAN_POINT('Ctrl Pts',(4.89068365232167,-6.87554957758499,-45.5397430590373));
#23140=CARTESIAN_POINT('Ctrl Pts',(7.56352919268905,-3.73965168591192,-45.4219684533702));
#23141=CARTESIAN_POINT('Ctrl Pts',(8.43261385803414,0.288083498271241,-45.3041938477031));
#23142=CARTESIAN_POINT('Ctrl Pts',(7.29067713854007,4.2471161324196,-45.1864192420359));
#23143=CARTESIAN_POINT('Ctrl Pts',(4.41004967826638,7.19329065281592,-45.0686446363688));
#23144=CARTESIAN_POINT('Ctrl Pts',(0.477707487483417,8.42399929588601,-44.9508700307017));
#23145=CARTESIAN_POINT('Ctrl Pts',(-3.56855904386543,7.64574096678149,-44.8330954250346));
#23146=CARTESIAN_POINT('Ctrl Pts',(-6.76379069195239,5.04411578536195,-44.7153208193674));
#23147=CARTESIAN_POINT('Ctrl Pts',(-7.97621164796412,2.12872042471518,-44.6250711762331));
#23148=CARTESIAN_POINT('Ctrl Pts',(-8.10158728999186,0.398389348818652,
-44.5740797349878));
#23149=CARTESIAN_POINT('Ctrl Pts',(-8.1012379593904,0.000186305278623185,
-44.5623464956316));
#23150=CARTESIAN_POINT('Ctrl Pts',(-8.10097060232049,0.000123429424611493,
-46.1876535043684));
#23151=CARTESIAN_POINT('Ctrl Pts',(-8.10051945174223,-0.815000391918625,
-46.1636377726876));
#23152=CARTESIAN_POINT('Ctrl Pts',(-7.77817455032938,-2.96294542208346,
-46.1003638391178));
#23153=CARTESIAN_POINT('Ctrl Pts',(-5.90793090228909,-6.02397877694788,
-45.9978317036589));
#23154=CARTESIAN_POINT('Ctrl Pts',(-2.35072454748789,-8.10345988234339,
-45.8800570979917));
#23155=CARTESIAN_POINT('Ctrl Pts',(1.76708584413041,-8.25041668822644,-45.7622824923246));
#23156=CARTESIAN_POINT('Ctrl Pts',(5.46347916408095,-6.42980274600106,-45.6445078866575));
#23157=CARTESIAN_POINT('Ctrl Pts',(7.85693443764436,-3.07580057347912,-45.5267332809903));
#23158=CARTESIAN_POINT('Ctrl Pts',(8.37665714814605,1.01172276152054,-45.4089586753233));
#23159=CARTESIAN_POINT('Ctrl Pts',(6.89870310741494,4.85796905729832,-45.291184069656));
#23160=CARTESIAN_POINT('Ctrl Pts',(3.77553683341622,7.54568019093911,-45.173409463989));
#23161=CARTESIAN_POINT('Ctrl Pts',(-0.248024672543488,8.4338871042367,-45.0556348583218));
#23162=CARTESIAN_POINT('Ctrl Pts',(-4.21243691249803,7.31076898712496,-44.9378602526548));
#23163=CARTESIAN_POINT('Ctrl Pts',(-7.17226138689772,4.44416859749758,-44.8200856469875));
#23164=CARTESIAN_POINT('Ctrl Pts',(-8.05700708526735,1.66364630693569,-44.7366833975588));
#23165=CARTESIAN_POINT('Ctrl Pts',(-8.10205836662772,0.165922997669041,
-44.6925393500191));
#23166=CARTESIAN_POINT('Ctrl Pts',(-8.10191814333787,0.00014714996734987,
-44.6876535043684));
#23167=CARTESIAN_POINT('Origin',(0.,0.,-51.3123464956316));
#23168=CARTESIAN_POINT('',(-8.1010842906964,-0.000174961242810356,-47.6876535043684));
#23169=CARTESIAN_POINT('',(-8.10173447928736,-0.000181404600999652,-47.5623464956316));
#23170=CARTESIAN_POINT('',(-8.1015,-2.19835914433334E-13,-51.3123464956316));
#23171=CARTESIAN_POINT('',(-2.10185380438479,7.8240982122538,-48.));
#23172=CARTESIAN_POINT('Ctrl Pts',(-2.10185380438476,7.82409821225381,-48.));
#23173=CARTESIAN_POINT('Ctrl Pts',(-3.38848271769056,7.47846018434309,-47.960741798111));
#23174=CARTESIAN_POINT('Ctrl Pts',(-5.7867414247356,6.14069431107141,-47.8822253943329));
#23175=CARTESIAN_POINT('Ctrl Pts',(-7.74755312548167,3.07031331488377,-47.778109895789));
#23176=CARTESIAN_POINT('Ctrl Pts',(-8.10047270114376,0.868629507982853,
-47.7132525991342));
#23177=CARTESIAN_POINT('Ctrl Pts',(-8.1010842906964,-0.000174961242810426,
-47.6876535043684));
#23178=CARTESIAN_POINT('',(2.10210202563587,7.82452631996418,-48.));
#23179=CARTESIAN_POINT('Origin',(0.,0.,-48.));
#23180=CARTESIAN_POINT('Ctrl Pts',(2.10210202563587,7.82452631996418,-48.));
#23181=CARTESIAN_POINT('Ctrl Pts',(0.957565047422177,8.13102709012696,-47.9650783907933));
#23182=CARTESIAN_POINT('Ctrl Pts',(-1.61897608126858,8.24429472572672,-47.8908985796976));
#23183=CARTESIAN_POINT('Ctrl Pts',(-5.23779660691551,6.61495420237904,-47.7774605667127));
#23184=CARTESIAN_POINT('Ctrl Pts',(-7.6007788734818,3.5348165809474,-47.6664976744634));
#23185=CARTESIAN_POINT('Ctrl Pts',(-8.10066624715266,1.10079321078201,-47.5947929841029));
#23186=CARTESIAN_POINT('Ctrl Pts',(-8.10173447928736,-0.000181404600998816,
-47.5623464956316));
#23187=CARTESIAN_POINT('Origin',(0.,0.,-51.3123464956316));
#23188=CARTESIAN_POINT('Ctrl Pts',(-8.10173447928736,-0.000181404600998816,
-47.5623464956316));
#23189=CARTESIAN_POINT('Ctrl Pts',(-8.10195874057133,-0.231316541667576,
-47.5555347822139));
#23190=CARTESIAN_POINT('Ctrl Pts',(-8.03636740777228,-1.79443477535343,
-47.5094648669071));
#23191=CARTESIAN_POINT('Ctrl Pts',(-7.06261736652514,-4.61642869377352,
-47.4241367497114));
#23192=CARTESIAN_POINT('Ctrl Pts',(-4.03429160538818,-7.41056347354498,
-47.3063621440442));
#23193=CARTESIAN_POINT('Ctrl Pts',(-0.04386199881008,-8.4374196345273,-47.1885875383771));
#23194=CARTESIAN_POINT('Ctrl Pts',(3.95702767181747,-7.45210695417129,-47.07081293271));
#23195=CARTESIAN_POINT('Ctrl Pts',(7.0142400262719,-4.68960620126019,-46.9530383270429));
#23196=CARTESIAN_POINT('Ctrl Pts',(8.39868669392937,-0.808721361269664,
-46.8352637213757));
#23197=CARTESIAN_POINT('Ctrl Pts',(7.78020299818498,3.26502830145453,-46.7174891157086));
#23198=CARTESIAN_POINT('Ctrl Pts',(5.30628574732215,6.56012959129681,-46.5997145100415));
#23199=CARTESIAN_POINT('Ctrl Pts',(1.56691815787412,8.290762087659,-46.4819399043743));
#23200=CARTESIAN_POINT('Ctrl Pts',(-2.54613023819965,8.04420222448489,-46.3641652987072));
#23201=CARTESIAN_POINT('Ctrl Pts',(-6.05197398148885,5.87924990905731,-46.2463906930401));
#23202=CARTESIAN_POINT('Ctrl Pts',(-7.81386931352349,2.83218407214127,-46.1457844253482));
#23203=CARTESIAN_POINT('Ctrl Pts',(-8.10064066681339,0.749708164640068,
-46.0844363595454));
#23204=CARTESIAN_POINT('Ctrl Pts',(-8.10088198729152,-7.28186706448752E-5,
-46.0623464956316));
#23205=CARTESIAN_POINT('Ctrl Pts',(-8.1010842906964,-0.000174961242810426,
-47.6876535043684));
#23206=CARTESIAN_POINT('Ctrl Pts',(-8.10141062126752,-0.463749686165932,
-47.6739943972452));
#23207=CARTESIAN_POINT('Ctrl Pts',(-7.94970659616376,-2.25948586872497,
-47.6210770882329));
#23208=CARTESIAN_POINT('Ctrl Pts',(-6.63976806498755,-5.20635630979624,
-47.5289015773315));
#23209=CARTESIAN_POINT('Ctrl Pts',(-3.38248655907778,-7.72983620180326,
-47.4111269716644));
#23210=CARTESIAN_POINT('Ctrl Pts',(0.681413555862794,-8.40998264592954,
-47.2933523659973));
#23211=CARTESIAN_POINT('Ctrl Pts',(4.58282963250162,-7.08446123670512,-47.1755777603301));
#23212=CARTESIAN_POINT('Ctrl Pts',(7.39131613068618,-4.06944919929777,-47.057803154663));
#23213=CARTESIAN_POINT('Ctrl Pts',(8.43711630815339,-0.0839387386951516,
-46.9400285489959));
#23214=CARTESIAN_POINT('Ctrl Pts',(7.47081891547249,3.92158434705153,-46.8222539433287));
#23215=CARTESIAN_POINT('Ctrl Pts',(4.72287152121607,6.99188514875576,-46.7044793376616));
#23216=CARTESIAN_POINT('Ctrl Pts',(0.848606621735488,8.39475027502305,-46.5867047319945));
#23217=CARTESIAN_POINT('Ctrl Pts',(-3.22803486495866,7.79562439652349,-46.4689301263274));
#23218=CARTESIAN_POINT('Ctrl Pts',(-6.53485028731455,5.33738695312811,-46.3511555206602));
#23219=CARTESIAN_POINT('Ctrl Pts',(-7.92670970382778,2.36710169478299,-46.2573966466739));
#23220=CARTESIAN_POINT('Ctrl Pts',(-8.10125694168087,0.517471837874847,
-46.2028959745766));
#23221=CARTESIAN_POINT('Ctrl Pts',(-8.10097060232049,0.000123429424611493,
-46.1876535043684));
#23222=CARTESIAN_POINT('Ctrl Pts',(5.46288453460432,-4.78623668048091,-48.));
#23223=CARTESIAN_POINT('Ctrl Pts',(6.2499542175215,-3.88789606644505,-47.960741798111));
#23224=CARTESIAN_POINT('Ctrl Pts',(7.37171595554078,-1.69639746569614,-47.8822253943329));
#23225=CARTESIAN_POINT('Ctrl Pts',(7.29581740547595,1.99731954537833,-47.7644507886657));
#23226=CARTESIAN_POINT('Ctrl Pts',(5.4801165872417,5.21397460516973,-47.6466761829987));
#23227=CARTESIAN_POINT('Ctrl Pts',(2.3574553976849,7.18755200305922,-47.5289015773315));
#23228=CARTESIAN_POINT('Ctrl Pts',(-1.32738855178181,7.4468564743695,-47.4111269716644));
#23229=CARTESIAN_POINT('Ctrl Pts',(-4.69568805233936,5.9303107291093,-47.2933523659972));
#23230=CARTESIAN_POINT('Ctrl Pts',(-6.94414699118569,2.99945379218927,-47.1755777603301));
#23231=CARTESIAN_POINT('Ctrl Pts',(-7.53655932503615,-0.646696104264617,
-47.057803154663));
#23232=CARTESIAN_POINT('Ctrl Pts',(-6.3316410458646,-4.13863131554368,-46.9400285489958));
#23233=CARTESIAN_POINT('Ctrl Pts',(-3.61674503856499,-6.64357495628676,
-46.8222539433288));
#23234=CARTESIAN_POINT('Ctrl Pts',(-0.0393223103570487,-7.5641521700391,
-46.7044793376616));
#23235=CARTESIAN_POINT('Ctrl Pts',(3.54747787204966,-6.68081871358959,-46.5867047319945));
#23236=CARTESIAN_POINT('Ctrl Pts',(6.2882707289777,-4.20423499842656,-46.4689301263273));
#23237=CARTESIAN_POINT('Ctrl Pts',(7.52942806369302,-0.725019224452457,
-46.3511555206603));
#23238=CARTESIAN_POINT('Ctrl Pts',(6.97495702966333,2.92709998808421,-46.233380914993));
#23239=CARTESIAN_POINT('Ctrl Pts',(4.7570886110968,5.88116042974619,-46.115606309326));
#23240=CARTESIAN_POINT('Ctrl Pts',(1.40474314394121,7.43267358423345,-45.9978317036588));
#23241=CARTESIAN_POINT('Ctrl Pts',(-2.28260740851004,7.21163250712014,-45.8800570979917));
#23242=CARTESIAN_POINT('Ctrl Pts',(-5.42559859625422,5.27075135338927,-45.7622824923246));
#23243=CARTESIAN_POINT('Ctrl Pts',(-7.27468554731165,2.07289415063032,-45.6445078866575));
#23244=CARTESIAN_POINT('Ctrl Pts',(-7.38889545401083,-1.61930971060316,
-45.5267332809903));
#23245=CARTESIAN_POINT('Ctrl Pts',(-5.7409913807268,-4.92533835734985,-45.4089586753232));
#23246=CARTESIAN_POINT('Ctrl Pts',(-2.72396776375072,-7.056765519112,-45.2911840696561));
#23247=CARTESIAN_POINT('Ctrl Pts',(0.942671442936654,-7.50528550550551,
-45.173409463989));
#23248=CARTESIAN_POINT('Ctrl Pts',(4.38450106360703,-6.16393465185457,-45.0556348583218));
#23249=CARTESIAN_POINT('Ctrl Pts',(6.7807088226255,-3.35260015981957,-44.9378602526547));
#23250=CARTESIAN_POINT('Ctrl Pts',(7.55984378829871,0.258267042886377,-44.8200856469876));
#23251=CARTESIAN_POINT('Ctrl Pts',(6.53609677926514,3.80754236496496,-44.7023110413205));
#23252=CARTESIAN_POINT('Ctrl Pts',(3.95361239440211,6.44878973170425,-44.5845364356533));
#23253=CARTESIAN_POINT('Ctrl Pts',(0.42826507209678,7.55212082775043,-44.4667618299862));
#23254=CARTESIAN_POINT('Ctrl Pts',(-3.19921549535205,6.85441173137493,-44.3489872243191));
#23255=CARTESIAN_POINT('Ctrl Pts',(-6.06374273846204,4.52205307030598,-44.2312126186519));
#23256=CARTESIAN_POINT('Ctrl Pts',(-7.4821802489587,1.11126895529654,-44.1134380129848));
#23257=CARTESIAN_POINT('Ctrl Pts',(-7.11625709274196,-2.56453211305952,
-43.9956634073177));
#23258=CARTESIAN_POINT('Ctrl Pts',(-5.05323912886181,-5.62874002557001,
-43.8778888016506));
#23259=CARTESIAN_POINT('Ctrl Pts',(-1.78511772707755,-7.35059825248172,
-43.7601141959834));
#23260=CARTESIAN_POINT('Ctrl Pts',(1.90872101265689,-7.31947566870441,-43.6423395903163));
#23261=CARTESIAN_POINT('Ctrl Pts',(5.14736533239743,-5.54279443094788,-43.5245649846491));
#23262=CARTESIAN_POINT('Ctrl Pts',(7.15845886737674,-2.44425993155172,-43.406790378982));
#23263=CARTESIAN_POINT('Ctrl Pts',(7.46239325726449,1.23718504794034,-43.2890157733149));
#23264=CARTESIAN_POINT('Ctrl Pts',(5.98668580951229,4.62358443062285,-43.1712411676478));
#23265=CARTESIAN_POINT('Ctrl Pts',(3.08326527185531,6.90734502050424,-43.0534665619806));
#23266=CARTESIAN_POINT('Ctrl Pts',(-0.55545662089904,7.54383244188345,-42.9356919563136));
#23267=CARTESIAN_POINT('Ctrl Pts',(-4.06171245250289,6.38125629653729,-42.8179173506464));
#23268=CARTESIAN_POINT('Ctrl Pts',(-6.59932549569553,3.69686934726893,-42.7001427449793));
#23269=CARTESIAN_POINT('Ctrl Pts',(-7.56312229154544,0.130847896591264,
-42.5823681393121));
#23270=CARTESIAN_POINT('Ctrl Pts',(-6.7232552507141,-3.46637834095748,-42.4645935336451));
#23271=CARTESIAN_POINT('Ctrl Pts',(-4.2800170236141,-6.23693789022203,-42.3468189279779));
#23272=CARTESIAN_POINT('Ctrl Pts',(-0.816074432854366,-7.5201038881757,
-42.2290443223108));
#23273=CARTESIAN_POINT('Ctrl Pts',(2.84248671434799,-7.00986513762347,-42.1112697166436));
#23274=CARTESIAN_POINT('Ctrl Pts',(5.82316770897799,-4.82790407962191,-41.9934951109766));
#23275=CARTESIAN_POINT('Ctrl Pts',(7.415131635876,-1.49457779708679,-41.8757205053093));
#23276=CARTESIAN_POINT('Ctrl Pts',(7.23872474179556,2.19517746012267,-41.7579458996423));
#23277=CARTESIAN_POINT('Ctrl Pts',(5.33601678617319,5.36142376860771,-41.6401712939751));
#23278=CARTESIAN_POINT('Ctrl Pts',(2.16076818686676,7.24907034119122,-41.522396688308));
#23279=CARTESIAN_POINT('Ctrl Pts',(-1.52978339021372,7.4079486194182,-41.4046220826408));
#23280=CARTESIAN_POINT('Ctrl Pts',(-4.8555101142083,5.80016909233988,-41.2868474769738));
#23281=CARTESIAN_POINT('Ctrl Pts',(-7.0232880884613,2.80915723934978,-41.1690728713066));
#23282=CARTESIAN_POINT('Ctrl Pts',(-7.51614263143352,-0.85178630704034,
-41.0512982656395));
#23283=CARTESIAN_POINT('Ctrl Pts',(-6.21653711187188,-4.30959467997091,
-40.9335236599724));
#23284=CARTESIAN_POINT('Ctrl Pts',(-3.43440324676116,-6.73964496895424,
-40.8157490543052));
#23285=CARTESIAN_POINT('Ctrl Pts',(0.166771842063232,-7.56241542905497,
-40.6979744486381));
#23286=CARTESIAN_POINT('Ctrl Pts',(3.72817495194683,-6.58169062601625,-40.580199842971));
#23287=CARTESIAN_POINT('Ctrl Pts',(6.40047775663446,-4.03135516368146,-40.4624252373039));
#23288=CARTESIAN_POINT('Ctrl Pts',(7.5463857970818,-0.5196165610486,-40.3446506316367));
#23289=CARTESIAN_POINT('Ctrl Pts',(6.89262134313397,3.11604091582377,-40.2268760259696));
#23290=CARTESIAN_POINT('Ctrl Pts',(4.5950950435731,6.00858065681437,-40.1091014203025));
#23291=CARTESIAN_POINT('Ctrl Pts',(1.20172413953307,7.46818579451377,-39.9913268146353));
#23292=CARTESIAN_POINT('Ctrl Pts',(-2.47823559496468,7.14676768229974,-39.8735522089682));
#23293=CARTESIAN_POINT('Ctrl Pts',(-5.56718228628964,5.12097855493816,-39.7557776033011));
#23294=CARTESIAN_POINT('Ctrl Pts',(-7.32845966659239,1.87393139790187,-39.638002997634));
#23295=CARTESIAN_POINT('Ctrl Pts',(-7.34203587670703,-1.82001350381267,
-39.5202283919668));
#23296=CARTESIAN_POINT('Ctrl Pts',(-5.60467324331843,-5.07991907460583,
-39.4024537862997));
#23297=CARTESIAN_POINT('Ctrl Pts',(-2.53070040376012,-7.12835853723164,
-39.2846791806325));
#23298=CARTESIAN_POINT('Ctrl Pts',(1.14679735894242,-7.47681722301901,-39.1669045749655));
#23299=CARTESIAN_POINT('Ctrl Pts',(4.55080530558902,-6.04219422391756,-39.0491299692983));
#23300=CARTESIAN_POINT('Ctrl Pts',(6.86953092556355,-3.16662041167394,-38.9313553636312));
#23301=CARTESIAN_POINT('Ctrl Pts',(7.55000133455977,0.464133404388116,-38.8135807579641));
#23302=CARTESIAN_POINT('Ctrl Pts',(6.42993701079272,3.98420004595123,-38.695806152297));
#23303=CARTESIAN_POINT('Ctrl Pts',(3.77645243922374,6.55410916472519,-38.5780315466298));
#23304=CARTESIAN_POINT('Ctrl Pts',(0.222354280686254,7.5609852891647,-38.4602569409627));
#23305=CARTESIAN_POINT('Ctrl Pts',(-3.38477123339968,6.76470721214373,-38.3424823352955));
#23306=CARTESIAN_POINT('Ctrl Pts',(-6.1846918348333,4.3551724280248,-38.2247077296285));
#23307=CARTESIAN_POINT('Ctrl Pts',(-7.50967859620706,0.907010115506259,
-38.1069331239613));
#23308=CARTESIAN_POINT('Ctrl Pts',(-7.04374684730056,-2.75745722003065,
-37.9891585182942));
#23309=CARTESIAN_POINT('Ctrl Pts',(-4.89801263364484,-5.76432235502473,
-37.871383912627));
#23310=CARTESIAN_POINT('Ctrl Pts',(-1.58419361167746,-7.39650394156935,
-37.7536093069599));
#23311=CARTESIAN_POINT('Ctrl Pts',(2.10742608985921,-7.26475706922933,-37.6358347012928));
#23312=CARTESIAN_POINT('Ctrl Pts',(5.29646390680803,-5.40050090214708,-37.5180600956257));
#23313=CARTESIAN_POINT('Ctrl Pts',(7.22239371279843,-2.24832584639531,-37.4002854899585));
#23314=CARTESIAN_POINT('Ctrl Pts',(7.42591708833791,1.44003309094744,-37.2825108842915));
#23315=CARTESIAN_POINT('Ctrl Pts',(5.85849754427007,4.78497088454414,-37.1647362786242));
#23316=CARTESIAN_POINT('Ctrl Pts',(2.8939353617182,6.98878235496782,-37.0469616729572));
#23317=CARTESIAN_POINT('Ctrl Pts',(-0.760776389984131,7.52589909718257,
-36.92918706729));
#23318=CARTESIAN_POINT('Ctrl Pts',(-4.23405739852132,6.26822959388264,-36.8114124616229));
#23319=CARTESIAN_POINT('Ctrl Pts',(-6.69759403037466,3.51570292801806,-36.6936378559558));
#23320=CARTESIAN_POINT('Ctrl Pts',(-7.56388027176127,-0.0752511404343053,
-36.5758632502887));
#23321=CARTESIAN_POINT('Ctrl Pts',(-6.62631973269411,-3.64826384889705,
-36.4580886446215));
#23322=CARTESIAN_POINT('Ctrl Pts',(-4.10850975262302,-6.35122414179136,
-36.3403140389544));
#23323=CARTESIAN_POINT('Ctrl Pts',(-0.610887698769837,-7.53955488395458,
-36.2225394332872));
#23324=CARTESIAN_POINT('Ctrl Pts',(3.03240140566261,-6.92980327514396,-36.1047648276202));
#23325=CARTESIAN_POINT('Ctrl Pts',(5.95255640869504,-4.66750168184842,-35.986990221953));
#23326=CARTESIAN_POINT('Ctrl Pts',(7.45306200829349,-1.2919271239697,-35.8692156162859));
#23327=CARTESIAN_POINT('Ctrl Pts',(7.17630464094038,2.39141980438688,-35.7514410106187));
#23328=CARTESIAN_POINT('Ctrl Pts',(5.18781717002348,5.50513519372634,-35.6336664049517));
#23329=CARTESIAN_POINT('Ctrl Pts',(3.03777695224176,6.70444440151624,-35.5551500011735));
#23330=CARTESIAN_POINT('Ctrl Pts',(1.88431329769136,7.01430911752138,-35.5158917992845));
#23331=CARTESIAN_POINT('Ctrl Pts',(5.67311119403182,-4.9704240895673,-48.1613694002385));
#23332=CARTESIAN_POINT('Ctrl Pts',(6.49046945968001,-4.03751288464296,-48.1221111983495));
#23333=CARTESIAN_POINT('Ctrl Pts',(7.65539964128684,-1.76167945546099,-48.0435947945714));
#23334=CARTESIAN_POINT('Ctrl Pts',(7.57658030852297,2.07418183546964,-47.9258201889043));
#23335=CARTESIAN_POINT('Ctrl Pts',(5.69100638293687,5.41462253331856,-47.8080455832371));
#23336=CARTESIAN_POINT('Ctrl Pts',(2.44817669517256,7.46414855887019,-47.69027097757));
#23337=CARTESIAN_POINT('Ctrl Pts',(-1.37847007459924,7.73343177171031,-47.5724963719029));
#23338=CARTESIAN_POINT('Ctrl Pts',(-4.87639090386474,6.15852522019922,-47.4547217662358));
#23339=CARTESIAN_POINT('Ctrl Pts',(-7.21137665992263,3.11488093454325,-47.3369471605686));
#23340=CARTESIAN_POINT('Ctrl Pts',(-7.82658663211968,-0.671582729783266,
-47.2191725549015));
#23341=CARTESIAN_POINT('Ctrl Pts',(-6.57529981941811,-4.29789710828696,
-47.1013979492344));
#23342=CARTESIAN_POINT('Ctrl Pts',(-3.75592722750606,-6.89923779537283,
-46.9836233435672));
#23343=CARTESIAN_POINT('Ctrl Pts',(-0.0408355398413912,-7.85524132486851,
-46.8658487379001));
#23344=CARTESIAN_POINT('Ctrl Pts',(3.68399447197226,-6.93791479378349,-46.748074132233));
#23345=CARTESIAN_POINT('Ctrl Pts',(6.53026049474244,-4.36602539937111,-46.6302995265658));
#23346=CARTESIAN_POINT('Ctrl Pts',(7.81918094043847,-0.75291993672486,-46.5125249208988));
#23347=CARTESIAN_POINT('Ctrl Pts',(7.24337235250388,3.03974275920765,-46.3947503152315));
#23348=CARTESIAN_POINT('Ctrl Pts',(4.94015432317192,6.10748348359639,-46.2769757095645));
#23349=CARTESIAN_POINT('Ctrl Pts',(1.45880148191885,7.7187030853753,-46.1592011038973));
#23350=CARTESIAN_POINT('Ctrl Pts',(-2.37044835173991,7.48915574624172,-46.0414264982303));
#23351=CARTESIAN_POINT('Ctrl Pts',(-5.63439039133243,5.47358420527862,-45.9236518925631));
#23352=CARTESIAN_POINT('Ctrl Pts',(-7.55463523896436,2.15266475714294,-45.805877286896));
#23353=CARTESIAN_POINT('Ctrl Pts',(-7.67324025359723,-1.68162515382409,
-45.6881026812288));
#23354=CARTESIAN_POINT('Ctrl Pts',(-5.96192034822138,-5.11487877740758,
-45.5703280755617));
#23355=CARTESIAN_POINT('Ctrl Pts',(-2.82879345423239,-7.32832905519788,
-45.4525534698945));
#23356=CARTESIAN_POINT('Ctrl Pts',(0.978948004729415,-7.79410931092872,
-45.3347788642275));
#23357=CARTESIAN_POINT('Ctrl Pts',(4.55322859317857,-6.40113962709804,-45.2170042585603));
#23358=CARTESIAN_POINT('Ctrl Pts',(7.04164894598002,-3.48161733518369,-45.0992296528932));
#23359=CARTESIAN_POINT('Ctrl Pts',(7.85076714487718,0.268205861347997,-44.9814550472261));
#23360=CARTESIAN_POINT('Ctrl Pts',(6.78762356569012,3.95406695411651,-44.863680441559));
#23361=CARTESIAN_POINT('Ctrl Pts',(4.10575815569019,6.69695670540814,-44.7459058358918));
#23362=CARTESIAN_POINT('Ctrl Pts',(0.444745877225661,7.84274698379562,-44.6281312302247));
#23363=CARTESIAN_POINT('Ctrl Pts',(-3.32233001152318,7.11818814317712,-44.5103566245576));
#23364=CARTESIAN_POINT('Ctrl Pts',(-6.29709205629216,4.69607397532464,-44.3925820188905));
#23365=CARTESIAN_POINT('Ctrl Pts',(-7.77011490124893,1.15403360805785,-44.2748074132233));
#23366=CARTESIAN_POINT('Ctrl Pts',(-7.39011002643621,-2.66322228593577,
-44.1570328075562));
#23367=CARTESIAN_POINT('Ctrl Pts',(-5.24770151857913,-5.84534925552276,
-44.0392582018891));
#23368=CARTESIAN_POINT('Ctrl Pts',(-1.85381391387615,-7.63346927156042,
-43.9214835962219));
#23369=CARTESIAN_POINT('Ctrl Pts',(1.98217379016447,-7.60114900608606,-43.8037089905548));
#23370=CARTESIAN_POINT('Ctrl Pts',(5.34544995451021,-5.75609624059265,-43.6859343848877));
#23371=CARTESIAN_POINT('Ctrl Pts',(7.43393584017472,-2.53832170366637,-43.5681597792206));
#23372=CARTESIAN_POINT('Ctrl Pts',(7.74956645228107,1.2847952945188,-43.4503851735534));
#23373=CARTESIAN_POINT('Ctrl Pts',(6.21706976707235,4.80151253861666,-43.3326105678863));
#23374=CARTESIAN_POINT('Ctrl Pts',(3.2019177079676,7.17315844928449,-43.2148359622191));
#23375=CARTESIAN_POINT('Ctrl Pts',(-0.576832102868098,7.83413963829078,
-43.0970613565521));
#23376=CARTESIAN_POINT('Ctrl Pts',(-4.21801819812791,6.62682439992187,-42.9792867508849));
#23377=CARTESIAN_POINT('Ctrl Pts',(-6.85328549515125,3.83913493759823,-42.8615121452178));
#23378=CARTESIAN_POINT('Ctrl Pts',(-7.85417181384847,0.135883279641968,
-42.7437375395506));
#23379=CARTESIAN_POINT('Ctrl Pts',(-6.98198440431105,-3.59977401028112,
-42.6259629338836));
#23380=CARTESIAN_POINT('Ctrl Pts',(-4.44472372306338,-6.47695222869333,
-42.5081883282163));
#23381=CARTESIAN_POINT('Ctrl Pts',(-0.847479197274412,-7.80949794527952,
-42.3904137225493));
#23382=CARTESIAN_POINT('Ctrl Pts',(2.95187333649589,-7.27962381943069,-42.2726391168821));
#23383=CARTESIAN_POINT('Ctrl Pts',(6.04725904515579,-5.01369496358918,-42.1548645112151));
#23384=CARTESIAN_POINT('Ctrl Pts',(7.70048607511974,-1.55209321692512,-42.0370899055479));
#23385=CARTESIAN_POINT('Ctrl Pts',(7.51729056381565,2.27965386107329,-41.9193152998808));
#23386=CARTESIAN_POINT('Ctrl Pts',(5.54136122947973,5.56774594172155,-41.8015406942136));
#23387=CARTESIAN_POINT('Ctrl Pts',(2.24392042536729,7.5280342900227,-41.6837660885465));
#23388=CARTESIAN_POINT('Ctrl Pts',(-1.58865361705728,7.69302663664625,-41.5659914828794));
#23389=CARTESIAN_POINT('Ctrl Pts',(-5.0423633534925,6.02337537917852,-41.4482168772123));
#23390=CARTESIAN_POINT('Ctrl Pts',(-7.29356332193576,2.91726125262229,-41.3304422715451));
#23391=CARTESIAN_POINT('Ctrl Pts',(-7.80538424860076,-0.884565361538173,
-41.212667665878));
#23392=CARTESIAN_POINT('Ctrl Pts',(-6.45576637288911,-4.47543960810693,
-41.0948930602109));
#23393=CARTESIAN_POINT('Ctrl Pts',(-3.56656842746744,-6.99900484349956,
-40.9771184545437));
#23394=CARTESIAN_POINT('Ctrl Pts',(0.173189676271779,-7.85343774936625,
-40.8593438488766));
#23395=CARTESIAN_POINT('Ctrl Pts',(3.87164526711537,-6.8349719877086,-40.7415692432095));
#23396=CARTESIAN_POINT('Ctrl Pts',(6.64678555409823,-4.18649267824142,-40.6237946375423));
#23397=CARTESIAN_POINT('Ctrl Pts',(7.83679125354391,-0.539612820006756,
-40.5060200318753));
#23398=CARTESIAN_POINT('Ctrl Pts',(7.1578681647512,3.23595464788666,-40.3882454262081));
#23399=CARTESIAN_POINT('Ctrl Pts',(4.77192680244391,6.23980718766658,-40.270470820541));
#23400=CARTESIAN_POINT('Ctrl Pts',(1.24796975387969,7.75558190212311,-40.1526962148738));
#23401=CARTESIAN_POINT('Ctrl Pts',(-2.57360484304297,7.42179474648848,-40.0349216092068));
#23402=CARTESIAN_POINT('Ctrl Pts',(-5.7814226069585,5.31804774206541,-39.9171470035396));
#23403=CARTESIAN_POINT('Ctrl Pts',(-7.61047873265497,1.9460453763837,-39.7993723978725));
#23404=CARTESIAN_POINT('Ctrl Pts',(-7.6245773922708,-1.89005257503884,-39.6815977922054));
#23405=CARTESIAN_POINT('Ctrl Pts',(-5.82035631801311,-5.27540818122188,
-39.5638231865382));
#23406=CARTESIAN_POINT('Ctrl Pts',(-2.62808864041866,-7.40267716743352,
-39.4460485808711));
#23407=CARTESIAN_POINT('Ctrl Pts',(1.19092924133598,-7.76454549148023,-39.328273975204));
#23408=CARTESIAN_POINT('Ctrl Pts',(4.72593267484581,-6.27471429628227,-39.2104993695368));
#23409=CARTESIAN_POINT('Ctrl Pts',(7.13388916509199,-3.28848058034568,-39.0927247638697));
#23410=CARTESIAN_POINT('Ctrl Pts',(7.84054592674062,0.481994520528341,-38.9749501582026));
#23411=CARTESIAN_POINT('Ctrl Pts',(6.67737848050448,4.13752290328889,-38.8571755525354));
#23412=CARTESIAN_POINT('Ctrl Pts',(3.9217806034483,6.80632911674786,-38.7394009468683));
#23413=CARTESIAN_POINT('Ctrl Pts',(0.230911078352757,7.85195257380211,-38.6216263412012));
#23414=CARTESIAN_POINT('Ctrl Pts',(-3.51502643920103,7.0250315499923,-38.5038517355341));
#23415=CARTESIAN_POINT('Ctrl Pts',(-6.4226956029506,4.52277131190652,-38.3860771298669));
#23416=CARTESIAN_POINT('Ctrl Pts',(-7.79867145971248,0.941914332397903,
-38.2683025241998));
#23417=CARTESIAN_POINT('Ctrl Pts',(-7.31480938947604,-2.86357167590268,
-38.1505279185327));
#23418=CARTESIAN_POINT('Ctrl Pts',(-5.08650148551097,-5.98614916188545,
-38.0327533128655));
#23419=CARTESIAN_POINT('Ctrl Pts',(-1.6451576918735,-7.68114153645695,-37.9149787071984));
#23420=CARTESIAN_POINT('Ctrl Pts',(2.1885255793423,-7.54432468603362,-37.7972041015313));
#23421=CARTESIAN_POINT('Ctrl Pts',(5.5002862477075,-5.60832686967428,-37.6794294958642));
#23422=CARTESIAN_POINT('Ctrl Pts',(7.50033107239187,-2.33484754184726,-37.5616548901971));
#23423=CARTESIAN_POINT('Ctrl Pts',(7.71168658113571,1.49544948209707,-37.4438802845299));
#23424=CARTESIAN_POINT('Ctrl Pts',(6.08394846862963,4.96910958235911,-37.3261056788628));
#23425=CARTESIAN_POINT('Ctrl Pts',(3.0053018677901,7.2577297139398,-37.2083310731957));
#23426=CARTESIAN_POINT('Ctrl Pts',(-0.790053135268523,7.81551616969566,
-37.0905564675285));
#23427=CARTESIAN_POINT('Ctrl Pts',(-4.39699544655749,6.50944812224422,-36.9727818618614));
#23428=CARTESIAN_POINT('Ctrl Pts',(-6.95533567039803,3.65099674164618,-36.8550072561943));
#23429=CARTESIAN_POINT('Ctrl Pts',(-7.8549589632052,-0.078147009049392,
-36.7372326505271));
#23430=CARTESIAN_POINT('Ctrl Pts',(-6.88131854383111,-3.78865896741099,
-36.61945804486));
#23431=CARTESIAN_POINT('Ctrl Pts',(-4.26661638567522,-6.59563652615466,
-36.5016834391929));
#23432=CARTESIAN_POINT('Ctrl Pts',(-0.634396319423309,-7.82969746829512,
-36.3839088335257));
#23433=CARTESIAN_POINT('Ctrl Pts',(3.14909646182159,-7.19648095866354,-36.2661342278587));
#23434=CARTESIAN_POINT('Ctrl Pts',(6.18162697405788,-4.84711984515238,-36.1483596221915));
#23435=CARTESIAN_POINT('Ctrl Pts',(7.73987611146271,-1.34164399456718,-36.0305850165244));
#23436=CARTESIAN_POINT('Ctrl Pts',(7.45246836765699,2.48344814464932,-35.9128104108572));
#23437=CARTESIAN_POINT('Ctrl Pts',(5.38745848890295,5.71698777346563,-35.7950358051902));
#23438=CARTESIAN_POINT('Ctrl Pts',(3.15467887405803,6.96244966245852,-35.716519401412));
#23439=CARTESIAN_POINT('Ctrl Pts',(1.9568267999225,7.28423881576552,-35.677261199523));
#23440=CARTESIAN_POINT('Ctrl Pts',(5.88333785345931,-5.15461149865368,-48.322738800477));
#23441=CARTESIAN_POINT('Ctrl Pts',(6.73098470183852,-4.18712970284087,-48.283480598588));
#23442=CARTESIAN_POINT('Ctrl Pts',(7.9390833270329,-1.82696144522583,-48.2049641948099));
#23443=CARTESIAN_POINT('Ctrl Pts',(7.85734321156999,2.15104412556096,-48.0871895891428));
#23444=CARTESIAN_POINT('Ctrl Pts',(5.90189617863205,5.61527046146739,-47.9694149834756));
#23445=CARTESIAN_POINT('Ctrl Pts',(2.53889799266023,7.74074511468116,-47.8516403778085));
#23446=CARTESIAN_POINT('Ctrl Pts',(-1.42955159741667,8.02000706905112,-47.7338657721414));
#23447=CARTESIAN_POINT('Ctrl Pts',(-5.05709375539013,6.38673971128913,-47.6160911664743));
#23448=CARTESIAN_POINT('Ctrl Pts',(-7.47860632865957,3.23030807689722,-47.4983165608071));
#23449=CARTESIAN_POINT('Ctrl Pts',(-8.11661393920319,-0.696469355301917,
-47.38054195514));
#23450=CARTESIAN_POINT('Ctrl Pts',(-6.81895859297162,-4.45716290103025,
-47.2627673494729));
#23451=CARTESIAN_POINT('Ctrl Pts',(-3.89510941644712,-7.1549006344589,-47.1449927438057));
#23452=CARTESIAN_POINT('Ctrl Pts',(-0.0423487693257355,-8.1463304796979,
-47.0272181381386));
#23453=CARTESIAN_POINT('Ctrl Pts',(3.82051107189486,-7.19501087397739,-46.9094435324715));
#23454=CARTESIAN_POINT('Ctrl Pts',(6.77225026050717,-4.52781580031565,-46.7916689268043));
#23455=CARTESIAN_POINT('Ctrl Pts',(8.10893381718392,-0.780820648997262,
-46.6738943211373));
#23456=CARTESIAN_POINT('Ctrl Pts',(7.51178767534443,3.15238553033109,-46.5561197154701));
#23457=CARTESIAN_POINT('Ctrl Pts',(5.12322003524703,6.3338065374466,-46.438345109803));
#23458=CARTESIAN_POINT('Ctrl Pts',(1.51285981989648,8.00473258651715,-46.3205705041358));
#23459=CARTESIAN_POINT('Ctrl Pts',(-2.45828929496978,7.76667898536331,-46.2027958984687));
#23460=CARTESIAN_POINT('Ctrl Pts',(-5.84318218641065,5.67641705716796,-46.0850212928016));
#23461=CARTESIAN_POINT('Ctrl Pts',(-7.83458493061706,2.23243536365556,-45.9672466871344));
#23462=CARTESIAN_POINT('Ctrl Pts',(-7.95758505318363,-1.74394059704502,
-45.8494720814674));
#23463=CARTESIAN_POINT('Ctrl Pts',(-6.18284931571595,-5.30441919746531,
-45.7316974758002));
#23464=CARTESIAN_POINT('Ctrl Pts',(-2.93361914471405,-7.59989259128377,
-45.6139228701331));
#23465=CARTESIAN_POINT('Ctrl Pts',(1.01522456652217,-8.08293311635193,-45.496148264466));
#23466=CARTESIAN_POINT('Ctrl Pts',(4.72195612275012,-6.63834460234152,-45.3783736587988));
#23467=CARTESIAN_POINT('Ctrl Pts',(7.30258906933454,-3.61063451054781,-45.2605990531317));
#23468=CARTESIAN_POINT('Ctrl Pts',(8.14169050145566,0.278144679809618,-45.1428244474646));
#23469=CARTESIAN_POINT('Ctrl Pts',(7.0391503521151,4.10059154326806,-45.0250498417974));
#23470=CARTESIAN_POINT('Ctrl Pts',(4.25790391697829,6.94512367911202,-44.9072752361303));
#23471=CARTESIAN_POINT('Ctrl Pts',(0.461226682354538,8.13337313984082,-44.7895006304633));
#23472=CARTESIAN_POINT('Ctrl Pts',(-3.4454445276943,7.3819645549793,-44.671726024796));
#23473=CARTESIAN_POINT('Ctrl Pts',(-6.53044137412228,4.8700948803433,-44.553951419129));
#23474=CARTESIAN_POINT('Ctrl Pts',(-8.05804955353917,1.19679826081915,-44.4361768134618));
#23475=CARTESIAN_POINT('Ctrl Pts',(-7.66396296013046,-2.761912458812,-44.3184022077947));
#23476=CARTESIAN_POINT('Ctrl Pts',(-5.44216390829645,-6.06195848547551,
-44.2006276021275));
#23477=CARTESIAN_POINT('Ctrl Pts',(-1.92251010067474,-7.91634029063913,
-44.0828529964604));
#23478=CARTESIAN_POINT('Ctrl Pts',(2.05562656767206,-7.8828223434677,-43.9650783907933));
#23479=CARTESIAN_POINT('Ctrl Pts',(5.54353457662299,-5.96939805023741,-43.8473037851262));
#23480=CARTESIAN_POINT('Ctrl Pts',(7.70941281297271,-2.63238347578102,-43.729529179459));
#23481=CARTESIAN_POINT('Ctrl Pts',(8.03673964729766,1.33240554109725,-43.611754573792));
#23482=CARTESIAN_POINT('Ctrl Pts',(6.4474537246324,4.97944064661048,-43.4939799681247));
#23483=CARTESIAN_POINT('Ctrl Pts',(3.32057014407989,7.43897187806474,-43.3762053624577));
#23484=CARTESIAN_POINT('Ctrl Pts',(-0.598207584837165,8.12444683469811,
-43.2584307567905));
#23485=CARTESIAN_POINT('Ctrl Pts',(-4.37432394375293,6.87239250330645,-43.1406561511235));
#23486=CARTESIAN_POINT('Ctrl Pts',(-7.10724549460698,3.98140052792752,-43.0228815454562));
#23487=CARTESIAN_POINT('Ctrl Pts',(-8.14522133615151,0.140918662692672,
-42.9051069397892));
#23488=CARTESIAN_POINT('Ctrl Pts',(-7.24071355790799,-3.73316967960476,
-42.787332334122));
#23489=CARTESIAN_POINT('Ctrl Pts',(-4.60943042251266,-6.71696656716463,
-42.6695577284549));
#23490=CARTESIAN_POINT('Ctrl Pts',(-0.878883961694459,-8.09889200238335,
-42.5517831227878));
#23491=CARTESIAN_POINT('Ctrl Pts',(3.0612599586438,-7.5493825012379,-42.4340085171206));
#23492=CARTESIAN_POINT('Ctrl Pts',(6.27135038133359,-5.19948584755646,-42.3162339114535));
#23493=CARTESIAN_POINT('Ctrl Pts',(7.98584051436349,-1.60960863676344,-42.1984593057864));
#23494=CARTESIAN_POINT('Ctrl Pts',(7.79585638583573,2.3641302620239,-42.0806847001193));
#23495=CARTESIAN_POINT('Ctrl Pts',(5.74670567278627,5.7740681148354,-41.9629100944521));
#23496=CARTESIAN_POINT('Ctrl Pts',(2.3270726638678,7.80699823885416,-41.845135488785));
#23497=CARTESIAN_POINT('Ctrl Pts',(-1.64752384390083,7.97810465387431,-41.7273608831179));
#23498=CARTESIAN_POINT('Ctrl Pts',(-5.22921659277671,6.24658166601716,-41.6095862774508));
#23499=CARTESIAN_POINT('Ctrl Pts',(-7.56383855541021,3.0253652658948,-41.4918116717836));
#23500=CARTESIAN_POINT('Ctrl Pts',(-8.094625865768,-0.917344416036007,-41.3740370661165));
#23501=CARTESIAN_POINT('Ctrl Pts',(-6.69499563390635,-4.64128453624294,
-41.2562624604494));
#23502=CARTESIAN_POINT('Ctrl Pts',(-3.69873360817373,-7.25836471804489,
-41.1384878547822));
#23503=CARTESIAN_POINT('Ctrl Pts',(0.179607510480324,-8.14446006967754,
-41.0207132491151));
#23504=CARTESIAN_POINT('Ctrl Pts',(4.01511558228392,-7.08825334940095,-40.902938643448));
#23505=CARTESIAN_POINT('Ctrl Pts',(6.893093351562,-4.34163019280138,-40.7851640377808));
#23506=CARTESIAN_POINT('Ctrl Pts',(8.12719671000602,-0.559609078964911,
-40.6673894321138));
#23507=CARTESIAN_POINT('Ctrl Pts',(7.42311498636844,3.35586837994955,-40.5496148264466));
#23508=CARTESIAN_POINT('Ctrl Pts',(4.94875856131471,6.47103371851879,-40.4318402207795));
#23509=CARTESIAN_POINT('Ctrl Pts',(1.29421536822631,8.04297800973245,-40.3140656151123));
#23510=CARTESIAN_POINT('Ctrl Pts',(-2.66897409112126,7.69682181067721,-40.1962910094452));
#23511=CARTESIAN_POINT('Ctrl Pts',(-5.99566292762737,5.51511692919266,-40.0785164037781));
#23512=CARTESIAN_POINT('Ctrl Pts',(-7.89249779871756,2.01815935486554,-39.960741798111));
#23513=CARTESIAN_POINT('Ctrl Pts',(-7.90711890783457,-1.960091646265,-39.8429671924438));
#23514=CARTESIAN_POINT('Ctrl Pts',(-6.03603939270779,-5.47089728783792,
-39.7251925867767));
#23515=CARTESIAN_POINT('Ctrl Pts',(-2.7254768770772,-7.67699579763541,-39.6074179811095));
#23516=CARTESIAN_POINT('Ctrl Pts',(1.23506112372953,-8.05227375994144,-39.4896433754425));
#23517=CARTESIAN_POINT('Ctrl Pts',(4.90106004410261,-6.50723436864699,-39.3718687697753));
#23518=CARTESIAN_POINT('Ctrl Pts',(7.39824740462043,-3.41034074901742,-39.2540941641082));
#23519=CARTESIAN_POINT('Ctrl Pts',(8.13109051892145,0.49985563666857,-39.1363195584411));
#23520=CARTESIAN_POINT('Ctrl Pts',(6.92481995021625,4.29084576062654,-39.0185449527739));
#23521=CARTESIAN_POINT('Ctrl Pts',(4.06710876767287,7.05854906877053,-38.9007703471068));
#23522=CARTESIAN_POINT('Ctrl Pts',(0.239467876019258,8.14291985843953,-38.7829957414397));
#23523=CARTESIAN_POINT('Ctrl Pts',(-3.64528164500238,7.28535588784087,-38.6652211357726));
#23524=CARTESIAN_POINT('Ctrl Pts',(-6.66069937106789,4.69037019578824,-38.5474465301054));
#23525=CARTESIAN_POINT('Ctrl Pts',(-8.0876643232179,0.976818549289544,-38.4296719244383));
#23526=CARTESIAN_POINT('Ctrl Pts',(-7.58587193165152,-2.96968613177471,
-38.3118973187712));
#23527=CARTESIAN_POINT('Ctrl Pts',(-5.2749903373771,-6.20797596874618,-38.194122713104));
#23528=CARTESIAN_POINT('Ctrl Pts',(-1.70612177206955,-7.96577913134455,
-38.0763481074369));
#23529=CARTESIAN_POINT('Ctrl Pts',(2.26962506882539,-7.82389230283792,-37.9585735017698));
#23530=CARTESIAN_POINT('Ctrl Pts',(5.70410858860697,-5.81615283720149,-37.8407988961027));
#23531=CARTESIAN_POINT('Ctrl Pts',(7.77826843198531,-2.4213692372992,-37.7230242904356));
#23532=CARTESIAN_POINT('Ctrl Pts',(7.99745607393352,1.55086587324671,-37.6052496847684));
#23533=CARTESIAN_POINT('Ctrl Pts',(6.30939939298919,5.15324828017407,-37.4874750791013));
#23534=CARTESIAN_POINT('Ctrl Pts',(3.11666837386201,7.52667707291178,-37.3697004734342));
#23535=CARTESIAN_POINT('Ctrl Pts',(-0.819329880552923,8.10513324220875,
-37.251925867767));
#23536=CARTESIAN_POINT('Ctrl Pts',(-4.55993349459366,6.7506666506058,-37.1341512620999));
#23537=CARTESIAN_POINT('Ctrl Pts',(-7.2130773104214,3.78629055527431,-37.0163766564328));
#23538=CARTESIAN_POINT('Ctrl Pts',(-8.14603765464913,-0.0810428776644847,
-36.8986020507657));
#23539=CARTESIAN_POINT('Ctrl Pts',(-7.13631735496811,-3.92905408592493,
-36.7808274450985));
#23540=CARTESIAN_POINT('Ctrl Pts',(-4.42472301872742,-6.84004891051797,
-36.6630528394314));
#23541=CARTESIAN_POINT('Ctrl Pts',(-0.657904940076782,-8.11984005263565,
-36.5452782337643));
#23542=CARTESIAN_POINT('Ctrl Pts',(3.26579151798057,-7.46315864218313,-36.4275036280972));
#23543=CARTESIAN_POINT('Ctrl Pts',(6.41069753942071,-5.02673800845634,-36.30972902243));
#23544=CARTESIAN_POINT('Ctrl Pts',(8.02669021463193,-1.39136086516467,-36.1919544167629));
#23545=CARTESIAN_POINT('Ctrl Pts',(7.72863209437362,2.57547648491176,-36.0741798110958));
#23546=CARTESIAN_POINT('Ctrl Pts',(5.58709980778241,5.92884035320494,-35.9564052054286));
#23547=CARTESIAN_POINT('Ctrl Pts',(3.2715807958743,7.22045492340081,-35.8778888016505));
#23548=CARTESIAN_POINT('Ctrl Pts',(2.02934030215363,7.55416851400967,-35.8386305997615));
#23549=CARTESIAN_POINT('Ctrl Pts',(6.09356451288681,-5.33879890774007,-48.4841082007155));
#23550=CARTESIAN_POINT('Ctrl Pts',(6.97149994399703,-4.33674652103877,-48.4448499988265));
#23551=CARTESIAN_POINT('Ctrl Pts',(8.22276701277896,-1.89224343499068,-48.3663335950484));
#23552=CARTESIAN_POINT('Ctrl Pts',(8.13810611461702,2.22790641565228,-48.2485589893812));
#23553=CARTESIAN_POINT('Ctrl Pts',(6.11278597432722,5.81591838961622,-48.1307843837142));
#23554=CARTESIAN_POINT('Ctrl Pts',(2.6296192901479,8.01734167049212,-48.0130097780469));
#23555=CARTESIAN_POINT('Ctrl Pts',(-1.4806331202341,8.30658236639193,-47.8952351723799));
#23556=CARTESIAN_POINT('Ctrl Pts',(-5.23779660691551,6.61495420237904,-47.7774605667127));
#23557=CARTESIAN_POINT('Ctrl Pts',(-7.74583599739651,3.34573521925119,-47.6596859610457));
#23558=CARTESIAN_POINT('Ctrl Pts',(-8.40664124628672,-0.721355980820569,
-47.5419113553785));
#23559=CARTESIAN_POINT('Ctrl Pts',(-7.06261736652514,-4.61642869377352,
-47.4241367497114));
#23560=CARTESIAN_POINT('Ctrl Pts',(-4.03429160538818,-7.41056347354498,
-47.3063621440442));
#23561=CARTESIAN_POINT('Ctrl Pts',(-0.04386199881008,-8.4374196345273,-47.1885875383771));
#23562=CARTESIAN_POINT('Ctrl Pts',(3.95702767181747,-7.45210695417129,-47.07081293271));
#23563=CARTESIAN_POINT('Ctrl Pts',(7.0142400262719,-4.68960620126019,-46.9530383270429));
#23564=CARTESIAN_POINT('Ctrl Pts',(8.39868669392937,-0.808721361269664,
-46.8352637213757));
#23565=CARTESIAN_POINT('Ctrl Pts',(7.78020299818498,3.26502830145453,-46.7174891157086));
#23566=CARTESIAN_POINT('Ctrl Pts',(5.30628574732215,6.56012959129681,-46.5997145100415));
#23567=CARTESIAN_POINT('Ctrl Pts',(1.56691815787412,8.290762087659,-46.4819399043743));
#23568=CARTESIAN_POINT('Ctrl Pts',(-2.54613023819965,8.04420222448489,-46.3641652987072));
#23569=CARTESIAN_POINT('Ctrl Pts',(-6.05197398148885,5.87924990905731,-46.2463906930401));
#23570=CARTESIAN_POINT('Ctrl Pts',(-8.11453462226977,2.31220597016818,-46.1286160873729));
#23571=CARTESIAN_POINT('Ctrl Pts',(-8.24192985277003,-1.80625604026594,
-46.0108414817058));
#23572=CARTESIAN_POINT('Ctrl Pts',(-6.40377828321054,-5.49395961752304,
-45.8930668760387));
#23573=CARTESIAN_POINT('Ctrl Pts',(-3.03844483519571,-7.87145612736966,
-45.7752922703716));
#23574=CARTESIAN_POINT('Ctrl Pts',(1.05150112831493,-8.37175692177514,-45.6575176647045));
#23575=CARTESIAN_POINT('Ctrl Pts',(4.89068365232167,-6.87554957758499,-45.5397430590373));
#23576=CARTESIAN_POINT('Ctrl Pts',(7.56352919268905,-3.73965168591192,-45.4219684533702));
#23577=CARTESIAN_POINT('Ctrl Pts',(8.43261385803414,0.288083498271241,-45.3041938477031));
#23578=CARTESIAN_POINT('Ctrl Pts',(7.29067713854007,4.2471161324196,-45.1864192420359));
#23579=CARTESIAN_POINT('Ctrl Pts',(4.41004967826638,7.19329065281592,-45.0686446363688));
#23580=CARTESIAN_POINT('Ctrl Pts',(0.477707487483417,8.42399929588601,-44.9508700307017));
#23581=CARTESIAN_POINT('Ctrl Pts',(-3.56855904386543,7.64574096678149,-44.8330954250346));
#23582=CARTESIAN_POINT('Ctrl Pts',(-6.76379069195239,5.04411578536195,-44.7153208193674));
#23583=CARTESIAN_POINT('Ctrl Pts',(-8.3459842058294,1.23956291358046,-44.5975462137003));
#23584=CARTESIAN_POINT('Ctrl Pts',(-7.93781589382472,-2.86060263168824,
-44.4797716080332));
#23585=CARTESIAN_POINT('Ctrl Pts',(-5.63662629801377,-6.27856771542826,
-44.3619970023661));
#23586=CARTESIAN_POINT('Ctrl Pts',(-1.99120628747333,-8.19921130971783,
-44.2442223966989));
#23587=CARTESIAN_POINT('Ctrl Pts',(2.12907934517964,-8.16449568084935,-44.1264477910318));
#23588=CARTESIAN_POINT('Ctrl Pts',(5.74161919873576,-6.18269985988217,-44.0086731853647));
#23589=CARTESIAN_POINT('Ctrl Pts',(7.98488978577069,-2.72644524789567,-43.8908985796975));
#23590=CARTESIAN_POINT('Ctrl Pts',(8.32391284231425,1.38001578767571,-43.7731239740304));
#23591=CARTESIAN_POINT('Ctrl Pts',(6.67783768219246,5.1573687546043,-43.6553493683633));
#23592=CARTESIAN_POINT('Ctrl Pts',(3.43922258019218,7.70478530684499,-43.5375747626961));
#23593=CARTESIAN_POINT('Ctrl Pts',(-0.619583066806221,8.41475403110543,
-43.4198001570291));
#23594=CARTESIAN_POINT('Ctrl Pts',(-4.53062968937796,7.11796060669102,-43.3020255513619));
#23595=CARTESIAN_POINT('Ctrl Pts',(-7.36120549406269,4.12366611825681,-43.1842509456948));
#23596=CARTESIAN_POINT('Ctrl Pts',(-8.43627085845454,0.145954045743379,
-43.0664763400276));
#23597=CARTESIAN_POINT('Ctrl Pts',(-7.49944271150493,-3.86656534892841,
-42.9487017343606));
#23598=CARTESIAN_POINT('Ctrl Pts',(-4.77413712196194,-6.95698090563593,
-42.8309271286933));
#23599=CARTESIAN_POINT('Ctrl Pts',(-0.910288726114504,-8.38828605948718,
-42.7131525230263));
#23600=CARTESIAN_POINT('Ctrl Pts',(3.17064658079171,-7.8191411830451,-42.5953779173591));
#23601=CARTESIAN_POINT('Ctrl Pts',(6.49544171751139,-5.38527673152374,-42.477603311692));
#23602=CARTESIAN_POINT('Ctrl Pts',(8.27119495360724,-1.66712405660176,-42.3598287060249));
#23603=CARTESIAN_POINT('Ctrl Pts',(8.07442220785581,2.44860666297451,-42.2420541003577));
#23604=CARTESIAN_POINT('Ctrl Pts',(5.95205011609281,5.98039028794925,-42.1242794946906));
#23605=CARTESIAN_POINT('Ctrl Pts',(2.41022490236832,8.08596218768562,-42.0065048890235));
#23606=CARTESIAN_POINT('Ctrl Pts',(-1.70639407074438,8.26318267110237,-41.8887302833564));
#23607=CARTESIAN_POINT('Ctrl Pts',(-5.41606983206093,6.46978795285578,-41.7709556776892));
#23608=CARTESIAN_POINT('Ctrl Pts',(-7.83411378888465,3.13346927916731,-41.6531810720221));
#23609=CARTESIAN_POINT('Ctrl Pts',(-8.38386748293525,-0.950123470533844,
-41.535406466355));
#23610=CARTESIAN_POINT('Ctrl Pts',(-6.93422489492358,-4.80712946437895,
-41.4176318606879));
#23611=CARTESIAN_POINT('Ctrl Pts',(-3.83089878888002,-7.51772459259022,
-41.2998572550207));
#23612=CARTESIAN_POINT('Ctrl Pts',(0.186025344688875,-8.43548238998882,
-41.1820826493536));
#23613=CARTESIAN_POINT('Ctrl Pts',(4.15858589745246,-7.3415347110933,-41.0643080436865));
#23614=CARTESIAN_POINT('Ctrl Pts',(7.13940114902576,-4.49676770736134,-40.9465334380193));
#23615=CARTESIAN_POINT('Ctrl Pts',(8.41760216646814,-0.579605337923066,
-40.8287588323522));
#23616=CARTESIAN_POINT('Ctrl Pts',(7.68836180798567,3.47578211201243,-40.7109842266851));
#23617=CARTESIAN_POINT('Ctrl Pts',(5.12559032018552,6.70226024937101,-40.593209621018));
#23618=CARTESIAN_POINT('Ctrl Pts',(1.34046098257293,8.33037411734177,-40.4754350153508));
#23619=CARTESIAN_POINT('Ctrl Pts',(-2.76434333919955,7.97184887486595,-40.3576604096838));
#23620=CARTESIAN_POINT('Ctrl Pts',(-6.20990324829623,5.71218611631991,-40.2398858040166));
#23621=CARTESIAN_POINT('Ctrl Pts',(-8.17451686478015,2.09027333334737,-40.1221111983495));
#23622=CARTESIAN_POINT('Ctrl Pts',(-8.18966042339832,-2.03013071749117,
-40.0043365926823));
#23623=CARTESIAN_POINT('Ctrl Pts',(-6.25172246740249,-5.66638639445397,
-39.8865619870152));
#23624=CARTESIAN_POINT('Ctrl Pts',(-2.82286511373573,-7.95131442783728,
-39.768787381348));
#23625=CARTESIAN_POINT('Ctrl Pts',(1.27919300612309,-8.34000202840266,-39.651012775681));
#23626=CARTESIAN_POINT('Ctrl Pts',(5.07618741335941,-6.73975444101172,-39.5332381700138));
#23627=CARTESIAN_POINT('Ctrl Pts',(7.66260564414886,-3.53220091768916,-39.4154635643467));
#23628=CARTESIAN_POINT('Ctrl Pts',(8.42163511110229,0.517716752808797,-39.2976889586796));
#23629=CARTESIAN_POINT('Ctrl Pts',(7.17226141992802,4.4441686179642,-39.1799143530125));
#23630=CARTESIAN_POINT('Ctrl Pts',(4.21243693189744,7.31076902079321,-39.0621397473453));
#23631=CARTESIAN_POINT('Ctrl Pts',(0.248024673685762,8.43388714307694,-38.9443651416782));
#23632=CARTESIAN_POINT('Ctrl Pts',(-3.77553685080373,7.54568022568945,-38.8265905360111));
#23633=CARTESIAN_POINT('Ctrl Pts',(-6.89870313918519,4.85796907966996,-38.7088159303439));
#23634=CARTESIAN_POINT('Ctrl Pts',(-8.37665718672332,1.01172276618119,-38.5910413246768));
#23635=CARTESIAN_POINT('Ctrl Pts',(-7.856934473827,-3.07580058764674,-38.4732667190097));
#23636=CARTESIAN_POINT('Ctrl Pts',(-5.46347918924325,-6.4298027756069,-38.3554921133425));
#23637=CARTESIAN_POINT('Ctrl Pts',(-1.76708585226559,-8.25041672623214,
-38.2377175076754));
#23638=CARTESIAN_POINT('Ctrl Pts',(2.35072455830847,-8.10345991964222,-38.1199429020083));
#23639=CARTESIAN_POINT('Ctrl Pts',(5.90793092950644,-6.02397880472869,-38.0021682963412));
#23640=CARTESIAN_POINT('Ctrl Pts',(8.05620579157874,-2.50789093275115,-37.8843936906741));
#23641=CARTESIAN_POINT('Ctrl Pts',(8.28322556673132,1.60628226439634,-37.7666190850069));
#23642=CARTESIAN_POINT('Ctrl Pts',(6.53485031734875,5.33738697798904,-37.6488444793398));
#23643=CARTESIAN_POINT('Ctrl Pts',(3.22803487993391,7.79562443188376,-37.5310698736727));
#23644=CARTESIAN_POINT('Ctrl Pts',(-0.848606625837317,8.39475031472183,
-37.4132952680055));
#23645=CARTESIAN_POINT('Ctrl Pts',(-4.72287154262983,6.99188517896739,-37.2955206623384));
#23646=CARTESIAN_POINT('Ctrl Pts',(-7.47081895044476,3.92158436890243,-37.1777460566712));
#23647=CARTESIAN_POINT('Ctrl Pts',(-8.43711634609307,-0.0839387462795732,
-37.0599714510042));
#23648=CARTESIAN_POINT('Ctrl Pts',(-7.39131616610511,-4.06944920443886,
-36.942196845337));
#23649=CARTESIAN_POINT('Ctrl Pts',(-4.58282965177962,-7.08446129488128,
-36.8244222396699));
#23650=CARTESIAN_POINT('Ctrl Pts',(-0.681413560730255,-8.40998263697618,
-36.7066476340027));
#23651=CARTESIAN_POINT('Ctrl Pts',(3.38248657413956,-7.72983632570271,-36.5888730283357));
#23652=CARTESIAN_POINT('Ctrl Pts',(6.63976810478354,-5.20635617176029,-36.4710984226685));
#23653=CARTESIAN_POINT('Ctrl Pts',(8.31350431780115,-1.44107773576215,-36.3533238170014));
#23654=CARTESIAN_POINT('Ctrl Pts',(8.00479582109024,2.66750482517421,-36.2355492113343));
#23655=CARTESIAN_POINT('Ctrl Pts',(5.78674112666189,6.14069293294423,-36.1177746056671));
#23656=CARTESIAN_POINT('Ctrl Pts',(3.38848271769057,7.47846018434309,-36.039258201889));
#23657=CARTESIAN_POINT('Ctrl Pts',(2.10185380438477,7.82409821225381,-36.));
#23658=CARTESIAN_POINT('Ctrl Pts',(2.10185380438477,7.82409821225381,-36.));
#23659=CARTESIAN_POINT('Ctrl Pts',(2.30082749329421,7.7596064443525,-36.));
#23660=CARTESIAN_POINT('Ctrl Pts',(2.49685155452529,7.68738684032504,-36.));
#23661=CARTESIAN_POINT('Ctrl Pts',(2.689555562529,7.60776034250278,-36.));
#23662=CARTESIAN_POINT('Ctrl Pts',(2.88412146665351,7.5273644975925,-36.));
#23663=CARTESIAN_POINT('Ctrl Pts',(3.07530344788642,7.43941759948373,-36.));
#23664=CARTESIAN_POINT('Ctrl Pts',(3.26270123260074,7.3442002249883,-36.));
#23665=CARTESIAN_POINT('Ctrl Pts',(3.45039098213973,7.24883450229285,-36.));
#23666=CARTESIAN_POINT('Ctrl Pts',(3.63428531442281,7.14617523423964,-36.));
#23667=CARTESIAN_POINT('Ctrl Pts',(3.81395427779333,7.0364602726816,-36.));
#23668=CARTESIAN_POINT('Ctrl Pts',(3.99143524378484,6.92808141305137,-36.));
#23669=CARTESIAN_POINT('Ctrl Pts',(4.16479360607289,6.81281720683301,-36.));
#23670=CARTESIAN_POINT('Ctrl Pts',(4.33358005423134,6.69086045395404,-36.));
#23671=CARTESIAN_POINT('Ctrl Pts',(4.43066189457222,6.62071390995915,-36.));
#23672=CARTESIAN_POINT('Ctrl Pts',(4.52623053968623,6.54835265306457,-36.));
#23673=CARTESIAN_POINT('Ctrl Pts',(4.62019422903912,6.47380866470389,-36.));
#23674=CARTESIAN_POINT('Ctrl Pts',(4.66632187332592,6.4372143312704,-36.));
#23675=CARTESIAN_POINT('Ctrl Pts',(4.71206266158868,6.40009392819384,-36.));
#23676=CARTESIAN_POINT('Ctrl Pts',(4.75740528585098,6.36245096836916,-36.));
#23677=CARTESIAN_POINT('Ctrl Pts',(4.77704327692769,6.34614771902784,-36.));
#23678=CARTESIAN_POINT('Ctrl Pts',(4.79660790428669,6.32974532323648,-36.));
#23679=CARTESIAN_POINT('Ctrl Pts',(4.81609406394226,6.31324758769124,-36.));
#23680=CARTESIAN_POINT('Ctrl Pts',(4.97467824697507,6.17898409198058,-36.));
#23681=CARTESIAN_POINT('Ctrl Pts',(5.12764651540678,6.03876779721708,-36.));
#23682=CARTESIAN_POINT('Ctrl Pts',(5.2746131961221,5.89285549710303,-36.));
#23683=CARTESIAN_POINT('Ctrl Pts',(5.32270090376221,5.84511278430017,-36.));
#23684=CARTESIAN_POINT('Ctrl Pts',(5.37014581825667,5.79675992826811,-36.));
#23685=CARTESIAN_POINT('Ctrl Pts',(5.41693362537058,5.74780501532688,-36.));
#23686=CARTESIAN_POINT('Ctrl Pts',(5.55998414133242,5.59812872171345,-36.));
#23687=CARTESIAN_POINT('Ctrl Pts',(5.69689520934925,5.44282686808312,-36.));
#23688=CARTESIAN_POINT('Ctrl Pts',(5.82744384911316,5.28234284303486,-36.));
#23689=CARTESIAN_POINT('Ctrl Pts',(5.95822183969036,5.12157687600901,-36.));
#23690=CARTESIAN_POINT('Ctrl Pts',(6.08261535950187,4.95560987748997,-36.));
#23691=CARTESIAN_POINT('Ctrl Pts',(6.20035566189897,4.78486047060351,-36.));
#23692=CARTESIAN_POINT('Ctrl Pts',(6.31730039604029,4.61526481315583,-36.));
#23693=CARTESIAN_POINT('Ctrl Pts',(6.42768178546486,4.44095051821423,-36.));
#23694=CARTESIAN_POINT('Ctrl Pts',(6.5311881819826,4.26231063676596,-36.));
#23695=CARTESIAN_POINT('Ctrl Pts',(6.57281068005803,4.1904750945007,-36.));
#23696=CARTESIAN_POINT('Ctrl Pts',(6.61332089089221,4.11793994409325,-36.));
#23697=CARTESIAN_POINT('Ctrl Pts',(6.65269617438066,4.04473030956882,-36.));
#23698=CARTESIAN_POINT('Ctrl Pts',(6.66624691189691,4.01953570896632,-36.));
#23699=CARTESIAN_POINT('Ctrl Pts',(6.67966322249545,3.99426122477837,-36.));
#23700=CARTESIAN_POINT('Ctrl Pts',(6.69294414431972,3.96890787749673,-36.));
#23701=CARTESIAN_POINT('Ctrl Pts',(6.70467576680984,3.9465121505205,-36.));
#23702=CARTESIAN_POINT('Ctrl Pts',(6.71630216391417,3.92405397007754,-36.));
#23703=CARTESIAN_POINT('Ctrl Pts',(6.72781502483286,3.90154926003667,-36.));
#23704=CARTESIAN_POINT('Ctrl Pts',(6.82109912412433,3.71920261129266,-36.));
#23705=CARTESIAN_POINT('Ctrl Pts',(6.90705463802017,3.53357359685618,-36.));
#23706=CARTESIAN_POINT('Ctrl Pts',(6.98547179470946,3.34508790000042,-36.));
#23707=CARTESIAN_POINT('Ctrl Pts',(7.06354641293418,3.1574255382912,-36.));
#23708=CARTESIAN_POINT('Ctrl Pts',(7.13414864143153,2.96693075444826,-36.));
#23709=CARTESIAN_POINT('Ctrl Pts',(7.1970241992718,2.77400366738376,-36.));
#23710=CARTESIAN_POINT('Ctrl Pts',(7.23384826254667,2.66101287246235,-36.));
#23711=CARTESIAN_POINT('Ctrl Pts',(7.26802113681645,2.5471874598649,-36.));
#23712=CARTESIAN_POINT('Ctrl Pts',(7.29948362757048,2.43260592056936,-36.));
#23713=CARTESIAN_POINT('Ctrl Pts',(7.3534896782826,2.23592421249213,-36.));
#23714=CARTESIAN_POINT('Ctrl Pts',(7.39951253414964,2.03701441433134,-36.));
#23715=CARTESIAN_POINT('Ctrl Pts',(7.43751281341565,1.83636829928625,-36.));
#23716=CARTESIAN_POINT('Ctrl Pts',(7.46184111046734,1.70791191992879,-36.));
#23717=CARTESIAN_POINT('Ctrl Pts',(7.48288011604595,1.57874381119794,-36.));
#23718=CARTESIAN_POINT('Ctrl Pts',(7.50060831271862,1.44899412782466,-36.));
#23719=CARTESIAN_POINT('Ctrl Pts',(7.50964573314831,1.3828507709501,-36.));
#23720=CARTESIAN_POINT('Ctrl Pts',(7.51782262655261,1.31655630325051,-36.));
#23721=CARTESIAN_POINT('Ctrl Pts',(7.5251352705533,1.25012817277057,-36.));
#23722=CARTESIAN_POINT('Ctrl Pts',(7.52928149862857,1.21246379589706,-36.));
#23723=CARTESIAN_POINT('Ctrl Pts',(7.53314987483263,1.17475645171563,-36.));
#23724=CARTESIAN_POINT('Ctrl Pts',(7.53673963659345,1.13700934710221,-36.));
#23725=CARTESIAN_POINT('Ctrl Pts',(7.5398457973277,1.10434740962724,-36.));
#23726=CARTESIAN_POINT('Ctrl Pts',(7.54274371571818,1.07165049518016,-36.));
#23727=CARTESIAN_POINT('Ctrl Pts',(7.54543050825926,1.03895175486804,-36.));
#23728=CARTESIAN_POINT('Ctrl Pts',(7.56194131066929,0.838012370045629,-36.));
#23729=CARTESIAN_POINT('Ctrl Pts',(7.57050463381881,0.636810188211384,-36.));
#23730=CARTESIAN_POINT('Ctrl Pts',(7.5711535550322,0.435821667465856,-36.));
#23731=CARTESIAN_POINT('Ctrl Pts',(7.57180236612707,0.234867253413772,-36.));
#23732=CARTESIAN_POINT('Ctrl Pts',(7.56453941489479,0.03412571703456,-36.));
#23733=CARTESIAN_POINT('Ctrl Pts',(7.54934569594904,-0.165927099754431,
-36.));
#23734=CARTESIAN_POINT('Ctrl Pts',(7.53434530981631,-0.363434340048337,
-36.));
#23735=CARTESIAN_POINT('Ctrl Pts',(7.51161456525456,-0.560270924380012,
-36.));
#23736=CARTESIAN_POINT('Ctrl Pts',(7.48108594581124,-0.755969235382515,
-36.));
#23737=CARTESIAN_POINT('Ctrl Pts',(7.45371072786321,-0.931453224290022,
-36.));
#23738=CARTESIAN_POINT('Ctrl Pts',(7.42006472051527,-1.10602214252325,-36.));
#23739=CARTESIAN_POINT('Ctrl Pts',(7.3800660535423,-1.27932570484005,-36.));
#23740=CARTESIAN_POINT('Ctrl Pts',(7.34592028888866,-1.42727020150302,-36.));
#23741=CARTESIAN_POINT('Ctrl Pts',(7.30714422290839,-1.5742924439295,-36.));
#23742=CARTESIAN_POINT('Ctrl Pts',(7.26380602496235,-1.72018741510414,-36.));
#23743=CARTESIAN_POINT('Ctrl Pts',(7.25535126498663,-1.74864976521113,-36.));
#23744=CARTESIAN_POINT('Ctrl Pts',(7.24672283231802,-1.77706917955542,-36.));
#23745=CARTESIAN_POINT('Ctrl Pts',(7.23792117432662,-1.80544408661968,-36.));
#23746=CARTESIAN_POINT('Ctrl Pts',(7.23013840559116,-1.83053428437413,-36.));
#23747=CARTESIAN_POINT('Ctrl Pts',(7.22222273184584,-1.85558146827501,-36.));
#23748=CARTESIAN_POINT('Ctrl Pts',(7.21417570637184,-1.88058164144947,-36.));
#23749=CARTESIAN_POINT('Ctrl Pts',(7.15325531511497,-2.06984664827677,-36.));
#23750=CARTESIAN_POINT('Ctrl Pts',(7.08479320734585,-2.25647542918358,-36.));
#23751=CARTESIAN_POINT('Ctrl Pts',(7.00902681125197,-2.44004188332158,-36.));
#23752=CARTESIAN_POINT('Ctrl Pts',(6.93177164355565,-2.62721532602142,-36.));
#23753=CARTESIAN_POINT('Ctrl Pts',(6.84692207561124,-2.81120566590633,-36.));
#23754=CARTESIAN_POINT('Ctrl Pts',(6.75468151121674,-2.99153375862684,-36.));
#23755=CARTESIAN_POINT('Ctrl Pts',(6.71535300589298,-3.06842004397361,-36.));
#23756=CARTESIAN_POINT('Ctrl Pts',(6.67468031908831,-3.14464016518226,-36.));
#23757=CARTESIAN_POINT('Ctrl Pts',(6.63267679451784,-3.22015498690596,-36.));
#23758=CARTESIAN_POINT('Ctrl Pts',(6.60409277041902,-3.27154394785723,-36.));
#23759=CARTESIAN_POINT('Ctrl Pts',(6.57489240539613,-3.32260625824744,-36.));
#23760=CARTESIAN_POINT('Ctrl Pts',(6.54507954995881,-3.3733292184608,-36.));
#23761=CARTESIAN_POINT('Ctrl Pts',(6.52647860828883,-3.40497646628117,-36.));
#23762=CARTESIAN_POINT('Ctrl Pts',(6.50763779811667,-3.43649380740715,-36.));
#23763=CARTESIAN_POINT('Ctrl Pts',(6.4885706896475,-3.46785768454478,-36.));
#23764=CARTESIAN_POINT('Ctrl Pts',(6.38641008318404,-3.63590375794958,-36.));
#23765=CARTESIAN_POINT('Ctrl Pts',(6.27768402389073,-3.79967230920287,-36.));
#23766=CARTESIAN_POINT('Ctrl Pts',(6.16259229716626,-3.95873109508268,-36.));
#23767=CARTESIAN_POINT('Ctrl Pts',(6.04877580733772,-4.11602748119538,-36.));
#23768=CARTESIAN_POINT('Ctrl Pts',(5.92873351593867,-4.26871840542356,-36.));
#23769=CARTESIAN_POINT('Ctrl Pts',(5.80262143415048,-4.41635115060161,-36.));
#23770=CARTESIAN_POINT('Ctrl Pts',(5.77983952847348,-4.44302072284079,-36.));
#23771=CARTESIAN_POINT('Ctrl Pts',(5.75685945345182,-4.46952512396077,-36.));
#23772=CARTESIAN_POINT('Ctrl Pts',(5.73368201345117,-4.49586154264461,-36.));
#23773=CARTESIAN_POINT('Ctrl Pts',(5.64631446617484,-4.59513688558089,-36.));
#23774=CARTESIAN_POINT('Ctrl Pts',(5.55614292429607,-4.69202604818322,-36.));
#23775=CARTESIAN_POINT('Ctrl Pts',(5.46328275624301,-4.78643223329955,-36.));
#23776=CARTESIAN_POINT('Ctrl Pts',(5.46288453460432,-4.78623668048091,-48.));
#23777=CARTESIAN_POINT('Ctrl Pts',(5.59774281609631,-4.64891404164603,-48.));
#23778=CARTESIAN_POINT('Ctrl Pts',(5.72676707811106,-4.50639591331986,-48.));
#23779=CARTESIAN_POINT('Ctrl Pts',(5.84982506430564,-4.35916096560483,-48.));
#23780=CARTESIAN_POINT('Ctrl Pts',(5.97480997239641,-4.20962051742283,-48.));
#23781=CARTESIAN_POINT('Ctrl Pts',(6.09364072129775,-4.05521394491186,-48.));
#23782=CARTESIAN_POINT('Ctrl Pts',(6.20615004774937,-3.89639687941618,-48.));
#23783=CARTESIAN_POINT('Ctrl Pts',(6.3253334379493,-3.72815877076906,-48.));
#23784=CARTESIAN_POINT('Ctrl Pts',(6.437424033659,-3.55497113855592,-48.));
#23785=CARTESIAN_POINT('Ctrl Pts',(6.54218080780119,-3.37732938918555,-48.));
#23786=CARTESIAN_POINT('Ctrl Pts',(6.64196722139062,-3.20811615005545,-48.));
#23787=CARTESIAN_POINT('Ctrl Pts',(6.73509931029878,-3.03486055006183,-48.));
#23788=CARTESIAN_POINT('Ctrl Pts',(6.82132597032137,-2.85795972896024,-48.));
#23789=CARTESIAN_POINT('Ctrl Pts',(6.86766051232553,-2.76290074692666,-48.));
#23790=CARTESIAN_POINT('Ctrl Pts',(6.91200033896626,-2.66678873196007,-48.));
#23791=CARTESIAN_POINT('Ctrl Pts',(6.95430087098005,-2.56968260604186,-48.));
#23792=CARTESIAN_POINT('Ctrl Pts',(6.97457089805417,-2.52315024089848,-48.));
#23793=CARTESIAN_POINT('Ctrl Pts',(6.99437259374271,-2.47638958030327,-48.));
#23794=CARTESIAN_POINT('Ctrl Pts',(7.01370070790936,-2.4294069894874,-48.));
#23795=CARTESIAN_POINT('Ctrl Pts',(7.02151887657497,-2.41040266158564,-48.));
#23796=CARTESIAN_POINT('Ctrl Pts',(7.02925902870664,-2.39136323223209,-48.));
#23797=CARTESIAN_POINT('Ctrl Pts',(7.03691728406108,-2.37229819353851,-48.));
#23798=CARTESIAN_POINT('Ctrl Pts',(7.11159745538058,-2.18638374044777,-48.));
#23799=CARTESIAN_POINT('Ctrl Pts',(7.17858966450582,-1.99780302602708,-48.));
#23800=CARTESIAN_POINT('Ctrl Pts',(7.23771290858855,-1.80701588371416,-48.));
#23801=CARTESIAN_POINT('Ctrl Pts',(7.25137618887209,-1.76292530241471,-48.));
#23802=CARTESIAN_POINT('Ctrl Pts',(7.26461905057976,-1.71871673873425,-48.));
#23803=CARTESIAN_POINT('Ctrl Pts',(7.27743895299859,-1.67439562023028,-48.));
#23804=CARTESIAN_POINT('Ctrl Pts',(7.33236359165557,-1.48450950884079,-48.));
#23805=CARTESIAN_POINT('Ctrl Pts',(7.37952838594581,-1.29255934235065,-48.));
#23806=CARTESIAN_POINT('Ctrl Pts',(7.41900439368324,-1.09903098681805,-48.));
#23807=CARTESIAN_POINT('Ctrl Pts',(7.45887410032125,-0.90357255007484,-48.));
#23808=CARTESIAN_POINT('Ctrl Pts',(7.49090103834248,-0.706503641732061,
-48.));
#23809=CARTESIAN_POINT('Ctrl Pts',(7.51510880906928,-0.508305269117967,
-48.));
#23810=CARTESIAN_POINT('Ctrl Pts',(7.53937115123289,-0.30966009906489,-48.));
#23811=CARTESIAN_POINT('Ctrl Pts',(7.55577912898259,-0.109879669117689,
-48.));
#23812=CARTESIAN_POINT('Ctrl Pts',(7.56430520033345,0.0905611110017474,
-48.));
#23813=CARTESIAN_POINT('Ctrl Pts',(7.56775652782499,0.171698923058889,-48.));
#23814=CARTESIAN_POINT('Ctrl Pts',(7.56991572882259,0.252944988440767,-48.));
#23815=CARTESIAN_POINT('Ctrl Pts',(7.57077853657819,0.334267836558012,-48.));
#23816=CARTESIAN_POINT('Ctrl Pts',(7.57111603563457,0.366078381055583,-48.));
#23817=CARTESIAN_POINT('Ctrl Pts',(7.57125515949273,0.397900673006978,-48.));
#23818=CARTESIAN_POINT('Ctrl Pts',(7.5711955934687,0.429732823440462,-48.));
#23819=CARTESIAN_POINT('Ctrl Pts',(7.57115223714762,0.45290249032953,-48.));
#23820=CARTESIAN_POINT('Ctrl Pts',(7.57100362858594,0.476067922578518,-48.));
#23821=CARTESIAN_POINT('Ctrl Pts',(7.57074992211655,0.499226939952169,-48.));
#23822=CARTESIAN_POINT('Ctrl Pts',(7.56852821147751,0.702030736842373,-48.));
#23823=CARTESIAN_POINT('Ctrl Pts',(7.55825105142857,0.904377024570949,-48.));
#23824=CARTESIAN_POINT('Ctrl Pts',(7.53999284572521,1.10576747908613,-48.));
#23825=CARTESIAN_POINT('Ctrl Pts',(7.52160273684829,1.30861284327355,-48.));
#23826=CARTESIAN_POINT('Ctrl Pts',(7.49511595853735,1.51048921493983,-48.));
#23827=CARTESIAN_POINT('Ctrl Pts',(7.46055733584223,1.71089962196904,-48.));
#23828=CARTESIAN_POINT('Ctrl Pts',(7.44239810129864,1.81620762623544,-48.));
#23829=CARTESIAN_POINT('Ctrl Pts',(7.42200928932642,1.92111100147053,-48.));
#23830=CARTESIAN_POINT('Ctrl Pts',(7.39938874174189,2.02553797493781,-48.));
#23831=CARTESIAN_POINT('Ctrl Pts',(7.35650614536241,2.22350399400051,-48.));
#23832=CARTESIAN_POINT('Ctrl Pts',(7.30560625006247,2.41975857637032,-48.));
#23833=CARTESIAN_POINT('Ctrl Pts',(7.2469351304453,2.61389361700967,-48.));
#23834=CARTESIAN_POINT('Ctrl Pts',(7.20801060017588,2.74268978307958,-48.));
#23835=CARTESIAN_POINT('Ctrl Pts',(7.16566449045406,2.8705529273773,-48.));
#23836=CARTESIAN_POINT('Ctrl Pts',(7.11995645101958,2.9973606630013,-48.));
#23837=CARTESIAN_POINT('Ctrl Pts',(7.09565931107824,3.06476817678271,-48.));
#23838=CARTESIAN_POINT('Ctrl Pts',(7.0704120324254,3.13187741049653,-48.));
#23839=CARTESIAN_POINT('Ctrl Pts',(7.04422251139379,3.19866954231277,-48.));
#23840=CARTESIAN_POINT('Ctrl Pts',(7.02727232497963,3.24189824756163,-48.));
#23841=CARTESIAN_POINT('Ctrl Pts',(7.00992743343007,3.28499411728753,-48.));
#23842=CARTESIAN_POINT('Ctrl Pts',(6.99218981795071,3.32795196703053,-48.));
#23843=CARTESIAN_POINT('Ctrl Pts',(6.98238546444813,3.35169664370825,-48.));
#23844=CARTESIAN_POINT('Ctrl Pts',(6.972464205672,3.37539162567257,-48.));
#23845=CARTESIAN_POINT('Ctrl Pts',(6.96242916936618,3.39903019071691,-48.));
#23846=CARTESIAN_POINT('Ctrl Pts',(6.88204014270503,3.58839485046199,-48.));
#23847=CARTESIAN_POINT('Ctrl Pts',(6.79430434720432,3.77425980468391,-48.));
#23848=CARTESIAN_POINT('Ctrl Pts',(6.6995390662541,3.95622432161017,-48.));
#23849=CARTESIAN_POINT('Ctrl Pts',(6.60408885004849,4.13950402392524,-48.));
#23850=CARTESIAN_POINT('Ctrl Pts',(6.50150693964798,4.31882734921869,-48.));
#23851=CARTESIAN_POINT('Ctrl Pts',(6.39206487423864,4.49377618287241,-48.));
#23852=CARTESIAN_POINT('Ctrl Pts',(6.28276639945468,4.66849547944328,-48.));
#23853=CARTESIAN_POINT('Ctrl Pts',(6.16662546550751,4.83885239762259,-48.));
#23854=CARTESIAN_POINT('Ctrl Pts',(6.04386422543394,5.00441223060582,-48.));
#23855=CARTESIAN_POINT('Ctrl Pts',(5.93619140677786,5.14962332380472,-48.));
#23856=CARTESIAN_POINT('Ctrl Pts',(5.82342482808063,5.2911440803551,-48.));
#23857=CARTESIAN_POINT('Ctrl Pts',(5.70568636114417,5.42866369628278,-48.));
#23858=CARTESIAN_POINT('Ctrl Pts',(5.59912526890868,5.55312803540967,-48.));
#23859=CARTESIAN_POINT('Ctrl Pts',(5.48849099337009,5.67431475663495,-48.));
#23860=CARTESIAN_POINT('Ctrl Pts',(5.3739712089178,5.79208620502323,-48.));
#23861=CARTESIAN_POINT('Ctrl Pts',(5.35469219530606,5.81191262512533,-48.));
#23862=CARTESIAN_POINT('Ctrl Pts',(5.3353030320026,5.8316422195084,-48.));
#23863=CARTESIAN_POINT('Ctrl Pts',(5.31580457648251,5.85127428800012,-48.));
#23864=CARTESIAN_POINT('Ctrl Pts',(5.29758402265168,5.86961969799404,-48.));
#23865=CARTESIAN_POINT('Ctrl Pts',(5.27927476383158,5.88787316488096,-48.));
#23866=CARTESIAN_POINT('Ctrl Pts',(5.26087839653079,5.90603362442133,-48.));
#23867=CARTESIAN_POINT('Ctrl Pts',(5.11313196865418,6.05188541036452,-48.));
#23868=CARTESIAN_POINT('Ctrl Pts',(4.9597563132659,6.19175476807782,-48.));
#23869=CARTESIAN_POINT('Ctrl Pts',(4.80120569678638,6.32542442409823,-48.));
#23870=CARTESIAN_POINT('Ctrl Pts',(4.64119263820284,6.46032702476013,-48.));
#23871=CARTESIAN_POINT('Ctrl Pts',(4.47590823781459,6.58891549829174,-48.));
#23872=CARTESIAN_POINT('Ctrl Pts',(4.30577791160318,6.71093376130789,-48.));
#23873=CARTESIAN_POINT('Ctrl Pts',(4.16782007827905,6.8098777624542,-48.));
#23874=CARTESIAN_POINT('Ctrl Pts',(4.02667489872999,6.90450099949382,-48.));
#23875=CARTESIAN_POINT('Ctrl Pts',(3.88255276675076,6.99464809660295,-48.));
#23876=CARTESIAN_POINT('Ctrl Pts',(3.84870261005292,7.01582106511995,-48.));
#23877=CARTESIAN_POINT('Ctrl Pts',(3.8146849955381,7.03674886278265,-48.));
#23878=CARTESIAN_POINT('Ctrl Pts',(3.78052548102958,7.05741572459137,-48.));
#23879=CARTESIAN_POINT('Ctrl Pts',(3.59938595616017,7.16700702243138,-48.));
#23880=CARTESIAN_POINT('Ctrl Pts',(3.41413884653443,7.26934117499804,-48.));
#23881=CARTESIAN_POINT('Ctrl Pts',(3.2252257455022,7.36416892349042,-48.));
#23882=CARTESIAN_POINT('Ctrl Pts',(3.03641084043487,7.45894738105373,-48.));
#23883=CARTESIAN_POINT('Ctrl Pts',(2.84393319138116,7.5462276669538,-48.));
#23884=CARTESIAN_POINT('Ctrl Pts',(2.6482016111633,7.62572029240467,-48.));
#23885=CARTESIAN_POINT('Ctrl Pts',(2.60498561173223,7.64327164131033,-48.));
#23886=CARTESIAN_POINT('Ctrl Pts',(2.5616108804781,7.66044317667659,-48.));
#23887=CARTESIAN_POINT('Ctrl Pts',(2.51808164906492,7.67723148270866,-48.));
#23888=CARTESIAN_POINT('Ctrl Pts',(2.38090159934801,7.73013893320513,-48.));
#23889=CARTESIAN_POINT('Ctrl Pts',(2.24218744160261,7.77924116547427,-48.));
#23890=CARTESIAN_POINT('Ctrl Pts',(2.10210202563547,7.82452631996428,-48.));
#23891=CARTESIAN_POINT('Ctrl Pts',(-7.26359129981488,-2.41004779799603E-5,
-36.5782382949161));
#23892=CARTESIAN_POINT('Ctrl Pts',(-7.26336357111336,1.16995354780479,-36.6167048152626));
#23893=CARTESIAN_POINT('Ctrl Pts',(-6.97516456706758,2.34003869460332,-36.6551713356092));
#23894=CARTESIAN_POINT('Ctrl Pts',(-6.43138563196355,3.37596502758674,-36.6936378559558));
#23895=CARTESIAN_POINT('Ctrl Pts',(-5.87641515309022,4.43321181663958,-36.7328960578448));
#23896=CARTESIAN_POINT('Ctrl Pts',(-5.05523627580577,5.35072070526111,-36.7721542597339));
#23897=CARTESIAN_POINT('Ctrl Pts',(-4.06576666907401,6.0190867334552,-36.8114124616229));
#23898=CARTESIAN_POINT('Ctrl Pts',(-3.07629706234226,6.68745276164928,-36.8506706635119));
#23899=CARTESIAN_POINT('Ctrl Pts',(-1.91853672616322,7.10667592941592,-36.889928865401));
#23900=CARTESIAN_POINT('Ctrl Pts',(-0.730537932789972,7.22676805626345,
-36.92918706729));
#23901=CARTESIAN_POINT('Ctrl Pts',(0.45746086058329,7.34686018311099,-36.9684452691791));
#23902=CARTESIAN_POINT('Ctrl Pts',(1.67569811115074,7.16782126903941,-37.0077034710681));
#23903=CARTESIAN_POINT('Ctrl Pts',(2.77891043352645,6.71099990026633,-37.0469616729572));
#23904=CARTESIAN_POINT('Ctrl Pts',(3.88212275590215,6.25417853149326,-37.0862198748462));
#23905=CARTESIAN_POINT('Ctrl Pts',(4.8703101500861,5.51957470801871,-37.1254780767352));
#23906=CARTESIAN_POINT('Ctrl Pts',(5.62564043785605,4.59478316401532,-37.1647362786243));
#23907=CARTESIAN_POINT('Ctrl Pts',(6.380970725626,3.66999162001192,-37.2039944805133));
#23908=CARTESIAN_POINT('Ctrl Pts',(6.90344390698194,2.55501235547971,-37.2432526824024));
#23909=CARTESIAN_POINT('Ctrl Pts',(7.13075993507001,1.38279623365648,-37.2825108842914));
#23910=CARTESIAN_POINT('Ctrl Pts',(7.35807596315808,0.210580111833238,-37.3217690861805));
#23911=CARTESIAN_POINT('Ctrl Pts',(7.29023483797825,-1.01887286728106,-37.3610272880695));
#23912=CARTESIAN_POINT('Ctrl Pts',(6.93532597438994,-2.15896186613015,-37.4002854899585));
#23913=CARTESIAN_POINT('Ctrl Pts',(6.58041711080162,-3.29905086497925,-37.4395436918476));
#23914=CARTESIAN_POINT('Ctrl Pts',(5.93844050880484,-4.34977588356314,-37.4788018937366));
#23915=CARTESIAN_POINT('Ctrl Pts',(5.08594590498163,-5.18584775403549,-37.5180600956257));
#23916=CARTESIAN_POINT('Ctrl Pts',(4.23345130115843,-6.02191962450782,-37.5573182975147));
#23917=CARTESIAN_POINT('Ctrl Pts',(3.17043869550879,-6.64333834686859,-37.5965764994038));
#23918=CARTESIAN_POINT('Ctrl Pts',(2.02366244242788,-6.97600552010563,-37.6358347012928));
#23919=CARTESIAN_POINT('Ctrl Pts',(0.876886189346959,-7.30867269334268,
-37.6750929031818));
#23920=CARTESIAN_POINT('Ctrl Pts',(-0.353653711165226,-7.35258831745601,
-37.7143511050709));
#23921=CARTESIAN_POINT('Ctrl Pts',(-1.52122683174925,-7.10251586508858,
-37.7536093069599));
#23922=CARTESIAN_POINT('Ctrl Pts',(-2.68879995233323,-6.85244341272115,
-37.792867508849));
#23923=CARTESIAN_POINT('Ctrl Pts',(-3.79340629298905,-6.30838288387294,
-37.832125710738));
#23924=CARTESIAN_POINT('Ctrl Pts',(-4.70333183225955,-5.53520843028317,
-37.871383912627));
#23925=CARTESIAN_POINT('Ctrl Pts',(-5.61325737153008,-4.76203397669338,
-37.9106421145161));
#23926=CARTESIAN_POINT('Ctrl Pts',(-6.32850210941532,-3.75974559836202,
-37.9499003164052));
#23927=CARTESIAN_POINT('Ctrl Pts',(-6.76377976984235,-2.64785685327351,
-37.9891585182942));
#23928=CARTESIAN_POINT('Ctrl Pts',(-7.09300555276655,-1.80687079791927,
-38.0188517771682));
#23929=CARTESIAN_POINT('Ctrl Pts',(-7.26206845007066,-0.903184830974666,
-38.0485450360421));
#23930=CARTESIAN_POINT('Ctrl Pts',(-7.26295522622064,0.000178426625192518,
-38.0782382949161));
#23931=CARTESIAN_POINT('Ctrl Pts',(-2.10185380438476,7.82409821225381,-48.));
#23932=CARTESIAN_POINT('Ctrl Pts',(-3.38848271769056,7.47846018434309,-47.960741798111));
#23933=CARTESIAN_POINT('Ctrl Pts',(-5.7867414247356,6.14069431107141,-47.8822253943329));
#23934=CARTESIAN_POINT('Ctrl Pts',(-8.00479568248447,2.66750428527037,-47.7644507886658));
#23935=CARTESIAN_POINT('Ctrl Pts',(-8.31350431498314,-1.4410774330594,-47.6466761829986));
#23936=CARTESIAN_POINT('Ctrl Pts',(-6.63976806498755,-5.20635630979624,
-47.5289015773315));
#23937=CARTESIAN_POINT('Ctrl Pts',(-3.38248655907778,-7.72983620180326,
-47.4111269716644));
#23938=CARTESIAN_POINT('Ctrl Pts',(0.681413555862794,-8.40998264592954,
-47.2933523659973));
#23939=CARTESIAN_POINT('Ctrl Pts',(4.58282963250162,-7.08446123670512,-47.1755777603301));
#23940=CARTESIAN_POINT('Ctrl Pts',(7.39131613068618,-4.06944919929777,-47.057803154663));
#23941=CARTESIAN_POINT('Ctrl Pts',(8.43711630815339,-0.0839387386951516,
-46.9400285489959));
#23942=CARTESIAN_POINT('Ctrl Pts',(7.47081891547249,3.92158434705153,-46.8222539433287));
#23943=CARTESIAN_POINT('Ctrl Pts',(4.72287152121607,6.99188514875576,-46.7044793376616));
#23944=CARTESIAN_POINT('Ctrl Pts',(0.848606621735488,8.39475027502305,-46.5867047319945));
#23945=CARTESIAN_POINT('Ctrl Pts',(-3.22803486495866,7.79562439652349,-46.4689301263274));
#23946=CARTESIAN_POINT('Ctrl Pts',(-6.53485028731455,5.33738695312811,-46.3511555206602));
#23947=CARTESIAN_POINT('Ctrl Pts',(-8.28322552855154,1.60628225714427,-46.2333809149931));
#23948=CARTESIAN_POINT('Ctrl Pts',(-8.05620575449563,-2.50789092127668,
-46.115606309326));
#23949=CARTESIAN_POINT('Ctrl Pts',(-5.90793090228909,-6.02397877694788,
-45.9978317036589));
#23950=CARTESIAN_POINT('Ctrl Pts',(-2.35072454748789,-8.10345988234339,
-45.8800570979917));
#23951=CARTESIAN_POINT('Ctrl Pts',(1.76708584413041,-8.25041668822644,-45.7622824923246));
#23952=CARTESIAN_POINT('Ctrl Pts',(5.46347916408095,-6.42980274600106,-45.6445078866575));
#23953=CARTESIAN_POINT('Ctrl Pts',(7.85693443764436,-3.07580057347912,-45.5267332809903));
#23954=CARTESIAN_POINT('Ctrl Pts',(8.37665714814605,1.01172276152054,-45.4089586753233));
#23955=CARTESIAN_POINT('Ctrl Pts',(6.89870310741494,4.85796905729832,-45.291184069656));
#23956=CARTESIAN_POINT('Ctrl Pts',(3.77553683341622,7.54568019093911,-45.173409463989));
#23957=CARTESIAN_POINT('Ctrl Pts',(-0.248024672543488,8.4338871042367,-45.0556348583218));
#23958=CARTESIAN_POINT('Ctrl Pts',(-4.21243691249803,7.31076898712496,-44.9378602526548));
#23959=CARTESIAN_POINT('Ctrl Pts',(-7.17226138689772,4.44416859749758,-44.8200856469875));
#23960=CARTESIAN_POINT('Ctrl Pts',(-8.4216350723183,0.517716750424533,-44.7023110413205));
#23961=CARTESIAN_POINT('Ctrl Pts',(-7.66260560886039,-3.5322009014224,-44.5845364356533));
#23962=CARTESIAN_POINT('Ctrl Pts',(-5.0761873899821,-6.73975440997329,-44.4667618299862));
#23963=CARTESIAN_POINT('Ctrl Pts',(-1.27919300023199,-8.3400019899946,-44.3489872243191));
#23964=CARTESIAN_POINT('Ctrl Pts',(2.82286510073567,-7.95131439121922,-44.2312126186519));
#23965=CARTESIAN_POINT('Ctrl Pts',(6.25172243861154,-5.66638636835865,-44.1134380129848));
#23966=CARTESIAN_POINT('Ctrl Pts',(8.18966038568263,-2.03013070814185,-43.9956634073177));
#23967=CARTESIAN_POINT('Ctrl Pts',(8.17451682713419,2.09027332372109,-43.8778888016505));
#23968=CARTESIAN_POINT('Ctrl Pts',(6.20990321969786,5.71218609001371,-43.7601141959834));
#23969=CARTESIAN_POINT('Ctrl Pts',(2.76434332646893,7.97184883815334,-43.6423395903163));
#23970=CARTESIAN_POINT('Ctrl Pts',(-1.34046097639977,8.33037407897806,-43.5245649846492));
#23971=CARTESIAN_POINT('Ctrl Pts',(-5.12559029658075,6.70226021850519,-43.406790378982));
#23972=CARTESIAN_POINT('Ctrl Pts',(-7.68836177257858,3.47578209600548,-43.2890157733149));
#23973=CARTESIAN_POINT('Ctrl Pts',(-8.41760212770272,-0.579605335253821,
-43.1712411676478));
#23974=CARTESIAN_POINT('Ctrl Pts',(-7.1394011161468,-4.49676768665247,-43.0534665619807));
#23975=CARTESIAN_POINT('Ctrl Pts',(-4.15858587830098,-7.34153467728348,
-42.9356919563136));
#23976=CARTESIAN_POINT('Ctrl Pts',(-0.186025343832157,-8.43548235114104,
-42.8179173506464));
#23977=CARTESIAN_POINT('Ctrl Pts',(3.83089877123767,-7.51772455796898,-42.7001427449793));
#23978=CARTESIAN_POINT('Ctrl Pts',(6.93422486298953,-4.80712944224074,-42.5823681393122));
#23979=CARTESIAN_POINT('Ctrl Pts',(8.38386744432517,-0.950123466158245,
-42.464593533645));
#23980=CARTESIAN_POINT('Ctrl Pts',(7.83411375280636,3.13346926473683,-42.3468189279779));
#23981=CARTESIAN_POINT('Ctrl Pts',(5.41606980711838,6.46978792306059,-42.2290443223107));
#23982=CARTESIAN_POINT('Ctrl Pts',(1.70639406288594,8.2631826330481,-42.1112697166436));
#23983=CARTESIAN_POINT('Ctrl Pts',(-2.4102248912686,8.08596215044749,-41.9934951109765));
#23984=CARTESIAN_POINT('Ctrl Pts',(-5.95205008868199,5.98039026040782,-41.8757205053094));
#23985=CARTESIAN_POINT('Ctrl Pts',(-8.07442217067084,2.44860665169793,-41.7579458996422));
#23986=CARTESIAN_POINT('Ctrl Pts',(-8.27119491551605,-1.66712404892423,
-41.6401712939752));
#23987=CARTESIAN_POINT('Ctrl Pts',(-6.49544168759803,-5.38527670672303,
-41.522396688308));
#23988=CARTESIAN_POINT('Ctrl Pts',(-3.17064656618999,-7.81914114703574,
-41.4046220826409));
#23989=CARTESIAN_POINT('Ctrl Pts',(0.910288721922364,-8.38828602085676,
-41.2868474769737));
#23990=CARTESIAN_POINT('Ctrl Pts',(4.77413709997572,-6.95698087359707,-41.1690728713066));
#23991=CARTESIAN_POINT('Ctrl Pts',(7.4994426769679,-3.86656533112174,-41.0512982656395));
#23992=CARTESIAN_POINT('Ctrl Pts',(8.43627081960314,0.145954045071271,-40.9335236599723));
#23993=CARTESIAN_POINT('Ctrl Pts',(7.36120546016224,4.12366609926623,-40.8157490543053));
#23994=CARTESIAN_POINT('Ctrl Pts',(4.53062966851309,7.11796057391082,-40.6979744486381));
#23995=CARTESIAN_POINT('Ctrl Pts',(0.619583063952851,8.41475399235312,-40.5801998429711));
#23996=CARTESIAN_POINT('Ctrl Pts',(-3.43922256435361,7.70478527136227,-40.4624252373038));
#23997=CARTESIAN_POINT('Ctrl Pts',(-6.67783765143915,5.15736873085314,-40.3446506316368));
#23998=CARTESIAN_POINT('Ctrl Pts',(-8.32391280398028,1.38001578132032,-40.2268760259696));
#23999=CARTESIAN_POINT('Ctrl Pts',(-7.98488974899803,-2.72644523533966,
-40.1091014203025));
#24000=CARTESIAN_POINT('Ctrl Pts',(-5.74161917229395,-6.18269983140913,
-39.9913268146354));
#24001=CARTESIAN_POINT('Ctrl Pts',(-2.12907933537458,-8.16449564324956,
-39.8735522089682));
#24002=CARTESIAN_POINT('Ctrl Pts',(1.9912062783033,-8.19921127195815,-39.7557776033011));
#24003=CARTESIAN_POINT('Ctrl Pts',(5.63662627205554,-6.27856768651366,-39.638002997634));
#24004=CARTESIAN_POINT('Ctrl Pts',(7.93781585726883,-2.86060261851435,-39.5202283919668));
#24005=CARTESIAN_POINT('Ctrl Pts',(8.3459841673938,1.23956290787192,-39.4024537862997));
#24006=CARTESIAN_POINT('Ctrl Pts',(6.76379066080322,5.0441157621324,-39.2846791806326));
#24007=CARTESIAN_POINT('Ctrl Pts',(3.56855902743119,7.64574093157071,-39.1669045749655));
#24008=CARTESIAN_POINT('Ctrl Pts',(-0.477707485283489,8.42399925709112,
-39.0491299692983));
#24009=CARTESIAN_POINT('Ctrl Pts',(-4.4100496579569,7.19329061968874,-38.9313553636312));
#24010=CARTESIAN_POINT('Ctrl Pts',(-7.29067710496446,4.24711611286043,-38.8135807579641));
#24011=CARTESIAN_POINT('Ctrl Pts',(-8.43261381919959,0.288083496944457,
-38.695806152297));
#24012=CARTESIAN_POINT('Ctrl Pts',(-7.56352915785683,-3.73965166868971,
-38.5780315466298));
#24013=CARTESIAN_POINT('Ctrl Pts',(-4.89068362979871,-6.87554954592136,
-38.4602569409627));
#24014=CARTESIAN_POINT('Ctrl Pts',(-1.05150112347229,-8.3717568832205,-38.3424823352955));
#24015=CARTESIAN_POINT('Ctrl Pts',(3.03844482120267,-7.87145609112005,-38.2247077296284));
#24016=CARTESIAN_POINT('Ctrl Pts',(6.40377825371979,-5.49395959222041,-38.1069331239613));
#24017=CARTESIAN_POINT('Ctrl Pts',(8.24192981481277,-1.80625603195024,-37.9891585182942));
#24018=CARTESIAN_POINT('Ctrl Pts',(8.11453458490175,2.31220595952502,-37.871383912627));
#24019=CARTESIAN_POINT('Ctrl Pts',(6.05197395361438,5.87924988197173,-37.7536093069599));
#24020=CARTESIAN_POINT('Ctrl Pts',(2.54613022648071,8.0442021874585,-37.6358347012928));
#24021=CARTESIAN_POINT('Ctrl Pts',(-1.56691815067151,8.29076204944015,-37.5180600956257));
#24022=CARTESIAN_POINT('Ctrl Pts',(-5.30628572285852,6.56012956115795,-37.4002854899586));
#24023=CARTESIAN_POINT('Ctrl Pts',(-7.78020296240809,3.26502828627881,-37.2825108842914));
#24024=CARTESIAN_POINT('Ctrl Pts',(-8.39868665514552,-0.808721357278217,
-37.1647362786243));
#24025=CARTESIAN_POINT('Ctrl Pts',(-7.01423999417884,-4.68960618017365,
-37.0469616729571));
#24026=CARTESIAN_POINT('Ctrl Pts',(-3.95702765317846,-7.45210691888099,
-36.92918706729));
#24027=CARTESIAN_POINT('Ctrl Pts',(0.0438619977836959,-8.43741959751058,
-36.8114124616229));
#24028=CARTESIAN_POINT('Ctrl Pts',(4.03429158844322,-7.41056343594989,-36.6936378559558));
#24029=CARTESIAN_POINT('Ctrl Pts',(7.06261733076329,-4.61642867900756,-36.5758632502887));
#24030=CARTESIAN_POINT('Ctrl Pts',(8.40664121397815,-0.721355965422936,
-36.4580886446215));
#24031=CARTESIAN_POINT('Ctrl Pts',(7.74583594905282,3.34573518158168,-36.3403140389544));
#24032=CARTESIAN_POINT('Ctrl Pts',(5.23779660784082,6.61495421252791,-36.2225394332873));
#24033=CARTESIAN_POINT('Ctrl Pts',(1.48063306394132,8.30658225499598,-36.1047648276201));
#24034=CARTESIAN_POINT('Ctrl Pts',(-2.62961918038579,8.01734176317378,-35.986990221953));
#24035=CARTESIAN_POINT('Ctrl Pts',(-6.11278614011418,5.81591813633449,-35.8692156162859));
#24036=CARTESIAN_POINT('Ctrl Pts',(-8.1381056994787,2.22790678763051,-35.7514410106188));
#24037=CARTESIAN_POINT('Ctrl Pts',(-8.2227680260995,-1.89224441543144,-35.6336664049516));
#24038=CARTESIAN_POINT('Ctrl Pts',(-6.97149994399699,-4.33674652103884,
-35.5551500011735));
#24039=CARTESIAN_POINT('Ctrl Pts',(-6.09356451288676,-5.33879890774012,
-35.5158917992845));
#24040=CARTESIAN_POINT('Ctrl Pts',(-2.02934030215363,7.55416851400967,-48.1613694002385));
#24041=CARTESIAN_POINT('Ctrl Pts',(-3.27158079587429,7.22045492340081,-48.1221111983495));
#24042=CARTESIAN_POINT('Ctrl Pts',(-5.58710009557265,5.92884168378703,-48.0435947945714));
#24043=CARTESIAN_POINT('Ctrl Pts',(-7.72863196054971,2.5754759636345,-47.9258201889042));
#24044=CARTESIAN_POINT('Ctrl Pts',(-8.02669021191114,-1.3913605729051,-47.8080455832372));
#24045=CARTESIAN_POINT('Ctrl Pts',(-6.41069750099766,-5.02673814173007,
-47.69027097757));
#24046=CARTESIAN_POINT('Ctrl Pts',(-3.26579150343843,-7.46315852255819,
-47.5724963719029));
#24047=CARTESIAN_POINT('Ctrl Pts',(0.657904935377249,-8.11984006128011,
-47.4547217662357));
#24048=CARTESIAN_POINT('Ctrl Pts',(4.42472300011451,-6.84004885434888,-47.3369471605686));
#24049=CARTESIAN_POINT('Ctrl Pts',(7.13631732077113,-3.9290540809612,-47.2191725549015));
#24050=CARTESIAN_POINT('Ctrl Pts',(8.14603761801837,-0.0810428703417254,
-47.1013979492344));
#24051=CARTESIAN_POINT('Ctrl Pts',(7.21307727665566,3.78629053417727,-46.9836233435672));
#24052=CARTESIAN_POINT('Ctrl Pts',(4.55993347391867,6.75066662143647,-46.8658487379002));
#24053=CARTESIAN_POINT('Ctrl Pts',(0.819329876592602,8.10513320387957,-46.748074132233));
#24054=CARTESIAN_POINT('Ctrl Pts',(-3.11666835940339,7.52667703877142,-46.6302995265659));
#24055=CARTESIAN_POINT('Ctrl Pts',(-6.30939936399117,5.15324825617085,-46.5125249208987));
#24056=CARTESIAN_POINT('Ctrl Pts',(-7.99745603707093,1.55086586624483,-46.3947503152316));
#24057=CARTESIAN_POINT('Ctrl Pts',(-7.77826839618155,-2.4213692262206,-46.2769757095645));
#24058=CARTESIAN_POINT('Ctrl Pts',(-5.70410856232861,-5.8161528103791,-46.1592011038973));
#24059=CARTESIAN_POINT('Ctrl Pts',(-2.26962505837811,-7.8238922668259,-46.0414264982302));
#24060=CARTESIAN_POINT('Ctrl Pts',(1.70612176421503,-7.96577909465003,-45.9236518925631));
#24061=CARTESIAN_POINT('Ctrl Pts',(5.27499031308291,-6.20797594016174,-45.8058772868959));
#24062=CARTESIAN_POINT('Ctrl Pts',(7.58587189671717,-2.96968611809587,-45.6881026812289));
#24063=CARTESIAN_POINT('Ctrl Pts',(8.08766428597154,0.97681854478969,-45.5703280755617));
#24064=CARTESIAN_POINT('Ctrl Pts',(6.66069934039371,4.69037017418842,-45.4525534698946));
#24065=CARTESIAN_POINT('Ctrl Pts',(3.64528162821473,7.28535585428942,-45.3347788642275));
#24066=CARTESIAN_POINT('Ctrl Pts',(-0.239467874916397,8.14291982093926,
-45.2170042585603));
#24067=CARTESIAN_POINT('Ctrl Pts',(-4.06710874894274,7.05854903626383,-45.0992296528932));
#24068=CARTESIAN_POINT('Ctrl Pts',(-6.92481991832549,4.29084574086602,-44.9814550472261));
#24069=CARTESIAN_POINT('Ctrl Pts',(-8.1310904814755,0.499855634366561,-44.863680441559));
#24070=CARTESIAN_POINT('Ctrl Pts',(-7.3982473705494,-3.41034073331186,-44.7459058358918));
#24071=CARTESIAN_POINT('Ctrl Pts',(-4.90106002153181,-6.50723433867939,
-44.6281312302247));
#24072=CARTESIAN_POINT('Ctrl Pts',(-1.23506111804168,-8.05227372285845,
-44.5103566245576));
#24073=CARTESIAN_POINT('Ctrl Pts',(2.72547686452563,-7.67699576228066,-44.3925820188904));
#24074=CARTESIAN_POINT('Ctrl Pts',(6.03603936491014,-5.47089726264288,-44.2748074132233));
#24075=CARTESIAN_POINT('Ctrl Pts',(7.90711887142005,-1.96009163723823,-44.1570328075562));
#24076=CARTESIAN_POINT('Ctrl Pts',(7.89249776237038,2.01815934557136,-44.0392582018891));
#24077=CARTESIAN_POINT('Ctrl Pts',(5.99566290001563,5.51511690379401,-43.9214835962219));
#24078=CARTESIAN_POINT('Ctrl Pts',(2.66897407882984,7.69682177523119,-43.8037089905548));
#24079=CARTESIAN_POINT('Ctrl Pts',(-1.29421536226612,8.04297797269226,-43.6859343848877));
#24080=CARTESIAN_POINT('Ctrl Pts',(-4.9487585385243,6.47103368871784,-43.5681597792205));
#24081=CARTESIAN_POINT('Ctrl Pts',(-7.42311495218289,3.35586836449482,-43.4503851735534));
#24082=CARTESIAN_POINT('Ctrl Pts',(-8.127196672578,-0.559609076387755,-43.3326105678863));
#24083=CARTESIAN_POINT('Ctrl Pts',(-6.89309331981735,-4.34163017280696,
-43.2148359622192));
#24084=CARTESIAN_POINT('Ctrl Pts',(-4.01511556379315,-7.08825331675756,
-43.097061356552));
#24085=CARTESIAN_POINT('Ctrl Pts',(-0.179607509653168,-8.14446003217,-42.9792867508849));
#24086=CARTESIAN_POINT('Ctrl Pts',(3.69873359114005,-7.25836468461807,-42.8615121452178));
#24087=CARTESIAN_POINT('Ctrl Pts',(6.69499560307401,-4.64128451486849,-42.7437375395506));
#24088=CARTESIAN_POINT('Ctrl Pts',(8.09462582848997,-0.917344411811364,
-42.6259629338836));
#24089=CARTESIAN_POINT('Ctrl Pts',(7.5638385205766,3.02536525196216,-42.5081883282164));
#24090=CARTESIAN_POINT('Ctrl Pts',(5.22921656869468,6.24658163724989,-42.3904137225493));
#24091=CARTESIAN_POINT('Ctrl Pts',(1.6475238363135,7.9781046171329,-42.2726391168821));
#24092=CARTESIAN_POINT('Ctrl Pts',(-2.32707265315102,7.80699820290073,-42.1548645112151));
#24093=CARTESIAN_POINT('Ctrl Pts',(-5.74670564632112,5.77406808824415,-42.0370899055479));
#24094=CARTESIAN_POINT('Ctrl Pts',(-7.79585634993363,2.36413025113635,-41.9193152998808));
#24095=CARTESIAN_POINT('Ctrl Pts',(-7.98584047758644,-1.60960862935077,
-41.8015406942137));
#24096=CARTESIAN_POINT('Ctrl Pts',(-6.27135035245223,-5.19948582361138,
-41.6837660885465));
#24097=CARTESIAN_POINT('Ctrl Pts',(-3.06125994454584,-7.54938246647084,
-41.5659914828794));
#24098=CARTESIAN_POINT('Ctrl Pts',(0.878883957646947,-8.09889196508568,
-41.4482168772122));
#24099=CARTESIAN_POINT('Ctrl Pts',(4.60943040128496,-6.7169665362311,-41.3304422715451));
#24100=CARTESIAN_POINT('Ctrl Pts',(7.24071352456248,-3.73316966241243,-41.212667665878));
#24101=CARTESIAN_POINT('Ctrl Pts',(8.14522129864046,0.140918662043758,-41.0948930602109));
#24102=CARTESIAN_POINT('Ctrl Pts',(7.10724546187608,3.9814005095921,-40.9771184545438));
#24103=CARTESIAN_POINT('Ctrl Pts',(4.3743239236079,6.87239247165716,-40.8593438488766));
#24104=CARTESIAN_POINT('Ctrl Pts',(0.598207582082232,8.12444679728274,-40.7415692432096));
#24105=CARTESIAN_POINT('Ctrl Pts',(-3.32057012878775,7.43897184380617,-40.6237946375423));
#24106=CARTESIAN_POINT('Ctrl Pts',(-6.44745369494008,4.97944062367873,-40.5060200318753));
#24107=CARTESIAN_POINT('Ctrl Pts',(-8.03673961028621,1.33240553496112,-40.3882454262081));
#24108=CARTESIAN_POINT('Ctrl Pts',(-7.70941277746869,-2.63238346365819,
-40.270470820541));
#24109=CARTESIAN_POINT('Ctrl Pts',(-5.54353455109341,-5.96939802274668,
-40.1526962148739));
#24110=CARTESIAN_POINT('Ctrl Pts',(-2.05562655820527,-7.8828223071651,-40.0349216092067));
#24111=CARTESIAN_POINT('Ctrl Pts',(1.92251009182108,-7.91634025418214,-39.9171470035396));
#24112=CARTESIAN_POINT('Ctrl Pts',(5.44216388323377,-6.06195845755845,-39.7993723978724));
#24113=CARTESIAN_POINT('Ctrl Pts',(7.66396292483574,-2.76191244609261,-39.6815977922053));
#24114=CARTESIAN_POINT('Ctrl Pts',(8.05804951642959,1.19679825530756,-39.5638231865382));
#24115=CARTESIAN_POINT('Ctrl Pts',(6.53044134404774,4.87009485791515,-39.4460485808711));
#24116=CARTESIAN_POINT('Ctrl Pts',(3.44544451182704,7.38196452098329,-39.328273975204));
#24117=CARTESIAN_POINT('Ctrl Pts',(-0.461226680230507,8.13337310238434,
-39.2104993695368));
#24118=CARTESIAN_POINT('Ctrl Pts',(-4.25790389736948,6.94512364712774,-39.0927247638697));
#24119=CARTESIAN_POINT('Ctrl Pts',(-7.03915031969784,4.10059152438366,-38.9749501582026));
#24120=CARTESIAN_POINT('Ctrl Pts',(-8.1416904639609,0.278144678528614,-38.8571755525354));
#24121=CARTESIAN_POINT('Ctrl Pts',(-7.30258903570402,-3.61063449391976,
-38.7394009468683));
#24122=CARTESIAN_POINT('Ctrl Pts',(-4.7219561010042,-6.63834457177027,-38.6216263412012));
#24123=CARTESIAN_POINT('Ctrl Pts',(-1.01522456184661,-8.08293307912742,
-38.5038517355341));
#24124=CARTESIAN_POINT('Ctrl Pts',(2.93361913120376,-7.59989255628477,-38.3860771298669));
#24125=CARTESIAN_POINT('Ctrl Pts',(6.18284928724263,-5.30441917303561,-38.2683025241998));
#24126=CARTESIAN_POINT('Ctrl Pts',(7.95758501653589,-1.74394058901621,-38.1505279185327));
#24127=CARTESIAN_POINT('Ctrl Pts',(7.83458489453823,2.23243535337958,-38.0327533128655));
#24128=CARTESIAN_POINT('Ctrl Pts',(5.84318215949784,5.67641703101683,-37.9149787071985));
#24129=CARTESIAN_POINT('Ctrl Pts',(2.45828928365514,7.76667894961431,-37.7972041015313));
#24130=CARTESIAN_POINT('Ctrl Pts',(-1.51285981294236,8.00473254961685,-37.6794294958642));
#24131=CARTESIAN_POINT('Ctrl Pts',(-5.12322001162739,6.33380650834752,-37.561654890197));
#24132=CARTESIAN_POINT('Ctrl Pts',(-7.51178764080184,3.15238551567893,-37.4438802845299));
#24133=CARTESIAN_POINT('Ctrl Pts',(-8.1089337797381,-0.780820645143519,
-37.3261056788628));
#24134=CARTESIAN_POINT('Ctrl Pts',(-6.77225022952131,-4.52781577995659,
-37.2083310731957));
#24135=CARTESIAN_POINT('Ctrl Pts',(-3.82051105389889,-7.1950108399046,-37.0905564675286));
#24136=CARTESIAN_POINT('Ctrl Pts',(0.0423487683347632,-8.14633044395825,
-36.9727818618614));
#24137=CARTESIAN_POINT('Ctrl Pts',(3.89510940008676,-7.15490059816084,-36.8550072561943));
#24138=CARTESIAN_POINT('Ctrl Pts',(6.81895855844356,-4.4571628867737,-36.7372326505271));
#24139=CARTESIAN_POINT('Ctrl Pts',(8.11661390800927,-0.6964693404355,-36.61945804486));
#24140=CARTESIAN_POINT('Ctrl Pts',(7.47860628198373,3.23030804052729,-36.5016834391929));
#24141=CARTESIAN_POINT('Ctrl Pts',(5.05709375628351,6.38673972108787,-36.3839088335257));
#24142=CARTESIAN_POINT('Ctrl Pts',(1.42955154306598,8.0200069614983,-36.2661342278587));
#24143=CARTESIAN_POINT('Ctrl Pts',(-2.53889788668489,7.74074520416533,-36.1483596221915));
#24144=CARTESIAN_POINT('Ctrl Pts',(-5.90189633869939,5.61527021692382,-36.0305850165244));
#24145=CARTESIAN_POINT('Ctrl Pts',(-7.85734281075386,2.15104448470603,-35.9128104108573));
#24146=CARTESIAN_POINT('Ctrl Pts',(-7.9390843053941,-1.8269623918416,-35.7950358051901));
#24147=CARTESIAN_POINT('Ctrl Pts',(-6.73098470183848,-4.18712970284093,
-35.716519401412));
#24148=CARTESIAN_POINT('Ctrl Pts',(-5.88333785345927,-5.15461149865373,
-35.677261199523));
#24149=CARTESIAN_POINT('Ctrl Pts',(-1.95682679992249,7.28423881576552,-48.322738800477));
#24150=CARTESIAN_POINT('Ctrl Pts',(-3.15467887405802,6.96244966245853,-48.283480598588));
#24151=CARTESIAN_POINT('Ctrl Pts',(-5.38745876640971,5.71698905650265,-48.2049641948099));
#24152=CARTESIAN_POINT('Ctrl Pts',(-7.45246823861496,2.48344764199862,-48.0871895891427));
#24153=CARTESIAN_POINT('Ctrl Pts',(-7.73987610883915,-1.34164371275079,
-47.9694149834756));
#24154=CARTESIAN_POINT('Ctrl Pts',(-6.18162693700778,-4.84711997366391,
-47.8516403778085));
#24155=CARTESIAN_POINT('Ctrl Pts',(-3.14909644779907,-7.19648084331311,
-47.7338657721414));
#24156=CARTESIAN_POINT('Ctrl Pts',(0.634396314891706,-7.82969747663068,
-47.6160911664742));
#24157=CARTESIAN_POINT('Ctrl Pts',(4.26661636772739,-6.59563647199265,-47.4983165608071));
#24158=CARTESIAN_POINT('Ctrl Pts',(6.88131851085609,-3.78865896262463,-47.38054195514));
#24159=CARTESIAN_POINT('Ctrl Pts',(7.85495892788334,-0.0781470019882984,
-47.2627673494728));
#24160=CARTESIAN_POINT('Ctrl Pts',(6.95533563783883,3.65099672130299,-47.1449927438058));
#24161=CARTESIAN_POINT('Ctrl Pts',(4.39699542662127,6.50944809411718,-47.0272181381386));
#24162=CARTESIAN_POINT('Ctrl Pts',(0.790053131449719,7.81551613273609,-46.9094435324715));
#24163=CARTESIAN_POINT('Ctrl Pts',(-3.00530185384814,7.25772968101937,-46.7916689268043));
#24164=CARTESIAN_POINT('Ctrl Pts',(-6.08394844066777,4.96910955921358,-46.6738943211372));
#24165=CARTESIAN_POINT('Ctrl Pts',(-7.71168654559033,1.49544947534539,-46.5561197154701));
#24166=CARTESIAN_POINT('Ctrl Pts',(-7.50033103786747,-2.33484753116452,
-46.438345109803));
#24167=CARTESIAN_POINT('Ctrl Pts',(-5.50028622236814,-5.60832684381034,
-46.3205705041358));
#24168=CARTESIAN_POINT('Ctrl Pts',(-2.18852556926833,-7.5443246513084,-46.2027958984687));
#24169=CARTESIAN_POINT('Ctrl Pts',(1.64515768429965,-7.68114150107363,-46.0850212928016));
#24170=CARTESIAN_POINT('Ctrl Pts',(5.08650146208487,-5.98614913432241,-45.9672466871344));
#24171=CARTESIAN_POINT('Ctrl Pts',(7.31480935578999,-2.86357166271262,-45.8494720814674));
#24172=CARTESIAN_POINT('Ctrl Pts',(7.79867142379702,0.941914328058838,-45.7316974758002));
#24173=CARTESIAN_POINT('Ctrl Pts',(6.42269557337249,4.52277129107851,-45.6139228701331));
#24174=CARTESIAN_POINT('Ctrl Pts',(3.51502642301324,7.02503151763973,-45.4961482644659));
#24175=CARTESIAN_POINT('Ctrl Pts',(-0.230911077289297,7.85195253764182,
-45.3783736587988));
#24176=CARTESIAN_POINT('Ctrl Pts',(-3.92178058538745,6.80632908540271,-45.2605990531317));
#24177=CARTESIAN_POINT('Ctrl Pts',(-6.67737844975326,4.13752288423446,-45.1428244474646));
#24178=CARTESIAN_POINT('Ctrl Pts',(-7.8405458906327,0.481994518308594,-45.0250498417974));
#24179=CARTESIAN_POINT('Ctrl Pts',(-7.13388913223841,-3.28848056520132,
-44.9072752361303));
#24180=CARTESIAN_POINT('Ctrl Pts',(-4.72593265308153,-6.27471426738548,
-44.7895006304632));
#24181=CARTESIAN_POINT('Ctrl Pts',(-1.19092923585136,-7.7645454557223,-44.6717260247961));
#24182=CARTESIAN_POINT('Ctrl Pts',(2.62808862831559,-7.4026771333421,-44.5539514191289));
#24183=CARTESIAN_POINT('Ctrl Pts',(5.82035629120873,-5.27540815692712,-44.4361768134618));
#24184=CARTESIAN_POINT('Ctrl Pts',(7.62457735715747,-1.89005256633461,-44.3184022077947));
#24185=CARTESIAN_POINT('Ctrl Pts',(7.61047869760657,1.94604536742163,-44.2006276021275));
#24186=CARTESIAN_POINT('Ctrl Pts',(5.78142258033341,5.31804771757433,-44.0828529964604));
#24187=CARTESIAN_POINT('Ctrl Pts',(2.57360483119075,7.42179471230903,-43.9650783907933));
#24188=CARTESIAN_POINT('Ctrl Pts',(-1.24796974813247,7.75558186640647,-43.8473037851262));
#24189=CARTESIAN_POINT('Ctrl Pts',(-4.77192678046785,6.23980715893049,-43.729529179459));
#24190=CARTESIAN_POINT('Ctrl Pts',(-7.15786813178719,3.23595463298417,-43.6117545737919));
#24191=CARTESIAN_POINT('Ctrl Pts',(-7.83679121745328,-0.539612817521684,
-43.4939799681248));
#24192=CARTESIAN_POINT('Ctrl Pts',(-6.6467855234879,-4.18649265896147,-43.3762053624577));
#24193=CARTESIAN_POINT('Ctrl Pts',(-3.87164524928533,-6.83497195623163,
-43.2584307567905));
#24194=CARTESIAN_POINT('Ctrl Pts',(-0.173189675474176,-7.85343771319897,
-43.1406561511234));
#24195=CARTESIAN_POINT('Ctrl Pts',(3.56656841104242,-6.99900481126716,-43.0228815454563));
#24196=CARTESIAN_POINT('Ctrl Pts',(6.45576634315849,-4.47543958749625,-42.9051069397891));
#24197=CARTESIAN_POINT('Ctrl Pts',(7.80538421265478,-0.884565357464481,
-42.787332334122));
#24198=CARTESIAN_POINT('Ctrl Pts',(7.29356328834684,2.9172612391875,-42.6695577284549));
#24199=CARTESIAN_POINT('Ctrl Pts',(5.04236333027098,6.02337535143919,-42.5517831227878));
#24200=CARTESIAN_POINT('Ctrl Pts',(1.58865360974106,7.6930266012177,-42.4340085171206));
#24201=CARTESIAN_POINT('Ctrl Pts',(-2.24392041503344,7.52803425535397,-42.3162339114536));
#24202=CARTESIAN_POINT('Ctrl Pts',(-5.54136120396024,5.56774591608048,-42.1984593057864));
#24203=CARTESIAN_POINT('Ctrl Pts',(-7.51729052919641,2.27965385057478,-42.0806847001193));
#24204=CARTESIAN_POINT('Ctrl Pts',(-7.70048603965684,-1.55209320977732,
-41.9629100944521));
#24205=CARTESIAN_POINT('Ctrl Pts',(-6.04725901730644,-5.01369494049972,
-41.845135488785));
#24206=CARTESIAN_POINT('Ctrl Pts',(-2.95187332290169,-7.27962378590596,
-41.7273608831179));
#24207=CARTESIAN_POINT('Ctrl Pts',(0.84747919337153,-7.80949790931459,-41.6095862774508));
#24208=CARTESIAN_POINT('Ctrl Pts',(4.4447237025942,-6.47695219886514,-41.4918116717836));
#24209=CARTESIAN_POINT('Ctrl Pts',(6.98198437215706,-3.59977399370311,-41.3740370661165));
#24210=CARTESIAN_POINT('Ctrl Pts',(7.85417177767779,0.135883279016239,-41.2562624604493));
#24211=CARTESIAN_POINT('Ctrl Pts',(6.85328546358993,3.83913491991798,-41.1384878547823));
#24212=CARTESIAN_POINT('Ctrl Pts',(4.2180181787027,6.62682436940348,-41.0207132491151));
#24213=CARTESIAN_POINT('Ctrl Pts',(0.576832100211618,7.83413960221236,-40.902938643448));
#24214=CARTESIAN_POINT('Ctrl Pts',(-3.20191769322189,7.17315841625007,-40.7851640377808));
#24215=CARTESIAN_POINT('Ctrl Pts',(-6.21706973844099,4.80151251650432,-40.6673894321137));
#24216=CARTESIAN_POINT('Ctrl Pts',(-7.74956641659215,1.28479528860193,-40.5496148264466));
#24217=CARTESIAN_POINT('Ctrl Pts',(-7.43393580593934,-2.53832169197672,
-40.4318402207795));
#24218=CARTESIAN_POINT('Ctrl Pts',(-5.34544992989288,-5.75609621408423,
-40.3140656151123));
#24219=CARTESIAN_POINT('Ctrl Pts',(-1.98217378103596,-7.60114897108064,
-40.1962910094452));
#24220=CARTESIAN_POINT('Ctrl Pts',(1.85381390533885,-7.63346923640613,-40.0785164037781));
#24221=CARTESIAN_POINT('Ctrl Pts',(5.247701494412,-5.84534922860326,-39.960741798111));
#24222=CARTESIAN_POINT('Ctrl Pts',(7.39010999240267,-2.66322227367086,-39.8429671924438));
#24223=CARTESIAN_POINT('Ctrl Pts',(7.77011486546537,1.1540336027432,-39.7251925867767));
#24224=CARTESIAN_POINT('Ctrl Pts',(6.29709202729227,4.6960739536979,-39.6074179811096));
#24225=CARTESIAN_POINT('Ctrl Pts',(3.32232999622289,7.11818811039587,-39.4896433754424));
#24226=CARTESIAN_POINT('Ctrl Pts',(-0.44474587517752,7.84274694767756,-39.3718687697753));
#24227=CARTESIAN_POINT('Ctrl Pts',(-4.10575813678208,6.69695667456673,-39.2540941641082));
#24228=CARTESIAN_POINT('Ctrl Pts',(-6.7876235344312,3.9540669359069,-39.1363195584411));
#24229=CARTESIAN_POINT('Ctrl Pts',(-7.85076710872221,0.268205860112767,
-39.018544952774));
#24230=CARTESIAN_POINT('Ctrl Pts',(-7.0416489135512,-3.4816173191498,-38.9007703471068));
#24231=CARTESIAN_POINT('Ctrl Pts',(-4.55322857220969,-6.40113959761918,
-38.7829957414397));
#24232=CARTESIAN_POINT('Ctrl Pts',(-0.978948000220917,-7.79410927503433,
-38.6652211357725));
#24233=CARTESIAN_POINT('Ctrl Pts',(2.82879344120486,-7.32832902144949,-38.5474465301054));
#24234=CARTESIAN_POINT('Ctrl Pts',(5.96192032076547,-5.11487875385082,-38.4296719244383));
#24235=CARTESIAN_POINT('Ctrl Pts',(7.673240218259,-1.68162514608217,-38.3118973187712));
#24236=CARTESIAN_POINT('Ctrl Pts',(7.55463520417472,2.15266474723415,-38.194122713104));
#24237=CARTESIAN_POINT('Ctrl Pts',(5.63439036538128,5.47358418006194,-38.0763481074369));
#24238=CARTESIAN_POINT('Ctrl Pts',(2.37044834082958,7.48915571177013,-37.9585735017698));
#24239=CARTESIAN_POINT('Ctrl Pts',(-1.45880147521322,7.71870304979355,-37.8407988961027));
#24240=CARTESIAN_POINT('Ctrl Pts',(-4.94015430039627,6.1074834555371,-37.7230242904356));
#24241=CARTESIAN_POINT('Ctrl Pts',(-7.24337231919559,3.03974274507905,-37.6052496847684));
#24242=CARTESIAN_POINT('Ctrl Pts',(-7.81918090433069,-0.752919933008821,
-37.4874750791013));
#24243=CARTESIAN_POINT('Ctrl Pts',(-6.53026046486378,-4.36602537973952,
-37.3697004734342));
#24244=CARTESIAN_POINT('Ctrl Pts',(-3.68399445461933,-6.93791476092821,
-37.251925867767));
#24245=CARTESIAN_POINT('Ctrl Pts',(0.0408355388858274,-7.85524129040592,
-37.1341512620999));
#24246=CARTESIAN_POINT('Ctrl Pts',(3.7559272117303,-6.89923776037179,-37.0163766564328));
#24247=CARTESIAN_POINT('Ctrl Pts',(6.57529978612382,-4.29789709453984,-36.8986020507657));
#24248=CARTESIAN_POINT('Ctrl Pts',(7.82658660204039,-0.671582715448067,
-36.7808274450985));
#24249=CARTESIAN_POINT('Ctrl Pts',(7.21137661491463,3.11488089947291,-36.6630528394314));
#24250=CARTESIAN_POINT('Ctrl Pts',(4.87639090472621,6.15852522964781,-36.5452782337643));
#24251=CARTESIAN_POINT('Ctrl Pts',(1.37847002219063,7.73343166800063,-36.4275036280971));
#24252=CARTESIAN_POINT('Ctrl Pts',(-2.44817659298399,7.46414864515686,-36.30972902243));
#24253=CARTESIAN_POINT('Ctrl Pts',(-5.69100653728461,5.41462229751315,-36.1919544167629));
#24254=CARTESIAN_POINT('Ctrl Pts',(-7.57657992202902,2.07418218178154,-36.0741798110957));
#24255=CARTESIAN_POINT('Ctrl Pts',(-7.6554005846887,-1.76168036825176,-35.9564052054286));
#24256=CARTESIAN_POINT('Ctrl Pts',(-6.49046945967997,-4.03751288464302,
-35.8778888016505));
#24257=CARTESIAN_POINT('Ctrl Pts',(-5.67311119403177,-4.97042408956735,
-35.8386305997615));
#24258=CARTESIAN_POINT('Ctrl Pts',(-1.88431329769136,7.01430911752138,-48.4841082007155));
#24259=CARTESIAN_POINT('Ctrl Pts',(-3.03777695224175,6.70444440151624,-48.4448499988265));
#24260=CARTESIAN_POINT('Ctrl Pts',(-5.18781743724676,5.50513642921826,-48.3663335950484));
#24261=CARTESIAN_POINT('Ctrl Pts',(-7.17630451668021,2.39141932036274,-48.2485589893813));
#24262=CARTESIAN_POINT('Ctrl Pts',(-7.45306200576714,-1.29192685259649,
-48.1307843837141));
#24263=CARTESIAN_POINT('Ctrl Pts',(-5.9525563730179,-4.66750180559774,-48.013009778047));
#24264=CARTESIAN_POINT('Ctrl Pts',(-3.03240139215972,-6.92980316406803,
-47.8952351723799));
#24265=CARTESIAN_POINT('Ctrl Pts',(0.61088769440616,-7.53955489198126,-47.7774605667127));
#24266=CARTESIAN_POINT('Ctrl Pts',(4.10850973534028,-6.35122408963641,-47.6596859610457));
#24267=CARTESIAN_POINT('Ctrl Pts',(6.62631970094104,-3.64826384428806,-47.5419113553785));
#24268=CARTESIAN_POINT('Ctrl Pts',(7.56388023774832,-0.075251133634871,
-47.4241367497114));
#24269=CARTESIAN_POINT('Ctrl Pts',(6.697593999022,3.51570290842873,-47.3063621440442));
#24270=CARTESIAN_POINT('Ctrl Pts',(4.23405737932386,6.26822956679788,-47.1885875383771));
#24271=CARTESIAN_POINT('Ctrl Pts',(0.76077638630684,7.5258990615926,-47.07081293271));
#24272=CARTESIAN_POINT('Ctrl Pts',(-2.89393534829288,6.98878232326731,-46.9530383270428));
#24273=CARTESIAN_POINT('Ctrl Pts',(-5.85849751734439,4.7849708622563,-46.8352637213758));
#24274=CARTESIAN_POINT('Ctrl Pts',(-7.42591705410972,1.44003308444595,-46.7174891157086));
#24275=CARTESIAN_POINT('Ctrl Pts',(-7.22239367955339,-2.24832583610844,
-46.5997145100415));
#24276=CARTESIAN_POINT('Ctrl Pts',(-5.29646388240766,-5.40050087724156,
-46.4819399043744));
#24277=CARTESIAN_POINT('Ctrl Pts',(-2.10742608015855,-7.26475703579091,
-46.3641652987072));
#24278=CARTESIAN_POINT('Ctrl Pts',(1.58419360438427,-7.39650390749722,-46.2463906930401));
#24279=CARTESIAN_POINT('Ctrl Pts',(4.89801261108683,-5.76432232848308,-46.1286160873729));
#24280=CARTESIAN_POINT('Ctrl Pts',(7.0437468148628,-2.75745720732937,-46.0108414817059));
#24281=CARTESIAN_POINT('Ctrl Pts',(7.50967856162251,0.907010111327988,-45.8930668760387));
#24282=CARTESIAN_POINT('Ctrl Pts',(6.18469180635125,4.35517240796861,-45.7752922703716));
#24283=CARTESIAN_POINT('Ctrl Pts',(3.38477121781176,6.76470718099003,-45.6575176647045));
#24284=CARTESIAN_POINT('Ctrl Pts',(-0.222354279662207,7.5609852543444,-45.5397430590373));
#24285=CARTESIAN_POINT('Ctrl Pts',(-3.77645242183215,6.55410913454158,-45.4219684533702));
#24286=CARTESIAN_POINT('Ctrl Pts',(-6.42993698118103,3.9842000276029,-45.304193847703));
#24287=CARTESIAN_POINT('Ctrl Pts',(-7.55000129978989,0.464133402250619,
-45.186419242036));
#24288=CARTESIAN_POINT('Ctrl Pts',(-6.86953089392742,-3.16662039709077,
-45.0686446363688));
#24289=CARTESIAN_POINT('Ctrl Pts',(-4.55080528463124,-6.04219419609158,
-44.9508700307017));
#24290=CARTESIAN_POINT('Ctrl Pts',(-1.14679735366105,-7.47681718858616,
-44.8330954250346));
#24291=CARTESIAN_POINT('Ctrl Pts',(2.53070039210556,-7.12835850440353,-44.7153208193674));
#24292=CARTESIAN_POINT('Ctrl Pts',(5.60467321750733,-5.07991905121136,-44.5975462137003));
#24293=CARTESIAN_POINT('Ctrl Pts',(7.34203584289489,-1.820013495431,-44.4797716080332));
#24294=CARTESIAN_POINT('Ctrl Pts',(7.32845963284276,1.8739313892719,-44.361997002366));
#24295=CARTESIAN_POINT('Ctrl Pts',(5.56718226065119,5.12097853135463,-44.244222396699));
#24296=CARTESIAN_POINT('Ctrl Pts',(2.47823558355166,7.14676764938687,-44.1264477910318));
#24297=CARTESIAN_POINT('Ctrl Pts',(-1.20172413399882,7.46818576012066,-44.0086731853647));
#24298=CARTESIAN_POINT('Ctrl Pts',(-4.59509502241141,6.00858062914315,-43.8908985796975));
#24299=CARTESIAN_POINT('Ctrl Pts',(-6.8926213113915,3.11604090147352,-43.7731239740304));
#24300=CARTESIAN_POINT('Ctrl Pts',(-7.54638576232856,-0.519616558655614,
-43.6553493683633));
#24301=CARTESIAN_POINT('Ctrl Pts',(-6.40047772715846,-4.03135514511596,
-43.5375747626962));
#24302=CARTESIAN_POINT('Ctrl Pts',(-3.72817493477751,-6.58169059570571,
-43.419800157029));
#24303=CARTESIAN_POINT('Ctrl Pts',(-0.166771841295187,-7.56241539422793,
-43.3020255513619));
#24304=CARTESIAN_POINT('Ctrl Pts',(3.43440323094479,-6.73964493791626,-43.1842509456948));
#24305=CARTESIAN_POINT('Ctrl Pts',(6.21653708324298,-4.309594660124,-43.0664763400276));
#24306=CARTESIAN_POINT('Ctrl Pts',(7.51614259681957,-0.851786303117605,
-42.9487017343606));
#24307=CARTESIAN_POINT('Ctrl Pts',(7.02328805611709,2.80915722641283,-42.8309271286934));
#24308=CARTESIAN_POINT('Ctrl Pts',(4.85551009184728,5.80016906562848,-42.7131525230263));
#24309=CARTESIAN_POINT('Ctrl Pts',(1.52978338316862,7.40794858530251,-42.5953779173591));
#24310=CARTESIAN_POINT('Ctrl Pts',(-2.16076817691586,7.24907030780721,-42.477603311692));
#24311=CARTESIAN_POINT('Ctrl Pts',(-5.33601676159937,5.3614237439168,-42.3598287060249));
#24312=CARTESIAN_POINT('Ctrl Pts',(-7.2387247084592,2.19517745001321,-42.2420541003578));
#24313=CARTESIAN_POINT('Ctrl Pts',(-7.41513160172723,-1.49457779020387,
-42.1242794946906));
#24314=CARTESIAN_POINT('Ctrl Pts',(-5.82316768216064,-4.82790405738806,
-42.0065048890235));
#24315=CARTESIAN_POINT('Ctrl Pts',(-2.84248670125753,-7.00986510534107,
-41.8887302833564));
#24316=CARTESIAN_POINT('Ctrl Pts',(0.81607442909611,-7.5201038535435,-41.7709556776893));
#24317=CARTESIAN_POINT('Ctrl Pts',(4.28001700390344,-6.23693786149917,-41.6531810720221));
#24318=CARTESIAN_POINT('Ctrl Pts',(6.72325521975163,-3.46637832499379,-41.535406466355));
#24319=CARTESIAN_POINT('Ctrl Pts',(7.56312225671513,0.130847895988726,-41.4176318606878));
#24320=CARTESIAN_POINT('Ctrl Pts',(6.59932546530375,3.69686933024385,-41.2998572550208));
#24321=CARTESIAN_POINT('Ctrl Pts',(4.06171243379752,6.38125626714983,-41.1820826493536));
#24322=CARTESIAN_POINT('Ctrl Pts',(0.555456618340993,7.54383240714197,-41.0643080436865));
#24323=CARTESIAN_POINT('Ctrl Pts',(-3.08326525765602,6.90734498869397,-40.9465334380193));
#24324=CARTESIAN_POINT('Ctrl Pts',(-5.98668578194193,4.62358440932992,-40.8287588323522));
#24325=CARTESIAN_POINT('Ctrl Pts',(-7.46239322289808,1.23718504224273,-40.7109842266851));
#24326=CARTESIAN_POINT('Ctrl Pts',(-7.15845883441,-2.44425992029525,-40.593209621018));
#24327=CARTESIAN_POINT('Ctrl Pts',(-5.14736530869233,-5.54279440542178,
-40.4754350153509));
#24328=CARTESIAN_POINT('Ctrl Pts',(-1.90872100386664,-7.31947563499618,
-40.3576604096837));
#24329=CARTESIAN_POINT('Ctrl Pts',(1.78511771885662,-7.35059821863013,-40.2398858040166));
#24330=CARTESIAN_POINT('Ctrl Pts',(5.05323910559024,-5.62873999964806,-40.1221111983495));
#24331=CARTESIAN_POINT('Ctrl Pts',(7.11625705996958,-2.56453210124912,-40.0043365926823));
#24332=CARTESIAN_POINT('Ctrl Pts',(7.48218021450115,1.11126895017883,-39.8865619870152));
#24333=CARTESIAN_POINT('Ctrl Pts',(6.0637427105368,4.52205304948066,-39.7687873813481));
#24334=CARTESIAN_POINT('Ctrl Pts',(3.19921548061873,6.85441169980844,-39.651012775681));
#24335=CARTESIAN_POINT('Ctrl Pts',(-0.428265070124539,7.55212079297079,
-39.5332381700138));
#24336=CARTESIAN_POINT('Ctrl Pts',(-3.95361237619466,6.44878970200573,-39.4154635643467));
#24337=CARTESIAN_POINT('Ctrl Pts',(-6.53609674916458,3.80754234743014,-39.2976889586796));
#24338=CARTESIAN_POINT('Ctrl Pts',(-7.55984375348351,0.258267041696921,
-39.1799143530124));
#24339=CARTESIAN_POINT('Ctrl Pts',(-6.7807087913984,-3.35260014437985,-39.0621397473453));
#24340=CARTESIAN_POINT('Ctrl Pts',(-4.38450104341517,-6.1639346234681,-38.9443651416782));
#24341=CARTESIAN_POINT('Ctrl Pts',(-0.942671438595233,-7.50528547094125,
-38.8265905360111));
#24342=CARTESIAN_POINT('Ctrl Pts',(2.72396775120595,-7.0567654866142,-38.7088159303439));
#24343=CARTESIAN_POINT('Ctrl Pts',(5.74099135428831,-4.92533833466603,-38.5910413246768));
#24344=CARTESIAN_POINT('Ctrl Pts',(7.38889541998213,-1.61930970314814,-38.4732667190097));
#24345=CARTESIAN_POINT('Ctrl Pts',(7.2746855138112,2.07289414108871,-38.3554921133426));
#24346=CARTESIAN_POINT('Ctrl Pts',(5.42559857126474,5.27075132910704,-38.2377175076754));
#24347=CARTESIAN_POINT('Ctrl Pts',(2.282607398004,7.21163247392595,-38.1199429020083));
#24348=CARTESIAN_POINT('Ctrl Pts',(-1.40474313748407,7.43267354997024,-38.0021682963412));
#24349=CARTESIAN_POINT('Ctrl Pts',(-4.75708858916514,5.88116040272668,-37.8843936906741));
#24350=CARTESIAN_POINT('Ctrl Pts',(-6.97495699758933,2.92709997447918,-37.7666190850069));
#24351=CARTESIAN_POINT('Ctrl Pts',(-7.52942802892327,-0.725019220874125,
-37.6488444793398));
#24352=CARTESIAN_POINT('Ctrl Pts',(-6.28827070020625,-4.20423497952246,
-37.5310698736727));
#24353=CARTESIAN_POINT('Ctrl Pts',(-3.54747785533976,-6.68081868195182,
-37.4132952680055));
#24354=CARTESIAN_POINT('Ctrl Pts',(0.0393223094368914,-7.56415213685359,
-37.2955206623384));
#24355=CARTESIAN_POINT('Ctrl Pts',(3.61674502337384,-6.64357492258274,-37.1777460566713));
#24356=CARTESIAN_POINT('Ctrl Pts',(6.33164101380409,-4.13863130230598,-37.0599714510042));
#24357=CARTESIAN_POINT('Ctrl Pts',(7.5365592960715,-0.646696090460631,-36.942196845337));
#24358=CARTESIAN_POINT('Ctrl Pts',(6.94414694784554,2.99945375841853,-36.8244222396699));
#24359=CARTESIAN_POINT('Ctrl Pts',(4.6956880531689,5.93031073820777,-36.7066476340028));
#24360=CARTESIAN_POINT('Ctrl Pts',(1.32738850131529,7.44685637450296,-36.5888730283356));
#24361=CARTESIAN_POINT('Ctrl Pts',(-2.3574552992831,7.1875520861484,-36.4710984226685));
#24362=CARTESIAN_POINT('Ctrl Pts',(-5.48011673586982,5.21397437810249,-36.3533238170014));
#24363=CARTESIAN_POINT('Ctrl Pts',(-7.29581703330418,1.99731987885706,-36.2355492113343));
#24364=CARTESIAN_POINT('Ctrl Pts',(-7.3717168639833,-1.69639834466192,-36.1177746056671));
#24365=CARTESIAN_POINT('Ctrl Pts',(-6.24995421752146,-3.88789606644511,
-36.039258201889));
#24366=CARTESIAN_POINT('Ctrl Pts',(-5.46288453460428,-4.78623668048096,
-36.));
#24367=CARTESIAN_POINT('Ctrl Pts',(-5.46288453460428,-4.78623668048096,
-36.));
#24368=CARTESIAN_POINT('Ctrl Pts',(-5.5977429381527,-4.64891391735923,-36.));
#24369=CARTESIAN_POINT('Ctrl Pts',(-5.72676732341115,-4.50639566671148,
-36.));
#24370=CARTESIAN_POINT('Ctrl Pts',(-5.84982542989412,-4.35916059628739,
-36.));
#24371=CARTESIAN_POINT('Ctrl Pts',(-5.97481042968556,-4.20962005993278,
-36.));
#24372=CARTESIAN_POINT('Ctrl Pts',(-6.09364127024401,-4.05521340122182,
-36.));
#24373=CARTESIAN_POINT('Ctrl Pts',(-6.20615068412284,-3.89639624867873,
-36.));
#24374=CARTESIAN_POINT('Ctrl Pts',(-6.32533404445892,-3.7281582207082,-36.));
#24375=CARTESIAN_POINT('Ctrl Pts',(-6.43742462013448,-3.55497067838873,
-36.));
#24376=CARTESIAN_POINT('Ctrl Pts',(-6.54218137983461,-3.37732902325465,
-36.));
#24377=CARTESIAN_POINT('Ctrl Pts',(-6.6419677919629,-3.20811585303918,-36.));
#24378=CARTESIAN_POINT('Ctrl Pts',(-6.73509988284937,-3.03486032491094,
-36.));
#24379=CARTESIAN_POINT('Ctrl Pts',(-6.82132654460192,-2.85795957462792,
-36.));
#24380=CARTESIAN_POINT('Ctrl Pts',(-6.86766107917013,-2.76290064781184,
-36.));
#24381=CARTESIAN_POINT('Ctrl Pts',(-6.91200089902377,-2.66678868814126,
-36.));
#24382=CARTESIAN_POINT('Ctrl Pts',(-6.95430142435144,-2.56968261694418,
-36.));
#24383=CARTESIAN_POINT('Ctrl Pts',(-6.97457148673207,-2.52315018961722,
-36.));
#24384=CARTESIAN_POINT('Ctrl Pts',(-6.99437321597084,-2.47638946583898,
-36.));
#24385=CARTESIAN_POINT('Ctrl Pts',(-7.01370136184102,-2.42940681080466,
-36.));
#24386=CARTESIAN_POINT('Ctrl Pts',(-7.02151953803784,-2.41040246979236,
-36.));
#24387=CARTESIAN_POINT('Ctrl Pts',(-7.02925969742251,-2.39136302740604,
-36.));
#24388=CARTESIAN_POINT('Ctrl Pts',(-7.03691795983629,-2.37229797553799,
-36.));
#24389=CARTESIAN_POINT('Ctrl Pts',(-7.11159816098769,-2.18638349108455,
-36.));
#24390=CARTESIAN_POINT('Ctrl Pts',(-7.17859038835048,-1.99780273753807,
-36.));
#24391=CARTESIAN_POINT('Ctrl Pts',(-7.23771363498118,-1.80701554492453,
-36.));
#24392=CARTESIAN_POINT('Ctrl Pts',(-7.25137682897175,-1.76292523236309,
-36.));
#24393=CARTESIAN_POINT('Ctrl Pts',(-7.26461960889502,-1.71871693832445,
-36.));
#24394=CARTESIAN_POINT('Ctrl Pts',(-7.27743943403625,-1.67439609022036,
-36.));
#24395=CARTESIAN_POINT('Ctrl Pts',(-7.33236404335992,-1.48451009410166,
-36.));
#24396=CARTESIAN_POINT('Ctrl Pts',(-7.37952880573868,-1.29256003410601,
-36.));
#24397=CARTESIAN_POINT('Ctrl Pts',(-7.41900478204454,-1.09903177851102,
-36.));
#24398=CARTESIAN_POINT('Ctrl Pts',(-7.45887446791156,-0.903573388902557,
-36.));
#24399=CARTESIAN_POINT('Ctrl Pts',(-7.49090138133267,-0.706504520118917,
-36.));
#24400=CARTESIAN_POINT('Ctrl Pts',(-7.51510912682397,-0.508306182126472,
-36.));
#24401=CARTESIAN_POINT('Ctrl Pts',(-7.53937145031977,-0.309660992535023,
-36.));
#24402=CARTESIAN_POINT('Ctrl Pts',(-7.55577940447303,-0.109880537467743,
-36.));
#24403=CARTESIAN_POINT('Ctrl Pts',(-7.56430545051381,0.0905602703403912,
-36.));
#24404=CARTESIAN_POINT('Ctrl Pts',(-7.56775676889125,0.171698120202889,
-36.));
#24405=CARTESIAN_POINT('Ctrl Pts',(-7.56991595964691,0.252944223882185,
-36.));
#24406=CARTESIAN_POINT('Ctrl Pts',(-7.57077875624231,0.334267110558196,
-36.));
#24407=CARTESIAN_POINT('Ctrl Pts',(-7.57111625441944,0.366077998731034,
-36.));
#24408=CARTESIAN_POINT('Ctrl Pts',(-7.57125537315957,0.39790063464037,-36.));
#24409=CARTESIAN_POINT('Ctrl Pts',(-7.57119579778133,0.429733129242087,
-36.));
#24410=CARTESIAN_POINT('Ctrl Pts',(-7.57115243537445,0.45290266040532,-36.));
#24411=CARTESIAN_POINT('Ctrl Pts',(-7.57100382199647,0.476067956682383,
-36.));
#24412=CARTESIAN_POINT('Ctrl Pts',(-7.57075011198204,0.499226838302265,
-36.));
#24413=CARTESIAN_POINT('Ctrl Pts',(-7.56852835775061,0.702030591829401,
-36.));
#24414=CARTESIAN_POINT('Ctrl Pts',(-7.55825116056467,0.904376836416967,
-36.));
#24415=CARTESIAN_POINT('Ctrl Pts',(-7.53999292732573,1.10576724548481,-36.));
#24416=CARTESIAN_POINT('Ctrl Pts',(-7.52160278416925,1.30861263608914,-36.));
#24417=CARTESIAN_POINT('Ctrl Pts',(-7.49511597555556,1.51048903114456,-36.));
#24418=CARTESIAN_POINT('Ctrl Pts',(-7.46055732979923,1.71089945545224,-36.));
#24419=CARTESIAN_POINT('Ctrl Pts',(-7.44239807242019,1.81620753095109,-36.));
#24420=CARTESIAN_POINT('Ctrl Pts',(-7.42200923698019,1.92111097525443,-36.));
#24421=CARTESIAN_POINT('Ctrl Pts',(-7.39938866576489,2.02553801505189,-36.));
#24422=CARTESIAN_POINT('Ctrl Pts',(-7.35650604167764,2.22350408096407,-36.));
#24423=CARTESIAN_POINT('Ctrl Pts',(-7.30560612447398,2.41975870171209,-36.));
#24424=CARTESIAN_POINT('Ctrl Pts',(-7.24693498701336,2.61389377398034,-36.));
#24425=CARTESIAN_POINT('Ctrl Pts',(-7.20801045153952,2.74268993908444,-36.));
#24426=CARTESIAN_POINT('Ctrl Pts',(-7.16566433956697,2.87055307976224,-36.));
#24427=CARTESIAN_POINT('Ctrl Pts',(-7.11995630029871,2.99736080966695,-36.));
#24428=CARTESIAN_POINT('Ctrl Pts',(-7.0956591489905,3.06476835218834,-36.));
#24429=CARTESIAN_POINT('Ctrl Pts',(-7.07041185875794,3.13187761376778,-36.));
#24430=CARTESIAN_POINT('Ctrl Pts',(-7.04422232586475,3.19866977263125,-36.));
#24431=CARTESIAN_POINT('Ctrl Pts',(-7.02727219339145,3.24189833823913,-36.));
#24432=CARTESIAN_POINT('Ctrl Pts',(-7.00992735853431,3.28499406894694,-36.));
#24433=CARTESIAN_POINT('Ctrl Pts',(-6.99218980245843,3.32795178036667,-36.));
#24434=CARTESIAN_POINT('Ctrl Pts',(-6.98238542220851,3.35169652488635,-36.));
#24435=CARTESIAN_POINT('Ctrl Pts',(-6.97246413601817,3.37539157447853,-36.));
#24436=CARTESIAN_POINT('Ctrl Pts',(-6.96242907172261,3.39903020671605,-36.));
#24437=CARTESIAN_POINT('Ctrl Pts',(-6.8820400364091,3.58839489693994,-36.));
#24438=CARTESIAN_POINT('Ctrl Pts',(-6.79430423304295,3.77425987667949,-36.));
#24439=CARTESIAN_POINT('Ctrl Pts',(-6.69953894329377,3.95622441588123,-36.));
#24440=CARTESIAN_POINT('Ctrl Pts',(-6.60408872841896,4.13950412105991,-36.));
#24441=CARTESIAN_POINT('Ctrl Pts',(-6.50150681992606,4.31882744677142,-36.));
#24442=CARTESIAN_POINT('Ctrl Pts',(-6.39206475516827,4.49377628022932,-36.));
#24443=CARTESIAN_POINT('Ctrl Pts',(-6.28276629228395,4.66849555862261,-36.));
#24444=CARTESIAN_POINT('Ctrl Pts',(-6.16662537039312,4.83885245890798,-36.));
#24445=CARTESIAN_POINT('Ctrl Pts',(-6.04386414064415,5.00441227621188,-36.));
#24446=CARTESIAN_POINT('Ctrl Pts',(-5.93619135704333,5.1496233205946,-36.));
#24447=CARTESIAN_POINT('Ctrl Pts',(-5.8234248145294,5.29114403181261,-36.));
#24448=CARTESIAN_POINT('Ctrl Pts',(-5.70568638354113,5.42866360742757,-36.));
#24449=CARTESIAN_POINT('Ctrl Pts',(-5.59912529758274,5.55312794073882,-36.));
#24450=CARTESIAN_POINT('Ctrl Pts',(-5.4884910261217,5.67431465864635,-36.));
#24451=CARTESIAN_POINT('Ctrl Pts',(-5.37397124395929,5.79208610573226,-36.));
#24452=CARTESIAN_POINT('Ctrl Pts',(-5.35469223029994,5.8119125260605,-36.));
#24453=CARTESIAN_POINT('Ctrl Pts',(-5.33530306689327,5.83164212072248,-36.));
#24454=CARTESIAN_POINT('Ctrl Pts',(-5.31580461121635,5.85127418954356,-36.));
#24455=CARTESIAN_POINT('Ctrl Pts',(-5.29758405791643,5.86961959916314,-36.));
#24456=CARTESIAN_POINT('Ctrl Pts',(-5.27927479958802,5.88787306572556,-36.));
#24457=CARTESIAN_POINT('Ctrl Pts',(-5.2608784327401,5.90603352499053,-36.));
#24458=CARTESIAN_POINT('Ctrl Pts',(-5.11313200936276,6.05188530787087,-36.));
#24459=CARTESIAN_POINT('Ctrl Pts',(-4.95975635606592,6.19175466572801,-36.));
#24460=CARTESIAN_POINT('Ctrl Pts',(-4.8012057401011,6.32542432410788,-36.));
#24461=CARTESIAN_POINT('Ctrl Pts',(-4.64119267814809,6.46032693042967,-36.));
#24462=CARTESIAN_POINT('Ctrl Pts',(-4.47590827252764,6.58891541157199,-36.));
#24463=CARTESIAN_POINT('Ctrl Pts',(-4.30577794008802,6.71093368313889,-36.));
#24464=CARTESIAN_POINT('Ctrl Pts',(-4.1678201015731,6.80987769131963,-36.));
#24465=CARTESIAN_POINT('Ctrl Pts',(-4.0266749161711,6.90450093600378,-36.));
#24466=CARTESIAN_POINT('Ctrl Pts',(-3.88255277813534,6.99464804083222,-36.));
#24467=CARTESIAN_POINT('Ctrl Pts',(-3.84870261918472,7.0158210116816,-36.));
#24468=CARTESIAN_POINT('Ctrl Pts',(-3.81468500239647,7.03674881166959,-36.));
#24469=CARTESIAN_POINT('Ctrl Pts',(-3.78052548560284,7.05741567578707,-36.));
#24470=CARTESIAN_POINT('Ctrl Pts',(-3.5993859527263,7.16700698338312,-36.));
#24471=CARTESIAN_POINT('Ctrl Pts',(-3.41413883495251,7.26934114557307,-36.));
#24472=CARTESIAN_POINT('Ctrl Pts',(-3.22522572651255,7.36416890252957,-36.));
#24473=CARTESIAN_POINT('Ctrl Pts',(-3.03641081725833,7.45894736693779,-36.));
#24474=CARTESIAN_POINT('Ctrl Pts',(-2.84393316488135,7.54622765878111,-36.));
#24475=CARTESIAN_POINT('Ctrl Pts',(-2.64820158305729,7.62572028826821,-36.));
#24476=CARTESIAN_POINT('Ctrl Pts',(-2.60498558090497,7.64327163902619,-36.));
#24477=CARTESIAN_POINT('Ctrl Pts',(-2.56161084699581,7.66044317611024,-36.));
#24478=CARTESIAN_POINT('Ctrl Pts',(-2.51808161300395,7.67723148371408,-36.));
#24479=CARTESIAN_POINT('Ctrl Pts',(-2.38090156124179,7.73013893681846,-36.));
#24480=CARTESIAN_POINT('Ctrl Pts',(-2.2421874023443,7.77924117058327,-36.));
#24481=CARTESIAN_POINT('Ctrl Pts',(-2.10210198597179,7.8245263256498,-36.));
#24482=CARTESIAN_POINT('Ctrl Pts',(-7.26313420453275,-0.000171068891272981,
-37.6717617050839));
#24483=CARTESIAN_POINT('Ctrl Pts',(-7.26336489575239,-0.232559497234902,
-37.6641226298359));
#24484=CARTESIAN_POINT('Ctrl Pts',(-7.25242649701633,-0.464926300116374,
-37.6564835545879));
#24485=CARTESIAN_POINT('Ctrl Pts',(-7.23015663558145,-0.696201981423296,
-37.6488444793398));
#24486=CARTESIAN_POINT('Ctrl Pts',(-7.11570891935093,-1.88475780709024,
-37.6095862774508));
#24487=CARTESIAN_POINT('Ctrl Pts',(-6.70198980977859,-3.04449639330636,
-37.5703280755617));
#24488=CARTESIAN_POINT('Ctrl Pts',(-6.03833144751466,-4.03712963681931,
-37.5310698736727));
#24489=CARTESIAN_POINT('Ctrl Pts',(-5.37467308525075,-5.02976288033225,
-37.4918116717836));
#24490=CARTESIAN_POINT('Ctrl Pts',(-4.46107547029526,-5.85529078114203,
-37.4525534698946));
#24491=CARTESIAN_POINT('Ctrl Pts',(-3.40647663535475,-6.41527697403055,
-37.4132952680055));
#24492=CARTESIAN_POINT('Ctrl Pts',(-2.35187780041423,-6.97526316691907,
-37.3740370661165));
#24493=CARTESIAN_POINT('Ctrl Pts',(-1.15627774548866,-7.26970765188633,
-37.3347788642275));
#24494=CARTESIAN_POINT('Ctrl Pts',(0.0377594009636062,-7.26350035865815,
-37.2955206623384));
#24495=CARTESIAN_POINT('Ctrl Pts',(1.23179654741588,-7.25729306542997,-37.2562624604494));
#24496=CARTESIAN_POINT('Ctrl Pts',(2.42427078539487,-6.95043399400635,-37.2170042585603));
#24497=CARTESIAN_POINT('Ctrl Pts',(3.47299056945607,-6.37951385491508,-37.1777460566713));
#24498=CARTESIAN_POINT('Ctrl Pts',(4.52171035351726,-5.80859371582382,-37.1384878547822));
#24499=CARTESIAN_POINT('Ctrl Pts',(5.42667568366067,-4.9736125090649,-37.0992296528932));
#24500=CARTESIAN_POINT('Ctrl Pts',(6.07997806244361,-3.97413270371123,-37.0599714510042));
#24501=CARTESIAN_POINT('Ctrl Pts',(6.73328044122656,-2.97465289835754,-37.0207132491151));
#24502=CARTESIAN_POINT('Ctrl Pts',(7.13491986864902,-1.81067449440914,-36.9814550472261));
#24503=CARTESIAN_POINT('Ctrl Pts',(7.23700419098927,-0.620993650955046,
-36.942196845337));
#24504=CARTESIAN_POINT('Ctrl Pts',(7.33908851332952,0.568687192499043,-36.902938643448));
#24505=CARTESIAN_POINT('Ctrl Pts',(7.14161773058753,1.78407047545882,-36.8636804415589));
#24506=CARTESIAN_POINT('Ctrl Pts',(6.66813919010376,2.88023828023689,-36.8244222396699));
#24507=CARTESIAN_POINT('Ctrl Pts',(6.19466064962,3.97640608501494,-36.7851640377808));
#24508=CARTESIAN_POINT('Ctrl Pts',(5.44517435139446,4.95335841161134,-36.7459058358918));
#24509=CARTESIAN_POINT('Ctrl Pts',(4.50904794363943,5.69459218095874,-36.7066476340028));
#24510=CARTESIAN_POINT('Ctrl Pts',(3.57292153588436,6.43582595030617,-36.6673894321137));
#24511=CARTESIAN_POINT('Ctrl Pts',(2.45015501859983,6.94134116240457,-36.6281312302247));
#24512=CARTESIAN_POINT('Ctrl Pts',(1.27463112652446,7.15088138706134,-36.5888730283356));
#24513=CARTESIAN_POINT('Ctrl Pts',(0.0991072344491403,7.36042161171811,
-36.5496148264466));
#24514=CARTESIAN_POINT('Ctrl Pts',(-1.12917403241698,7.27398684893325,-36.5103566245576));
#24515=CARTESIAN_POINT('Ctrl Pts',(-2.26375823861449,6.90183984953318,-36.4710984226685));
#24516=CARTESIAN_POINT('Ctrl Pts',(-3.39834244481199,6.5296928501331,-36.4318402207795));
#24517=CARTESIAN_POINT('Ctrl Pts',(-4.43922959034089,5.8718336141178,-36.3925820188904));
#24518=CARTESIAN_POINT('Ctrl Pts',(-5.2622898793444,5.00679491290259,-36.3533238170014));
#24519=CARTESIAN_POINT('Ctrl Pts',(-6.08535016834793,4.14175621168736,-36.3140656151123));
#24520=CARTESIAN_POINT('Ctrl Pts',(-6.69058360082606,3.06953804527219,-36.2748074132233));
#24521=CARTESIAN_POINT('Ctrl Pts',(-7.00585028884498,1.91780925814477,-36.2355492113343));
#24522=CARTESIAN_POINT('Ctrl Pts',(-7.17660081455138,1.29402532109461,-36.2142867092508));
#24523=CARTESIAN_POINT('Ctrl Pts',(-7.26229315301422,0.64691791887602,-36.1930242071674));
#24524=CARTESIAN_POINT('Ctrl Pts',(-7.26243100057087,-0.00011786593126363,
-36.1717617050839));
#24525=CARTESIAN_POINT('Ctrl Pts',(-2.10185380438476,7.82409821225381,-48.));
#24526=CARTESIAN_POINT('Ctrl Pts',(-2.30082761392273,7.75960640525413,-48.));
#24527=CARTESIAN_POINT('Ctrl Pts',(-2.49685179586882,7.68738676969109,-48.));
#24528=CARTESIAN_POINT('Ctrl Pts',(-2.6895559228274,7.60776024312852,-48.));
#24529=CARTESIAN_POINT('Ctrl Pts',(-2.88412187838993,7.52736439757352,-48.));
#24530=CARTESIAN_POINT('Ctrl Pts',(-3.07530391165674,7.43941750700123,-48.));
#24531=CARTESIAN_POINT('Ctrl Pts',(-3.26270174750119,7.34420014302048,-48.));
#24532=CARTESIAN_POINT('Ctrl Pts',(-3.45039148143023,7.2488344648074,-48.));
#24533=CARTESIAN_POINT('Ctrl Pts',(-3.63428579989924,7.14617524942011,-48.));
#24534=CARTESIAN_POINT('Ctrl Pts',(-3.81395475017913,7.03646034322168,-48.));
#24535=CARTESIAN_POINT('Ctrl Pts',(-3.991435635466,6.92808157966276,-48.));
#24536=CARTESIAN_POINT('Ctrl Pts',(-4.16479392090228,6.81281747740625,-48.));
#24537=CARTESIAN_POINT('Ctrl Pts',(-4.33358029554524,6.69086083083259,-48.));
#24538=CARTESIAN_POINT('Ctrl Pts',(-4.43066212905975,6.62071432236176,-48.));
#24539=CARTESIAN_POINT('Ctrl Pts',(-4.52623076734692,6.54835310014871,-48.));
#24540=CARTESIAN_POINT('Ctrl Pts',(-4.62019444968023,6.47380914459575,-48.));
#24541=CARTESIAN_POINT('Ctrl Pts',(-4.66632206375462,6.43721484850242,-48.));
#24542=CARTESIAN_POINT('Ctrl Pts',(-4.71206282220744,6.40009448292469,-48.));
#24543=CARTESIAN_POINT('Ctrl Pts',(-4.75740541705904,6.3624515606279,-48.));
#24544=CARTESIAN_POINT('Ctrl Pts',(-4.77704340810378,6.34614831699173,-48.));
#24545=CARTESIAN_POINT('Ctrl Pts',(-4.79660803540916,6.32974592678438,-48.));
#24546=CARTESIAN_POINT('Ctrl Pts',(-4.81609419498694,6.31324819669125,-48.));
#24547=CARTESIAN_POINT('Ctrl Pts',(-4.9746783621459,6.17898475825485,-48.));
#24548=CARTESIAN_POINT('Ctrl Pts',(-5.12764661424143,6.03876851300631,-48.));
#24549=CARTESIAN_POINT('Ctrl Pts',(-5.27461327719733,5.89285624935101,-48.));
#24550=CARTESIAN_POINT('Ctrl Pts',(-5.32270100774501,5.84511351996507,-48.));
#24551=CARTESIAN_POINT('Ctrl Pts',(-5.37014594422701,5.79676064522343,-48.));
#24552=CARTESIAN_POINT('Ctrl Pts',(-5.41693377234936,5.74780571127434,-48.));
#24553=CARTESIAN_POINT('Ctrl Pts',(-5.55998425669422,5.59812945371915,-48.));
#24554=CARTESIAN_POINT('Ctrl Pts',(-5.69689529217084,5.44282762220933,-48.));
#24555=CARTESIAN_POINT('Ctrl Pts',(-5.82744389958942,5.28234360952657,-48.));
#24556=CARTESIAN_POINT('Ctrl Pts',(-5.95822188709384,5.12157761883323,-48.));
#24557=CARTESIAN_POINT('Ctrl Pts',(-6.08261540116493,4.955610584521,-48.));
#24558=CARTESIAN_POINT('Ctrl Pts',(-6.20035569612236,4.78486113417545,-48.));
#24559=CARTESIAN_POINT('Ctrl Pts',(-6.31730043838319,4.61526541107098,-48.));
#24560=CARTESIAN_POINT('Ctrl Pts',(-6.42768183251017,4.44095104165386,-48.));
#24561=CARTESIAN_POINT('Ctrl Pts',(-6.53118823114018,4.2623110814615,-48.));
#24562=CARTESIAN_POINT('Ctrl Pts',(-6.57281072552227,4.19047551537149,-48.));
#24563=CARTESIAN_POINT('Ctrl Pts',(-6.61332093248692,4.11794034060233,-48.));
#24564=CARTESIAN_POINT('Ctrl Pts',(-6.65269621199041,4.04473068147045,-48.));
#24565=CARTESIAN_POINT('Ctrl Pts',(-6.66624687762794,4.01953620349232,-48.));
#24566=CARTESIAN_POINT('Ctrl Pts',(-6.67966311773293,3.99426184273103,-48.));
#24567=CARTESIAN_POINT('Ctrl Pts',(-6.69294397046647,3.96890861967423,-48.));
#24568=CARTESIAN_POINT('Ctrl Pts',(-6.70467566316242,3.94651275189961,-48.));
#24569=CARTESIAN_POINT('Ctrl Pts',(-6.7163021292488,3.92405442981521,-48.));
#24570=CARTESIAN_POINT('Ctrl Pts',(-6.72781505779003,3.90154957756383,-48.));
#24571=CARTESIAN_POINT('Ctrl Pts',(-6.82109913847309,3.71920288396099,-48.));
#24572=CARTESIAN_POINT('Ctrl Pts',(-6.90705463463742,3.5335738251812,-48.));
#24573=CARTESIAN_POINT('Ctrl Pts',(-6.98547177545329,3.3450880887619,-48.));
#24574=CARTESIAN_POINT('Ctrl Pts',(-7.06354639296283,3.15742565139383,-48.));
#24575=CARTESIAN_POINT('Ctrl Pts',(-7.13414861969922,2.96693079553113,-48.));
#24576=CARTESIAN_POINT('Ctrl Pts',(-7.1970241755622,2.77400364453458,-48.));
#24577=CARTESIAN_POINT('Ctrl Pts',(-7.2338482323043,2.66101282866221,-48.));
#24578=CARTESIAN_POINT('Ctrl Pts',(-7.26802110074051,2.54718739813178,-48.));
#24579=CARTESIAN_POINT('Ctrl Pts',(-7.29948358655117,2.43260584479025,-48.));
#24580=CARTESIAN_POINT('Ctrl Pts',(-7.35348963043526,2.23592410656683,-48.));
#24581=CARTESIAN_POINT('Ctrl Pts',(-7.39951248160726,2.03701428957662,-48.));
#24582=CARTESIAN_POINT('Ctrl Pts',(-7.43751275781667,1.83636816437194,-48.));
#24583=CARTESIAN_POINT('Ctrl Pts',(-7.46184105249056,1.70791178073268,-48.));
#24584=CARTESIAN_POINT('Ctrl Pts',(-7.48288005647684,1.57874367129889,-48.));
#24585=CARTESIAN_POINT('Ctrl Pts',(-7.50060825221396,1.44899399010199,-48.));
#24586=CARTESIAN_POINT('Ctrl Pts',(-7.50964567380242,1.38285062236542,-48.));
#24587=CARTESIAN_POINT('Ctrl Pts',(-7.5178225682247,1.31655614449737,-48.));
#24588=CARTESIAN_POINT('Ctrl Pts',(-7.52513521308343,1.25012800445878,-48.));
#24589=CARTESIAN_POINT('Ctrl Pts',(-7.52928146266447,1.2124634312263,-48.));
#24590=CARTESIAN_POINT('Ctrl Pts',(-7.53314985750579,1.17475589044629,-48.));
#24591=CARTESIAN_POINT('Ctrl Pts',(-7.53673963502003,1.13700858902824,-48.));
#24592=CARTESIAN_POINT('Ctrl Pts',(-7.53984577077182,1.10434688729227,-48.));
#24593=CARTESIAN_POINT('Ctrl Pts',(-7.54274366719671,1.07165020930486,-48.));
#24594=CARTESIAN_POINT('Ctrl Pts',(-7.54543044083257,1.03895170566994,-48.));
#24595=CARTESIAN_POINT('Ctrl Pts',(-7.56194124628142,0.838012324406245,
-48.));
#24596=CARTESIAN_POINT('Ctrl Pts',(-7.57050457306246,0.636810151048556,
-48.));
#24597=CARTESIAN_POINT('Ctrl Pts',(-7.5711534980168,0.435821641100334,-48.));
#24598=CARTESIAN_POINT('Ctrl Pts',(-7.57180231283319,0.234867243670862,
-48.));
#24599=CARTESIAN_POINT('Ctrl Pts',(-7.56453936589094,0.0341257262245018,
-48.));
#24600=CARTESIAN_POINT('Ctrl Pts',(-7.54934565132248,-0.165927071930631,
-48.));
#24601=CARTESIAN_POINT('Ctrl Pts',(-7.5343452687912,-0.363434303309763,
-48.));
#24602=CARTESIAN_POINT('Ctrl Pts',(-7.51161452717462,-0.56027087895125,
-48.));
#24603=CARTESIAN_POINT('Ctrl Pts',(-7.48108590954362,-0.755969183945798,
-48.));
#24604=CARTESIAN_POINT('Ctrl Pts',(-7.45371069442,-0.931453159778154,-48.));
#24605=CARTESIAN_POINT('Ctrl Pts',(-7.42006468953489,-1.10602206717178,
-48.));
#24606=CARTESIAN_POINT('Ctrl Pts',(-7.38006602431795,-1.27932562273681,
-48.));
#24607=CARTESIAN_POINT('Ctrl Pts',(-7.3459202615715,-1.42727011186773,-48.));
#24608=CARTESIAN_POINT('Ctrl Pts',(-7.30714419709347,-1.57429234976623,
-48.));
#24609=CARTESIAN_POINT('Ctrl Pts',(-7.26380600031078,-1.7201873188581,-48.));
#24610=CARTESIAN_POINT('Ctrl Pts',(-7.25535124039227,-1.74864966913019,
-48.));
#24611=CARTESIAN_POINT('Ctrl Pts',(-7.24672280776097,-1.77706908373106,
-48.));
#24612=CARTESIAN_POINT('Ctrl Pts',(-7.23792114978756,-1.80544399113884,
-48.));
#24613=CARTESIAN_POINT('Ctrl Pts',(-7.23013838133962,-1.83053418832141,
-48.));
#24614=CARTESIAN_POINT('Ctrl Pts',(-7.22222270787628,-1.85558137172037,
-48.));
#24615=CARTESIAN_POINT('Ctrl Pts',(-7.21417568267861,-1.88058154446126,
-48.));
#24616=CARTESIAN_POINT('Ctrl Pts',(-7.15325529115503,-2.06984655533421,
-48.));
#24617=CARTESIAN_POINT('Ctrl Pts',(-7.08479318222008,-2.25647534397251,
-48.));
#24618=CARTESIAN_POINT('Ctrl Pts',(-7.00902678423338,-2.44004180818918,
-48.));
#24619=CARTESIAN_POINT('Ctrl Pts',(-6.9317716169254,-2.62721525554879,-48.));
#24620=CARTESIAN_POINT('Ctrl Pts',(-6.84692204906886,-2.8112056027263,-48.));
#24621=CARTESIAN_POINT('Ctrl Pts',(-6.75468148462008,-2.99153370400441,
-48.));
#24622=CARTESIAN_POINT('Ctrl Pts',(-6.71535297813714,-3.06841999522078,
-48.));
#24623=CARTESIAN_POINT('Ctrl Pts',(-6.67468029006978,-3.14464012249059,
-48.));
#24624=CARTESIAN_POINT('Ctrl Pts',(-6.63267676414671,-3.22015495035686,
-48.));
#24625=CARTESIAN_POINT('Ctrl Pts',(-6.6040927348478,-3.27154392318225,-48.));
#24626=CARTESIAN_POINT('Ctrl Pts',(-6.57489236439856,-3.32260624538659,
-48.));
#24627=CARTESIAN_POINT('Ctrl Pts',(-6.54507950331467,-3.37332921731332,
-48.));
#24628=CARTESIAN_POINT('Ctrl Pts',(-6.52647856726046,-3.40497645689337,
-48.));
#24629=CARTESIAN_POINT('Ctrl Pts',(-6.50763776285718,-3.43649378986221,
-48.));
#24630=CARTESIAN_POINT('Ctrl Pts',(-6.48857066029989,-3.46785765893643,
-48.));
#24631=CARTESIAN_POINT('Ctrl Pts',(-6.38641005460389,-3.63590373997915,
-48.));
#24632=CARTESIAN_POINT('Ctrl Pts',(-6.27768399621447,-3.79967229895934,
-48.));
#24633=CARTESIAN_POINT('Ctrl Pts',(-6.16259227067162,-3.95873109139948,
-48.));
#24634=CARTESIAN_POINT('Ctrl Pts',(-6.0487757902373,-4.11602747263176,-48.));
#24635=CARTESIAN_POINT('Ctrl Pts',(-5.92873350940336,-4.26871839150529,
-48.));
#24636=CARTESIAN_POINT('Ctrl Pts',(-5.80262143945877,-4.4163511297274,-48.));
#24637=CARTESIAN_POINT('Ctrl Pts',(-5.77983952334256,-4.44302071543526,
-48.));
#24638=CARTESIAN_POINT('Ctrl Pts',(-5.75685943770476,-4.46952512978906,
-48.));
#24639=CARTESIAN_POINT('Ctrl Pts',(-5.73368198691278,-4.49586156146085,
-48.));
#24640=CARTESIAN_POINT('Ctrl Pts',(-5.64631443946142,-4.59513690733195,
-48.));
#24641=CARTESIAN_POINT('Ctrl Pts',(-5.55614289752022,-4.69202607158615,
-48.));
#24642=CARTESIAN_POINT('Ctrl Pts',(-5.46328272950438,-4.78643225728898,
-48.));
#24643=CARTESIAN_POINT('Origin',(0.,0.,-48.));
#24644=CARTESIAN_POINT('',(-12.,-1.46957615897682E-15,-48.));
#24645=CARTESIAN_POINT('Origin',(0.,0.,-48.));
#24646=CARTESIAN_POINT('Origin',(0.,0.,-48.));
#24647=CARTESIAN_POINT('Origin',(0.,0.,-48.));
#24648=CARTESIAN_POINT('',(-12.,-1.46957615897682E-15,-40.));
#24649=CARTESIAN_POINT('Origin',(0.,0.,-40.));
#24650=CARTESIAN_POINT('',(-12.,-1.46957615897682E-15,-48.));
#24651=CARTESIAN_POINT('Origin',(0.,0.,-40.));
#24652=CARTESIAN_POINT('',(-29.,75.,-40.));
#24653=CARTESIAN_POINT('',(-29.,-75.,-40.));
#24654=CARTESIAN_POINT('',(-29.,35.,-40.));
#24655=CARTESIAN_POINT('',(24.,75.,-40.));
#24656=CARTESIAN_POINT('',(12.,75.,-40.));
#24657=CARTESIAN_POINT('',(24.,-75.,-40.));
#24658=CARTESIAN_POINT('',(24.,-70.,-40.));
#24659=CARTESIAN_POINT('',(-12.,-75.,-40.));
#24660=CARTESIAN_POINT('Ctrl Pts',(20.7937992825328,-52.9692229537457,-40.));
#24661=CARTESIAN_POINT('Ctrl Pts',(20.8868641368446,-52.9351794143205,-40.));
#24662=CARTESIAN_POINT('Ctrl Pts',(20.9778637119143,-52.8963692338032,-40.));
#24663=CARTESIAN_POINT('Ctrl Pts',(21.0665893040918,-52.8531201756825,-40.));
#24664=CARTESIAN_POINT('Ctrl Pts',(21.1572747443127,-52.8089157947528,-40.));
#24665=CARTESIAN_POINT('Ctrl Pts',(21.2455853007886,-52.7600736546262,-40.));
#24666=CARTESIAN_POINT('Ctrl Pts',(21.3312692081619,-52.7068981949415,-40.));
#24667=CARTESIAN_POINT('Ctrl Pts',(21.4136986594278,-52.6557424517338,-40.));
#24668=CARTESIAN_POINT('Ctrl Pts',(21.493697487121,-52.6005754396168,-40.));
#24669=CARTESIAN_POINT('Ctrl Pts',(21.5710085728572,-52.5416381747672,-40.));
#24670=CARTESIAN_POINT('Ctrl Pts',(21.6386557728764,-52.4900680680238,-40.));
#24671=CARTESIAN_POINT('Ctrl Pts',(21.7042448803152,-52.4356106648705,-40.));
#24672=CARTESIAN_POINT('Ctrl Pts',(21.7675790260379,-52.3784147256319,-40.));
#24673=CARTESIAN_POINT('Ctrl Pts',(21.7817032133443,-52.3656594235787,-40.));
#24674=CARTESIAN_POINT('Ctrl Pts',(21.7957178825123,-52.352765201296,-40.));
#24675=CARTESIAN_POINT('Ctrl Pts',(21.8096013024796,-52.3397522015173,-40.));
#24676=CARTESIAN_POINT('Ctrl Pts',(21.8820339673279,-52.2718606982811,-40.));
#24677=CARTESIAN_POINT('Ctrl Pts',(21.9510009955896,-52.2006479598651,-40.));
#24678=CARTESIAN_POINT('Ctrl Pts',(22.0162623182284,-52.1264040004137,-40.));
#24679=CARTESIAN_POINT('Ctrl Pts',(22.0811616750937,-52.0525718280842,-40.));
#24680=CARTESIAN_POINT('Ctrl Pts',(22.1423968052921,-51.975741170508,-40.));
#24681=CARTESIAN_POINT('Ctrl Pts',(22.1996880080389,-51.8961704744865,-40.));
#24682=CARTESIAN_POINT('Ctrl Pts',(22.2548537759022,-51.8195517558178,-40.));
#24683=CARTESIAN_POINT('Ctrl Pts',(22.3063629816812,-51.7403917956857,-40.));
#24684=CARTESIAN_POINT('Ctrl Pts',(22.3539210639109,-51.6589077247976,-40.));
#24685=CARTESIAN_POINT('Ctrl Pts',(22.3738667733396,-51.6247335629137,-40.));
#24686=CARTESIAN_POINT('Ctrl Pts',(22.3931169356095,-51.5901504976334,-40.));
#24687=CARTESIAN_POINT('Ctrl Pts',(22.4116472377174,-51.5551742475532,-40.));
#24688=CARTESIAN_POINT('Ctrl Pts',(22.4245263808776,-51.5308646529568,-40.));
#24689=CARTESIAN_POINT('Ctrl Pts',(22.4370577496651,-51.5063651203315,-40.));
#24690=CARTESIAN_POINT('Ctrl Pts',(22.4492327155052,-51.4816809210378,-40.));
#24691=CARTESIAN_POINT('Ctrl Pts',(22.4571463279311,-51.4656364254049,-40.));
#24692=CARTESIAN_POINT('Ctrl Pts',(22.4649104788499,-51.4495112843647,-40.));
#24693=CARTESIAN_POINT('Ctrl Pts',(22.4725126070347,-51.4333291644309,-40.));
#24694=CARTESIAN_POINT('Ctrl Pts',(22.5146350497842,-51.3436660590602,-40.));
#24695=CARTESIAN_POINT('Ctrl Pts',(22.5518581247129,-51.2521171179474,-40.));
#24696=CARTESIAN_POINT('Ctrl Pts',(22.583890412798,-51.1589539662439,-40.));
#24697=CARTESIAN_POINT('Ctrl Pts',(22.6137693466924,-51.0720536597857,-40.));
#24698=CARTESIAN_POINT('Ctrl Pts',(22.6391317579652,-50.9837480859561,-40.));
#24699=CARTESIAN_POINT('Ctrl Pts',(22.6596906010889,-50.894248963726,-40.));
#24700=CARTESIAN_POINT('Ctrl Pts',(22.6611722627557,-50.8877988236176,-40.));
#24701=CARTESIAN_POINT('Ctrl Pts',(22.6626289522036,-50.8813424830588,-40.));
#24702=CARTESIAN_POINT('Ctrl Pts',(22.6640605513299,-50.8748800209782,-40.));
#24703=CARTESIAN_POINT('Ctrl Pts',(22.6846661151432,-50.781863287207,-40.));
#24704=CARTESIAN_POINT('Ctrl Pts',(22.7000779522779,-50.6875773770759,-40.));
#24705=CARTESIAN_POINT('Ctrl Pts',(22.7103730991959,-50.5924307647528,-40.));
#24706=CARTESIAN_POINT('Ctrl Pts',(22.7161681739401,-50.5388733231281,-40.));
#24707=CARTESIAN_POINT('Ctrl Pts',(22.7203410991825,-50.4850433569999,-40.));
#24708=CARTESIAN_POINT('Ctrl Pts',(22.7228988539051,-50.4310163552227,-40.));
#24709=CARTESIAN_POINT('Ctrl Pts',(22.7235594196372,-50.4170633417972,-40.));
#24710=CARTESIAN_POINT('Ctrl Pts',(22.7241121360516,-50.4030977822463,-40.));
#24711=CARTESIAN_POINT('Ctrl Pts',(22.7245568821007,-50.389134351788,-40.));
#24712=CARTESIAN_POINT('Ctrl Pts',(22.7275259772316,-50.2959154160083,-40.));
#24713=CARTESIAN_POINT('Ctrl Pts',(22.7256954800801,-50.202635958812,-40.));
#24714=CARTESIAN_POINT('Ctrl Pts',(22.7192004014839,-50.1096716609144,-40.));
#24715=CARTESIAN_POINT('Ctrl Pts',(22.712694547308,-50.0165531317502,-40.));
#24716=CARTESIAN_POINT('Ctrl Pts',(22.7015082431827,-49.9237498276012,-40.));
#24717=CARTESIAN_POINT('Ctrl Pts',(22.6857262377269,-49.8316513834847,-40.));
#24718=CARTESIAN_POINT('Ctrl Pts',(22.6701704615353,-49.7408731368111,-40.));
#24719=CARTESIAN_POINT('Ctrl Pts',(22.6501493336621,-49.6507788422637,-40.));
#24720=CARTESIAN_POINT('Ctrl Pts',(22.6257009917886,-49.5617668173943,-40.));
#24721=CARTESIAN_POINT('Ctrl Pts',(22.6166026728921,-49.5286414712221,-40.));
#24722=CARTESIAN_POINT('Ctrl Pts',(22.6068908241138,-49.4956663271259,-40.));
#24723=CARTESIAN_POINT('Ctrl Pts',(22.5965660505575,-49.4628631797602,-40.));
#24724=CARTESIAN_POINT('Ctrl Pts',(22.5895982917682,-49.4407257045769,-40.));
#24725=CARTESIAN_POINT('Ctrl Pts',(22.5823513715533,-49.418666577747,-40.));
#24726=CARTESIAN_POINT('Ctrl Pts',(22.5748252991941,-49.3966927085346,-40.));
#24727=CARTESIAN_POINT('Ctrl Pts',(22.5698112245824,-49.3820531177256,-40.));
#24728=CARTESIAN_POINT('Ctrl Pts',(22.564673834239,-49.3674532968898,-40.));
#24729=CARTESIAN_POINT('Ctrl Pts',(22.5594172561101,-49.3529059808729,-40.));
#24730=CARTESIAN_POINT('Ctrl Pts',(22.527768723656,-49.2653202565106,-40.));
#24731=CARTESIAN_POINT('Ctrl Pts',(22.4917659891604,-49.1795245866921,-40.));
#24732=CARTESIAN_POINT('Ctrl Pts',(22.4514723792244,-49.0959295354423,-40.));
#24733=CARTESIAN_POINT('Ctrl Pts',(22.4212521717724,-49.033233247005,-40.));
#24734=CARTESIAN_POINT('Ctrl Pts',(22.3886173177637,-48.971775295946,-40.));
#24735=CARTESIAN_POINT('Ctrl Pts',(22.3535788443229,-48.9117442537613,-40.));
#24736=CARTESIAN_POINT('Ctrl Pts',(22.339751300498,-48.8880536706635,-40.));
#24737=CARTESIAN_POINT('Ctrl Pts',(22.3255492797115,-48.8645854808741,-40.));
#24738=CARTESIAN_POINT('Ctrl Pts',(22.3109729414368,-48.8413519730355,-40.));
#24739=CARTESIAN_POINT('Ctrl Pts',(22.30148687725,-48.8262319516358,-40.));
#24740=CARTESIAN_POINT('Ctrl Pts',(22.2918421409525,-48.8112113122026,-40.));
#24741=CARTESIAN_POINT('Ctrl Pts',(22.2820470683987,-48.796305696781,-40.));
#24742=CARTESIAN_POINT('Ctrl Pts',(22.2348460902122,-48.7244777828469,-40.));
#24743=CARTESIAN_POINT('Ctrl Pts',(22.1841115061796,-48.6552447286811,-40.));
#24744=CARTESIAN_POINT('Ctrl Pts',(22.1298762142565,-48.5889589949056,-40.));
#24745=CARTESIAN_POINT('Ctrl Pts',(22.0811918382369,-48.5294575250427,-40.));
#24746=CARTESIAN_POINT('Ctrl Pts',(22.0296860640005,-48.4723310319801,-40.));
#24747=CARTESIAN_POINT('Ctrl Pts',(21.9753623932829,-48.4178640169946,-40.));
#24748=CARTESIAN_POINT('Ctrl Pts',(21.9562793980543,-48.3987306673266,-40.));
#24749=CARTESIAN_POINT('Ctrl Pts',(21.9368485049632,-48.3799257876768,-40.));
#24750=CARTESIAN_POINT('Ctrl Pts',(21.917080287283,-48.3614538548662,-40.));
#24751=CARTESIAN_POINT('Ctrl Pts',(18.086534003335,-48.364012796625,-40.));
#24752=CARTESIAN_POINT('Ctrl Pts',(18.0249120467864,-48.4219223043634,-40.));
#24753=CARTESIAN_POINT('Ctrl Pts',(17.9666585528288,-48.4829816337199,-40.));
#24754=CARTESIAN_POINT('Ctrl Pts',(17.9117715849683,-48.5468061809736,-40.));
#24755=CARTESIAN_POINT('Ctrl Pts',(17.8554328022428,-48.6123189509525,-40.));
#24756=CARTESIAN_POINT('Ctrl Pts',(17.80264055923,-48.6807455909207,-40.));
#24757=CARTESIAN_POINT('Ctrl Pts',(17.7534182575179,-48.7517187155437,-40.));
#24758=CARTESIAN_POINT('Ctrl Pts',(17.7028584818801,-48.8246203299024,-40.));
#24759=CARTESIAN_POINT('Ctrl Pts',(17.6560647570637,-48.9002092533494,-40.));
#24760=CARTESIAN_POINT('Ctrl Pts',(17.6130964864067,-48.9781302762513,-40.));
#24761=CARTESIAN_POINT('Ctrl Pts',(17.5941949709457,-49.0124073229323,-40.));
#24762=CARTESIAN_POINT('Ctrl Pts',(17.5760341928623,-49.0471361452102,-40.));
#24763=CARTESIAN_POINT('Ctrl Pts',(17.5586216279894,-49.0822885783659,-40.));
#24764=CARTESIAN_POINT('Ctrl Pts',(17.5486910755096,-49.1023363475942,-40.));
#24765=CARTESIAN_POINT('Ctrl Pts',(17.539003909918,-49.1225219182463,-40.));
#24766=CARTESIAN_POINT('Ctrl Pts',(17.5295617519229,-49.1428402140162,-40.));
#24767=CARTESIAN_POINT('Ctrl Pts',(17.5210540661992,-49.1611476470141,-40.));
#24768=CARTESIAN_POINT('Ctrl Pts',(17.5127429170722,-49.1795685600238,-40.));
#24769=CARTESIAN_POINT('Ctrl Pts',(17.5046431538033,-49.1980674925815,-40.));
#24770=CARTESIAN_POINT('Ctrl Pts',(17.4680646114337,-49.2816086981564,-40.));
#24771=CARTESIAN_POINT('Ctrl Pts',(17.4357469371754,-49.3668332960487,-40.));
#24772=CARTESIAN_POINT('Ctrl Pts',(17.407715666334,-49.4533428436751,-40.));
#24773=CARTESIAN_POINT('Ctrl Pts',(17.3792231832159,-49.541275775409,-40.));
#24774=CARTESIAN_POINT('Ctrl Pts',(17.3551588225761,-49.6305370435133,-40.));
#24775=CARTESIAN_POINT('Ctrl Pts',(17.3355884709166,-49.72074532758,-40.));
#24776=CARTESIAN_POINT('Ctrl Pts',(17.3166112065531,-49.808219813695,-40.));
#24777=CARTESIAN_POINT('Ctrl Pts',(17.3018595365194,-49.8965857029214,-40.));
#24778=CARTESIAN_POINT('Ctrl Pts',(17.2914342702294,-49.9855171579377,-40.));
#24779=CARTESIAN_POINT('Ctrl Pts',(17.2870630038552,-50.0228057094342,-40.));
#24780=CARTESIAN_POINT('Ctrl Pts',(17.2834528721364,-50.0601938842692,-40.));
#24781=CARTESIAN_POINT('Ctrl Pts',(17.2806136391016,-50.097658280858,-40.));
#24782=CARTESIAN_POINT('Ctrl Pts',(17.2788322041313,-50.1211647649707,-40.));
#24783=CARTESIAN_POINT('Ctrl Pts',(17.2773542809704,-50.1447012611546,-40.));
#24784=CARTESIAN_POINT('Ctrl Pts',(17.2761825773384,-50.1682620220258,-40.));
#24785=CARTESIAN_POINT('Ctrl Pts',(17.2754967486151,-50.1820527504206,-40.));
#24786=CARTESIAN_POINT('Ctrl Pts',(17.2749161233417,-50.1958468418363,-40.));
#24787=CARTESIAN_POINT('Ctrl Pts',(17.2744412045133,-50.2096353105391,-40.));
#24788=CARTESIAN_POINT('Ctrl Pts',(17.2711047392125,-50.3065039639283,-40.));
#24789=CARTESIAN_POINT('Ctrl Pts',(17.2729755345434,-50.4032090699245,-40.));
#24790=CARTESIAN_POINT('Ctrl Pts',(17.2801185032147,-50.4993314325988,-40.));
#24791=CARTESIAN_POINT('Ctrl Pts',(17.2872614718861,-50.5954537952731,-40.));
#24792=CARTESIAN_POINT('Ctrl Pts',(17.2996761825003,-50.6909944574365,-40.));
#24793=CARTESIAN_POINT('Ctrl Pts',(17.3174800113019,-50.7855530099381,-40.));
#24794=CARTESIAN_POINT('Ctrl Pts',(17.3345350799895,-50.8761347957937,-40.));
#24795=CARTESIAN_POINT('Ctrl Pts',(17.3565353752775,-50.965816309671,-40.));
#24796=CARTESIAN_POINT('Ctrl Pts',(17.3832059787172,-51.0543578996475,-40.));
#24797=CARTESIAN_POINT('Ctrl Pts',(17.3920732513301,-51.0837956443795,-40.));
#24798=CARTESIAN_POINT('Ctrl Pts',(17.4014572042998,-51.1131073476298,-40.));
#24799=CARTESIAN_POINT('Ctrl Pts',(17.4113489818483,-51.1422840281894,-40.));
#24800=CARTESIAN_POINT('Ctrl Pts',(17.4206503121436,-51.1697191318883,-40.));
#24801=CARTESIAN_POINT('Ctrl Pts',(17.4304006578653,-51.1970348520032,-40.));
#24802=CARTESIAN_POINT('Ctrl Pts',(17.4405931275984,-51.2242235977629,-40.));
#24803=CARTESIAN_POINT('Ctrl Pts',(17.4457734086336,-51.2380421665416,-40.));
#24804=CARTESIAN_POINT('Ctrl Pts',(17.4510648730829,-51.2518197891935,-40.));
#24805=CARTESIAN_POINT('Ctrl Pts',(17.456464709971,-51.2655518102258,-40.));
#24806=CARTESIAN_POINT('Ctrl Pts',(17.490715740235,-51.3526536760249,-40.));
#24807=CARTESIAN_POINT('Ctrl Pts',(17.529340743901,-51.4379689505696,-40.));
#24808=CARTESIAN_POINT('Ctrl Pts',(17.5720094560872,-51.5212629155659,-40.));
#24809=CARTESIAN_POINT('Ctrl Pts',(17.6162431165096,-51.6076118296556,-40.));
#24810=CARTESIAN_POINT('Ctrl Pts',(17.6648226743584,-51.6917891759745,-40.));
#24811=CARTESIAN_POINT('Ctrl Pts',(17.7174360338155,-51.7735300066221,-40.));
#24812=CARTESIAN_POINT('Ctrl Pts',(17.7706149150164,-51.8561494395403,-40.));
#24813=CARTESIAN_POINT('Ctrl Pts',(17.827915194887,-51.9362805192111,-40.));
#24814=CARTESIAN_POINT('Ctrl Pts',(17.8890661284005,-52.013634320114,-40.));
#24815=CARTESIAN_POINT('Ctrl Pts',(17.9117391701769,-52.0423149282203,-40.));
#24816=CARTESIAN_POINT('Ctrl Pts',(17.9349420408772,-52.0706135254148,-40.));
#24817=CARTESIAN_POINT('Ctrl Pts',(17.9586625307952,-52.0985144997782,-40.));
#24818=CARTESIAN_POINT('Ctrl Pts',(17.9792967362419,-52.1227852648073,-40.));
#24819=CARTESIAN_POINT('Ctrl Pts',(18.0003226424187,-52.14675513991,-40.));
#24820=CARTESIAN_POINT('Ctrl Pts',(18.021732691825,-52.1704134738951,-40.));
#24821=CARTESIAN_POINT('Ctrl Pts',(18.0322751898043,-52.1820630471163,-40.));
#24822=CARTESIAN_POINT('Ctrl Pts',(18.0429077480725,-52.1936336023933,-40.));
#24823=CARTESIAN_POINT('Ctrl Pts',(18.053623710656,-52.205118119964,-40.));
#24824=CARTESIAN_POINT('Ctrl Pts',(18.1224864208474,-52.2789197032564,-40.));
#24825=CARTESIAN_POINT('Ctrl Pts',(18.1948566984041,-52.3492444555942,-40.));
#24826=CARTESIAN_POINT('Ctrl Pts',(18.2704248223711,-52.4158013759963,-40.));
#24827=CARTESIAN_POINT('Ctrl Pts',(18.3329140343801,-52.4708389935967,-40.));
#24828=CARTESIAN_POINT('Ctrl Pts',(18.397591040769,-52.5233001055479,-40.));
#24829=CARTESIAN_POINT('Ctrl Pts',(18.4643035650292,-52.5730066630244,-40.));
#24830=CARTESIAN_POINT('Ctrl Pts',(18.4874416953864,-52.5902465564215,-40.));
#24831=CARTESIAN_POINT('Ctrl Pts',(18.5108248507278,-52.6071549623375,-40.));
#24832=CARTESIAN_POINT('Ctrl Pts',(18.5344471800034,-52.6237239909632,-40.));
#24833=CARTESIAN_POINT('Ctrl Pts',(18.5545056123854,-52.6377932529926,-40.));
#24834=CARTESIAN_POINT('Ctrl Pts',(18.5747397224013,-52.6516198045524,-40.));
#24835=CARTESIAN_POINT('Ctrl Pts',(18.5951234326702,-52.6651840620199,-40.));
#24836=CARTESIAN_POINT('Ctrl Pts',(18.6800750900225,-52.7217147984472,-40.));
#24837=CARTESIAN_POINT('Ctrl Pts',(18.7676928928528,-52.773743896814,-40.));
#24838=CARTESIAN_POINT('Ctrl Pts',(18.857686322517,-52.8209628481135,-40.));
#24839=CARTESIAN_POINT('Ctrl Pts',(18.9406316584209,-52.8644837117052,-40.));
#24840=CARTESIAN_POINT('Ctrl Pts',(19.0255959104309,-52.9039185971562,-40.));
#24841=CARTESIAN_POINT('Ctrl Pts',(19.1123786609832,-52.9389975140129,-40.));
#24842=CARTESIAN_POINT('Ctrl Pts',(19.1428109210872,-52.951298699619,-40.));
#24843=CARTESIAN_POINT('Ctrl Pts',(19.173467007344,-52.9630639420694,-40.));
#24844=CARTESIAN_POINT('Ctrl Pts',(19.2043340224364,-52.9742969733088,-40.));
#24845=CARTESIAN_POINT('Ctrl Pts',(20.7937992825328,47.0307770462543,-40.));
#24846=CARTESIAN_POINT('Ctrl Pts',(20.8868641717184,47.0648205984365,-40.));
#24847=CARTESIAN_POINT('Ctrl Pts',(20.9778637814419,47.1036307868822,-40.));
#24848=CARTESIAN_POINT('Ctrl Pts',(21.0665894075274,47.1468798494389,-40.));
#24849=CARTESIAN_POINT('Ctrl Pts',(21.1572748647162,47.1910842262801,-40.));
#24850=CARTESIAN_POINT('Ctrl Pts',(21.245585438308,47.23992635686,-40.));
#24851=CARTESIAN_POINT('Ctrl Pts',(21.3312693624983,47.2931018031361,-40.));
#24852=CARTESIAN_POINT('Ctrl Pts',(21.4136988092816,47.3442575206223,-40.));
#24853=CARTESIAN_POINT('Ctrl Pts',(21.4936976334333,47.3994245014315,-40.));
#24854=CARTESIAN_POINT('Ctrl Pts',(21.5710087163438,47.4583617309845,-40.));
#24855=CARTESIAN_POINT('Ctrl Pts',(21.6386559138905,47.5099318068434,-40.));
#24856=CARTESIAN_POINT('Ctrl Pts',(21.7042450194051,47.5643891760566,-40.));
#24857=CARTESIAN_POINT('Ctrl Pts',(21.7675791636027,47.6215850793763,-40.));
#24858=CARTESIAN_POINT('Ctrl Pts',(21.7817033221825,47.6343403477839,-40.));
#24859=CARTESIAN_POINT('Ctrl Pts',(21.7957179630638,47.6472345357438,-40.));
#24860=CARTESIAN_POINT('Ctrl Pts',(21.8096013552832,47.6602475006384,-40.));
#24861=CARTESIAN_POINT('Ctrl Pts',(21.8820340261626,47.7281389632204,-40.));
#24862=CARTESIAN_POINT('Ctrl Pts',(21.9510010606037,47.7993516594532,-40.));
#24863=CARTESIAN_POINT('Ctrl Pts',(22.0162623892813,47.8735955768846,-40.));
#24864=CARTESIAN_POINT('Ctrl Pts',(22.0811617452106,47.9474276995307,-40.));
#24865=CARTESIAN_POINT('Ctrl Pts',(22.1423968751173,48.0242583069407,-40.));
#24866=CARTESIAN_POINT('Ctrl Pts',(22.1996880780212,48.1038289540701,-40.));
#24867=CARTESIAN_POINT('Ctrl Pts',(22.2548538529654,48.1804476352851,-40.));
#24868=CARTESIAN_POINT('Ctrl Pts',(22.306363065324,48.2596075597805,-40.));
#24869=CARTESIAN_POINT('Ctrl Pts',(22.3539211533538,48.3410915983807,-40.));
#24870=CARTESIAN_POINT('Ctrl Pts',(22.3738668610994,48.3752657396715,-40.));
#24871=CARTESIAN_POINT('Ctrl Pts',(22.3931170218359,48.4098487847799,-40.));
#24872=CARTESIAN_POINT('Ctrl Pts',(22.4116473225538,48.4448250152362,-40.));
#24873=CARTESIAN_POINT('Ctrl Pts',(22.4245264566452,48.4691345808995,-40.));
#24874=CARTESIAN_POINT('Ctrl Pts',(22.4370578168709,48.4936340846175,-40.));
#24875=CARTESIAN_POINT('Ctrl Pts',(22.4492327746705,48.5183182550832,-40.));
#24876=CARTESIAN_POINT('Ctrl Pts',(22.4571464007594,48.5343627702754,-40.));
#24877=CARTESIAN_POINT('Ctrl Pts',(22.4649105648593,48.5504879313153,-40.));
#24878=CARTESIAN_POINT('Ctrl Pts',(22.4725127056892,48.5666700716157,-40.));
#24879=CARTESIAN_POINT('Ctrl Pts',(22.5146351538768,48.6563331522688,-40.));
#24880=CARTESIAN_POINT('Ctrl Pts',(22.5518582329025,48.7478820741464,-40.));
#24881=CARTESIAN_POINT('Ctrl Pts',(22.5838905234092,48.8410452138574,-40.));
#24882=CARTESIAN_POINT('Ctrl Pts',(22.6137694553261,48.9279454968081,-40.));
#24883=CARTESIAN_POINT('Ctrl Pts',(22.6391318644434,49.0162510530317,-40.));
#24884=CARTESIAN_POINT('Ctrl Pts',(22.6596907050679,49.1057501651513,-40.));
#24885=CARTESIAN_POINT('Ctrl Pts',(22.6611723696795,49.1122003181352,-40.));
#24886=CARTESIAN_POINT('Ctrl Pts',(22.6626290619652,49.1186566716347,-40.));
#24887=CARTESIAN_POINT('Ctrl Pts',(22.6640606638213,49.1251191467213,-40.));
#24888=CARTESIAN_POINT('Ctrl Pts',(22.6846662259577,49.2181358827524,-40.));
#24889=CARTESIAN_POINT('Ctrl Pts',(22.7000780597252,49.3124218036144,-40.));
#24890=CARTESIAN_POINT('Ctrl Pts',(22.7103732018717,49.4075684336347,-40.));
#24891=CARTESIAN_POINT('Ctrl Pts',(22.7161682730423,49.4611258770159,-40.));
#24892=CARTESIAN_POINT('Ctrl Pts',(22.7203411947628,49.514955847025,-40.));
#24893=CARTESIAN_POINT('Ctrl Pts',(22.7228989460627,49.5689828545753,-40.));
#24894=CARTESIAN_POINT('Ctrl Pts',(22.7235595110321,49.5829358720506,-40.));
#24895=CARTESIAN_POINT('Ctrl Pts',(22.7241122266512,49.5969014357913,-40.));
#24896=CARTESIAN_POINT('Ctrl Pts',(22.7245569718737,49.61086487056,-40.));
#24897=CARTESIAN_POINT('Ctrl Pts',(22.7275260613783,49.7040838317261,-40.));
#24898=CARTESIAN_POINT('Ctrl Pts',(22.7256955575492,49.797363319751,-40.));
#24899=CARTESIAN_POINT('Ctrl Pts',(22.7192004715102,49.8903276524339,-40.));
#24900=CARTESIAN_POINT('Ctrl Pts',(22.7126946099576,49.9834462153179,-40.));
#24901=CARTESIAN_POINT('Ctrl Pts',(22.7015082978001,50.0762495571672,-40.));
#24902=CARTESIAN_POINT('Ctrl Pts',(22.6857262839338,50.1683480415187,-40.));
#24903=CARTESIAN_POINT('Ctrl Pts',(22.6701705009221,50.2591263192725,-40.));
#24904=CARTESIAN_POINT('Ctrl Pts',(22.6501493667039,50.3492206474941,-40.));
#24905=CARTESIAN_POINT('Ctrl Pts',(22.6257010192203,50.4382327073517,-40.));
#24906=CARTESIAN_POINT('Ctrl Pts',(22.6166027019945,50.4713580528603,-40.));
#24907=CARTESIAN_POINT('Ctrl Pts',(22.6068908554958,50.5043331965987,-40.));
#24908=CARTESIAN_POINT('Ctrl Pts',(22.5965660848416,50.5371363438728,-40.));
#24909=CARTESIAN_POINT('Ctrl Pts',(22.5895984002548,50.5592735894651,-40.));
#24910=CARTESIAN_POINT('Ctrl Pts',(22.5823515603147,50.5813324884496,-40.));
#24911=CARTESIAN_POINT('Ctrl Pts',(22.5748255743073,50.6033061317659,-40.));
#24912=CARTESIAN_POINT('Ctrl Pts',(22.5698115155151,50.6179456938587,-40.));
#24913=CARTESIAN_POINT('Ctrl Pts',(22.5646741414619,50.6325454866863,-40.));
#24914=CARTESIAN_POINT('Ctrl Pts',(22.5594175802594,50.647092774896,-40.));
#24915=CARTESIAN_POINT('Ctrl Pts',(22.5277690412619,50.734678631977,-40.));
#24916=CARTESIAN_POINT('Ctrl Pts',(22.4917662925164,50.8204744325049,-40.));
#24917=CARTESIAN_POINT('Ctrl Pts',(22.4514726612107,50.9040696099987,-40.));
#24918=CARTESIAN_POINT('Ctrl Pts',(22.4212524377315,50.9667659931192,-40.));
#24919=CARTESIAN_POINT('Ctrl Pts',(22.3886175636867,51.028224036349,-40.));
#24920=CARTESIAN_POINT('Ctrl Pts',(22.353579066392,51.0882551670977,-40.));
#24921=CARTESIAN_POINT('Ctrl Pts',(22.3397516120993,51.1119456156231,-40.));
#24922=CARTESIAN_POINT('Ctrl Pts',(22.325549685609,51.1354136734597,-40.));
#24923=CARTESIAN_POINT('Ctrl Pts',(22.310973446402,51.1586470521603,-40.));
#24924=CARTESIAN_POINT('Ctrl Pts',(22.3014872869241,51.1737672441684,-40.));
#24925=CARTESIAN_POINT('Ctrl Pts',(22.291842451823,51.1887880523519,-40.));
#24926=CARTESIAN_POINT('Ctrl Pts',(22.2820472773129,51.2036938339823,-40.));
#24927=CARTESIAN_POINT('Ctrl Pts',(22.2348463161877,51.2755217752358,-40.));
#24928=CARTESIAN_POINT('Ctrl Pts',(22.1841117513564,51.3447548552043,-40.));
#24929=CARTESIAN_POINT('Ctrl Pts',(22.1298764810566,51.4110406123198,-40.));
#24930=CARTESIAN_POINT('Ctrl Pts',(22.0811919981176,51.4705422575325,-40.));
#24931=CARTESIAN_POINT('Ctrl Pts',(22.0296861042788,51.5276689116495,-40.));
#24932=CARTESIAN_POINT('Ctrl Pts',(21.9753623015053,51.5821360704448,-40.));
#24933=CARTESIAN_POINT('Ctrl Pts',(21.9562793052671,51.6012694251315,-40.));
#24934=CARTESIAN_POINT('Ctrl Pts',(21.9368484112827,51.6200743092308,-40.));
#24935=CARTESIAN_POINT('Ctrl Pts',(21.9170801928212,51.6385462459494,-40.));
#24936=CARTESIAN_POINT('Ctrl Pts',(18.086534003335,51.635987203375,-40.));
#24937=CARTESIAN_POINT('Ctrl Pts',(18.0249120118231,51.5780776627796,-40.));
#24938=CARTESIAN_POINT('Ctrl Pts',(17.9666584811321,51.517018302892,-40.));
#24939=CARTESIAN_POINT('Ctrl Pts',(17.9117714759284,51.4531937268802,-40.));
#24940=CARTESIAN_POINT('Ctrl Pts',(17.8554326587671,51.387680931912,-40.));
#24941=CARTESIAN_POINT('Ctrl Pts',(17.8026403801833,51.3192542692251,-40.));
#24942=CARTESIAN_POINT('Ctrl Pts',(17.753418042989,51.2482811234662,-40.));
#24943=CARTESIAN_POINT('Ctrl Pts',(17.7028582625625,51.1753795330443,-40.));
#24944=CARTESIAN_POINT('Ctrl Pts',(17.6560645283358,51.0997906385659,-40.));
#24945=CARTESIAN_POINT('Ctrl Pts',(17.6130962448594,51.0218696482571,-40.));
#24946=CARTESIAN_POINT('Ctrl Pts',(17.5941947509285,50.9875926651839,-40.));
#24947=CARTESIAN_POINT('Ctrl Pts',(17.5760339915857,50.9528639085148,-40.));
#24948=CARTESIAN_POINT('Ctrl Pts',(17.5586214427303,50.9177115427326,-40.));
#24949=CARTESIAN_POINT('Ctrl Pts',(17.5486908909937,50.8976637949869,-40.));
#24950=CARTESIAN_POINT('Ctrl Pts',(17.5390037256709,50.8774782461587,-40.));
#24951=CARTESIAN_POINT('Ctrl Pts',(17.5295615674849,50.857159972524,-40.));
#24952=CARTESIAN_POINT('Ctrl Pts',(17.5210538764243,50.8388525483564,-40.));
#24953=CARTESIAN_POINT('Ctrl Pts',(17.5127427218279,50.8204316443034,-40.));
#24954=CARTESIAN_POINT('Ctrl Pts',(17.5046429529782,50.801932720795,-40.));
#24955=CARTESIAN_POINT('Ctrl Pts',(17.4680643678851,50.7183915160718,-40.));
#24956=CARTESIAN_POINT('Ctrl Pts',(17.4357466526846,50.6331669193299,-40.));
#24957=CARTESIAN_POINT('Ctrl Pts',(17.4077153439705,50.54665737229,-40.));
#24958=CARTESIAN_POINT('Ctrl Pts',(17.3792228278356,50.4587244580619,-40.));
#24959=CARTESIAN_POINT('Ctrl Pts',(17.3551584356458,50.3694632073917,-40.));
#24960=CARTESIAN_POINT('Ctrl Pts',(17.335588055227,50.2792549395642,-40.));
#24961=CARTESIAN_POINT('Ctrl Pts',(17.3166107688801,50.191780496411,-40.));
#24962=CARTESIAN_POINT('Ctrl Pts',(17.3018590768574,50.1034146495783,-40.));
#24963=CARTESIAN_POINT('Ctrl Pts',(17.2914337897018,50.0144832350641,-40.));
#24964=CARTESIAN_POINT('Ctrl Pts',(17.2870625173661,49.9771947243273,-40.));
#24965=CARTESIAN_POINT('Ctrl Pts',(17.2834523789126,49.9398065900466,-40.));
#24966=CARTESIAN_POINT('Ctrl Pts',(17.2806131384336,49.9023422336642,-40.));
#24967=CARTESIAN_POINT('Ctrl Pts',(17.2788316977985,49.8788357616608,-40.));
#24968=CARTESIAN_POINT('Ctrl Pts',(17.2773537690321,49.8552992774157,-40.));
#24969=CARTESIAN_POINT('Ctrl Pts',(17.2761820598737,49.8317385282873,-40.));
#24970=CARTESIAN_POINT('Ctrl Pts',(17.2754962276114,49.8179478006491,-40.));
#24971=CARTESIAN_POINT('Ctrl Pts',(17.2749155989209,49.8041537099236,-40.));
#24972=CARTESIAN_POINT('Ctrl Pts',(17.2744406768029,49.7903652418327,-40.));
#24973=CARTESIAN_POINT('Ctrl Pts',(17.2711041892475,49.6934966175952,-40.));
#24974=CARTESIAN_POINT('Ctrl Pts',(17.2729749659192,49.5967915369097,-40.));
#24975=CARTESIAN_POINT('Ctrl Pts',(17.2801179208972,49.5006691942515,-40.));
#24976=CARTESIAN_POINT('Ctrl Pts',(17.2872608758751,49.4045468515933,-40.));
#24977=CARTESIAN_POINT('Ctrl Pts',(17.2996755777587,49.3090062041544,-40.));
#24978=CARTESIAN_POINT('Ctrl Pts',(17.3174794041662,49.214447659627,-40.));
#24979=CARTESIAN_POINT('Ctrl Pts',(17.334534466704,49.1238659018917,-40.));
#24980=CARTESIAN_POINT('Ctrl Pts',(17.3565347594197,49.0341844095363,-40.));
#24981=CARTESIAN_POINT('Ctrl Pts',(17.3832053630372,48.9456428353218,-40.));
#24982=CARTESIAN_POINT('Ctrl Pts',(17.3920726307165,48.9162051124052,-40.));
#24983=CARTESIAN_POINT('Ctrl Pts',(17.4014565784749,48.8868934301911,-40.));
#24984=CARTESIAN_POINT('Ctrl Pts',(17.4113483505188,48.8577167699025,-40.));
#24985=CARTESIAN_POINT('Ctrl Pts',(17.4206496316742,48.8302818149405,-40.));
#24986=CARTESIAN_POINT('Ctrl Pts',(17.4303999237523,48.8029662417575,-40.));
#24987=CARTESIAN_POINT('Ctrl Pts',(17.4405923354209,48.7757776410274,-40.));
#24988=CARTESIAN_POINT('Ctrl Pts',(17.4457726757404,48.7619589090953,-40.));
#24989=CARTESIAN_POINT('Ctrl Pts',(17.4510642023782,48.7481811235908,-40.));
#24990=CARTESIAN_POINT('Ctrl Pts',(17.45646410399,48.7344489408886,-40.));
#24991=CARTESIAN_POINT('Ctrl Pts',(17.4907151349945,48.6473470917609,-40.));
#24992=CARTESIAN_POINT('Ctrl Pts',(17.5293401405757,48.5620318281544,-40.));
#24993=CARTESIAN_POINT('Ctrl Pts',(17.5720088551052,48.4787378691761,-40.));
#24994=CARTESIAN_POINT('Ctrl Pts',(17.6162425271352,48.3923889434079,-40.));
#24995=CARTESIAN_POINT('Ctrl Pts',(17.6648220988544,48.3082115810238,-40.));
#24996=CARTESIAN_POINT('Ctrl Pts',(17.7174354734165,48.2264707309132,-40.));
#24997=CARTESIAN_POINT('Ctrl Pts',(17.7706143764448,48.1438512681309,-40.));
#24998=CARTESIAN_POINT('Ctrl Pts',(17.8279146804215,48.0637201557371,-40.));
#24999=CARTESIAN_POINT('Ctrl Pts',(17.8890656391782,47.9863663203166,-40.));
#25000=CARTESIAN_POINT('Ctrl Pts',(17.9117386404853,47.9576857624437,-40.));
#25001=CARTESIAN_POINT('Ctrl Pts',(17.9349414685443,47.9293872135568,-40.));
#25002=CARTESIAN_POINT('Ctrl Pts',(17.9586619136712,47.9014862855243,-40.));
#25003=CARTESIAN_POINT('Ctrl Pts',(17.9792958092928,47.8772158793964,-40.));
#25004=CARTESIAN_POINT('Ctrl Pts',(18.0003213937351,47.8532463538005,-40.));
#25005=CARTESIAN_POINT('Ctrl Pts',(18.0217311098025,47.8295883594692,-40.));
#25006=CARTESIAN_POINT('Ctrl Pts',(18.0322734470095,47.8179389497762,-40.));
#25007=CARTESIAN_POINT('Ctrl Pts',(18.0429058427987,47.8063685545443,-40.));
#25008=CARTESIAN_POINT('Ctrl Pts',(18.0536216401407,47.7948841947313,-40.));
#25009=CARTESIAN_POINT('Ctrl Pts',(18.1224843127581,47.7210825274562,-40.));
#25010=CARTESIAN_POINT('Ctrl Pts',(18.1948545546408,47.6507576872252,-40.));
#25011=CARTESIAN_POINT('Ctrl Pts',(18.2704226433781,47.5842006758549,-40.));
#25012=CARTESIAN_POINT('Ctrl Pts',(18.332912008939,47.5291628221304,-40.));
#25013=CARTESIAN_POINT('Ctrl Pts',(18.3975891819685,47.4767014870064,-40.));
#25014=CARTESIAN_POINT('Ctrl Pts',(18.4643018838579,47.4269947212888,-40.));
#25015=CARTESIAN_POINT('Ctrl Pts',(18.487439448026,47.40975522343,-40.));
#25016=CARTESIAN_POINT('Ctrl Pts',(18.5108220252072,47.3928471968628,-40.));
#25017=CARTESIAN_POINT('Ctrl Pts',(18.534443764743,47.3762785308372,-40.));
#25018=CARTESIAN_POINT('Ctrl Pts',(18.5545032544247,47.3622084838503,-40.));
#25019=CARTESIAN_POINT('Ctrl Pts',(18.5747384411063,47.3483811726599,-40.));
#25020=CARTESIAN_POINT('Ctrl Pts',(18.5951232442218,47.3348161834234,-40.));
#25021=CARTESIAN_POINT('Ctrl Pts',(18.6800749291183,47.2782854097527,-40.));
#25022=CARTESIAN_POINT('Ctrl Pts',(18.7676927569613,47.2262562766525,-40.));
#25023=CARTESIAN_POINT('Ctrl Pts',(18.8576862078851,47.1790372942811,-40.));
#25024=CARTESIAN_POINT('Ctrl Pts',(18.9406316367841,47.1355163635382,-40.));
#25025=CARTESIAN_POINT('Ctrl Pts',(19.0255959821725,47.0960814212715,-40.));
#25026=CARTESIAN_POINT('Ctrl Pts',(19.1123788250024,47.0610024595712,-40.));
#25027=CARTESIAN_POINT('Ctrl Pts',(19.1428110902835,47.0487012692271,-40.));
#25028=CARTESIAN_POINT('Ctrl Pts',(19.1734671811829,47.0369360225547,-40.));
#25029=CARTESIAN_POINT('Ctrl Pts',(19.2043342004084,47.0257029875827,-40.));
#25030=CARTESIAN_POINT('Ctrl Pts',(-19.2062007174672,47.0307770462543,-40.));
#25031=CARTESIAN_POINT('Ctrl Pts',(-19.113135789485,47.0648206126285,-40.));
#25032=CARTESIAN_POINT('Ctrl Pts',(-19.0221361412093,47.1036308098944,-40.));
#25033=CARTESIAN_POINT('Ctrl Pts',(-18.9334104774012,47.1468798773863,-40.));
#25034=CARTESIAN_POINT('Ctrl Pts',(-18.8427250013391,47.1910842496773,-40.));
#25035=CARTESIAN_POINT('Ctrl Pts',(-18.7544144087091,47.2399263696347,-40.));
#25036=CARTESIAN_POINT('Ctrl Pts',(-18.6687304658127,47.2931018009917,-40.));
#25037=CARTESIAN_POINT('Ctrl Pts',(-18.5863010240148,47.3442574898636,-40.));
#25038=CARTESIAN_POINT('Ctrl Pts',(-18.5063022038013,47.3994244358441,-40.));
#25039=CARTESIAN_POINT('Ctrl Pts',(-18.4289911240327,47.4583616261313,-40.));
#25040=CARTESIAN_POINT('Ctrl Pts',(-18.3613439292353,47.5099316676326,-40.));
#25041=CARTESIAN_POINT('Ctrl Pts',(-18.29575482586,47.5643889990892,-40.));
#25042=CARTESIAN_POINT('Ctrl Pts',(-18.2324206833574,47.6215848624513,-40.));
#25043=CARTESIAN_POINT('Ctrl Pts',(-18.2182965567006,47.6343400934602,-40.));
#25044=CARTESIAN_POINT('Ctrl Pts',(-18.2042819472534,47.6472342432689,-40.));
#25045=CARTESIAN_POINT('Ctrl Pts',(-18.1903985858695,47.6602471693883,-40.));
#25046=CARTESIAN_POINT('Ctrl Pts',(-18.1179659082848,47.7281385867458,-40.));
#25047=CARTESIAN_POINT('Ctrl Pts',(-18.0489988669731,47.7993512360535,-40.));
#25048=CARTESIAN_POINT('Ctrl Pts',(-17.9837375315815,47.8735951067416,-40.));
#25049=CARTESIAN_POINT('Ctrl Pts',(-17.9188381766974,47.9474271741188,-40.));
#25050=CARTESIAN_POINT('Ctrl Pts',(-17.8576030471192,48.024257725723,-40.));
#25051=CARTESIAN_POINT('Ctrl Pts',(-17.8003118440444,48.1038283184647,-40.));
#25052=CARTESIAN_POINT('Ctrl Pts',(-17.7451460612301,48.1804469580116,-40.));
#25053=CARTESIAN_POINT('Ctrl Pts',(-17.6936368415585,48.2596068428605,-40.));
#25054=CARTESIAN_POINT('Ctrl Pts',(-17.6460787470823,48.34109084554,-40.));
#25055=CARTESIAN_POINT('Ctrl Pts',(-17.6261330412026,48.3752649639367,-40.));
#25056=CARTESIAN_POINT('Ctrl Pts',(-17.6068828821661,48.4098479866198,-40.));
#25057=CARTESIAN_POINT('Ctrl Pts',(-17.5883525829892,48.444824195261,-40.));
#25058=CARTESIAN_POINT('Ctrl Pts',(-17.5754734589502,48.4691337288093,-40.));
#25059=CARTESIAN_POINT('Ctrl Pts',(-17.5629421082152,48.4936332004423,-40.));
#25060=CARTESIAN_POINT('Ctrl Pts',(-17.5507671593283,48.5183173389123,-40.));
#25061=CARTESIAN_POINT('Ctrl Pts',(-17.5428535180885,48.5343618757708,-40.));
#25062=CARTESIAN_POINT('Ctrl Pts',(-17.5350893393722,48.5504870589659,-40.));
#25063=CARTESIAN_POINT('Ctrl Pts',(-17.5274871845203,48.5666692218289,-40.));
#25064=CARTESIAN_POINT('Ctrl Pts',(-17.485364730287,48.6563322749854,-40.));
#25065=CARTESIAN_POINT('Ctrl Pts',(-17.4481416467071,48.7478811754663,-40.));
#25066=CARTESIAN_POINT('Ctrl Pts',(-17.4161093535095,48.8410443018387,-40.));
#25067=CARTESIAN_POINT('Ctrl Pts',(-17.3862304237933,48.927944558647,-40.));
#25068=CARTESIAN_POINT('Ctrl Pts',(-17.3608680170749,49.0162500952945,-40.));
#25069=CARTESIAN_POINT('Ctrl Pts',(-17.340309179232,49.1057491961777,-40.));
#25070=CARTESIAN_POINT('Ctrl Pts',(-17.338827511346,49.112199363479,-40.));
#25071=CARTESIAN_POINT('Ctrl Pts',(-17.337370815905,49.1186557313683,-40.));
#25072=CARTESIAN_POINT('Ctrl Pts',(-17.3359392110137,49.1251182209172,-40.));
#25073=CARTESIAN_POINT('Ctrl Pts',(-17.3153336507421,49.2181349594804,-40.));
#25074=CARTESIAN_POINT('Ctrl Pts',(-17.2999218207206,49.3124208922995,-40.));
#25075=CARTESIAN_POINT('Ctrl Pts',(-17.2896266838834,49.4075675420277,-40.));
#25076=CARTESIAN_POINT('Ctrl Pts',(-17.2838316166888,49.4611249873763,-40.));
#25077=CARTESIAN_POINT('Ctrl Pts',(-17.2796586988872,49.5149549617163,-40.));
#25078=CARTESIAN_POINT('Ctrl Pts',(-17.2771009513959,49.568981975703,-40.));
#25079=CARTESIAN_POINT('Ctrl Pts',(-17.2764403872718,49.5829349977661,-40.));
#25080=CARTESIAN_POINT('Ctrl Pts',(-17.2758876725352,49.5969005662504,-40.));
#25081=CARTESIAN_POINT('Ctrl Pts',(-17.2754429282314,49.6108640058968,-40.));
#25082=CARTESIAN_POINT('Ctrl Pts',(-17.2724738449968,49.7040829953194,-40.));
#25083=CARTESIAN_POINT('Ctrl Pts',(-17.2743043562655,49.7973625176552,-40.));
#25084=CARTESIAN_POINT('Ctrl Pts',(-17.2807994505954,49.8903268890503,-40.));
#25085=CARTESIAN_POINT('Ctrl Pts',(-17.287305320365,49.9834454894571,-40.));
#25086=CARTESIAN_POINT('Ctrl Pts',(-17.2984916414684,50.0762488732571,-40.));
#25087=CARTESIAN_POINT('Ctrl Pts',(-17.3142736647013,50.1683474023781,-40.));
#25088=CARTESIAN_POINT('Ctrl Pts',(-17.3298294553088,50.2591257147104,-40.));
#25089=CARTESIAN_POINT('Ctrl Pts',(-17.3498505965932,50.3492200803956,-40.));
#25090=CARTESIAN_POINT('Ctrl Pts',(-17.3742989503246,50.4382321791774,-40.));
#25091=CARTESIAN_POINT('Ctrl Pts',(-17.3833972657162,50.4713575240284,-40.));
#25092=CARTESIAN_POINT('Ctrl Pts',(-17.3931091097062,50.5043326674485,-40.));
#25093=CARTESIAN_POINT('Ctrl Pts',(-17.4034338771622,50.5371358146991,-40.));
#25094=CARTESIAN_POINT('Ctrl Pts',(-17.4104014795578,50.5592728060012,-40.));
#25095=CARTESIAN_POINT('Ctrl Pts',(-17.4176482305802,50.5813314526292,-40.));
#25096=CARTESIAN_POINT('Ctrl Pts',(-17.4251741209375,50.6033048457485,-40.));
#25097=CARTESIAN_POINT('Ctrl Pts',(-17.430188162207,50.6179443760499,-40.));
#25098=CARTESIAN_POINT('Ctrl Pts',(-17.4353255182162,50.6325441378708,-40.));
#25099=CARTESIAN_POINT('Ctrl Pts',(-17.4405820606693,50.6470913952962,-40.));
#25100=CARTESIAN_POINT('Ctrl Pts',(-17.472230606961,50.7346773996235,-40.));
#25101=CARTESIAN_POINT('Ctrl Pts',(-17.5082333715373,50.8204733451689,-40.));
#25102=CARTESIAN_POINT('Ctrl Pts',(-17.548527026559,50.9040686627239,-40.));
#25103=CARTESIAN_POINT('Ctrl Pts',(-17.5787472678254,50.9667651508901,-40.));
#25104=CARTESIAN_POINT('Ctrl Pts',(-17.6113821640973,51.0282232963771,-40.));
#25105=CARTESIAN_POINT('Ctrl Pts',(-17.6464206878467,51.0882545253784,-40.));
#25106=CARTESIAN_POINT('Ctrl Pts',(-17.6602480429408,51.1119448248349,-40.));
#25107=CARTESIAN_POINT('Ctrl Pts',(-17.6744498649535,51.1354127365043,-40.));
#25108=CARTESIAN_POINT('Ctrl Pts',(-17.6890259943953,51.1586459721552,-40.));
#25109=CARTESIAN_POINT('Ctrl Pts',(-17.6985122595296,51.1737663533366,-40.));
#25110=CARTESIAN_POINT('Ctrl Pts',(-17.708157204181,51.1887873486326,-40.));
#25111=CARTESIAN_POINT('Ctrl Pts',(-17.7179524917366,51.2036933145573,-40.));
#25112=CARTESIAN_POINT('Ctrl Pts',(-17.7651534339424,51.275521286134,-40.));
#25113=CARTESIAN_POINT('Ctrl Pts',(-17.8158879774711,51.3447543947345,-40.));
#25114=CARTESIAN_POINT('Ctrl Pts',(-17.8701232237717,51.4110401777378,-40.));
#25115=CARTESIAN_POINT('Ctrl Pts',(-17.9188078251789,51.4705420173089,-40.));
#25116=CARTESIAN_POINT('Ctrl Pts',(-17.9703138515323,51.5276688499289,-40.));
#25117=CARTESIAN_POINT('Ctrl Pts',(-18.0246378006122,51.5821361680994,-40.));
#25118=CARTESIAN_POINT('Ctrl Pts',(-18.0437207979735,51.6012695283674,-40.));
#25119=CARTESIAN_POINT('Ctrl Pts',(-18.0631516929516,51.6200744174145,-40.));
#25120=CARTESIAN_POINT('Ctrl Pts',(-18.0829199122823,51.6385463584782,-40.));
#25121=CARTESIAN_POINT('Ctrl Pts',(-21.913465996665,51.635987203375,-40.));
#25122=CARTESIAN_POINT('Ctrl Pts',(-21.9750878942349,51.5780777510621,-40.));
#25123=CARTESIAN_POINT('Ctrl Pts',(-22.0333413262282,51.5170184732071,-40.));
#25124=CARTESIAN_POINT('Ctrl Pts',(-22.0882282310954,51.4531939744632,-40.));
#25125=CARTESIAN_POINT('Ctrl Pts',(-22.1445669557314,51.3876812466377,-40.));
#25126=CARTESIAN_POINT('Ctrl Pts',(-22.1973591387396,51.3192546449921,-40.));
#25127=CARTESIAN_POINT('Ctrl Pts',(-22.2465813805965,51.2482815560211,-40.));
#25128=CARTESIAN_POINT('Ctrl Pts',(-22.2971411481564,51.175379901281,-40.));
#25129=CARTESIAN_POINT('Ctrl Pts',(-22.3439348570983,51.0997909289638,-40.));
#25130=CARTESIAN_POINT('Ctrl Pts',(-22.3869031061299,51.0218698510766,-40.));
#25131=CARTESIAN_POINT('Ctrl Pts',(-22.4058046579096,50.9875926970939,-40.));
#25132=CARTESIAN_POINT('Ctrl Pts',(-22.4239654676059,50.9528637641387,-40.));
#25133=CARTESIAN_POINT('Ctrl Pts',(-22.4413780594982,50.9177112173285,-40.));
#25134=CARTESIAN_POINT('Ctrl Pts',(-22.4513086132313,50.8976634118604,-40.));
#25135=CARTESIAN_POINT('Ctrl Pts',(-22.4609957792757,50.8774778043928,-40.));
#25136=CARTESIAN_POINT('Ctrl Pts',(-22.4704379369484,50.8571594712822,-40.));
#25137=CARTESIAN_POINT('Ctrl Pts',(-22.4789456136821,50.8388520233592,-40.));
#25138=CARTESIAN_POINT('Ctrl Pts',(-22.4872567535947,50.8204310952107,-40.));
#25139=CARTESIAN_POINT('Ctrl Pts',(-22.4953565074608,50.801932147358,-40.));
#25140=CARTESIAN_POINT('Ctrl Pts',(-22.5319349777541,50.7183909403439,-40.));
#25141=CARTESIAN_POINT('Ctrl Pts',(-22.5642525829406,50.6331663405078,-40.));
#25142=CARTESIAN_POINT('Ctrl Pts',(-22.5922837898878,50.5466567918879,-40.));
#25143=CARTESIAN_POINT('Ctrl Pts',(-22.6207762173038,50.4587238306182,-40.));
#25144=CARTESIAN_POINT('Ctrl Pts',(-22.6448405247148,50.3694625330981,-40.));
#25145=CARTESIAN_POINT('Ctrl Pts',(-22.6644108278527,50.2792542216303,-40.));
#25146=CARTESIAN_POINT('Ctrl Pts',(-22.6833880551243,50.1917796630377,-40.));
#25147=CARTESIAN_POINT('Ctrl Pts',(-22.6981396880567,50.1034137022911,-40.));
#25148=CARTESIAN_POINT('Ctrl Pts',(-22.7085649191393,50.0144821789446,-40.));
#25149=CARTESIAN_POINT('Ctrl Pts',(-22.712936175452,49.9771935586975,-40.));
#25150=CARTESIAN_POINT('Ctrl Pts',(-22.7165462958052,49.9398053154584,-40.));
#25151=CARTESIAN_POINT('Ctrl Pts',(-22.719385516278,49.9023408510524,-40.));
#25152=CARTESIAN_POINT('Ctrl Pts',(-22.7211669416888,49.878834346527,-40.));
#25153=CARTESIAN_POINT('Ctrl Pts',(-22.7226448553907,49.8552978302179,-40.));
#25154=CARTESIAN_POINT('Ctrl Pts',(-22.7238165496974,49.8317370495525,-40.));
#25155=CARTESIAN_POINT('Ctrl Pts',(-22.7245023724455,49.817946319965,-40.));
#25156=CARTESIAN_POINT('Ctrl Pts',(-22.7250829919506,49.8041522274683,-40.));
#25157=CARTESIAN_POINT('Ctrl Pts',(-22.725557905227,49.7903637578166,-40.));
#25158=CARTESIAN_POINT('Ctrl Pts',(-22.7288943329894,49.6934950551849,-40.));
#25159=CARTESIAN_POINT('Ctrl Pts',(-22.7270235061783,49.5967899064236,-40.));
#25160=CARTESIAN_POINT('Ctrl Pts',(-22.7198805143962,49.5006675099145,-40.));
#25161=CARTESIAN_POINT('Ctrl Pts',(-22.712737522614,49.4045451134053,-40.));
#25162=CARTESIAN_POINT('Ctrl Pts',(-22.7003227972537,49.3090044263321,-40.));
#25163=CARTESIAN_POINT('Ctrl Pts',(-22.6825189643874,49.2144458603069,-40.));
#25164=CARTESIAN_POINT('Ctrl Pts',(-22.665463885311,49.1238640270008,-40.));
#25165=CARTESIAN_POINT('Ctrl Pts',(-22.6434635856682,49.0341824768018,-40.));
#25166=CARTESIAN_POINT('Ctrl Pts',(-22.616792982512,48.9456408602185,-40.));
#25167=CARTESIAN_POINT('Ctrl Pts',(-22.6079257015727,48.9162030786856,-40.));
#25168=CARTESIAN_POINT('Ctrl Pts',(-22.5985417398083,48.8868913399485,-40.));
#25169=CARTESIAN_POINT('Ctrl Pts',(-22.5886499529707,48.8577146251926,-40.));
#25170=CARTESIAN_POINT('Ctrl Pts',(-22.5793485397899,48.8302792706246,-40.));
#25171=CARTESIAN_POINT('Ctrl Pts',(-22.5695981035871,48.802963302685,-40.));
#25172=CARTESIAN_POINT('Ctrl Pts',(-22.5594055359165,48.7757743123091,-40.));
#25173=CARTESIAN_POINT('Ctrl Pts',(-22.5542253548657,48.7619560186967,-40.));
#25174=CARTESIAN_POINT('Ctrl Pts',(-22.5489339952992,48.7481786707038,-40.));
#25175=CARTESIAN_POINT('Ctrl Pts',(-22.5435342675695,48.7344469223358,-40.));
#25176=CARTESIAN_POINT('Ctrl Pts',(-22.5092832385399,48.6473450284018,-40.));
#25177=CARTESIAN_POINT('Ctrl Pts',(-22.4706582380904,48.5620297353929,-40.));
#25178=CARTESIAN_POINT('Ctrl Pts',(-22.427989529844,48.4787357602314,-40.));
#25179=CARTESIAN_POINT('Ctrl Pts',(-22.3837558889833,48.3923868658173,-40.));
#25180=CARTESIAN_POINT('Ctrl Pts',(-22.3351763545133,48.3082095465738,-40.));
#25181=CARTESIAN_POINT('Ctrl Pts',(-22.2825630205183,48.2264687487337,-40.));
#25182=CARTESIAN_POINT('Ctrl Pts',(-22.2293841761177,48.1438493661654,-40.));
#25183=CARTESIAN_POINT('Ctrl Pts',(-22.1720839368917,48.063718341668,-40.));
#25184=CARTESIAN_POINT('Ctrl Pts',(-22.1109330459416,47.9863645989668,-40.));
#25185=CARTESIAN_POINT('Ctrl Pts',(-22.088259935904,47.9576839061292,-40.));
#25186=CARTESIAN_POINT('Ctrl Pts',(-22.0650569932795,47.9293852274522,-40.));
#25187=CARTESIAN_POINT('Ctrl Pts',(-22.0413364278114,47.9014841749402,-40.));
#25188=CARTESIAN_POINT('Ctrl Pts',(-22.0207016997641,47.87721280453,-40.));
#25189=CARTESIAN_POINT('Ctrl Pts',(-21.9996752508981,47.8532423398925,-40.));
#25190=CARTESIAN_POINT('Ctrl Pts',(-21.978264639229,47.8295834329929,-40.));
#25191=CARTESIAN_POINT('Ctrl Pts',(-21.9677218695906,47.8179335834141,-40.));
#25192=CARTESIAN_POINT('Ctrl Pts',(-21.9570890367767,47.8063627576625,-40.));
#25193=CARTESIAN_POINT('Ctrl Pts',(-21.9463727949803,47.794877973483,-40.));
#25194=CARTESIAN_POINT('Ctrl Pts',(-21.8775100213453,47.7210765318742,-40.));
#25195=CARTESIAN_POINT('Ctrl Pts',(-21.8051396835538,47.6507519278206,-40.));
#25196=CARTESIAN_POINT('Ctrl Pts',(-21.7295715001049,47.5841951608942,-40.));
#25197=CARTESIAN_POINT('Ctrl Pts',(-21.6670825471831,47.5291579417198,-40.));
#25198=CARTESIAN_POINT('Ctrl Pts',(-21.60240582197,47.4766972063418,-40.));
#25199=CARTESIAN_POINT('Ctrl Pts',(-21.535693597432,47.4269910002443,-40.));
#25200=CARTESIAN_POINT('Ctrl Pts',(-21.5125545115,47.4097504392795,-40.));
#25201=CARTESIAN_POINT('Ctrl Pts',(-21.4891703803795,47.3928413931205,-40.));
#25202=CARTESIAN_POINT('Ctrl Pts',(-21.4655470557819,47.3762717525203,-40.));
#25203=CARTESIAN_POINT('Ctrl Pts',(-21.4454904073927,47.362203814958,-40.));
#25204=CARTESIAN_POINT('Ctrl Pts',(-21.4252581140449,47.3483785451348,-40.));
#25205=CARTESIAN_POINT('Ctrl Pts',(-21.4048762477445,47.334815522396,-40.));
#25206=CARTESIAN_POINT('Ctrl Pts',(-21.3199246368295,47.2782848488273,-40.));
#25207=CARTESIAN_POINT('Ctrl Pts',(-21.2323068761709,47.2262558090893,-40.));
#25208=CARTESIAN_POINT('Ctrl Pts',(-21.1423134823526,47.1790369102475,-40.));
#25209=CARTESIAN_POINT('Ctrl Pts',(-21.0593683036803,47.1355161601684,-40.));
#25210=CARTESIAN_POINT('Ctrl Pts',(-20.9744042095711,47.0960813707627,-40.));
#25211=CARTESIAN_POINT('Ctrl Pts',(-20.8876216150834,47.0610025297207,-40.));
#25212=CARTESIAN_POINT('Ctrl Pts',(-20.8571893637145,47.0487013521099,-40.));
#25213=CARTESIAN_POINT('Ctrl Pts',(-20.8265332852914,47.0369361167847,-40.));
#25214=CARTESIAN_POINT('Ctrl Pts',(-20.7956662771738,47.0257030918457,-40.));
#25215=CARTESIAN_POINT('Ctrl Pts',(-19.2062007174672,-52.9692229537457,
-40.));
#25216=CARTESIAN_POINT('Ctrl Pts',(-19.1131357468007,-52.9351793717574,
-40.));
#25217=CARTESIAN_POINT('Ctrl Pts',(-19.0221360561095,-52.8963691647869,
-40.));
#25218=CARTESIAN_POINT('Ctrl Pts',(-18.9334103507984,-52.8531200918645,
-40.));
#25219=CARTESIAN_POINT('Ctrl Pts',(-18.8427248539677,-52.8089157245768,
-40.));
#25220=CARTESIAN_POINT('Ctrl Pts',(-18.7544142403876,-52.7600736163027,
-40.));
#25221=CARTESIAN_POINT('Ctrl Pts',(-18.6687302769065,-52.706898201355,-40.));
#25222=CARTESIAN_POINT('Ctrl Pts',(-18.5863008405935,-52.6557425439628,
-40.));
#25223=CARTESIAN_POINT('Ctrl Pts',(-18.5063020247127,-52.6005756362984,
-40.));
#25224=CARTESIAN_POINT('Ctrl Pts',(-18.4289909484007,-52.5416384892086,
-40.));
#25225=CARTESIAN_POINT('Ctrl Pts',(-18.3613437566276,-52.4900684855051,
-40.));
#25226=CARTESIAN_POINT('Ctrl Pts',(-18.2957546556056,-52.4356111955853,
-40.));
#25227=CARTESIAN_POINT('Ctrl Pts',(-18.2324205149676,-52.3784153761812,
-40.));
#25228=CARTESIAN_POINT('Ctrl Pts',(-18.2182964234727,-52.3656601863538,
-40.));
#25229=CARTESIAN_POINT('Ctrl Pts',(-18.2042818486488,-52.3527660785552,
-40.));
#25230=CARTESIAN_POINT('Ctrl Pts',(-18.1903985212288,-52.3397531951332,
-40.));
#25231=CARTESIAN_POINT('Ctrl Pts',(-18.1179658362636,-52.2718618275319,
-40.));
#25232=CARTESIAN_POINT('Ctrl Pts',(-18.0489987873894,-52.200649229851,-40.));
#25233=CARTESIAN_POINT('Ctrl Pts',(-17.9837374446072,-52.1264054105887,
-40.));
#25234=CARTESIAN_POINT('Ctrl Pts',(-17.9188380908689,-52.0525734040167,
-40.));
#25235=CARTESIAN_POINT('Ctrl Pts',(-17.8576029616476,-51.9757429138075,
-40.));
#25236=CARTESIAN_POINT('Ctrl Pts',(-17.8003117583802,-51.8961723809,-40.));
#25237=CARTESIAN_POINT('Ctrl Pts',(-17.7451459668942,-51.8195537871811,
-40.));
#25238=CARTESIAN_POINT('Ctrl Pts',(-17.693636739165,-51.7403939459348,-40.));
#25239=CARTESIAN_POINT('Ctrl Pts',(-17.6460786375857,-51.6589099827569,
-40.));
#25240=CARTESIAN_POINT('Ctrl Pts',(-17.6261329337694,-51.6247358895667,
-40.));
#25241=CARTESIAN_POINT('Ctrl Pts',(-17.6068827766128,-51.5901528915744,
-40.));
#25242=CARTESIAN_POINT('Ctrl Pts',(-17.5883524791399,-51.5551767069529,
-40.));
#25243=CARTESIAN_POINT('Ctrl Pts',(-17.5754733662171,-51.5308672088453,
-40.));
#25244=CARTESIAN_POINT('Ctrl Pts',(-17.5629420259769,-51.5063677726217,
-40.));
#25245=CARTESIAN_POINT('Ctrl Pts',(-17.5507670869457,-51.4816836694644,
-40.));
#25246=CARTESIAN_POINT('Ctrl Pts',(-17.5428534289798,-51.4656391086596,
-40.));
#25247=CARTESIAN_POINT('Ctrl Pts',(-17.5350892341274,-51.4495139009789,
-40.));
#25248=CARTESIAN_POINT('Ctrl Pts',(-17.5274870637955,-51.433331713181,-40.));
#25249=CARTESIAN_POINT('Ctrl Pts',(-17.4853646028894,-51.3436686902377,
-40.));
#25250=CARTESIAN_POINT('Ctrl Pts',(-17.4481415142809,-51.2521198132569,
-40.));
#25251=CARTESIAN_POINT('Ctrl Pts',(-17.4161092181085,-51.1589567015166,
-40.));
#25252=CARTESIAN_POINT('Ctrl Pts',(-17.3862302908103,-51.0720564734599,
-40.));
#25253=CARTESIAN_POINT('Ctrl Pts',(-17.360867886728,-50.9837509583388,-40.));
#25254=CARTESIAN_POINT('Ctrl Pts',(-17.3403090519426,-50.8942518698057,
-40.));
#25255=CARTESIAN_POINT('Ctrl Pts',(-17.3388273804463,-50.8878016867186,
-40.));
#25256=CARTESIAN_POINT('Ctrl Pts',(-17.3373706815264,-50.8813453029637,
-40.));
#25257=CARTESIAN_POINT('Ctrl Pts',(-17.3359390732883,-50.8748827974692,
-40.));
#25258=CARTESIAN_POINT('Ctrl Pts',(-17.3153335150716,-50.781866056118,-40.));
#25259=CARTESIAN_POINT('Ctrl Pts',(-17.2999216891736,-50.6875801101407,
-40.));
#25260=CARTESIAN_POINT('Ctrl Pts',(-17.2896265581787,-50.5924334387263,
-40.));
#25261=CARTESIAN_POINT('Ctrl Pts',(-17.2838314953604,-50.538875991223,-40.));
#25262=CARTESIAN_POINT('Ctrl Pts',(-17.279658581871,-50.4850460121277,-40.));
#25263=CARTESIAN_POINT('Ctrl Pts',(-17.27710083857,-50.4310189910692,-40.));
#25264=CARTESIAN_POINT('Ctrl Pts',(-17.2764402753775,-50.4170659640024,
-40.));
#25265=CARTESIAN_POINT('Ctrl Pts',(-17.275887561613,-50.4031003903426,-40.));
#25266=CARTESIAN_POINT('Ctrl Pts',(-17.2754428183204,-50.3891369453735,
-40.));
#25267=CARTESIAN_POINT('Ctrl Pts',(-17.2724737419776,-50.2959179248492,
-40.));
#25268=CARTESIAN_POINT('Ctrl Pts',(-17.2743042614248,-50.2026383647503,
-40.));
#25269=CARTESIAN_POINT('Ctrl Pts',(-17.2807993648699,-50.1096739507498,
-40.));
#25270=CARTESIAN_POINT('Ctrl Pts',(-17.2873052436734,-50.0165553090462,
-40.));
#25271=CARTESIAN_POINT('Ctrl Pts',(-17.2984915746125,-49.923751879078,-40.));
#25272=CARTESIAN_POINT('Ctrl Pts',(-17.3142736081437,-49.8316533006875,
-40.));
#25273=CARTESIAN_POINT('Ctrl Pts',(-17.3298294071013,-49.7408749502994,
-40.));
#25274=CARTESIAN_POINT('Ctrl Pts',(-17.3498505561529,-49.6507805433845,
-40.));
#25275=CARTESIAN_POINT('Ctrl Pts',(-17.3742989167507,-49.5617684017665,
-40.));
#25276=CARTESIAN_POINT('Ctrl Pts',(-17.3833972300998,-49.5286430577144,
-40.));
#25277=CARTESIAN_POINT('Ctrl Pts',(-17.3931090713021,-49.4956679147191,
-40.));
#25278=CARTESIAN_POINT('Ctrl Pts',(-17.4034338352087,-49.4628647675681,
-40.));
#25279=CARTESIAN_POINT('Ctrl Pts',(-17.4104013467753,-49.4407280572992,
-40.));
#25280=CARTESIAN_POINT('Ctrl Pts',(-17.417647999536,-49.4186696895679,-40.));
#25281=CARTESIAN_POINT('Ctrl Pts',(-17.4251737841929,-49.3966965729596,
-40.));
#25282=CARTESIAN_POINT('Ctrl Pts',(-17.4301878061034,-49.382057077792,-40.));
#25283=CARTESIAN_POINT('Ctrl Pts',(-17.4353251421779,-49.3674573502381,
-40.));
#25284=CARTESIAN_POINT('Ctrl Pts',(-17.4405816639177,-49.3529101268342,
-40.));
#25285=CARTESIAN_POINT('Ctrl Pts',(-17.4722302182215,-49.2653239600375,
-40.));
#25286=CARTESIAN_POINT('Ctrl Pts',(-17.5082330002425,-49.179527854485,-40.));
#25287=CARTESIAN_POINT('Ctrl Pts',(-17.5485266814233,-49.0959323823922,
-40.));
#25288=CARTESIAN_POINT('Ctrl Pts',(-17.5787469423089,-49.0332357783227,
-40.));
#25289=CARTESIAN_POINT('Ctrl Pts',(-17.6113818631069,-48.9717775200094,
-40.));
#25290=CARTESIAN_POINT('Ctrl Pts',(-17.6464204160553,-48.9117461825991,
-40.));
#25291=CARTESIAN_POINT('Ctrl Pts',(-17.660247661566,-48.8880560478515,-40.));
#25292=CARTESIAN_POINT('Ctrl Pts',(-17.6744493681646,-48.8645882976847,
-40.));
#25293=CARTESIAN_POINT('Ctrl Pts',(-17.6890253763523,-48.841355220092,-40.));
#25294=CARTESIAN_POINT('Ctrl Pts',(-17.6985117582113,-48.8262346299435,
-40.));
#25295=CARTESIAN_POINT('Ctrl Pts',(-17.7081568238899,-48.8112134279567,
-40.));
#25296=CARTESIAN_POINT('Ctrl Pts',(-17.7179522363345,-48.7963072584545,
-40.));
#25297=CARTESIAN_POINT('Ctrl Pts',(-17.7651531576604,-48.7244792534651,
-40.));
#25298=CARTESIAN_POINT('Ctrl Pts',(-17.8158876776876,-48.6552461133118,
-40.));
#25299=CARTESIAN_POINT('Ctrl Pts',(-17.8701228975197,-48.5889603017741,
-40.));
#25300=CARTESIAN_POINT('Ctrl Pts',(-17.9188076297135,-48.5294582477039,
-40.));
#25301=CARTESIAN_POINT('Ctrl Pts',(-17.9703138023661,-48.472331218078,-40.));
#25302=CARTESIAN_POINT('Ctrl Pts',(-18.0246379129771,-48.4178637240035,
-40.));
#25303=CARTESIAN_POINT('Ctrl Pts',(-18.0437209115739,-48.3987303575976,
-40.));
#25304=CARTESIAN_POINT('Ctrl Pts',(-18.0631518076453,-48.3799254631098,
-40.));
#25305=CARTESIAN_POINT('Ctrl Pts',(-18.0829200279321,-48.3614535172687,
-40.));
#25306=CARTESIAN_POINT('Ctrl Pts',(-21.913465996665,-48.364012796625,-40.));
#25307=CARTESIAN_POINT('Ctrl Pts',(-21.9750879218973,-48.4219222749338,
-40.));
#25308=CARTESIAN_POINT('Ctrl Pts',(-22.0333413829535,-48.482981576944,-40.));
#25309=CARTESIAN_POINT('Ctrl Pts',(-22.0882283173664,-48.5468060984396,
-40.));
#25310=CARTESIAN_POINT('Ctrl Pts',(-22.1445670692492,-48.612318846037,-40.));
#25311=CARTESIAN_POINT('Ctrl Pts',(-22.1973592804025,-48.6807454656577,
-40.));
#25312=CARTESIAN_POINT('Ctrl Pts',(-22.2465815503343,-48.751718571351,-40.));
#25313=CARTESIAN_POINT('Ctrl Pts',(-22.2971413216833,-48.8246202071501,
-40.));
#25314=CARTESIAN_POINT('Ctrl Pts',(-22.3439350380711,-48.9002091565446,
-40.));
#25315=CARTESIAN_POINT('Ctrl Pts',(-22.3869032972462,-48.9781302086408,
-40.));
#25316=CARTESIAN_POINT('Ctrl Pts',(-22.4058048319915,-49.0124073122952,
-40.));
#25317=CARTESIAN_POINT('Ctrl Pts',(-22.4239656268606,-49.0471361933387,
-40.));
#25318=CARTESIAN_POINT('Ctrl Pts',(-22.4413782060802,-49.0822886868408,
-40.));
#25319=CARTESIAN_POINT('Ctrl Pts',(-22.4513087592254,-49.1023364753106,
-40.));
#25320=CARTESIAN_POINT('Ctrl Pts',(-22.4609959250573,-49.1225220655097,
-40.));
#25321=CARTESIAN_POINT('Ctrl Pts',(-22.4704380828812,-49.1428403811056,
-40.));
#25322=CARTESIAN_POINT('Ctrl Pts',(-22.4789457638369,-49.161147822039,-40.));
#25323=CARTESIAN_POINT('Ctrl Pts',(-22.4872569080763,-49.1795687430977,
-40.));
#25324=CARTESIAN_POINT('Ctrl Pts',(-22.4953566663574,-49.1980676837875,
-40.));
#25325=CARTESIAN_POINT('Ctrl Pts',(-22.5319351704572,-49.2816088901274,
-40.));
#25326=CARTESIAN_POINT('Ctrl Pts',(-22.5642528080409,-49.3668334890526,
-40.));
#25327=CARTESIAN_POINT('Ctrl Pts',(-22.5922840449568,-49.4533430372071,
-40.));
#25328=CARTESIAN_POINT('Ctrl Pts',(-22.620776498499,-49.5412759846236,-40.));
#25329=CARTESIAN_POINT('Ctrl Pts',(-22.6448408308761,-49.6305372683465,
-40.));
#25330=CARTESIAN_POINT('Ctrl Pts',(-22.6644111567722,-49.7207455669619,
-40.));
#25331=CARTESIAN_POINT('Ctrl Pts',(-22.6833884014399,-49.8082200915544,
-40.));
#25332=CARTESIAN_POINT('Ctrl Pts',(-22.6981400517734,-49.8965860187497,
-40.));
#25333=CARTESIAN_POINT('Ctrl Pts',(-22.7085652993693,-49.9855175100408,
-40.));
#25334=CARTESIAN_POINT('Ctrl Pts',(-22.7129365604003,-50.0228060980321,
-40.));
#25335=CARTESIAN_POINT('Ctrl Pts',(-22.7165466860838,-50.0601943091777,
-40.));
#25336=CARTESIAN_POINT('Ctrl Pts',(-22.7193859124485,-50.0976587417654,
-40.));
#25337=CARTESIAN_POINT('Ctrl Pts',(-22.721167342343,-50.1211652367108,-40.));
#25338=CARTESIAN_POINT('Ctrl Pts',(-22.7226452604816,-50.1447017435747,
-40.));
#25339=CARTESIAN_POINT('Ctrl Pts',(-22.7238169591624,-50.1682625149501,
-40.));
#25340=CARTESIAN_POINT('Ctrl Pts',(-22.7245027847159,-50.1820532440298,
-40.));
#25341=CARTESIAN_POINT('Ctrl Pts',(-22.7250834069287,-50.1958473360712,
-40.));
#25342=CARTESIAN_POINT('Ctrl Pts',(-22.7255583228104,-50.2096358053294,
-40.));
#25343=CARTESIAN_POINT('Ctrl Pts',(-22.7288947681752,-50.3065044848366,
-40.));
#25344=CARTESIAN_POINT('Ctrl Pts',(-22.7270239561279,-50.4032096135111,
-40.));
#25345=CARTESIAN_POINT('Ctrl Pts',(-22.7198809751868,-50.4993319941221,
-40.));
#25346=CARTESIAN_POINT('Ctrl Pts',(-22.7127379942457,-50.5954543747331,
-40.));
#25347=CARTESIAN_POINT('Ctrl Pts',(-22.7003232758061,-50.6909950500943,
-40.));
#25348=CARTESIAN_POINT('Ctrl Pts',(-22.6825194448535,-50.7855536097484,
-40.));
#25349=CARTESIAN_POINT('Ctrl Pts',(-22.6654643706524,-50.8761354207948,
-40.));
#25350=CARTESIAN_POINT('Ctrl Pts',(-22.643464073055,-50.9658169539538,-40.));
#25351=CARTESIAN_POINT('Ctrl Pts',(-22.6167934697688,-51.0543585580536,
-40.));
#25352=CARTESIAN_POINT('Ctrl Pts',(-22.6079261927359,-51.0837963223242,
-40.));
#25353=CARTESIAN_POINT('Ctrl Pts',(-22.5985422350976,-51.1131080444153,
-40.));
#25354=CARTESIAN_POINT('Ctrl Pts',(-22.588650452618,-51.1422847431305,-40.));
#25355=CARTESIAN_POINT('Ctrl Pts',(-22.5793490783144,-51.1697199800305,
-40.));
#25356=CARTESIAN_POINT('Ctrl Pts',(-22.5695986845515,-51.1970358317301,
-40.));
#25357=CARTESIAN_POINT('Ctrl Pts',(-22.5594061628182,-51.2242247073709,
-40.));
#25358=CARTESIAN_POINT('Ctrl Pts',(-22.5542259348717,-51.238043130045,-40.));
#25359=CARTESIAN_POINT('Ctrl Pts',(-22.5489345261121,-51.2518206068617,
-40.));
#25360=CARTESIAN_POINT('Ctrl Pts',(-22.543534747184,-51.2655524831179,-40.));
#25361=CARTESIAN_POINT('Ctrl Pts',(-22.5092837175801,-51.3526543638479,
-40.));
#25362=CARTESIAN_POINT('Ctrl Pts',(-22.4706587156271,-51.4379696481888,
-40.));
#25363=CARTESIAN_POINT('Ctrl Pts',(-22.4279900055383,-51.5212636185752,
-40.));
#25364=CARTESIAN_POINT('Ctrl Pts',(-22.3837563555061,-51.6076125222142,
-40.));
#25365=CARTESIAN_POINT('Ctrl Pts',(-22.3351768100742,-51.6917898541535,
-40.));
#25366=CARTESIAN_POINT('Ctrl Pts',(-22.2825634641401,-51.7735306673781,
-40.));
#25367=CARTESIAN_POINT('Ctrl Pts',(-22.2293846024825,-51.8561500735585,
-40.));
#25368=CARTESIAN_POINT('Ctrl Pts',(-22.1720843441963,-51.9362811239307,
-40.));
#25369=CARTESIAN_POINT('Ctrl Pts',(-22.1109334332859,-52.0136348939272,
-40.));
#25370=CARTESIAN_POINT('Ctrl Pts',(-22.0882603552691,-52.0423155470182,
-40.));
#25371=CARTESIAN_POINT('Ctrl Pts',(-22.0650574463836,-52.0706141874726,
-40.));
#25372=CARTESIAN_POINT('Ctrl Pts',(-22.0413369163553,-52.0985152033257,
-40.));
#25373=CARTESIAN_POINT('Ctrl Pts',(-22.0207024334489,-52.1227862897646,
-40.));
#25374=CARTESIAN_POINT('Ctrl Pts',(-21.9996762391468,-52.146756477864,-40.));
#25375=CARTESIAN_POINT('Ctrl Pts',(-21.9782658912232,-52.1704151160217,
-40.));
#25376=CARTESIAN_POINT('Ctrl Pts',(-21.9677232491215,-52.1820648358488,
-40.));
#25377=CARTESIAN_POINT('Ctrl Pts',(-21.9570905451999,-52.19363553461,-40.));
#25378=CARTESIAN_POINT('Ctrl Pts',(-21.9463744344869,-52.2051201936141,
-40.));
#25379=CARTESIAN_POINT('Ctrl Pts',(-21.8775116906258,-52.2789217016908,
-40.));
#25380=CARTESIAN_POINT('Ctrl Pts',(-21.805141381102,-52.349246375309,-40.));
#25381=CARTESIAN_POINT('Ctrl Pts',(-21.7295732255667,-52.415803214236,-40.));
#25382=CARTESIAN_POINT('Ctrl Pts',(-21.6670841510965,-52.4708406203331,
-40.));
#25383=CARTESIAN_POINT('Ctrl Pts',(-21.6024072939712,-52.5233015323814,
-40.));
#25384=CARTESIAN_POINT('Ctrl Pts',(-21.5356949288188,-52.5730079033295,
-40.));
#25385=CARTESIAN_POINT('Ctrl Pts',(-21.5125562912412,-52.5902481510713,
-40.));
#25386=CARTESIAN_POINT('Ctrl Pts',(-21.4891726179549,-52.6071568968281,
-40.));
#25387=CARTESIAN_POINT('Ctrl Pts',(-21.465549760361,-52.6237262502898,-40.));
#25388=CARTESIAN_POINT('Ctrl Pts',(-21.4454922749805,-52.637794809248,-40.));
#25389=CARTESIAN_POINT('Ctrl Pts',(-21.4252591293115,-52.6516206804198,
-40.));
#25390=CARTESIAN_POINT('Ctrl Pts',(-21.4048763978817,-52.6651842824533,
-40.));
#25391=CARTESIAN_POINT('Ctrl Pts',(-21.3199247651891,-52.7217149855095,
-40.));
#25392=CARTESIAN_POINT('Ctrl Pts',(-21.232306984753,-52.7737440527519,-40.));
#25393=CARTESIAN_POINT('Ctrl Pts',(-21.1423135741234,-52.8209629762043,
-40.));
#25394=CARTESIAN_POINT('Ctrl Pts',(-21.0593683216558,-52.8644837795565,
-40.));
#25395=CARTESIAN_POINT('Ctrl Pts',(-20.9744041534344,-52.9039186140383,
-40.));
#25396=CARTESIAN_POINT('Ctrl Pts',(-20.887621485693,-52.9389974906628,-40.));
#25397=CARTESIAN_POINT('Ctrl Pts',(-20.8571892302267,-52.9512986720242,
-40.));
#25398=CARTESIAN_POINT('Ctrl Pts',(-20.8265331481289,-52.9630639106919,
-40.));
#25399=CARTESIAN_POINT('Ctrl Pts',(-20.7956661367394,-52.9742969385866,
-40.));
#25400=CARTESIAN_POINT('Origin',(-20.,-50.,-25.));
#25401=CARTESIAN_POINT('Ctrl Pts',(-18.0865340033349,-48.3640127966251,
-25.));
#25402=CARTESIAN_POINT('Ctrl Pts',(-18.0243832850997,-48.4224192105103,
-25.));
#25403=CARTESIAN_POINT('Ctrl Pts',(-17.9656071264269,-48.4840785138675,
-25.));
#25404=CARTESIAN_POINT('Ctrl Pts',(-17.9102179711386,-48.5486144685222,
-25.));
#25405=CARTESIAN_POINT('Ctrl Pts',(-17.8534755897244,-48.6147271170159,
-25.));
#25406=CARTESIAN_POINT('Ctrl Pts',(-17.8002872616887,-48.6838591854776,
-25.));
#25407=CARTESIAN_POINT('Ctrl Pts',(-17.7506952446208,-48.7556524546743,
-25.));
#25408=CARTESIAN_POINT('Ctrl Pts',(-17.737728064412,-48.7744247554294,-25.));
#25409=CARTESIAN_POINT('Ctrl Pts',(-17.7250069365578,-48.7933792207731,
-25.));
#25410=CARTESIAN_POINT('Ctrl Pts',(-17.7125329944118,-48.8125098826575,
-25.));
#25411=CARTESIAN_POINT('Ctrl Pts',(-17.702405577042,-48.8280417967225,-25.));
#25412=CARTESIAN_POINT('Ctrl Pts',(-17.6924406896447,-48.8436907013992,
-25.));
#25413=CARTESIAN_POINT('Ctrl Pts',(-17.6826476852539,-48.8594389743045,
-25.));
#25414=CARTESIAN_POINT('Ctrl Pts',(-17.6351883455804,-48.9357590292394,
-25.));
#25415=CARTESIAN_POINT('Ctrl Pts',(-17.5917124377679,-49.0144857272152,
-25.));
#25416=CARTESIAN_POINT('Ctrl Pts',(-17.5522551555271,-49.095226864203,-25.));
#25417=CARTESIAN_POINT('Ctrl Pts',(-17.5204200254773,-49.1603708490493,
-25.));
#25418=CARTESIAN_POINT('Ctrl Pts',(-17.4912013880664,-49.226827255453,-25.));
#25419=CARTESIAN_POINT('Ctrl Pts',(-17.4646348766623,-49.2944078866059,
-25.));
#25420=CARTESIAN_POINT('Ctrl Pts',(-17.4539839348206,-49.3215020489175,
-25.));
#25421=CARTESIAN_POINT('Ctrl Pts',(-17.4437594637069,-49.3487770650009,
-25.));
#25422=CARTESIAN_POINT('Ctrl Pts',(-17.4339645308892,-49.3762213605602,
-25.));
#25423=CARTESIAN_POINT('Ctrl Pts',(-17.4287329400572,-49.3908796872388,
-25.));
#25424=CARTESIAN_POINT('Ctrl Pts',(-17.4236243316885,-49.4055852979435,
-25.));
#25425=CARTESIAN_POINT('Ctrl Pts',(-17.4186430808377,-49.4203242086228,
-25.));
#25426=CARTESIAN_POINT('Ctrl Pts',(-17.3890982615448,-49.5077437073873,
-25.));
#25427=CARTESIAN_POINT('Ctrl Pts',(-17.3639901618958,-49.5964439977786,
-25.));
#25428=CARTESIAN_POINT('Ctrl Pts',(-17.3433519062038,-49.6860276500902,
-25.));
#25429=CARTESIAN_POINT('Ctrl Pts',(-17.3223954629373,-49.7769924464998,
-25.));
#25430=CARTESIAN_POINT('Ctrl Pts',(-17.306047251885,-49.8688688586223,-25.));
#25431=CARTESIAN_POINT('Ctrl Pts',(-17.2943837746448,-49.9612739444462,
-25.));
#25432=CARTESIAN_POINT('Ctrl Pts',(-17.2828119061749,-50.0529532504608,
-25.));
#25433=CARTESIAN_POINT('Ctrl Pts',(-17.2758511252064,-50.1451538869544,
-25.));
#25434=CARTESIAN_POINT('Ctrl Pts',(-17.2736230843733,-50.2375210507824,
-25.));
#25435=CARTESIAN_POINT('Ctrl Pts',(-17.2725148765619,-50.283463661413,-25.));
#25436=CARTESIAN_POINT('Ctrl Pts',(-17.272578302097,-50.3294476832055,-25.));
#25437=CARTESIAN_POINT('Ctrl Pts',(-17.2738331202707,-50.375430153216,-25.));
#25438=CARTESIAN_POINT('Ctrl Pts',(-17.2742439451017,-50.3904847171926,
-25.));
#25439=CARTESIAN_POINT('Ctrl Pts',(-17.2747825691208,-50.4055406251206,
-25.));
#25440=CARTESIAN_POINT('Ctrl Pts',(-17.2754495535264,-50.4205916673977,
-25.));
#25441=CARTESIAN_POINT('Ctrl Pts',(-17.2796905507083,-50.516293197071,-25.));
#25442=CARTESIAN_POINT('Ctrl Pts',(-17.2891001105497,-50.6114301979472,
-25.));
#25443=CARTESIAN_POINT('Ctrl Pts',(-17.3037427186582,-50.7056047140635,
-25.));
#25444=CARTESIAN_POINT('Ctrl Pts',(-17.3078986693771,-50.7323338763174,
-25.));
#25445=CARTESIAN_POINT('Ctrl Pts',(-17.3124764735867,-50.758985634219,-25.));
#25446=CARTESIAN_POINT('Ctrl Pts',(-17.3174783250881,-50.7855511504669,
-25.));
#25447=CARTESIAN_POINT('Ctrl Pts',(-17.3344205238429,-50.8755334812447,
-25.));
#25448=CARTESIAN_POINT('Ctrl Pts',(-17.3562236803317,-50.9645262383779,
-25.));
#25449=CARTESIAN_POINT('Ctrl Pts',(-17.382584962494,-51.0522968717463,-25.));
#25450=CARTESIAN_POINT('Ctrl Pts',(-17.4095434902992,-51.1420560513483,
-25.));
#25451=CARTESIAN_POINT('Ctrl Pts',(-17.44126923195,-51.2305378030409,-25.));
#25452=CARTESIAN_POINT('Ctrl Pts',(-17.4774925519387,-51.3174897503804,
-25.));
#25453=CARTESIAN_POINT('Ctrl Pts',(-17.4899691547968,-51.3474391011035,
-25.));
#25454=CARTESIAN_POINT('Ctrl Pts',(-17.502979781103,-51.3772068812893,-25.));
#25455=CARTESIAN_POINT('Ctrl Pts',(-17.5165147798695,-51.4067824406253,
-25.));
#25456=CARTESIAN_POINT('Ctrl Pts',(-17.5231905157176,-51.4213697062096,
-25.));
#25457=CARTESIAN_POINT('Ctrl Pts',(-17.5299938239586,-51.4359102074969,
-25.));
#25458=CARTESIAN_POINT('Ctrl Pts',(-17.5369236053827,-51.4504026443194,
-25.));
#25459=CARTESIAN_POINT('Ctrl Pts',(-17.5430251409841,-51.46316294855,-25.));
#25460=CARTESIAN_POINT('Ctrl Pts',(-17.549223964339,-51.4758842663769,-25.));
#25461=CARTESIAN_POINT('Ctrl Pts',(-17.5555138729846,-51.488555244485,-25.));
#25462=CARTESIAN_POINT('Ctrl Pts',(-17.5983732491784,-51.5748951657893,
-25.));
#25463=CARTESIAN_POINT('Ctrl Pts',(-17.645521751679,-51.6590337918885,-25.));
#25464=CARTESIAN_POINT('Ctrl Pts',(-17.6966168151664,-51.7407208715959,
-25.));
#25465=CARTESIAN_POINT('Ctrl Pts',(-17.7487215795578,-51.8240221878382,
-25.));
#25466=CARTESIAN_POINT('Ctrl Pts',(-17.8049307394874,-51.9047748826328,
-25.));
#25467=CARTESIAN_POINT('Ctrl Pts',(-17.8649359851474,-51.9827064087797,
-25.));
#25468=CARTESIAN_POINT('Ctrl Pts',(-17.9254196422576,-52.061259269512,-25.));
#25469=CARTESIAN_POINT('Ctrl Pts',(-17.9897606186624,-52.1369466346382,
-25.));
#25470=CARTESIAN_POINT('Ctrl Pts',(-18.0576924116876,-52.2094699519837,
-25.));
#25471=CARTESIAN_POINT('Ctrl Pts',(-18.0946383138793,-52.2489130355524,
-25.));
#25472=CARTESIAN_POINT('Ctrl Pts',(-18.1326471623705,-52.2874198090281,
-25.));
#25473=CARTESIAN_POINT('Ctrl Pts',(-18.1716813643735,-52.3249384844083,
-25.));
#25474=CARTESIAN_POINT('Ctrl Pts',(-18.184337849379,-52.3371035736892,-25.));
#25475=CARTESIAN_POINT('Ctrl Pts',(-18.1971021587896,-52.3491647575441,
-25.));
#25476=CARTESIAN_POINT('Ctrl Pts',(-18.2099730859135,-52.3611201963401,
-25.));
#25477=CARTESIAN_POINT('Ctrl Pts',(-18.221458568745,-52.371788735266,-25.));
#25478=CARTESIAN_POINT('Ctrl Pts',(-18.2330235730151,-52.3823680223885,
-25.));
#25479=CARTESIAN_POINT('Ctrl Pts',(-18.2446616724208,-52.392852287093,-25.));
#25480=CARTESIAN_POINT('Ctrl Pts',(-18.320476523519,-52.4611506354522,-25.));
#25481=CARTESIAN_POINT('Ctrl Pts',(-18.3994575544252,-52.5254816235113,
-25.));
#25482=CARTESIAN_POINT('Ctrl Pts',(-18.4812783860139,-52.5855621951249,
-25.));
#25483=CARTESIAN_POINT('Ctrl Pts',(-18.563171620063,-52.6456959314536,-25.));
#25484=CARTESIAN_POINT('Ctrl Pts',(-18.6479102599513,-52.7015725637526,
-25.));
#25485=CARTESIAN_POINT('Ctrl Pts',(-18.7352120289865,-52.7528820895473,
-25.));
#25486=CARTESIAN_POINT('Ctrl Pts',(-18.8207515374939,-52.8031558888842,
-25.));
#25487=CARTESIAN_POINT('Ctrl Pts',(-18.9087524063426,-52.8490457775827,
-25.));
#25488=CARTESIAN_POINT('Ctrl Pts',(-18.9989828629694,-52.8902240100431,
-25.));
#25489=CARTESIAN_POINT('Ctrl Pts',(-19.0364028600903,-52.9073012741701,
-25.));
#25490=CARTESIAN_POINT('Ctrl Pts',(-19.0742066724074,-52.9235676922614,
-25.));
#25491=CARTESIAN_POINT('Ctrl Pts',(-19.1123791172294,-52.9389975882857,
-25.));
#25492=CARTESIAN_POINT('Ctrl Pts',(-19.1428008541822,-52.9512945276158,
-25.));
#25493=CARTESIAN_POINT('Ctrl Pts',(-19.1734567410254,-52.9630601291729,
-25.));
#25494=CARTESIAN_POINT('Ctrl Pts',(-19.2043345174297,-52.9742970828256,
-25.));
#25495=CARTESIAN_POINT('Ctrl Pts',(-20.7937992825329,-52.9692229537457,
-25.));
#25496=CARTESIAN_POINT('Ctrl Pts',(-20.8886442409227,-52.934528244297,-25.));
#25497=CARTESIAN_POINT('Ctrl Pts',(-20.981446133513,-52.8948452065297,-25.));
#25498=CARTESIAN_POINT('Ctrl Pts',(-21.0719638298413,-52.8504935643273,
-25.));
#25499=CARTESIAN_POINT('Ctrl Pts',(-21.1637466263856,-52.805522051377,-25.));
#25500=CARTESIAN_POINT('Ctrl Pts',(-21.2531815997536,-52.7557498214297,
-25.));
#25501=CARTESIAN_POINT('Ctrl Pts',(-21.3399833391246,-52.7014695233431,
-25.));
#25502=CARTESIAN_POINT('Ctrl Pts',(-21.3644995059587,-52.6861386687618,
-25.));
#25503=CARTESIAN_POINT('Ctrl Pts',(-21.3888053754925,-52.6704479886835,
-25.));
#25504=CARTESIAN_POINT('Ctrl Pts',(-21.4128939207048,-52.6544036208027,
-25.));
#25505=CARTESIAN_POINT('Ctrl Pts',(-21.4322113951179,-52.6415370627237,
-25.));
#25506=CARTESIAN_POINT('Ctrl Pts',(-21.4513911998519,-52.6284414304985,
-25.));
#25507=CARTESIAN_POINT('Ctrl Pts',(-21.4704104548933,-52.6151336299332,
-25.));
#25508=CARTESIAN_POINT('Ctrl Pts',(-21.5531190662063,-52.5572622936485,
-25.));
#25509=CARTESIAN_POINT('Ctrl Pts',(-21.6328730890496,-52.4953306936023,
-25.));
#25510=CARTESIAN_POINT('Ctrl Pts',(-21.7094060419017,-52.429635446766,-25.));
#25511=CARTESIAN_POINT('Ctrl Pts',(-21.7684006977073,-52.3789949274767,
-25.));
#25512=CARTESIAN_POINT('Ctrl Pts',(-21.825480777475,-52.3261171605589,-25.));
#25513=CARTESIAN_POINT('Ctrl Pts',(-21.8805066584147,-52.2711262352939,
-25.));
#25514=CARTESIAN_POINT('Ctrl Pts',(-21.9097989368823,-52.2418525650037,
-25.));
#25515=CARTESIAN_POINT('Ctrl Pts',(-21.9385088158922,-52.2119799147563,
-25.));
#25516=CARTESIAN_POINT('Ctrl Pts',(-21.9666132103813,-52.1815261718079,
-25.));
#25517=CARTESIAN_POINT('Ctrl Pts',(-21.9762498256991,-52.1710839967989,
-25.));
#25518=CARTESIAN_POINT('Ctrl Pts',(-21.9858145141289,-52.1605742164994,
-25.));
#25519=CARTESIAN_POINT('Ctrl Pts',(-21.995299714842,-52.150005155917,-25.));
#25520=CARTESIAN_POINT('Ctrl Pts',(-22.0610979628759,-52.0766882393088,
-25.));
#25521=CARTESIAN_POINT('Ctrl Pts',(-22.1231641141855,-52.000424838082,-25.));
#25522=CARTESIAN_POINT('Ctrl Pts',(-22.1812542925625,-51.9214927964729,
-25.));
#25523=CARTESIAN_POINT('Ctrl Pts',(-22.2388180795722,-51.8432760073639,
-25.));
#25524=CARTESIAN_POINT('Ctrl Pts',(-22.2924780587685,-51.7624379398908,
-25.));
#25525=CARTESIAN_POINT('Ctrl Pts',(-22.3419511803801,-51.6792265585039,
-25.));
#25526=CARTESIAN_POINT('Ctrl Pts',(-22.3900085390461,-51.5983964214488,
-25.));
#25527=CARTESIAN_POINT('Ctrl Pts',(-22.434115448639,-51.5153261622487,-25.));
#25528=CARTESIAN_POINT('Ctrl Pts',(-22.4739646868754,-51.4302327126893,
-25.));
#25529=CARTESIAN_POINT('Ctrl Pts',(-22.4947697706581,-51.3858058572261,
-25.));
#25530=CARTESIAN_POINT('Ctrl Pts',(-22.5144134671897,-51.3408274043328,
-25.));
#25531=CARTESIAN_POINT('Ctrl Pts',(-22.5328463597941,-51.2953279864297,
-25.));
#25532=CARTESIAN_POINT('Ctrl Pts',(-22.5399054107244,-51.2779035530991,
-25.));
#25533=CARTESIAN_POINT('Ctrl Pts',(-22.5467868448816,-51.2604027172689,
-25.));
#25534=CARTESIAN_POINT('Ctrl Pts',(-22.5534877247282,-51.242827207983,-25.));
#25535=CARTESIAN_POINT('Ctrl Pts',(-22.5587291589222,-51.22907962894,-25.));
#25536=CARTESIAN_POINT('Ctrl Pts',(-22.563860220659,-51.2152858632226,-25.));
#25537=CARTESIAN_POINT('Ctrl Pts',(-22.5688743760763,-51.2014614459675,
-25.));
#25538=CARTESIAN_POINT('Ctrl Pts',(-22.6005568065216,-51.1141105161159,
-25.));
#25539=CARTESIAN_POINT('Ctrl Pts',(-22.6276304308536,-51.0253962670702,
-25.));
#25540=CARTESIAN_POINT('Ctrl Pts',(-22.6498439278908,-50.9355415828215,
-25.));
#25541=CARTESIAN_POINT('Ctrl Pts',(-22.6548287984448,-50.9153775371108,
-25.));
#25542=CARTESIAN_POINT('Ctrl Pts',(-22.659568716376,-50.8951560208944,-25.));
#25543=CARTESIAN_POINT('Ctrl Pts',(-22.6640604805451,-50.8748794971407,
-25.));
#25544=CARTESIAN_POINT('Ctrl Pts',(-22.6844253433926,-50.7829493312365,
-25.));
#25545=CARTESIAN_POINT('Ctrl Pts',(-22.6996934291485,-50.6898881391101,
-25.));
#25546=CARTESIAN_POINT('Ctrl Pts',(-22.709974675792,-50.5960881004475,-25.));
#25547=CARTESIAN_POINT('Ctrl Pts',(-22.7207065967185,-50.4981763750765,
-25.));
#25548=CARTESIAN_POINT('Ctrl Pts',(-22.726004891523,-50.3994583705262,-25.));
#25549=CARTESIAN_POINT('Ctrl Pts',(-22.7259371354055,-50.3003947692319,
-25.));
#25550=CARTESIAN_POINT('Ctrl Pts',(-22.7259106318212,-50.2616449026909,
-25.));
#25551=CARTESIAN_POINT('Ctrl Pts',(-22.7250624840214,-50.2228424140868,
-25.));
#25552=CARTESIAN_POINT('Ctrl Pts',(-22.7233945124232,-50.1840161029993,
-25.));
#25553=CARTESIAN_POINT('Ctrl Pts',(-22.7228610952776,-50.1715994527069,
-25.));
#25554=CARTESIAN_POINT('Ctrl Pts',(-22.7222438367581,-50.1591816778759,
-25.));
#25555=CARTESIAN_POINT('Ctrl Pts',(-22.7215434984435,-50.146773388563,-25.));
#25556=CARTESIAN_POINT('Ctrl Pts',(-22.7163011580038,-50.0538918832931,
-25.));
#25557=CARTESIAN_POINT('Ctrl Pts',(-22.706402037016,-49.9613918757547,-25.));
#25558=CARTESIAN_POINT('Ctrl Pts',(-22.6919697095793,-49.8696455402477,
-25.));
#25559=CARTESIAN_POINT('Ctrl Pts',(-22.6775715875303,-49.7781166484613,
-25.));
#25560=CARTESIAN_POINT('Ctrl Pts',(-22.6586613112021,-49.6873369139881,
-25.));
#25561=CARTESIAN_POINT('Ctrl Pts',(-22.6353129020366,-49.5976928152581,
-25.));
#25562=CARTESIAN_POINT('Ctrl Pts',(-22.6123616860385,-49.5095737036597,
-25.));
#25563=CARTESIAN_POINT('Ctrl Pts',(-22.5851215841949,-49.4225511325324,
-25.));
#25564=CARTESIAN_POINT('Ctrl Pts',(-22.5536224723794,-49.3370212909107,
-25.));
#25565=CARTESIAN_POINT('Ctrl Pts',(-22.5377791669639,-49.2940018111589,
-25.));
#25566=CARTESIAN_POINT('Ctrl Pts',(-22.5208577966156,-49.251360504603,-25.));
#25567=CARTESIAN_POINT('Ctrl Pts',(-22.5028587458779,-49.2091515771324,
-25.));
#25568=CARTESIAN_POINT('Ctrl Pts',(-22.4972963310614,-49.1961073579137,
-25.));
#25569=CARTESIAN_POINT('Ctrl Pts',(-22.4916309765552,-49.1831044539104,
-25.));
#25570=CARTESIAN_POINT('Ctrl Pts',(-22.4858626529295,-49.1701445225163,
-25.));
#25571=CARTESIAN_POINT('Ctrl Pts',(-22.4801786597127,-49.1573740597418,
-25.));
#25572=CARTESIAN_POINT('Ctrl Pts',(-22.4743981571289,-49.1446531657103,
-25.));
#25573=CARTESIAN_POINT('Ctrl Pts',(-22.4685229605677,-49.1319863864487,
-25.));
#25574=CARTESIAN_POINT('Ctrl Pts',(-22.4310411834156,-49.0511765969249,
-25.));
#25575=CARTESIAN_POINT('Ctrl Pts',(-22.389689647437,-48.9725239641082,-25.));
#25576=CARTESIAN_POINT('Ctrl Pts',(-22.344538126016,-48.89637657445,-25.));
#25577=CARTESIAN_POINT('Ctrl Pts',(-22.3001458379325,-48.8215096208652,
-25.));
#25578=CARTESIAN_POINT('Ctrl Pts',(-22.2520798308501,-48.7490636963479,
-25.));
#25579=CARTESIAN_POINT('Ctrl Pts',(-22.2003702171762,-48.6794038046902,
-25.));
#25580=CARTESIAN_POINT('Ctrl Pts',(-22.150240791408,-48.6118726413384,-25.));
#25581=CARTESIAN_POINT('Ctrl Pts',(-22.0966866025685,-48.5469593952847,
-25.));
#25582=CARTESIAN_POINT('Ctrl Pts',(-22.039707393449,-48.4850369103578,-25.));
#25583=CARTESIAN_POINT('Ctrl Pts',(-22.018724090908,-48.4622331850097,-25.));
#25584=CARTESIAN_POINT('Ctrl Pts',(-21.9972760520149,-48.439835493521,-25.));
#25585=CARTESIAN_POINT('Ctrl Pts',(-21.9753624510336,-48.4178640718566,
-25.));
#25586=CARTESIAN_POINT('Ctrl Pts',(-21.9562845909508,-48.3987358734061,
-25.));
#25587=CARTESIAN_POINT('Ctrl Pts',(-21.9368538444216,-48.3799307827435,
-25.));
#25588=CARTESIAN_POINT('Ctrl Pts',(-21.9170803467229,-48.3614539181488,
-25.));
#25589=CARTESIAN_POINT('Origin',(-20.,-50.,-42.2084234471774));
#25590=CARTESIAN_POINT('Ctrl Pts',(-16.9232551256392,-49.9980895495447,
-39.7084234471775));
#25591=CARTESIAN_POINT('Ctrl Pts',(-16.9223299842891,-49.8748204265296,
-39.7020198504182));
#25592=CARTESIAN_POINT('Ctrl Pts',(-16.9848355034282,-48.7389612450556,
-39.6429667459281));
#25593=CARTESIAN_POINT('Ctrl Pts',(-18.3975850141438,-46.7464741122942,
-39.5312641337071));
#25594=CARTESIAN_POINT('Ctrl Pts',(-21.8481508174258,-46.8799262317611,
-39.3733156105146));
#25595=CARTESIAN_POINT('Ctrl Pts',(-23.623022297825,-49.8417650665615,-39.2153670873222));
#25596=CARTESIAN_POINT('Ctrl Pts',(-22.1130258164637,-52.9473164300811,
-39.0574185641297));
#25597=CARTESIAN_POINT('Ctrl Pts',(-18.6872049726298,-53.380502213004,-38.8994700409372));
#25598=CARTESIAN_POINT('Ctrl Pts',(-17.0406886962336,-51.4421741378802,
-38.7831383352865));
#25599=CARTESIAN_POINT('Ctrl Pts',(-16.923813258856,-50.2155563656135,-38.7194561373666));
#25600=CARTESIAN_POINT('Ctrl Pts',(-16.9257450511401,-50.0026845218917,
-38.7084234471775));
#25601=CARTESIAN_POINT('Ctrl Pts',(-16.9296932342852,-50.0033456701988,
-39.7915765528225));
#25602=CARTESIAN_POINT('Ctrl Pts',(-16.93470303559,-49.3102257217221,-39.7557520197534));
#25603=CARTESIAN_POINT('Ctrl Pts',(-17.5071826427202,-47.5885966321291,
-39.6672779789534));
#25604=CARTESIAN_POINT('Ctrl Pts',(-20.3515248249563,-46.3913860864081,
-39.5261544304226));
#25605=CARTESIAN_POINT('Ctrl Pts',(-23.2138549612499,-48.3201943023511,
-39.3682059072301));
#25606=CARTESIAN_POINT('Ctrl Pts',(-23.1634850140729,-51.7735630043146,
-39.2102573840376));
#25607=CARTESIAN_POINT('Ctrl Pts',(-20.2442744821096,-53.6181272821323,
-39.0523088608452));
#25608=CARTESIAN_POINT('Ctrl Pts',(-17.469492581831,-52.3497510624684,-38.9127485837735));
#25609=CARTESIAN_POINT('Ctrl Pts',(-16.9339707214102,-50.6610395236483,
-38.8258378144326));
#25610=CARTESIAN_POINT('Ctrl Pts',(-16.9296186885438,-49.9978504047438,
-38.7915765528226));
#25611=CARTESIAN_POINT('Ctrl Pts',(-21.913465996665,-48.364012796625,-40.));
#25612=CARTESIAN_POINT('Ctrl Pts',(-22.4546613829867,-48.9970000028465,
-39.9473504922692));
#25613=CARTESIAN_POINT('Ctrl Pts',(-22.8504302036551,-50.831572053257,-39.8420514768075));
#25614=CARTESIAN_POINT('Ctrl Pts',(-20.8590118257495,-52.8453303030972,
-39.6841029536151));
#25615=CARTESIAN_POINT('Ctrl Pts',(-18.0884180617819,-52.2727938259679,
-39.5261544304226));
#25616=CARTESIAN_POINT('Ctrl Pts',(-17.0511987917854,-49.6427658750915,
-39.3682059072301));
#25617=CARTESIAN_POINT('Ctrl Pts',(-18.6874638923401,-47.3350410208884,
-39.2102573840377));
#25618=CARTESIAN_POINT('Ctrl Pts',(-21.5138180194792,-47.4443514847759,
-39.0523088608452));
#25619=CARTESIAN_POINT('Ctrl Pts',(-22.9676130257929,-49.8703899642324,
-38.8943603376527));
#25620=CARTESIAN_POINT('Ctrl Pts',(-21.7307767993972,-52.4141431959425,
-38.7364118144602));
#25621=CARTESIAN_POINT('Ctrl Pts',(-18.9246912375453,-52.7689651281072,
-38.5784632912678));
#25622=CARTESIAN_POINT('Ctrl Pts',(-17.0935587667564,-50.6133013619587,
-38.4205147680753));
#25623=CARTESIAN_POINT('Ctrl Pts',(-17.8976064891825,-47.9015504057097,
-38.2625662448829));
#25624=CARTESIAN_POINT('Ctrl Pts',(-20.6078313089819,-47.09241268106,-38.1046177216904));
#25625=CARTESIAN_POINT('Ctrl Pts',(-22.7669535441375,-48.9194895166619,
-37.9466691984979));
#25626=CARTESIAN_POINT('Ctrl Pts',(-22.4173633664285,-51.726235575411,-37.7887206753054));
#25627=CARTESIAN_POINT('Ctrl Pts',(-19.876023238429,-52.9678547167293,-37.630772152113));
#25628=CARTESIAN_POINT('Ctrl Pts',(-17.4470891231681,-51.5186110643773,
-37.4728236289205));
#25629=CARTESIAN_POINT('Ctrl Pts',(-17.3328016297339,-48.6924885372187,
-37.314875105728));
#25630=CARTESIAN_POINT('Ctrl Pts',(-19.6367817929697,-47.0518470927161,
-37.1569265825355));
#25631=CARTESIAN_POINT('Ctrl Pts',(-22.2700808509466,-48.0842061220133,
-36.9989780593431));
#25632=CARTESIAN_POINT('Ctrl Pts',(-22.845166646169,-50.8535572460832,-36.8410295361506));
#25633=CARTESIAN_POINT('Ctrl Pts',(-20.840626373429,-52.8490139488643,-36.6830810129582));
#25634=CARTESIAN_POINT('Ctrl Pts',(-18.0739157352567,-52.2613563661284,
-36.5251324897657));
#25635=CARTESIAN_POINT('Ctrl Pts',(-17.0535271202902,-49.6233957357017,
-36.3671839665733));
#25636=CARTESIAN_POINT('Ctrl Pts',(-18.7046158526517,-47.3268907411116,
-36.2092354433807));
#25637=CARTESIAN_POINT('Ctrl Pts',(-21.530189993977,-47.454012610956,-36.0512869201883));
#25638=CARTESIAN_POINT('Ctrl Pts',(-22.9683874064431,-49.8895038145725,
-35.8933383969959));
#25639=CARTESIAN_POINT('Ctrl Pts',(-21.7152382368816,-52.4251785485085,
-35.7353898738033));
#25640=CARTESIAN_POINT('Ctrl Pts',(-18.9069347245663,-52.7620176511933,
-35.5774413506109));
#25641=CARTESIAN_POINT('Ctrl Pts',(-17.0896802534022,-50.5946193524052,
-35.4194928274184));
#25642=CARTESIAN_POINT('Ctrl Pts',(-17.9111241831078,-47.8880977713745,
-35.261544304226));
#25643=CARTESIAN_POINT('Ctrl Pts',(-20.6264882857017,-47.096373710409,-35.1035957810335));
#25644=CARTESIAN_POINT('Ctrl Pts',(-22.7738345134306,-48.9372792964274,
-34.945647257841));
#25645=CARTESIAN_POINT('Ctrl Pts',(-22.4062293501948,-51.7417214231792,
-34.7876987346485));
#25646=CARTESIAN_POINT('Ctrl Pts',(-19.8569692172952,-52.9669977076003,
-34.6297502114561));
#25647=CARTESIAN_POINT('Ctrl Pts',(-17.4373907449893,-51.5021874076948,
-34.4718016882636));
#25648=CARTESIAN_POINT('Ctrl Pts',(-17.3412521459643,-48.675389472198,-34.3138531650712));
#25649=CARTESIAN_POINT('Ctrl Pts',(-19.6557193640327,-47.0495756160508,
-34.1559046418787));
#25650=CARTESIAN_POINT('Ctrl Pts',(-22.2823353639105,-48.0988218157291,
-33.9979561186862));
#25651=CARTESIAN_POINT('Ctrl Pts',(-22.839627303423,-50.8718084533652,-33.8400075954937));
#25652=CARTESIAN_POINT('Ctrl Pts',(-20.8223155302823,-52.8543528811905,
-33.6820590723013));
#25653=CARTESIAN_POINT('Ctrl Pts',(-18.059435275431,-52.2489423628591,-33.5241105491088));
#25654=CARTESIAN_POINT('Ctrl Pts',(-17.0560060367383,-49.6044842026135,
-33.3661620259163));
#25655=CARTESIAN_POINT('Ctrl Pts',(-18.7218065870059,-47.318628186789,-33.2082135027239));
#25656=CARTESIAN_POINT('Ctrl Pts',(-21.54650623034,-47.4638904437655,-33.0502649795314));
#25657=CARTESIAN_POINT('Ctrl Pts',(-22.9690357094856,-49.9085661030944,
-32.8923164563389));
#25658=CARTESIAN_POINT('Ctrl Pts',(-21.6996308099799,-52.4361420959114,
-32.7343679331465));
#25659=CARTESIAN_POINT('Ctrl Pts',(-18.8892223469998,-52.754942142278,-32.576419409954));
#25660=CARTESIAN_POINT('Ctrl Pts',(-17.0859221992198,-50.575919936019,-32.4184708867615));
#25661=CARTESIAN_POINT('Ctrl Pts',(-17.9247277657372,-47.8747286395846,
-32.260522363569));
#25662=CARTESIAN_POINT('Ctrl Pts',(-20.6451195505088,-47.1004562484323,
-32.1025738403766));
#25663=CARTESIAN_POINT('Ctrl Pts',(-22.7806010592582,-48.9551119911895,
-31.9446253171841));
#25664=CARTESIAN_POINT('Ctrl Pts',(-22.3949961557367,-51.757135912703,-31.7866767939917));
#25665=CARTESIAN_POINT('Ctrl Pts',(-19.8379210783241,-52.9660181430417,
-31.6287282707992));
#25666=CARTESIAN_POINT('Ctrl Pts',(-17.4277980297875,-51.4857019304486,
-31.4707797476067));
#25667=CARTESIAN_POINT('Ctrl Pts',(-17.3498122776559,-48.6583449630995,
-31.3128312244143));
#25668=CARTESIAN_POINT('Ctrl Pts',(-19.6746711315577,-47.0474258131146,
-31.1548827012217));
#25669=CARTESIAN_POINT('Ctrl Pts',(-22.2944957760458,-48.1135158798941,
-30.9969341780293));
#25670=CARTESIAN_POINT('Ctrl Pts',(-22.8339708843277,-50.8900237235527,
-30.8389856548368));
#25671=CARTESIAN_POINT('Ctrl Pts',(-20.803970783118,-52.8595741259139,-30.6810371316444));
#25672=CARTESIAN_POINT('Ctrl Pts',(-18.0450348245211,-52.2364356383248,
-30.5230886084519));
#25673=CARTESIAN_POINT('Ctrl Pts',(-17.058606332953,-49.5855889755817,-30.3651400852594));
#25674=CARTESIAN_POINT('Ctrl Pts',(-18.7390500208516,-47.3104761849374,
-30.207191562067));
#25675=CARTESIAN_POINT('Ctrl Pts',(-21.5627587047845,-47.4738728392405,
-30.0492430388745));
#25676=CARTESIAN_POINT('Ctrl Pts',(-22.9695616002458,-49.9276321615209,
-29.891294515682));
#25677=CARTESIAN_POINT('Ctrl Pts',(-21.6839533078998,-52.4470052019794,
-29.7333459924896));
#25678=CARTESIAN_POINT('Ctrl Pts',(-18.8715557664016,-52.7477530481074,
-29.5753974692971));
#25679=CARTESIAN_POINT('Ctrl Pts',(-17.0822842914354,-50.5571967746374,
-29.4174489461046));
#25680=CARTESIAN_POINT('Ctrl Pts',(-17.9384169110962,-47.8614471319982,
-29.2595004229121));
#25681=CARTESIAN_POINT('Ctrl Pts',(-20.6637242172836,-47.1046583335895,
-29.1015518997197));
#25682=CARTESIAN_POINT('Ctrl Pts',(-22.7872529618541,-48.9729877663616,
-28.9436033765272));
#25683=CARTESIAN_POINT('Ctrl Pts',(-22.3836642165086,-51.7724779560436,
-28.7856548533348));
#25684=CARTESIAN_POINT('Ctrl Pts',(-19.8188796216655,-52.9649162907898,
-28.6277063301422));
#25685=CARTESIAN_POINT('Ctrl Pts',(-17.4183113658474,-51.469155197875,-28.4697578069498));
#25686=CARTESIAN_POINT('Ctrl Pts',(-17.3584816750768,-48.641355770686,-28.3118092837573));
#25687=CARTESIAN_POINT('Ctrl Pts',(-19.6936363134129,-47.0453977423244,
-28.1538607605649));
#25688=CARTESIAN_POINT('Ctrl Pts',(-22.3065615846713,-48.1282877259989,
-27.9959122373724));
#25689=CARTESIAN_POINT('Ctrl Pts',(-22.8281976261233,-50.9082022926661,
-27.8379637141799));
#25690=CARTESIAN_POINT('Ctrl Pts',(-20.7855928795529,-52.8646774827825,
-27.6800151909875));
#25691=CARTESIAN_POINT('Ctrl Pts',(-18.0307149939936,-52.2238366836986,
-27.522066667795));
#25692=CARTESIAN_POINT('Ctrl Pts',(-17.0613278662217,-49.5667108796552,
-27.3641181446025));
#25693=CARTESIAN_POINT('Ctrl Pts',(-18.7563455140292,-47.3024349814285,
-27.2061696214101));
#25694=CARTESIAN_POINT('Ctrl Pts',(-21.5789466062486,-47.4839595647848,
-27.0482210982176));
#25695=CARTESIAN_POINT('Ctrl Pts',(-22.9699653377665,-49.9467008477527,
-26.8902725750251));
#25696=CARTESIAN_POINT('Ctrl Pts',(-21.6682058180543,-52.457768127515,-26.7323240518326));
#25697=CARTESIAN_POINT('Ctrl Pts',(-18.8539368241228,-52.7404492541073,
-26.5743755286402));
#25698=CARTESIAN_POINT('Ctrl Pts',(-17.078764464007,-50.5384534495725,-26.4164270054477));
#25699=CARTESIAN_POINT('Ctrl Pts',(-17.9521954671408,-47.8482482024917,
-26.2584784822553));
#25700=CARTESIAN_POINT('Ctrl Pts',(-20.682292733498,-47.1089909302976,-26.1005299590627));
#25701=CARTESIAN_POINT('Ctrl Pts',(-22.7938074397502,-48.990883708662,-25.9425814358704));
#25702=CARTESIAN_POINT('Ctrl Pts',(-22.3721991697247,-51.7877910759886,
-25.7846329126778));
#25703=CARTESIAN_POINT('Ctrl Pts',(-19.7999149827311,-52.9636042777895,
-25.6266843894854));
#25704=CARTESIAN_POINT('Ctrl Pts',(-17.4087930587084,-51.4527229542004,
-25.4687358662929));
#25705=CARTESIAN_POINT('Ctrl Pts',(-17.3675349459595,-48.6240739391879,
-25.3107873431004));
#25706=CARTESIAN_POINT('Ctrl Pts',(-19.7120663609263,-47.0441868290824,
-25.152838819908));
#25707=CARTESIAN_POINT('Ctrl Pts',(-22.3196265018743,-48.1417377089596,
-24.9948902967155));
#25708=CARTESIAN_POINT('Ctrl Pts',(-22.8200820083521,-50.9293018303199,
-24.836941773523));
#25709=CARTESIAN_POINT('Ctrl Pts',(-21.4547503964622,-52.2169963426693,
-24.7316427580614));
#25710=CARTESIAN_POINT('Ctrl Pts',(-20.6501999979751,-52.4320868020351,
-24.6789932503306));
#25711=CARTESIAN_POINT('Ctrl Pts',(-22.0543315503421,-48.2435746787731,
-40.1070022498898));
#25712=CARTESIAN_POINT('Ctrl Pts',(-22.6353686625551,-48.9231611417519,
-40.054352742159));
#25713=CARTESIAN_POINT('Ctrl Pts',(-23.0602731951456,-50.8927907307295,
-39.9490537266973));
#25714=CARTESIAN_POINT('Ctrl Pts',(-20.9222505645932,-53.0547978500713,
-39.7911052035049));
#25715=CARTESIAN_POINT('Ctrl Pts',(-17.9476912087333,-52.4401123783993,
-39.6331566803124));
#25716=CARTESIAN_POINT('Ctrl Pts',(-16.8341139229649,-49.6164670106824,
-39.4752081571199));
#25717=CARTESIAN_POINT('Ctrl Pts',(-18.590837599608,-47.138852051357,-39.3172596339275));
#25718=CARTESIAN_POINT('Ctrl Pts',(-21.6252622854614,-47.2562097337709,
-39.159311110735));
#25719=CARTESIAN_POINT('Ctrl Pts',(-23.1860827831369,-49.8608483316754,
-39.0013625875425));
#25720=CARTESIAN_POINT('Ctrl Pts',(-21.8581931384194,-52.5918676073221,
-38.84341406435));
#25721=CARTESIAN_POINT('Ctrl Pts',(-18.8455291492401,-52.9728108230729,
-38.6854655411576));
#25722=CARTESIAN_POINT('Ctrl Pts',(-16.8795923548817,-50.6584513860896,
-38.5275170179651));
#25723=CARTESIAN_POINT('Ctrl Pts',(-17.7428324683928,-47.7470667281956,
-38.3695684947727));
#25724=CARTESIAN_POINT('Ctrl Pts',(-20.652578638713,-46.8783618966402,-38.2116199715802));
#25725=CARTESIAN_POINT('Ctrl Pts',(-22.9706511502998,-48.8399444880308,
-38.0536714483877));
#25726=CARTESIAN_POINT('Ctrl Pts',(-22.5953248403423,-51.8533175985726,
-37.8957229251952));
#25727=CARTESIAN_POINT('Ctrl Pts',(-19.8668963162929,-53.1863422668785,
-37.7377744020028));
#25728=CARTESIAN_POINT('Ctrl Pts',(-17.2591489116463,-51.6304081847737,
-37.5798258788103));
#25729=CARTESIAN_POINT('Ctrl Pts',(-17.1364478006882,-48.5962321488299,
-37.4218773556179));
#25730=CARTESIAN_POINT('Ctrl Pts',(-19.6100423923594,-46.8348099505181,
-37.2639288324254));
#25731=CARTESIAN_POINT('Ctrl Pts',(-22.4371996795631,-47.9431691943522,
-37.1059803092329));
#25732=CARTESIAN_POINT('Ctrl Pts',(-23.0546221450462,-50.9163944296412,
-36.9480317860405));
#25733=CARTESIAN_POINT('Ctrl Pts',(-20.9025116119098,-53.0587526784993,
-36.790083262848));
#25734=CARTESIAN_POINT('Ctrl Pts',(-17.9321212498284,-52.427832915558,-36.6321347396555));
#25735=CARTESIAN_POINT('Ctrl Pts',(-16.8366136583745,-49.5956708802301,
-36.474186216463));
#25736=CARTESIAN_POINT('Ctrl Pts',(-18.6092522530588,-47.1301017642242,
-36.3162376932706));
#25737=CARTESIAN_POINT('Ctrl Pts',(-21.6428395320971,-47.2665820928086,
-36.1582891700781));
#25738=CARTESIAN_POINT('Ctrl Pts',(-23.1869141721474,-49.881369305589,-36.0003406468857));
#25739=CARTESIAN_POINT('Ctrl Pts',(-21.8415106578954,-52.6037153605536,
-35.8423921236932));
#25740=CARTESIAN_POINT('Ctrl Pts',(-18.8264654371594,-52.9653518867529,
-35.6844436005007));
#25741=CARTESIAN_POINT('Ctrl Pts',(-16.8754283131031,-50.6383940442208,
-35.5264950773082));
#25742=CARTESIAN_POINT('Ctrl Pts',(-17.7573453080079,-47.7326237377279,
-35.3685465541157));
#25743=CARTESIAN_POINT('Ctrl Pts',(-20.6726091048808,-46.8826145290767,
-35.2105980309233));
#25744=CARTESIAN_POINT('Ctrl Pts',(-22.9780386828404,-48.8590439159327,
-35.0526495077308));
#25745=CARTESIAN_POINT('Ctrl Pts',(-22.5833711600205,-51.8699434835947,
-34.8947009845384));
#25746=CARTESIAN_POINT('Ctrl Pts',(-19.8464395760924,-53.1854221664451,
-34.7367524613459));
#25747=CARTESIAN_POINT('Ctrl Pts',(-17.248736558192,-51.6127754512139,-34.5788039381534));
#25748=CARTESIAN_POINT('Ctrl Pts',(-17.1455204270839,-48.577874284716,-34.4208554149609));
#25749=CARTESIAN_POINT('Ctrl Pts',(-19.6303741096669,-46.8323712522672,
-34.2629068917685));
#25750=CARTESIAN_POINT('Ctrl Pts',(-22.4503563453516,-47.9588608663144,
-34.104958368576));
#25751=CARTESIAN_POINT('Ctrl Pts',(-23.0486750069255,-50.9359892544338,
-33.9470098453836));
#25752=CARTESIAN_POINT('Ctrl Pts',(-20.882852760979,-53.0644846523845,-33.789061322191));
#25753=CARTESIAN_POINT('Ctrl Pts',(-17.9165747674058,-52.4145050181057,
-33.6311127989986));
#25754=CARTESIAN_POINT('Ctrl Pts',(-16.8392750677116,-49.5753671177612,
-33.4731642758062));
#25755=CARTESIAN_POINT('Ctrl Pts',(-18.6277085350199,-47.1212309371173,
-33.3152157526137));
#25756=CARTESIAN_POINT('Ctrl Pts',(-21.6603569372674,-47.2771871119858,
-33.1572672294212));
#25757=CARTESIAN_POINT('Ctrl Pts',(-23.1876102019681,-49.9018349218062,
-32.9993187062287));
#25758=CARTESIAN_POINT('Ctrl Pts',(-21.8247542433263,-52.615486022469,-32.8413701830363));
#25759=CARTESIAN_POINT('Ctrl Pts',(-18.8074491096521,-52.9577554929707,
-32.6834216598438));
#25760=CARTESIAN_POINT('Ctrl Pts',(-16.8713935984606,-50.6183180140628,
-32.5254731366514));
#25761=CARTESIAN_POINT('Ctrl Pts',(-17.7719503592824,-47.7182703970965,
-32.3675246134588));
#25762=CARTESIAN_POINT('Ctrl Pts',(-20.6926119662761,-46.8869976154139,
-32.2095760902664));
#25763=CARTESIAN_POINT('Ctrl Pts',(-22.9853033682881,-48.8781894181476,
-32.0516275670739));
#25764=CARTESIAN_POINT('Ctrl Pts',(-22.5713110001709,-51.8864927571205,
-31.8936790438815));
#25765=CARTESIAN_POINT('Ctrl Pts',(-19.8259891510878,-53.1843704882957,
-31.735730520689));
#25766=CARTESIAN_POINT('Ctrl Pts',(-17.2384376464126,-51.5950763459838,
-31.5777819974965));
#25767=CARTESIAN_POINT('Ctrl Pts',(-17.1547107386128,-48.5595749928225,
-31.4198334743041));
#25768=CARTESIAN_POINT('Ctrl Pts',(-19.6507210685515,-46.8300631851227,
-31.2618849511116));
#25769=CARTESIAN_POINT('Ctrl Pts',(-22.4634119827961,-47.9746366782021,
-31.1039364279191));
#25770=CARTESIAN_POINT('Ctrl Pts',(-23.0426021735282,-50.9555454965146,
-30.9459879047266));
#25771=CARTESIAN_POINT('Ctrl Pts',(-20.8631575100844,-53.07009027474,-30.7880393815342));
#25772=CARTESIAN_POINT('Ctrl Pts',(-17.901114183996,-52.4010775734335,-30.6300908583417));
#25773=CARTESIAN_POINT('Ctrl Pts',(-16.8420667925521,-49.5550808617682,
-30.4721423351492));
#25774=CARTESIAN_POINT('Ctrl Pts',(-18.6462213961039,-47.112478801134,-30.3141938119568));
#25775=CARTESIAN_POINT('Ctrl Pts',(-21.6778058864939,-47.2879043915235,
-30.1562452887643));
#25776=CARTESIAN_POINT('Ctrl Pts',(-23.1881748077581,-49.9223045854607,
-29.9982967655718));
#25777=CARTESIAN_POINT('Ctrl Pts',(-21.8079225947839,-52.6271488487587,
-29.8403482423794));
#25778=CARTESIAN_POINT('Ctrl Pts',(-18.7884819505949,-52.9500371520131,
-29.6823997191869));
#25779=CARTESIAN_POINT('Ctrl Pts',(-16.8674878751545,-50.5982164908504,
-29.5244511959945));
#25780=CARTESIAN_POINT('Ctrl Pts',(-17.7866472722441,-47.704011131388,-29.366502672802));
#25781=CARTESIAN_POINT('Ctrl Pts',(-20.7125862715451,-46.8915090497067,
-29.2085541496095));
#25782=CARTESIAN_POINT('Ctrl Pts',(-22.9924449706976,-48.8973811722666,
-29.0506056264171));
#25783=CARTESIAN_POINT('Ctrl Pts',(-22.5591448261582,-51.9029642511193,
-28.8926571032245));
#25784=CARTESIAN_POINT('Ctrl Pts',(-19.8055459003343,-53.1831875198767,
-28.7347085800321));
#25785=CARTESIAN_POINT('Ctrl Pts',(-17.2282525931775,-51.5773114759311,
-28.5767600568396));
#25786=CARTESIAN_POINT('Ctrl Pts',(-17.1640183597962,-48.5413350899183,
-28.4188115336472));
#25787=CARTESIAN_POINT('Ctrl Pts',(-19.6710824293027,-46.8278858118023,
-28.2608630104547));
#25788=CARTESIAN_POINT('Ctrl Pts',(-22.4763660522088,-47.990495998181,-28.1029144872622));
#25789=CARTESIAN_POINT('Ctrl Pts',(-23.0364038995592,-50.9750623356614,
-27.9449659640698));
#25790=CARTESIAN_POINT('Ctrl Pts',(-20.8434266618807,-53.0755693305717,
-27.7870174408773));
#25791=CARTESIAN_POINT('Ctrl Pts',(-17.8857401560804,-52.3875511088739,
-27.6290689176848));
#25792=CARTESIAN_POINT('Ctrl Pts',(-16.8449886796767,-49.5348129980383,
-27.4711203944923));
#25793=CARTESIAN_POINT('Ctrl Pts',(-18.6647901490243,-47.1038456202467,
-27.3131718712999));
#25794=CARTESIAN_POINT('Ctrl Pts',(-21.6951855090058,-47.2987336817025,
-27.1552233481074));
#25795=CARTESIAN_POINT('Ctrl Pts',(-23.1886082676306,-49.9427770703744,
-26.9972748249149));
#25796=CARTESIAN_POINT('Ctrl Pts',(-21.7910158061163,-52.6387041194248,
-26.8393263017225));
#25797=CARTESIAN_POINT('Ctrl Pts',(-18.769565936895,-52.9421956672531,-26.68137777853));
#25798=CARTESIAN_POINT('Ctrl Pts',(-16.8637089250448,-50.5780933195443,
-26.5234292553376));
#25799=CARTESIAN_POINT('Ctrl Pts',(-17.8014401781279,-47.6898405229929,
-26.365480732145));
#25800=CARTESIAN_POINT('Ctrl Pts',(-20.7325217649214,-46.8961606035508,
-26.2075322089526));
#25801=CARTESIAN_POINT('Ctrl Pts',(-22.9994819761952,-48.9165945781775,
-26.0495836857601));
#25802=CARTESIAN_POINT('Ctrl Pts',(-22.5468357454767,-51.9194046924401,
-25.8916351625677));
#25803=CARTESIAN_POINT('Ctrl Pts',(-19.7851851224727,-53.1817789190938,
-25.7336866393752));
#25804=CARTESIAN_POINT('Ctrl Pts',(-17.2180335672343,-51.559669523222,-25.5757381161827));
#25805=CARTESIAN_POINT('Ctrl Pts',(-17.1737381144405,-48.522781004423,-25.4177895929902));
#25806=CARTESIAN_POINT('Ctrl Pts',(-19.6908692601881,-46.8265857535405,
-25.2598410697978));
#25807=CARTESIAN_POINT('Ctrl Pts',(-22.4903927825817,-48.0049361420853,
-25.1018925466053));
#25808=CARTESIAN_POINT('Ctrl Pts',(-23.0276908261798,-50.9977151792319,
-24.9439440234128));
#25809=CARTESIAN_POINT('Ctrl Pts',(-21.561846221743,-52.3802071955689,-24.8386450079512));
#25810=CARTESIAN_POINT('Ctrl Pts',(-20.698066426161,-52.6111321859386,-24.7859955002204));
#25811=CARTESIAN_POINT('Ctrl Pts',(-22.1951971040191,-48.1231365609212,
-40.2140044997796));
#25812=CARTESIAN_POINT('Ctrl Pts',(-22.8160759421236,-48.8493222806572,
-40.1613549920488));
#25813=CARTESIAN_POINT('Ctrl Pts',(-23.2701161866361,-50.9540094082019,
-40.0560559765871));
#25814=CARTESIAN_POINT('Ctrl Pts',(-20.9854893034369,-53.2642653970455,
-39.8981074533947));
#25815=CARTESIAN_POINT('Ctrl Pts',(-17.8069643556847,-52.6074309308307,
-39.7401589302022));
#25816=CARTESIAN_POINT('Ctrl Pts',(-16.6170290541443,-49.5901681462734,
-39.5822104070097));
#25817=CARTESIAN_POINT('Ctrl Pts',(-18.4942113068759,-46.9426630818256,
-39.4242618838173));
#25818=CARTESIAN_POINT('Ctrl Pts',(-21.7367065514436,-47.068067982766,-39.2663133606248));
#25819=CARTESIAN_POINT('Ctrl Pts',(-23.4045525404809,-49.8513066991185,
-39.1083648374324));
#25820=CARTESIAN_POINT('Ctrl Pts',(-21.9856094774415,-52.7695920187016,
-38.9504163142398));
#25821=CARTESIAN_POINT('Ctrl Pts',(-18.7663670609349,-53.1766565180384,
-38.7924677910474));
#25822=CARTESIAN_POINT('Ctrl Pts',(-16.665625943007,-50.7036014102206,-38.6345192678549));
#25823=CARTESIAN_POINT('Ctrl Pts',(-17.5880584476031,-47.5925830506814,
-38.4765707446625));
#25824=CARTESIAN_POINT('Ctrl Pts',(-20.697325968444,-46.6643111122205,-38.31862222147));
#25825=CARTESIAN_POINT('Ctrl Pts',(-23.1743487564621,-48.7603994593997,
-38.1606736982775));
#25826=CARTESIAN_POINT('Ctrl Pts',(-22.7732863142562,-51.9803996217343,
-38.002725175085));
#25827=CARTESIAN_POINT('Ctrl Pts',(-19.8577693941567,-53.4048298170276,
-37.8447766518926));
#25828=CARTESIAN_POINT('Ctrl Pts',(-17.0712087001245,-51.7422053051701,
-37.6868281287001));
#25829=CARTESIAN_POINT('Ctrl Pts',(-16.9400939716425,-48.4999757604411,
-37.5288796055077));
#25830=CARTESIAN_POINT('Ctrl Pts',(-19.5833029917492,-46.6177728083202,
-37.3709310823152));
#25831=CARTESIAN_POINT('Ctrl Pts',(-22.6043185081796,-47.802132266691,-37.2129825591227));
#25832=CARTESIAN_POINT('Ctrl Pts',(-23.2640776439233,-50.9792316131993,
-37.0550340359303));
#25833=CARTESIAN_POINT('Ctrl Pts',(-20.9643968503907,-53.2684914081344,
-36.8970855127378));
#25834=CARTESIAN_POINT('Ctrl Pts',(-17.7903267644001,-52.5943094649876,
-36.7391369895453));
#25835=CARTESIAN_POINT('Ctrl Pts',(-16.6197001964587,-49.5679460247584,
-36.5811884663529));
#25836=CARTESIAN_POINT('Ctrl Pts',(-18.5138886534658,-46.9333127873368,
-36.4232399431604));
#25837=CARTESIAN_POINT('Ctrl Pts',(-21.755489070217,-47.0791515746612,-36.2652914199679));
#25838=CARTESIAN_POINT('Ctrl Pts',(-23.4054409378518,-49.8732347966055,
-36.1073428967755));
#25839=CARTESIAN_POINT('Ctrl Pts',(-21.9677830789091,-52.7822521725988,
-35.9493943735829));
#25840=CARTESIAN_POINT('Ctrl Pts',(-18.7459961497524,-53.1686861223123,
-35.7914458503905));
#25841=CARTESIAN_POINT('Ctrl Pts',(-16.6611763728041,-50.6821687360365,
-35.633497327198));
#25842=CARTESIAN_POINT('Ctrl Pts',(-17.603566432908,-47.5771497040813,-35.4755488040056));
#25843=CARTESIAN_POINT('Ctrl Pts',(-20.7187299240599,-46.6688553477443,
-35.3176002808131));
#25844=CARTESIAN_POINT('Ctrl Pts',(-23.1822428522502,-48.780808535438,-35.1596517576206));
#25845=CARTESIAN_POINT('Ctrl Pts',(-22.7605129698462,-51.9981655440101,
-35.0017032344282));
#25846=CARTESIAN_POINT('Ctrl Pts',(-19.8359099348896,-53.4038466252901,
-34.8437547112357));
#25847=CARTESIAN_POINT('Ctrl Pts',(-17.0600823713948,-51.7233634947331,
-34.6858061880432));
#25848=CARTESIAN_POINT('Ctrl Pts',(-16.9497887082035,-48.4803590972339,
-34.5278576648508));
#25849=CARTESIAN_POINT('Ctrl Pts',(-19.6050288553011,-46.6151668884836,
-34.3699091416583));
#25850=CARTESIAN_POINT('Ctrl Pts',(-22.6183773267928,-47.8188999168997,
-34.2119606184658));
#25851=CARTESIAN_POINT('Ctrl Pts',(-23.2577227104281,-51.0001700555025,
-34.0540120952734));
#25852=CARTESIAN_POINT('Ctrl Pts',(-20.9433899916757,-53.2746164235783,
-33.8960635720809));
#25853=CARTESIAN_POINT('Ctrl Pts',(-17.7737142593806,-52.5800676733523,
-33.7381150488884));
#25854=CARTESIAN_POINT('Ctrl Pts',(-16.622544098685,-49.5462500329089,-33.580166525696));
#25855=CARTESIAN_POINT('Ctrl Pts',(-18.5336104830338,-46.9238336874456,
-33.4222180025035));
#25856=CARTESIAN_POINT('Ctrl Pts',(-21.7742076441947,-47.0904837802061,
-33.264269479311));
#25857=CARTESIAN_POINT('Ctrl Pts',(-23.4061846944506,-49.895103740518,-33.1063209561185));
#25858=CARTESIAN_POINT('Ctrl Pts',(-21.9498776766727,-52.7948299490266,
-32.9483724329261));
#25859=CARTESIAN_POINT('Ctrl Pts',(-18.7256758723045,-53.1605688436634,
-32.7904239097336));
#25860=CARTESIAN_POINT('Ctrl Pts',(-16.6568649977014,-50.6607160921068,
-32.6324753865411));
#25861=CARTESIAN_POINT('Ctrl Pts',(-17.6191729528276,-47.5618121546085,
-32.4745268633487));
#25862=CARTESIAN_POINT('Ctrl Pts',(-20.7401043820435,-46.6735389823955,
-32.3165783401562));
#25863=CARTESIAN_POINT('Ctrl Pts',(-23.1900056773179,-48.8012668451058,
-32.1586298169638));
#25864=CARTESIAN_POINT('Ctrl Pts',(-22.7476258446051,-52.0158496015379,
-32.0006812937712));
#25865=CARTESIAN_POINT('Ctrl Pts',(-19.8140572238516,-53.4027228335498,
-31.8427327705788));
#25866=CARTESIAN_POINT('Ctrl Pts',(-17.0490772630378,-51.7044507615189,
-31.6847842473863));
#25867=CARTESIAN_POINT('Ctrl Pts',(-16.9596091995696,-48.4608050225456,
-31.5268357241939));
#25868=CARTESIAN_POINT('Ctrl Pts',(-19.6267710055454,-46.6127005571309,
-31.3688872010014));
#25869=CARTESIAN_POINT('Ctrl Pts',(-22.6323281895464,-47.83575747651,-31.2109386778089));
#25870=CARTESIAN_POINT('Ctrl Pts',(-23.2512334627286,-51.0210672694766,
-31.0529901546164));
#25871=CARTESIAN_POINT('Ctrl Pts',(-20.9223442370508,-53.2806064235659,
-30.895041631424));
#25872=CARTESIAN_POINT('Ctrl Pts',(-17.7571935434708,-52.5657195085423,
-30.7370931082315));
#25873=CARTESIAN_POINT('Ctrl Pts',(-16.6255272521511,-49.5245727479546,
-30.5791445850391));
#25874=CARTESIAN_POINT('Ctrl Pts',(-18.5533927713563,-46.9144814173307,
-30.4211960618466));
#25875=CARTESIAN_POINT('Ctrl Pts',(-21.7928530682033,-47.1019359438065,
-30.2632475386541));
#25876=CARTESIAN_POINT('Ctrl Pts',(-23.4067880152704,-49.9169770094005,
-30.1052990154616));
#25877=CARTESIAN_POINT('Ctrl Pts',(-21.931891881668,-52.807292495538,-29.9473504922692));
#25878=CARTESIAN_POINT('Ctrl Pts',(-18.7054081347881,-53.1523212559188,
-29.7894019690767));
#25879=CARTESIAN_POINT('Ctrl Pts',(-16.6526914588735,-50.6392362070634,
-29.6314534458842));
#25880=CARTESIAN_POINT('Ctrl Pts',(-17.6348776333921,-47.5465751307778,
-29.4735049226918));
#25881=CARTESIAN_POINT('Ctrl Pts',(-20.7614483258065,-46.6783597658239,
-29.3155563994993));
#25882=CARTESIAN_POINT('Ctrl Pts',(-23.1976369795411,-48.8217745781716,
-29.1576078763068));
#25883=CARTESIAN_POINT('Ctrl Pts',(-22.7346254358078,-52.0334505461951,
-28.9996593531144));
#25884=CARTESIAN_POINT('Ctrl Pts',(-19.7922121790031,-53.4014587489637,
-28.8417108299219));
#25885=CARTESIAN_POINT('Ctrl Pts',(-17.0381938205077,-51.6854677539872,
-28.6837623067294));
#25886=CARTESIAN_POINT('Ctrl Pts',(-16.9695550445155,-48.4413144091505,
-28.525813783537));
#25887=CARTESIAN_POINT('Ctrl Pts',(-19.6485285451925,-46.6103738812803,
-28.3678652603445));
#25888=CARTESIAN_POINT('Ctrl Pts',(-22.6461705197463,-47.8527042703631,
-28.209916737152));
#25889=CARTESIAN_POINT('Ctrl Pts',(-23.2446101729951,-51.0419223786568,
-28.0519682139596));
#25890=CARTESIAN_POINT('Ctrl Pts',(-20.9012604442086,-53.2864611783608,
-27.8940196907671));
#25891=CARTESIAN_POINT('Ctrl Pts',(-17.7407653181672,-52.5512655340492,
-27.7360711675746));
#25892=CARTESIAN_POINT('Ctrl Pts',(-16.6286494931318,-49.5029151164213,
-27.5781226443821));
#25893=CARTESIAN_POINT('Ctrl Pts',(-18.5732347840193,-46.9052562590649,
-27.4201741211897));
#25894=CARTESIAN_POINT('Ctrl Pts',(-21.8114244117631,-47.11350779862,-27.2622255979972));
#25895=CARTESIAN_POINT('Ctrl Pts',(-23.4072511974946,-49.9388532929962,
-27.1042770748047));
#25896=CARTESIAN_POINT('Ctrl Pts',(-21.9138257941783,-52.8196401113345,
-26.9463285516123));
#25897=CARTESIAN_POINT('Ctrl Pts',(-18.6851950496672,-53.1439420803989,
-26.7883800284198));
#25898=CARTESIAN_POINT('Ctrl Pts',(-16.6486533860826,-50.6177331895161,
-26.6304315052273));
#25899=CARTESIAN_POINT('Ctrl Pts',(-17.6506848891151,-47.5314328434942,
-26.4724829820349));
#25900=CARTESIAN_POINT('Ctrl Pts',(-20.7827507963447,-46.6833302768041,
-26.3145344588424));
#25901=CARTESIAN_POINT('Ctrl Pts',(-23.2051565126403,-48.842305447693,-26.1565859356499));
#25902=CARTESIAN_POINT('Ctrl Pts',(-22.7214723212287,-52.0510183088916,
-25.9986374124575));
#25903=CARTESIAN_POINT('Ctrl Pts',(-19.7704552622143,-53.3999535603981,
-25.840688889265));
#25904=CARTESIAN_POINT('Ctrl Pts',(-17.0272740757602,-51.6666160922435,
-25.6827403660725));
#25905=CARTESIAN_POINT('Ctrl Pts',(-16.9799412829216,-48.4214880696582,
-25.5247918428801));
#25906=CARTESIAN_POINT('Ctrl Pts',(-19.66967215945,-46.6089846779987,-25.3668433196876));
#25907=CARTESIAN_POINT('Ctrl Pts',(-22.661159063289,-47.8681345752109,-25.2088947964951));
#25908=CARTESIAN_POINT('Ctrl Pts',(-23.2352996440075,-51.0661285281439,
-25.0509462733027));
#25909=CARTESIAN_POINT('Ctrl Pts',(-21.6689420470237,-52.5434180484685,
-24.945647257841));
#25910=CARTESIAN_POINT('Ctrl Pts',(-20.7459328543469,-52.7901775698422,
-24.8929977501102));
#25911=CARTESIAN_POINT('Ctrl Pts',(-22.3360626576961,-48.0026984430693,
-40.3210067496694));
#25912=CARTESIAN_POINT('Ctrl Pts',(-22.996783221692,-48.7754834195626,-40.2683572419386));
#25913=CARTESIAN_POINT('Ctrl Pts',(-23.4799591781266,-51.0152280856744,
-40.1630582264769));
#25914=CARTESIAN_POINT('Ctrl Pts',(-21.0487280422805,-53.4737329440196,
-40.0051097032845));
#25915=CARTESIAN_POINT('Ctrl Pts',(-17.6662375026362,-52.7747494832621,
-39.847161180092));
#25916=CARTESIAN_POINT('Ctrl Pts',(-16.3999441853237,-49.5638692818644,
-39.6892126568996));
#25917=CARTESIAN_POINT('Ctrl Pts',(-18.3975850141438,-46.7464741122942,
-39.5312641337071));
#25918=CARTESIAN_POINT('Ctrl Pts',(-21.8481508174258,-46.8799262317611,
-39.3733156105146));
#25919=CARTESIAN_POINT('Ctrl Pts',(-23.623022297825,-49.8417650665615,-39.2153670873222));
#25920=CARTESIAN_POINT('Ctrl Pts',(-22.1130258164637,-52.9473164300811,
-39.0574185641297));
#25921=CARTESIAN_POINT('Ctrl Pts',(-18.6872049726298,-53.380502213004,-38.8994700409372));
#25922=CARTESIAN_POINT('Ctrl Pts',(-16.4516595311324,-50.7487514343516,
-38.7415215177447));
#25923=CARTESIAN_POINT('Ctrl Pts',(-17.4332844268133,-47.4380993731673,
-38.5835729945523));
#25924=CARTESIAN_POINT('Ctrl Pts',(-20.7420732981751,-46.4502603278007,
-38.4256244713598));
#25925=CARTESIAN_POINT('Ctrl Pts',(-23.3780463626243,-48.6808544307687,
-38.2676759481674));
#25926=CARTESIAN_POINT('Ctrl Pts',(-22.95124778817,-52.107481644896,-38.1097274249748));
#25927=CARTESIAN_POINT('Ctrl Pts',(-19.8486424720205,-53.6233173671768,
-37.9517789017825));
#25928=CARTESIAN_POINT('Ctrl Pts',(-16.8832684886027,-51.8540024255665,
-37.7938303785899));
#25929=CARTESIAN_POINT('Ctrl Pts',(-16.7437401425967,-48.4037193720523,
-37.6358818553975));
#25930=CARTESIAN_POINT('Ctrl Pts',(-19.5565635911389,-46.4007356661223,
-37.477933332205));
#25931=CARTESIAN_POINT('Ctrl Pts',(-22.7714373367961,-47.6610953390299,
-37.3199848090126));
#25932=CARTESIAN_POINT('Ctrl Pts',(-23.4735331428005,-51.0420687967573,
-37.1620362858201));
#25933=CARTESIAN_POINT('Ctrl Pts',(-21.0262820888715,-53.4782301377694,
-37.0040877626276));
#25934=CARTESIAN_POINT('Ctrl Pts',(-17.6485322789718,-52.7607860144173,
-36.8461392394351));
#25935=CARTESIAN_POINT('Ctrl Pts',(-16.402786734543,-49.5402211692867,-36.6881907162427));
#25936=CARTESIAN_POINT('Ctrl Pts',(-18.4185250538729,-46.7365238104494,
-36.5302421930502));
#25937=CARTESIAN_POINT('Ctrl Pts',(-21.868138608337,-46.8917210565137,-36.3722936698577));
#25938=CARTESIAN_POINT('Ctrl Pts',(-23.6239677035562,-49.865100287622,-36.2143451466653));
#25939=CARTESIAN_POINT('Ctrl Pts',(-22.0940554999228,-52.9607889846439,
-36.0563966234728));
#25940=CARTESIAN_POINT('Ctrl Pts',(-18.6655268623454,-53.3720203578719,
-35.8984481002803));
#25941=CARTESIAN_POINT('Ctrl Pts',(-16.4469244325051,-50.725943427852,-35.7404995770878));
#25942=CARTESIAN_POINT('Ctrl Pts',(-17.4497875578081,-47.4216756704347,
-35.5825510538954));
#25943=CARTESIAN_POINT('Ctrl Pts',(-20.764850743239,-46.4550961664119,-35.4246025307029));
#25944=CARTESIAN_POINT('Ctrl Pts',(-23.38644702166,-48.7025731549433,-35.2666540075105));
#25945=CARTESIAN_POINT('Ctrl Pts',(-22.9376547796718,-52.1263876044256,
-35.108705484318));
#25946=CARTESIAN_POINT('Ctrl Pts',(-19.8253802936868,-53.6222710841349,
-34.9507569611255));
#25947=CARTESIAN_POINT('Ctrl Pts',(-16.8714281845976,-51.8339515382522,
-34.792808437933));
#25948=CARTESIAN_POINT('Ctrl Pts',(-16.7540569893232,-48.3828439097519,
-34.6348599147406));
#25949=CARTESIAN_POINT('Ctrl Pts',(-19.5796836009353,-46.3979625246999,
-34.4769113915481));
#25950=CARTESIAN_POINT('Ctrl Pts',(-22.7863983082339,-47.678938967485,-34.3189628683557));
#25951=CARTESIAN_POINT('Ctrl Pts',(-23.4667704139307,-51.0643508565711,
-34.1610143451631));
#25952=CARTESIAN_POINT('Ctrl Pts',(-21.0039272223724,-53.4847481947722,
-34.0030658219707));
#25953=CARTESIAN_POINT('Ctrl Pts',(-17.6308537513554,-52.7456303285988,
-33.8451172987782));
#25954=CARTESIAN_POINT('Ctrl Pts',(-16.4058131296584,-49.5171329480567,
-33.6871687755858));
#25955=CARTESIAN_POINT('Ctrl Pts',(-18.4395124310478,-46.7264364377739,
-33.5292202523933));
#25956=CARTESIAN_POINT('Ctrl Pts',(-21.8880583511222,-46.9037804484265,
-33.3712717292008));
#25957=CARTESIAN_POINT('Ctrl Pts',(-23.6247591869331,-49.8883725592297,
-33.2133232060084));
#25958=CARTESIAN_POINT('Ctrl Pts',(-22.0750011100191,-52.9741738755843,
-33.0553746828159));
#25959=CARTESIAN_POINT('Ctrl Pts',(-18.6439026349568,-53.3633821943561,
-32.8974261596234));
#25960=CARTESIAN_POINT('Ctrl Pts',(-16.4423363969422,-50.7031141701506,
-32.739477636431));
#25961=CARTESIAN_POINT('Ctrl Pts',(-17.4663955463727,-47.4053539121205,
-32.5815291132385));
#25962=CARTESIAN_POINT('Ctrl Pts',(-20.7875967978108,-46.460080349377,-32.423580590046));
#25963=CARTESIAN_POINT('Ctrl Pts',(-23.3947079863477,-48.724344272064,-32.2656320668535));
#25964=CARTESIAN_POINT('Ctrl Pts',(-22.9239406890394,-52.1452064459554,
-32.1076835436611));
#25965=CARTESIAN_POINT('Ctrl Pts',(-19.8021252966153,-53.6210751788038,
-31.9497350204686));
#25966=CARTESIAN_POINT('Ctrl Pts',(-16.859716879663,-51.8138251770541,-31.7917864972762));
#25967=CARTESIAN_POINT('Ctrl Pts',(-16.7645076605265,-48.3620350522686,
-31.6338379740837));
#25968=CARTESIAN_POINT('Ctrl Pts',(-19.6028209425392,-46.3953379291391,
-31.4758894508912));
#25969=CARTESIAN_POINT('Ctrl Pts',(-22.8012443962967,-47.696878274818,-31.3179409276987));
#25970=CARTESIAN_POINT('Ctrl Pts',(-23.459864751929,-51.0865890424386,-31.1599924045063));
#25971=CARTESIAN_POINT('Ctrl Pts',(-20.9815309640172,-53.4911225723918,
-31.0020438813138));
#25972=CARTESIAN_POINT('Ctrl Pts',(-17.6132729029457,-52.730361443651,-30.8440953581213));
#25973=CARTESIAN_POINT('Ctrl Pts',(-16.4089877117502,-49.4940646341411,
-30.6861468349289));
#25974=CARTESIAN_POINT('Ctrl Pts',(-18.4605641466087,-46.7164840335274,
-30.5281983117364));
#25975=CARTESIAN_POINT('Ctrl Pts',(-21.9079002499127,-46.9159674960896,
-30.370249788544));
#25976=CARTESIAN_POINT('Ctrl Pts',(-23.6254012227827,-49.9116494333404,
-30.2123012653514));
#25977=CARTESIAN_POINT('Ctrl Pts',(-22.0558611685522,-52.9874361423172,
-30.054352742159));
#25978=CARTESIAN_POINT('Ctrl Pts',(-18.6223343189813,-53.3546053598246,
-29.8964042189665));
#25979=CARTESIAN_POINT('Ctrl Pts',(-16.4378950425926,-50.6802559232762,
-29.7384556957741));
#25980=CARTESIAN_POINT('Ctrl Pts',(-17.48310799454,-47.3891391301676,-29.5805071725815));
#25981=CARTESIAN_POINT('Ctrl Pts',(-20.810310380068,-46.4652104819412,-29.4225586493892));
#25982=CARTESIAN_POINT('Ctrl Pts',(-23.4028289883847,-48.7461679840765,
-29.2646101261966));
#25983=CARTESIAN_POINT('Ctrl Pts',(-22.9101060454574,-52.163936841271,-29.1066616030042));
#25984=CARTESIAN_POINT('Ctrl Pts',(-19.7788784576719,-53.6197299780505,
-28.9487130798117));
#25985=CARTESIAN_POINT('Ctrl Pts',(-16.8481350478379,-51.7936240320434,
-28.7907645566193));
#25986=CARTESIAN_POINT('Ctrl Pts',(-16.7750917292348,-48.3412937283827,
-28.6328160334268));
#25987=CARTESIAN_POINT('Ctrl Pts',(-19.6259746610823,-46.3928619507583,
-28.4748675102343));
#25988=CARTESIAN_POINT('Ctrl Pts',(-22.8159749872838,-47.7149125425452,
-28.3169189870419));
#25989=CARTESIAN_POINT('Ctrl Pts',(-23.4528164464309,-51.1087824216521,
-28.1589704638493));
#25990=CARTESIAN_POINT('Ctrl Pts',(-20.9590942265365,-53.4973530261498,
-28.0010219406569));
#25991=CARTESIAN_POINT('Ctrl Pts',(-17.595790480254,-52.7149799592246,-27.8430734174644));
#25992=CARTESIAN_POINT('Ctrl Pts',(-16.4123103065868,-49.4710172348044,
-27.685124894272));
#25993=CARTESIAN_POINT('Ctrl Pts',(-18.4816794190144,-46.7066668978831,
-27.5271763710795));
#25994=CARTESIAN_POINT('Ctrl Pts',(-21.9276633145204,-46.9282819155376,
-27.369227847887));
#25995=CARTESIAN_POINT('Ctrl Pts',(-23.6258941273587,-49.9349295156179,
-27.2112793246946));
#25996=CARTESIAN_POINT('Ctrl Pts',(-22.0366357822403,-53.0005761032442,
-27.0533308015021));
#25997=CARTESIAN_POINT('Ctrl Pts',(-18.6008241624394,-53.3456884935447,
-26.8953822783096));
#25998=CARTESIAN_POINT('Ctrl Pts',(-16.4335978471204,-50.657373059488,-26.7374337551171));
#25999=CARTESIAN_POINT('Ctrl Pts',(-17.4999296001022,-47.3730251639953,
-26.5794852319247));
#26000=CARTESIAN_POINT('Ctrl Pts',(-20.8329798277681,-46.4704999500574,
-26.4215367087322));
#26001=CARTESIAN_POINT('Ctrl Pts',(-23.4108310490853,-48.7680163172086,
-26.2635881855398));
#26002=CARTESIAN_POINT('Ctrl Pts',(-22.8961088969807,-52.1826319253429,
-26.1056396623473));
#26003=CARTESIAN_POINT('Ctrl Pts',(-19.7557254019559,-53.6181282017024,
-25.9476911391548));
#26004=CARTESIAN_POINT('Ctrl Pts',(-16.8365145842861,-51.7735626612651,
-25.7897426159623));
#26005=CARTESIAN_POINT('Ctrl Pts',(-16.7861444514027,-48.3201951348933,
-25.6317940927699));
#26006=CARTESIAN_POINT('Ctrl Pts',(-19.6484750587118,-46.3913836024568,
-25.4738455695774));
#26007=CARTESIAN_POINT('Ctrl Pts',(-22.8319253439964,-47.7313330083366,
-25.3158970463849));
#26008=CARTESIAN_POINT('Ctrl Pts',(-23.4429084618352,-51.1345418770559,
-25.1579485231925));
#26009=CARTESIAN_POINT('Ctrl Pts',(-21.7760378723045,-52.706628901368,-25.0526495077308));
#26010=CARTESIAN_POINT('Ctrl Pts',(-20.7937992825329,-52.9692229537457,
-25.));
#26011=CARTESIAN_POINT('Ctrl Pts',(-17.4818816223345,-50.0021988885187,
-38.387416697508));
#26012=CARTESIAN_POINT('Ctrl Pts',(-17.4802992936945,-50.1765619490587,
-38.3984493876971));
#26013=CARTESIAN_POINT('Ctrl Pts',(-17.4968845768144,-50.3506259225462,
-38.4094820778862));
#26014=CARTESIAN_POINT('Ctrl Pts',(-17.5327554656256,-50.5206201636086,
-38.4205147680753));
#26015=CARTESIAN_POINT('Ctrl Pts',(-17.7039362570194,-51.3318559506749,
-38.4731642758061));
#26016=CARTESIAN_POINT('Ctrl Pts',(-18.3143137472823,-52.0504105393911,
-38.525813783537));
#26017=CARTESIAN_POINT('Ctrl Pts',(-19.0871834193891,-52.350550845055,-38.5784632912678));
#26018=CARTESIAN_POINT('Ctrl Pts',(-19.8600530914959,-52.650691150719,-38.6311127989986));
#26019=CARTESIAN_POINT('Ctrl Pts',(-20.7954149454465,-52.5324171733308,
-38.6837623067294));
#26020=CARTESIAN_POINT('Ctrl Pts',(-21.4692352434878,-52.049321312685,-38.7364118144602));
#26021=CARTESIAN_POINT('Ctrl Pts',(-22.1430555415291,-51.5662254520392,
-38.7890613221911));
#26022=CARTESIAN_POINT('Ctrl Pts',(-22.555334283661,-50.7183077081358,-38.8417108299219));
#26023=CARTESIAN_POINT('Ctrl Pts',(-22.519174487008,-49.890009089608,-38.8943603376527));
#26024=CARTESIAN_POINT('Ctrl Pts',(-22.483014690355,-49.0617104710802,-38.9470098453835));
#26025=CARTESIAN_POINT('Ctrl Pts',(-21.9984163549171,-48.2530309779281,
-38.9996593531144));
#26026=CARTESIAN_POINT('Ctrl Pts',(-21.2850581660083,-47.8304728207041,
-39.0523088608452));
#26027=CARTESIAN_POINT('Ctrl Pts',(-20.5716999770995,-47.4079146634801,
-39.104958368576));
#26028=CARTESIAN_POINT('Ctrl Pts',(-19.6295819347198,-47.3714778421842,
-39.1576078763068));
#26029=CARTESIAN_POINT('Ctrl Pts',(-18.8858120634375,-47.7378802405701,
-39.2102573840377));
#26030=CARTESIAN_POINT('Ctrl Pts',(-18.1420421921552,-48.1042826389561,
-39.2629068917685));
#26031=CARTESIAN_POINT('Ctrl Pts',(-17.5966204919703,-48.8735242570238,
-39.3155563994993));
#26032=CARTESIAN_POINT('Ctrl Pts',(-17.4967795202106,-49.6964830578704,
-39.3682059072301));
#26033=CARTESIAN_POINT('Ctrl Pts',(-17.4846361716636,-49.7965769910764,
-39.3746095039894));
#26034=CARTESIAN_POINT('Ctrl Pts',(-17.4790843453548,-49.8974655681758,
-39.3810131007487));
#26035=CARTESIAN_POINT('Ctrl Pts',(-17.4798421274757,-49.9984351524252,
-39.387416697508));
#26036=CARTESIAN_POINT('Ctrl Pts',(-19.2062007174672,-52.9692229537457,
-40.));
#26037=CARTESIAN_POINT('Ctrl Pts',(-18.2239621276955,-52.7066289013681,
-39.9473504922692));
#26038=CARTESIAN_POINT('Ctrl Pts',(-16.5570904206518,-51.1345489516877,
-39.8420514768075));
#26039=CARTESIAN_POINT('Ctrl Pts',(-17.1680756287354,-47.7313299839058,
-39.6841029536151));
#26040=CARTESIAN_POINT('Ctrl Pts',(-20.3515248249563,-46.3913860864081,
-39.5261544304226));
#26041=CARTESIAN_POINT('Ctrl Pts',(-23.2138549612499,-48.3201943023511,
-39.3682059072301));
#26042=CARTESIAN_POINT('Ctrl Pts',(-23.1634850140729,-51.7735630043146,
-39.2102573840376));
#26043=CARTESIAN_POINT('Ctrl Pts',(-20.2442744821096,-53.6181272821323,
-39.0523088608452));
#26044=CARTESIAN_POINT('Ctrl Pts',(-17.1038916129568,-52.1826317747292,
-38.8943603376527));
#26045=CARTESIAN_POINT('Ctrl Pts',(-16.5891694547899,-48.7680164050864,
-38.7364118144603));
#26046=CARTESIAN_POINT('Ctrl Pts',(-19.1670203242729,-46.4705005646606,
-38.5784632912678));
#26047=CARTESIAN_POINT('Ctrl Pts',(-22.5000699934528,-47.373025546768,-38.4205147680754));
#26048=CARTESIAN_POINT('Ctrl Pts',(-23.5664015975527,-50.657372972797,-38.2625662448828));
#26049=CARTESIAN_POINT('Ctrl Pts',(-21.3991756129266,-53.3456879568638,
-38.1046177216904));
#26050=CARTESIAN_POINT('Ctrl Pts',(-17.9633645411529,-53.0005756349581,
-37.9466691984979));
#26051=CARTESIAN_POINT('Ctrl Pts',(-16.3741064431585,-49.9349295232864,
-37.7887206753054));
#26052=CARTESIAN_POINT('Ctrl Pts',(-18.0723369901302,-46.9282824012858,
-37.630772152113));
#26053=CARTESIAN_POINT('Ctrl Pts',(-21.5183203411933,-46.7066674164727,
-37.4728236289205));
#26054=CARTESIAN_POINT('Ctrl Pts',(-23.5876891278802,-49.4710173186029,
-37.3148751057281));
#26055=CARTESIAN_POINT('Ctrl Pts',(-22.4042091405233,-52.7149795309031,
-37.1569265825355));
#26056=CARTESIAN_POINT('Ctrl Pts',(-19.0409059247592,-53.4973524747668,
-36.9989780593431));
#26057=CARTESIAN_POINT('Ctrl Pts',(-16.5471840980045,-51.1087822467551,
-36.8410295361506));
#26058=CARTESIAN_POINT('Ctrl Pts',(-17.1840254567772,-47.7149129029046,
-36.6830810129582));
#26059=CARTESIAN_POINT('Ctrl Pts',(-20.3740252799296,-46.3928625195443,
-36.5251324897657));
#26060=CARTESIAN_POINT('Ctrl Pts',(-23.2249077622416,-48.3412939899481,
-36.3671839665732));
#26061=CARTESIAN_POINT('Ctrl Pts',(-23.1518644551494,-51.7936237492067,
-36.2092354433807));
#26062=CARTESIAN_POINT('Ctrl Pts',(-20.2211215074614,-53.6197294072659,
-36.0512869201883));
#26063=CARTESIAN_POINT('Ctrl Pts',(-17.0898944134298,-52.1639365000438,
-35.8933383969958));
#26064=CARTESIAN_POINT('Ctrl Pts',(-16.5971715481998,-48.746168181791,-35.7353898738033));
#26065=CARTESIAN_POINT('Ctrl Pts',(-19.1896897477077,-46.4652110393336,
-35.5774413506109));
#26066=CARTESIAN_POINT('Ctrl Pts',(-22.5168916085772,-47.3891395418682,
-35.4194928274184));
#26067=CARTESIAN_POINT('Ctrl Pts',(-23.5621043957074,-50.6802558160081,
-35.261544304226));
#26068=CARTESIAN_POINT('Ctrl Pts',(-21.3776654637779,-53.3546048308447,
-35.1035957810335));
#26069=CARTESIAN_POINT('Ctrl Pts',(-17.9441391556319,-52.9874356712354,
-34.945647257841));
#26070=CARTESIAN_POINT('Ctrl Pts',(-16.3745993488984,-49.9116494472723,
-34.7876987346485));
#26071=CARTESIAN_POINT('Ctrl Pts',(-18.0921000509396,-46.9159679824036,
-34.6297502114561));
#26072=CARTESIAN_POINT('Ctrl Pts',(-21.5394356106412,-46.7164845512972,
-34.4718016882636));
#26073=CARTESIAN_POINT('Ctrl Pts',(-23.5910117219915,-49.4940647139208,
-34.3138531650712));
#26074=CARTESIAN_POINT('Ctrl Pts',(-22.386726720697,-52.7303610131065,-34.1559046418786));
#26075=CARTESIAN_POINT('Ctrl Pts',(-19.0184691907583,-53.491122021885,-33.9979561186862));
#26076=CARTESIAN_POINT('Ctrl Pts',(-16.540135793649,-51.086588871097,-33.8400075954937));
#26077=CARTESIAN_POINT('Ctrl Pts',(-17.1987560454249,-47.696878637992,-33.6820590723013));
#26078=CARTESIAN_POINT('Ctrl Pts',(-20.3971789948304,-46.3953384975499,
-33.5241105491088));
#26079=CARTESIAN_POINT('Ctrl Pts',(-23.2354918292762,-48.3620353105553,
-33.3661620259163));
#26080=CARTESIAN_POINT('Ctrl Pts',(-23.1402826251531,-51.8138248910362,
-33.2082135027239));
#26081=CARTESIAN_POINT('Ctrl Pts',(-20.1978746721824,-53.6210746078049,
-33.0502649795314));
#26082=CARTESIAN_POINT('Ctrl Pts',(-17.0760597720301,-52.1452061076829,
-32.8923164563389));
#26083=CARTESIAN_POINT('Ctrl Pts',(-16.6052925489559,-48.7243444732193,
-32.7343679331465));
#26084=CARTESIAN_POINT('Ctrl Pts',(-19.2124033263834,-46.4600809075787,
-32.576419409954));
#26085=CARTESIAN_POINT('Ctrl Pts',(-22.533604054109,-47.405354321264,-32.4184708867615));
#26086=CARTESIAN_POINT('Ctrl Pts',(-23.5576630420582,-50.7031140592781,
-32.2605223635691));
#26087=CARTESIAN_POINT('Ctrl Pts',(-21.3560971512034,-53.3633816639922,
-32.1025738403766));
#26088=CARTESIAN_POINT('Ctrl Pts',(-17.9249992171831,-52.9741734065938,
-31.9446253171841));
#26089=CARTESIAN_POINT('Ctrl Pts',(-16.3752413846467,-49.8883725768321,
-31.7866767939917));
#26090=CARTESIAN_POINT('Ctrl Pts',(-18.1119419466013,-46.9037809366621,
-31.6287282707992));
#26091=CARTESIAN_POINT('Ctrl Pts',(-21.5604873228824,-46.7264369539744,
-31.4707797476067));
#26092=CARTESIAN_POINT('Ctrl Pts',(-23.5941863035827,-49.5171330241987,
-31.3128312244142));
#26093=CARTESIAN_POINT('Ctrl Pts',(-22.3691458750596,-52.7456298956467,
-31.1548827012218));
#26094=CARTESIAN_POINT('Ctrl Pts',(-18.9960729359346,-53.4847476452704,
-30.9969341780293));
#26095=CARTESIAN_POINT('Ctrl Pts',(-16.5332301327363,-51.0643506887362,
-30.8389856548368));
#26096=CARTESIAN_POINT('Ctrl Pts',(-17.2136021311466,-47.6789393334878,
-30.6810371316444));
#26097=CARTESIAN_POINT('Ctrl Pts',(-20.4203163327858,-46.3979630926968,
-30.5230886084519));
#26098=CARTESIAN_POINT('Ctrl Pts',(-23.2459424988316,-48.3828441647573,
-30.3651400852595));
#26099=CARTESIAN_POINT('Ctrl Pts',(-23.1285713220653,-51.8339512490605,
-30.207191562067));
#26100=CARTESIAN_POINT('Ctrl Pts',(-20.1746196787779,-53.6222705129474,
-30.0492430388745));
#26101=CARTESIAN_POINT('Ctrl Pts',(-17.0623456835602,-52.1263872691206,
-29.891294515682));
#26102=CARTESIAN_POINT('Ctrl Pts',(-16.6135535123409,-48.7025733595317,
-29.7333459924896));
#26103=CARTESIAN_POINT('Ctrl Pts',(-19.2351493773684,-46.4550967253995,
-29.5753974692971));
#26104=CARTESIAN_POINT('Ctrl Pts',(-22.5502120400548,-47.4216760770047,
-29.4174489461046));
#26105=CARTESIAN_POINT('Ctrl Pts',(-23.5530750072187,-50.7259433133794,
-29.2595004229121));
#26106=CARTESIAN_POINT('Ctrl Pts',(-21.3344729272248,-53.3720198261462,
-29.1015518997197));
#26107=CARTESIAN_POINT('Ctrl Pts',(-17.905944830284,-52.9607885177635,-28.9436033765272));
#26108=CARTESIAN_POINT('Ctrl Pts',(-16.3760328678989,-49.8651003088954,
-28.7856548533348));
#26109=CARTESIAN_POINT('Ctrl Pts',(-18.1318616862451,-46.8917215466485,
-28.6277063301423));
#26110=CARTESIAN_POINT('Ctrl Pts',(-21.5814746967481,-46.7365243250642,
-28.4697578069498));
#26111=CARTESIAN_POINT('Ctrl Pts',(-23.5972126982202,-49.5402212417787,
-28.3118092837573));
#26112=CARTESIAN_POINT('Ctrl Pts',(-22.3514673502323,-52.7607855790929,
-28.1538607605649));
#26113=CARTESIAN_POINT('Ctrl Pts',(-18.9737180729577,-53.4782295892619,
-27.9959122373724));
#26114=CARTESIAN_POINT('Ctrl Pts',(-16.5264674049389,-51.0420686324998,
-27.83796371418));
#26115=CARTESIAN_POINT('Ctrl Pts',(-17.2285631002129,-47.6610957077258,
-27.6800151909875));
#26116=CARTESIAN_POINT('Ctrl Pts',(-20.4434363389617,-46.4007362339102,
-27.522066667795));
#26117=CARTESIAN_POINT('Ctrl Pts',(-23.2562593438794,-48.403719623335,-27.3641181446025));
#26118=CARTESIAN_POINT('Ctrl Pts',(-23.1167310200335,-51.8540021340239,
-27.2061696214101));
#26119=CARTESIAN_POINT('Ctrl Pts',(-20.1513575038949,-53.623316794304,-27.0482210982176));
#26120=CARTESIAN_POINT('Ctrl Pts',(-17.0487526776507,-52.1074813154118,
-26.8902725750251));
#26121=CARTESIAN_POINT('Ctrl Pts',(-16.6219541691413,-48.6808546335012,
-26.7323240518326));
#26122=CARTESIAN_POINT('Ctrl Pts',(-19.2579268207016,-46.4502608973225,
-26.5743755286402));
#26123=CARTESIAN_POINT('Ctrl Pts',(-22.5667151646459,-47.4380997591695,
-26.4164270054477));
#26124=CARTESIAN_POINT('Ctrl Pts',(-23.5483399170972,-50.748751349135,-26.2584784822553));
#26125=CARTESIAN_POINT('Ctrl Pts',(-21.312794804531,-53.3805016203859,-26.1005299590628));
#26126=CARTESIAN_POINT('Ctrl Pts',(-17.8869745490034,-52.9473160722452,
-25.9425814358703));
#26127=CARTESIAN_POINT('Ctrl Pts',(-16.3769782077294,-49.8417649018331,
-25.7846329126779));
#26128=CARTESIAN_POINT('Ctrl Pts',(-18.1518496079148,-46.8799270552508,
-25.6266843894854));
#26129=CARTESIAN_POINT('Ctrl Pts',(-21.6024144605454,-46.7464740570925,
-25.468735866293));
#26130=CARTESIAN_POINT('Ctrl Pts',(-23.6000558022285,-49.5638703006617,
-25.3107873431004));
#26131=CARTESIAN_POINT('Ctrl Pts',(-22.3337609944815,-52.7747475021281,
-25.152838819908));
#26132=CARTESIAN_POINT('Ctrl Pts',(-18.9512744725129,-53.4737348854633,
-24.9948902967155));
#26133=CARTESIAN_POINT('Ctrl Pts',(-16.5200358935638,-51.0152228884625,
-24.836941773523));
#26134=CARTESIAN_POINT('Ctrl Pts',(-17.003216778308,-48.7754834195627,-24.7316427580614));
#26135=CARTESIAN_POINT('Ctrl Pts',(-17.6639373423038,-48.0026984430694,
-24.6789932503306));
#26136=CARTESIAN_POINT('Ctrl Pts',(-19.2540671456531,-52.7901775698422,
-40.1070022498898));
#26137=CARTESIAN_POINT('Ctrl Pts',(-18.3310579529763,-52.5434180484685,
-40.054352742159));
#26138=CARTESIAN_POINT('Ctrl Pts',(-16.764699305866,-51.0661351761724,-39.9490537266973));
#26139=CARTESIAN_POINT('Ctrl Pts',(-17.3388418507866,-47.8681317331546,
-39.7911052035049));
#26140=CARTESIAN_POINT('Ctrl Pts',(-20.330327731233,-46.6089870121667,-39.6331566803124));
#26141=CARTESIAN_POINT('Ctrl Pts',(-23.0200581651483,-48.4214872873186,
-39.4752081571199));
#26142=CARTESIAN_POINT('Ctrl Pts',(-22.9727255468179,-51.666616414607,-39.3172596339275));
#26143=CARTESIAN_POINT('Ctrl Pts',(-20.2295446288421,-53.3999526962785,
-39.159311110735));
#26144=CARTESIAN_POINT('Ctrl Pts',(-17.2785281579593,-52.0510181673598,
-39.0013625875425));
#26145=CARTESIAN_POINT('Ctrl Pts',(-16.7948439608511,-48.8423055302719,
-38.8434140643501));
#26146=CARTESIAN_POINT('Ctrl Pts',(-19.2172493465281,-46.6833308543465,
-38.6854655411576));
#26147=CARTESIAN_POINT('Ctrl Pts',(-22.3493147289487,-47.5314332031855,
-38.5275170179651));
#26148=CARTESIAN_POINT('Ctrl Pts',(-23.3513460920769,-50.6177331080526,
-38.3695684947727));
#26149=CARTESIAN_POINT('Ctrl Pts',(-21.3148047392443,-53.14394157608,-38.2116199715802));
#26150=CARTESIAN_POINT('Ctrl Pts',(-18.0861745097142,-52.8196396712863,
-38.0536714483877));
#26151=CARTESIAN_POINT('Ctrl Pts',(-16.5927493386201,-49.9388533002023,
-37.8957229251952));
#26152=CARTESIAN_POINT('Ctrl Pts',(-18.1885758745169,-47.1135082550774,
-37.7377744020028));
#26153=CARTESIAN_POINT('Ctrl Pts',(-21.426764990648,-46.9052567463833,-37.5798258788103));
#26154=CARTESIAN_POINT('Ctrl Pts',(-23.3713499754371,-49.5029151951668,
-37.4218773556179));
#26155=CARTESIAN_POINT('Ctrl Pts',(-22.2592343254774,-52.5512651315557,
-37.2639288324253));
#26156=CARTESIAN_POINT('Ctrl Pts',(-19.0987396979639,-53.2864606602264,
-37.1059803092329));
#26157=CARTESIAN_POINT('Ctrl Pts',(-16.7553903386107,-51.0419222143061,
-36.9480317860404));
#26158=CARTESIAN_POINT('Ctrl Pts',(-17.3538298975377,-47.8527046089926,
-36.790083262848));
#26159=CARTESIAN_POINT('Ctrl Pts',(-20.3514713993765,-46.6103744157683,
-36.6321347396555));
#26160=CARTESIAN_POINT('Ctrl Pts',(-23.0304444776251,-48.4413146549433,
-36.474186216463));
#26161=CARTESIAN_POINT('Ctrl Pts',(-22.9618057124497,-51.6854674882058,
-36.3162376932706));
#26162=CARTESIAN_POINT('Ctrl Pts',(-20.2077877882326,-53.4014582125975,
-36.1582891700781));
#26163=CARTESIAN_POINT('Ctrl Pts',(-17.2653749954083,-52.0334502255441,
-36.0003406468856));
#26164=CARTESIAN_POINT('Ctrl Pts',(-16.8023635246871,-48.8217747639638,
-35.8423921236932));
#26165=CARTESIAN_POINT('Ctrl Pts',(-19.2385517942642,-46.6783602896053,
-35.6844436005007));
#26166=CARTESIAN_POINT('Ctrl Pts',(-22.3651219936574,-47.5465755176528,
-35.5264950773082));
#26167=CARTESIAN_POINT('Ctrl Pts',(-23.3473080132972,-50.6392361062634,
-35.3685465541158));
#26168=CARTESIAN_POINT('Ctrl Pts',(-21.2945916610709,-53.1523207588367,
-35.2105980309233));
#26169=CARTESIAN_POINT('Ctrl Pts',(-18.0681084229676,-52.8072920528626,
-35.0526495077308));
#26170=CARTESIAN_POINT('Ctrl Pts',(-16.5932125219381,-49.9169770224924,
-34.8947009845383));
#26171=CARTESIAN_POINT('Ctrl Pts',(-18.2071472145074,-47.1019364007955,
-34.7367524613459));
#26172=CARTESIAN_POINT('Ctrl Pts',(-21.4466070005315,-46.9144819038789,
-34.5788039381534));
#26173=CARTESIAN_POINT('Ctrl Pts',(-23.3744722157361,-49.5245728229235,
-34.420855414961));
#26174=CARTESIAN_POINT('Ctrl Pts',(-22.2428061028663,-52.5657191039599,
-34.2629068917685));
#26175=CARTESIAN_POINT('Ctrl Pts',(-19.0776559083916,-53.2806059062547,
-34.104958368576));
#26176=CARTESIAN_POINT('Ctrl Pts',(-16.7487670499508,-51.021067108467,-33.9470098453835));
#26177=CARTESIAN_POINT('Ctrl Pts',(-17.3676722255392,-47.8357578177845,
-33.7890613221911));
#26178=CARTESIAN_POINT('Ctrl Pts',(-20.3732289356009,-46.6127010912662,
-33.6311127989986));
#26179=CARTESIAN_POINT('Ctrl Pts',(-23.0403903209982,-48.4608052652575,
-33.4731642758061));
#26180=CARTESIAN_POINT('Ctrl Pts',(-22.9509222716381,-51.704450492748,-33.3152157526137));
#26181=CARTESIAN_POINT('Ctrl Pts',(-20.1859427468276,-53.4027222969824,
-33.1572672294212));
#26182=CARTESIAN_POINT('Ctrl Pts',(-17.2523745886616,-52.0158492836633,
-32.9993187062287));
#26183=CARTESIAN_POINT('Ctrl Pts',(-16.8099948257066,-48.8012670341315,
-32.8413701830363));
#26184=CARTESIAN_POINT('Ctrl Pts',(-19.2598957346618,-46.6735395069373,
-32.6834216598438));
#26185=CARTESIAN_POINT('Ctrl Pts',(-22.3808266717453,-47.5618125390806,
-32.5254731366513));
#26186=CARTESIAN_POINT('Ctrl Pts',(-23.3431344751275,-50.6607159879198,
-32.3675246134589));
#26187=CARTESIAN_POINT('Ctrl Pts',(-21.2743239267504,-53.1605683452807,
-32.2095760902664));
#26188=CARTESIAN_POINT('Ctrl Pts',(-18.0501226307991,-52.7948295083164,
-32.0516275670739));
#26189=CARTESIAN_POINT('Ctrl Pts',(-16.5938158426627,-49.895103757059,-31.8936790438815));
#26190=CARTESIAN_POINT('Ctrl Pts',(-18.2257926355758,-47.0904842390009,
-31.7357305206889));
#26191=CARTESIAN_POINT('Ctrl Pts',(-21.4663892857345,-46.9238341725191,
-31.5777819974966));
#26192=CARTESIAN_POINT('Ctrl Pts',(-23.3774553687318,-49.5462501044595,
-31.419833474304));
#26193=CARTESIAN_POINT('Ctrl Pts',(-22.2262853895617,-52.5800672665074,
-31.2618849511117));
#26194=CARTESIAN_POINT('Ctrl Pts',(-19.0566101570854,-53.2746159072117,
-31.1039364279191));
#26195=CARTESIAN_POINT('Ctrl Pts',(-16.7422778032747,-51.000169897788,-30.9459879047267));
#26196=CARTESIAN_POINT('Ctrl Pts',(-17.3816230860929,-47.8189002608325,
-30.7880393815342));
#26197=CARTESIAN_POINT('Ctrl Pts',(-20.3949710824167,-46.6151674222299,
-30.6300908583417));
#26198=CARTESIAN_POINT('Ctrl Pts',(-23.0502108108157,-48.4803593368625,
-30.4721423351493));
#26199=CARTESIAN_POINT('Ctrl Pts',(-22.9399171650165,-51.7233632229797,
-30.3141938119568));
#26200=CARTESIAN_POINT('Ctrl Pts',(-20.1640900392355,-53.4038460885454,
-30.1562452887643));
#26201=CARTESIAN_POINT('Ctrl Pts',(-17.2394874654528,-51.9981652289242,
-29.9982967655718));
#26202=CARTESIAN_POINT('Ctrl Pts',(-16.8177576495502,-48.7808087276896,
-29.8403482423794));
#26203=CARTESIAN_POINT('Ctrl Pts',(-19.2812701892749,-46.6688558730247,
-29.6823997191869));
#26204=CARTESIAN_POINT('Ctrl Pts',(-22.3964331892039,-47.5771500861349,
-29.5244511959945));
#26205=CARTESIAN_POINT('Ctrl Pts',(-23.3388231007046,-50.6821686284665,
-29.3665026728019));
#26206=CARTESIAN_POINT('Ctrl Pts',(-21.2540036525068,-53.1686856226499,
-29.2085541496095));
#26207=CARTESIAN_POINT('Ctrl Pts',(-18.0322172313861,-52.7822517338714,
-29.050605626417));
#26208=CARTESIAN_POINT('Ctrl Pts',(-16.5945595991443,-49.8732348165961,
-28.8926571032245));
#26209=CARTESIAN_POINT('Ctrl Pts',(-18.2445112066017,-47.0791520352407,
-28.7347085800321));
#26210=CARTESIAN_POINT('Ctrl Pts',(-21.4861111121929,-46.93331327092,-28.5767600568396));
#26211=CARTESIAN_POINT('Ctrl Pts',(-23.3802992705091,-49.5679460928791,
-28.4188115336471));
#26212=CARTESIAN_POINT('Ctrl Pts',(-22.2096728871631,-52.5943090559135,
-28.2608630104547));
#26213=CARTESIAN_POINT('Ctrl Pts',(-19.0356033016802,-53.2684908927021,
-28.1029144872622));
#26214=CARTESIAN_POINT('Ctrl Pts',(-16.7359228707871,-50.9792314588465,
-27.9449659640698));
#26215=CARTESIAN_POINT('Ctrl Pts',(-17.3956819024776,-47.8021326131544,
-27.7870174408773));
#26216=CARTESIAN_POINT('Ctrl Pts',(-20.4166969425664,-46.6177733418703,
-27.6290689176848));
#26217=CARTESIAN_POINT('Ctrl Pts',(-23.0599055457993,-48.4999759965714,
-27.4711203944923));
#26218=CARTESIAN_POINT('Ctrl Pts',(-22.9287908381411,-51.7422050312076,
-27.3131718712999));
#26219=CARTESIAN_POINT('Ctrl Pts',(-20.1422305832111,-53.4048292786993,
-27.1552233481074));
#26220=CARTESIAN_POINT('Ctrl Pts',(-17.2267141234753,-51.9803993121182,
-26.9972748249149));
#26221=CARTESIAN_POINT('Ctrl Pts',(-16.8256517432378,-48.7603996499074,
-26.8393263017224));
#26222=CARTESIAN_POINT('Ctrl Pts',(-19.3026741432644,-46.6643116473999,
-26.68137777853));
#26223=CARTESIAN_POINT('Ctrl Pts',(-22.4119411684913,-47.5925834134076,
-26.5234292553375));
#26224=CARTESIAN_POINT('Ctrl Pts',(-23.3343735384945,-50.7036013301426,
-26.3654807321451));
#26225=CARTESIAN_POINT('Ctrl Pts',(-21.2336327296632,-53.1766559611554,
-26.2075322089526));
#26226=CARTESIAN_POINT('Ctrl Pts',(-18.0143908659877,-52.7695916824433,
-26.0495836857601));
#26227=CARTESIAN_POINT('Ctrl Pts',(-16.5954479345883,-49.8513065443232,
-25.8916351625677));
#26228=CARTESIAN_POINT('Ctrl Pts',(-18.2632938482488,-47.068068756599,-25.7336866393752));
#26229=CARTESIAN_POINT('Ctrl Pts',(-21.5057881994898,-46.9426630299526,
-25.5757381161827));
#26230=CARTESIAN_POINT('Ctrl Pts',(-23.3829709341586,-49.5901691036368,
-25.4177895929902));
#26231=CARTESIAN_POINT('Ctrl Pts',(-22.1930342320574,-52.60742906916,-25.2598410697978));
#26232=CARTESIAN_POINT('Ctrl Pts',(-19.0145130597135,-53.2642672214192,
-25.1018925466053));
#26233=CARTESIAN_POINT('Ctrl Pts',(-16.7298791822334,-50.9540045243841,
-24.9439440234128));
#26234=CARTESIAN_POINT('Ctrl Pts',(-17.1839240578764,-48.8493222806574,
-24.8386450079512));
#26235=CARTESIAN_POINT('Ctrl Pts',(-17.8048028959808,-48.1231365609213,
-24.7859955002204));
#26236=CARTESIAN_POINT('Ctrl Pts',(-19.301933573839,-52.6111321859386,-40.2140044997796));
#26237=CARTESIAN_POINT('Ctrl Pts',(-18.4381537782571,-52.3802071955689,
-40.1613549920488));
#26238=CARTESIAN_POINT('Ctrl Pts',(-16.9723081910803,-50.9977214006572,
-40.0560559765871));
#26239=CARTESIAN_POINT('Ctrl Pts',(-17.5096080728378,-48.0049334824034,
-39.8981074533947));
#26240=CARTESIAN_POINT('Ctrl Pts',(-20.3091306375097,-46.8265879379253,
-39.7401589302022));
#26241=CARTESIAN_POINT('Ctrl Pts',(-22.8262613690466,-48.522780272286,-39.5822104070098));
#26242=CARTESIAN_POINT('Ctrl Pts',(-22.781966079563,-51.5596698248994,-39.4242618838172));
#26243=CARTESIAN_POINT('Ctrl Pts',(-20.2148147755746,-53.1817781104246,
-39.2663133606248));
#26244=CARTESIAN_POINT('Ctrl Pts',(-17.4531647029619,-51.9194045599905,
-39.1083648374323));
#26245=CARTESIAN_POINT('Ctrl Pts',(-17.0005184669122,-48.9165946554572,
-38.9504163142399));
#26246=CARTESIAN_POINT('Ctrl Pts',(-19.2674783687833,-46.8961611440324,
-38.7924677910474));
#26247=CARTESIAN_POINT('Ctrl Pts',(-22.1985594644447,-47.6898408596029,
-38.634519267855));
#26248=CARTESIAN_POINT('Ctrl Pts',(-23.1362905866011,-50.5780932433083,
-38.4765707446625));
#26249=CARTESIAN_POINT('Ctrl Pts',(-21.2304338655621,-52.9421951952963,
-38.31862222147));
#26250=CARTESIAN_POINT('Ctrl Pts',(-18.2089844782754,-52.6387037076143,
-38.1606736982775));
#26251=CARTESIAN_POINT('Ctrl Pts',(-16.8113922340818,-49.9427770771181,
-38.002725175085));
#26252=CARTESIAN_POINT('Ctrl Pts',(-18.3048147589036,-47.298734108869,-37.8447766518926));
#26253=CARTESIAN_POINT('Ctrl Pts',(-21.3352096401026,-47.103846076294,-37.6868281287001));
#26254=CARTESIAN_POINT('Ctrl Pts',(-23.1550108229941,-49.5348130717306,
-37.5288796055077));
#26255=CARTESIAN_POINT('Ctrl Pts',(-22.1142595104314,-52.3875507322084,
-37.3709310823152));
#26256=CARTESIAN_POINT('Ctrl Pts',(-19.1565734711686,-53.0755688456859,
-37.2129825591228));
#26257=CARTESIAN_POINT('Ctrl Pts',(-16.9635965792169,-50.9750621818571,
-37.0550340359302));
#26258=CARTESIAN_POINT('Ctrl Pts',(-17.5236343382981,-47.9904963150807,
-36.8970855127378));
#26259=CARTESIAN_POINT('Ctrl Pts',(-20.3289175188232,-46.8278863119923,
-36.7391369895453));
#26260=CARTESIAN_POINT('Ctrl Pts',(-22.8359811930086,-48.5413353199386,
-36.5811884663528));
#26261=CARTESIAN_POINT('Ctrl Pts',(-22.77174696975,-51.5773112272049,-36.4232399431604));
#26262=CARTESIAN_POINT('Ctrl Pts',(-20.1944540690039,-53.1831870179292,
-36.2652914199679));
#26263=CARTESIAN_POINT('Ctrl Pts',(-17.4408555773868,-51.9029639510444,
-36.1073428967755));
#26264=CARTESIAN_POINT('Ctrl Pts',(-17.0075555011744,-48.8973813461366,
-35.949394373583));
#26265=CARTESIAN_POINT('Ctrl Pts',(-19.2874138408208,-46.8915095398771,
-35.7914458503905));
#26266=CARTESIAN_POINT('Ctrl Pts',(-22.2133523787375,-47.7040114934373,
-35.633497327198));
#26267=CARTESIAN_POINT('Ctrl Pts',(-23.1325116308869,-50.5982163965188,
-35.4755488040056));
#26268=CARTESIAN_POINT('Ctrl Pts',(-21.2115178583638,-52.9500366868287,
-35.3176002808131));
#26269=CARTESIAN_POINT('Ctrl Pts',(-18.1920776903032,-52.6271484344897,
-35.1596517576206));
#26270=CARTESIAN_POINT('Ctrl Pts',(-16.8118256949778,-49.9223045977125,
-35.0017032344282));
#26271=CARTESIAN_POINT('Ctrl Pts',(-18.3221943780753,-47.2879048191876,
-34.8437547112357));
#26272=CARTESIAN_POINT('Ctrl Pts',(-21.3537783904218,-47.1124792564605,
-34.6858061880432));
#26273=CARTESIAN_POINT('Ctrl Pts',(-23.1579327094808,-49.5550809319264,
-34.5278576648508));
#26274=CARTESIAN_POINT('Ctrl Pts',(-22.0988854850357,-52.4010771948131,
-34.3699091416583));
#26275=CARTESIAN_POINT('Ctrl Pts',(-19.136842626025,-53.0700897906246,-34.2119606184658));
#26276=CARTESIAN_POINT('Ctrl Pts',(-16.9573983062527,-50.955545345837,-34.0540120952733));
#26277=CARTESIAN_POINT('Ctrl Pts',(-17.5365884056535,-47.9746369975769,
-33.8960635720809));
#26278=CARTESIAN_POINT('Ctrl Pts',(-20.3492788763714,-46.8300636849827,
-33.7381150488884));
#26279=CARTESIAN_POINT('Ctrl Pts',(-22.8452888127201,-48.5595752199596,
-33.5801665256959));
#26280=CARTESIAN_POINT('Ctrl Pts',(-22.7615619181231,-51.5950760944598,
-33.4222180025035));
#26281=CARTESIAN_POINT('Ctrl Pts',(-20.1740108214729,-53.1843699861598,
-33.264269479311));
#26282=CARTESIAN_POINT('Ctrl Pts',(-17.4286894052932,-51.8864924596438,
-33.1063209561186));
#26283=CARTESIAN_POINT('Ctrl Pts',(-17.0146971024574,-48.8781895950435,
-32.9483724329261));
#26284=CARTESIAN_POINT('Ctrl Pts',(-19.3073881429401,-46.886998106296,-32.7904239097336));
#26285=CARTESIAN_POINT('Ctrl Pts',(-22.2280492893816,-47.7182707568971,
-32.6324753865411));
#26286=CARTESIAN_POINT('Ctrl Pts',(-23.1286059081968,-50.6183179165617,
-32.4745268633487));
#26287=CARTESIAN_POINT('Ctrl Pts',(-21.1925507022974,-52.9577550265691,
-32.3165783401562));
#26288=CARTESIAN_POINT('Ctrl Pts',(-18.1752460444151,-52.6154856100391,
-32.1586298169637));
#26289=CARTESIAN_POINT('Ctrl Pts',(-16.8123903006787,-49.9018349372858,
-32.0006812937713));
#26290=CARTESIAN_POINT('Ctrl Pts',(-18.3396433245503,-47.2771875413399,
-31.8427327705788));
#26291=CARTESIAN_POINT('Ctrl Pts',(-21.3722912485865,-47.1212313910636,
-31.6847842473863));
#26292=CARTESIAN_POINT('Ctrl Pts',(-23.160724433881,-49.5753671847204,-31.5268357241938));
#26293=CARTESIAN_POINT('Ctrl Pts',(-22.0834249040639,-52.414504637368,-31.3688872010014));
#26294=CARTESIAN_POINT('Ctrl Pts',(-19.1171473782361,-53.0644841691531,
-31.2109386778089));
#26295=CARTESIAN_POINT('Ctrl Pts',(-16.951325473813,-50.9359891068399,-31.0529901546164));
#26296=CARTESIAN_POINT('Ctrl Pts',(-17.5496440410392,-47.9588611881771,
-30.895041631424));
#26297=CARTESIAN_POINT('Ctrl Pts',(-20.3696258320475,-46.8323717517629,
-30.7370931082315));
#26298=CARTESIAN_POINT('Ctrl Pts',(-22.8544791227998,-48.5778745089676,
-30.5791445850391));
#26299=CARTESIAN_POINT('Ctrl Pts',(-22.7512630079677,-51.6127751968989,
-30.4211960618466));
#26300=CARTESIAN_POINT('Ctrl Pts',(-20.1535603996932,-53.1854216641434,
-30.2632475386541));
#26301=CARTESIAN_POINT('Ctrl Pts',(-17.4166292473454,-51.8699431887277,
-30.1052990154616));
#26302=CARTESIAN_POINT('Ctrl Pts',(-17.0219617867595,-48.8590440958476,
-29.9473504922692));
#26303=CARTESIAN_POINT('Ctrl Pts',(-19.3273910011813,-46.8826150206499,
-29.7894019690767));
#26304=CARTESIAN_POINT('Ctrl Pts',(-22.242654338353,-47.7326240952651,-29.6314534458843));
#26305=CARTESIAN_POINT('Ctrl Pts',(-23.1245711941905,-50.6383939435537,
-29.4735049226917));
#26306=CARTESIAN_POINT('Ctrl Pts',(-21.1735343777889,-52.9653514191537,
-29.3155563994993));
#26307=CARTESIAN_POINT('Ctrl Pts',(-18.1584896324882,-52.6037149499794,
-29.1576078763068));
#26308=CARTESIAN_POINT('Ctrl Pts',(-16.8130863303897,-49.8813693242968,
-28.9996593531144));
#26309=CARTESIAN_POINT('Ctrl Pts',(-18.3571607269583,-47.2665825238328,
-28.8417108299219));
#26310=CARTESIAN_POINT('Ctrl Pts',(-21.3907475276376,-47.1301022167759,
-28.6837623067294));
#26311=CARTESIAN_POINT('Ctrl Pts',(-23.163385842798,-49.5956709439795,-28.525813783537));
#26312=CARTESIAN_POINT('Ctrl Pts',(-22.067878424094,-52.4278325327341,-28.3678652603445));
#26313=CARTESIAN_POINT('Ctrl Pts',(-19.0974885304027,-53.0587521961423,
-28.209916737152));
#26314=CARTESIAN_POINT('Ctrl Pts',(-16.9453783366354,-50.9163942851932,
-28.0519682139596));
#26315=CARTESIAN_POINT('Ctrl Pts',(-17.5628007047423,-47.943169518583,-27.8940196907671));
#26316=CARTESIAN_POINT('Ctrl Pts',(-20.3899575461711,-46.8348104498304,
-27.7360711675746));
#26317=CARTESIAN_POINT('Ctrl Pts',(-22.8635517477194,-48.5962323698076,
-27.5781226443821));
#26318=CARTESIAN_POINT('Ctrl Pts',(-22.7408506562487,-51.6304079283914,
-27.4201741211897));
#26319=CARTESIAN_POINT('Ctrl Pts',(-20.1331036625272,-53.1863417630947,
-27.2622255979972));
#26320=CARTESIAN_POINT('Ctrl Pts',(-17.4046755693,-51.8533173088245,-27.1042770748047));
#26321=CARTESIAN_POINT('Ctrl Pts',(-17.0293493173344,-48.8399446663136,
-26.9463285516123));
#26322=CARTESIAN_POINT('Ctrl Pts',(-19.3474214658271,-46.8783623974773,
-26.7883800284198));
#26323=CARTESIAN_POINT('Ctrl Pts',(-22.2571671723368,-47.7470670676456,
-26.6304315052273));
#26324=CARTESIAN_POINT('Ctrl Pts',(-23.1204071598918,-50.6584513111502,
-26.4724829820349));
#26325=CARTESIAN_POINT('Ctrl Pts',(-21.1544706547953,-52.972810301925,-26.3145344588424));
#26326=CARTESIAN_POINT('Ctrl Pts',(-18.141807182972,-52.5918672926414,-26.1565859356499));
#26327=CARTESIAN_POINT('Ctrl Pts',(-16.8139176614472,-49.8608481868135,
-25.9986374124575));
#26328=CARTESIAN_POINT('Ctrl Pts',(-18.3747380885828,-47.2562104579471,
-25.840688889265));
#26329=CARTESIAN_POINT('Ctrl Pts',(-21.4091619384342,-47.1388520028128,
-25.6827403660725));
#26330=CARTESIAN_POINT('Ctrl Pts',(-23.1658860660886,-49.6164679066119,
-25.5247918428801));
#26331=CARTESIAN_POINT('Ctrl Pts',(-22.0523074696332,-52.4401106361917,
-25.3668433196876));
#26332=CARTESIAN_POINT('Ctrl Pts',(-19.077751646914,-53.0547995573753,-25.2088947964951));
#26333=CARTESIAN_POINT('Ctrl Pts',(-16.9397224709031,-50.8927861603057,
-25.0509462733027));
#26334=CARTESIAN_POINT('Ctrl Pts',(-17.3646313374448,-48.923161141752,-24.945647257841));
#26335=CARTESIAN_POINT('Ctrl Pts',(-17.9456684496579,-48.2435746787732,
-24.8929977501102));
#26336=CARTESIAN_POINT('Ctrl Pts',(-19.3498000020249,-52.4320868020351,
-40.3210067496694));
#26337=CARTESIAN_POINT('Ctrl Pts',(-18.5452496035378,-52.2169963426693,
-40.2683572419386));
#26338=CARTESIAN_POINT('Ctrl Pts',(-17.1799170762945,-50.9293076251419,
-40.163058226477));
#26339=CARTESIAN_POINT('Ctrl Pts',(-17.680374294889,-48.1417352316521,-40.0051097032845));
#26340=CARTESIAN_POINT('Ctrl Pts',(-20.2879335437864,-47.0441888636839,
-39.847161180092));
#26341=CARTESIAN_POINT('Ctrl Pts',(-22.632464572945,-48.6240732572535,-39.6892126568995));
#26342=CARTESIAN_POINT('Ctrl Pts',(-22.591206612308,-51.4527232351918,-39.5312641337071));
#26343=CARTESIAN_POINT('Ctrl Pts',(-20.2000849223071,-52.9636035245707,
-39.3733156105146));
#26344=CARTESIAN_POINT('Ctrl Pts',(-17.6278012479644,-51.7877909526211,
-39.2153670873221));
#26345=CARTESIAN_POINT('Ctrl Pts',(-17.2061929729734,-48.9908837806426,
-39.0574185641297));
#26346=CARTESIAN_POINT('Ctrl Pts',(-19.3177073910386,-47.1089914337183,
-38.8994700409372));
#26347=CARTESIAN_POINT('Ctrl Pts',(-22.0478041999406,-47.8482485160203,
-38.7415215177447));
#26348=CARTESIAN_POINT('Ctrl Pts',(-22.9212350811254,-50.538453378564,-38.5835729945523));
#26349=CARTESIAN_POINT('Ctrl Pts',(-21.1460629918798,-52.7404488145126,
-38.4256244713598));
#26350=CARTESIAN_POINT('Ctrl Pts',(-18.3317944468367,-52.4577677439425,
-38.2676759481673));
#26351=CARTESIAN_POINT('Ctrl Pts',(-17.0300351295434,-49.946700854034,-38.1097274249748));
#26352=CARTESIAN_POINT('Ctrl Pts',(-18.4210536432903,-47.4839599626605,
-37.9517789017824));
#26353=CARTESIAN_POINT('Ctrl Pts',(-21.2436542895572,-47.3024354062046,
-37.7938303785899));
#26354=CARTESIAN_POINT('Ctrl Pts',(-22.938671670551,-49.5667109482944,-37.6358818553975));
#26355=CARTESIAN_POINT('Ctrl Pts',(-21.9692846953855,-52.2238363328611,
-37.477933332205));
#26356=CARTESIAN_POINT('Ctrl Pts',(-19.2144072443732,-52.8646770311455,
-37.3199848090126));
#26357=CARTESIAN_POINT('Ctrl Pts',(-17.1718028198231,-50.9082021494081,
-37.1620362858201));
#26358=CARTESIAN_POINT('Ctrl Pts',(-17.6934387790586,-48.1282880211688,
-37.0040877626276));
#26359=CARTESIAN_POINT('Ctrl Pts',(-20.30636363827,-47.0453982082162,-36.8461392394351));
#26360=CARTESIAN_POINT('Ctrl Pts',(-22.6415179083921,-48.6413559849339,
-36.6881907162427));
#26361=CARTESIAN_POINT('Ctrl Pts',(-22.5816882270502,-51.4691549662039,
-36.5302421930502));
#26362=CARTESIAN_POINT('Ctrl Pts',(-20.1811203497752,-52.9649158232608,
-36.3722936698577));
#26363=CARTESIAN_POINT('Ctrl Pts',(-17.6163361593653,-51.7724776765447,
-36.2143451466653));
#26364=CARTESIAN_POINT('Ctrl Pts',(-17.2127474776616,-48.9729879283094,
-36.0563966234728));
#26365=CARTESIAN_POINT('Ctrl Pts',(-19.3362758873773,-47.1046587901488,
-35.8984481002803));
#26366=CARTESIAN_POINT('Ctrl Pts',(-22.0615827638175,-47.8614474692219,
-35.7404995770878));
#26367=CARTESIAN_POINT('Ctrl Pts',(-22.9177152484768,-50.5571966867741,
-35.5825510538954));
#26368=CARTESIAN_POINT('Ctrl Pts',(-21.1284440556567,-52.7477526148208,
-35.4246025307029));
#26369=CARTESIAN_POINT('Ctrl Pts',(-18.316046957639,-52.4470048161168,-35.2666540075105));
#26370=CARTESIAN_POINT('Ctrl Pts',(-17.0304388680174,-49.9276321729325,
-35.1087054843179));
#26371=CARTESIAN_POINT('Ctrl Pts',(-18.4372415416432,-47.4738732375796,
-34.9507569611255));
#26372=CARTESIAN_POINT('Ctrl Pts',(-21.2609497803121,-47.3104766090421,
-34.792808437933));
#26373=CARTESIAN_POINT('Ctrl Pts',(-22.9413932032255,-49.5855890409291,
-34.6348599147406));
#26374=CARTESIAN_POINT('Ctrl Pts',(-21.954964867205,-52.2364352856664,-34.4769113915481));
#26375=CARTESIAN_POINT('Ctrl Pts',(-19.1960293436584,-52.8595736749944,
-34.3189628683556));
#26376=CARTESIAN_POINT('Ctrl Pts',(-17.1660295625545,-50.890023583207,-34.1610143451632));
#26377=CARTESIAN_POINT('Ctrl Pts',(-17.7055045857678,-48.1135161773694,
-34.0030658219706));
#26378=CARTESIAN_POINT('Ctrl Pts',(-20.3253288171419,-47.0474262786991,
-33.8451172987783));
#26379=CARTESIAN_POINT('Ctrl Pts',(-22.6501873044421,-48.6583451746618,
-33.6871687755857));
#26380=CARTESIAN_POINT('Ctrl Pts',(-22.5722015646081,-51.4857016961716,
-33.5292202523933));
#26381=CARTESIAN_POINT('Ctrl Pts',(-20.1620788961182,-52.9660176753372,
-33.3712717292008));
#26382=CARTESIAN_POINT('Ctrl Pts',(-17.6050042219247,-51.7571356356244,
-33.2133232060083));
#26383=CARTESIAN_POINT('Ctrl Pts',(-17.2193993792082,-48.9551121559556,
-33.0553746828159));
#26384=CARTESIAN_POINT('Ctrl Pts',(-19.3548805512185,-47.1004567056546,
-32.8974261596234));
#26385=CARTESIAN_POINT('Ctrl Pts',(-22.0752719070179,-47.8747289747136,
-32.7394776364309));
#26386=CARTESIAN_POINT('Ctrl Pts',(-22.9140773412661,-50.5759198452034,
-32.5815291132385));
#26387=CARTESIAN_POINT('Ctrl Pts',(-21.1107774778443,-52.7549417078576,
-32.423580590046));
#26388=CARTESIAN_POINT('Ctrl Pts',(-18.3003694580311,-52.4361417117618,
-32.2656320668536));
#26389=CARTESIAN_POINT('Ctrl Pts',(-17.0309647586947,-49.9085661175126,
-32.107683543661));
#26390=CARTESIAN_POINT('Ctrl Pts',(-18.4534940135249,-47.4638908436788,
-31.9497350204686));
#26391=CARTESIAN_POINT('Ctrl Pts',(-21.2781932114386,-47.3186286096082,
-31.7917864972761));
#26392=CARTESIAN_POINT('Ctrl Pts',(-22.9439934990302,-49.6044842649813,
-31.6338379740836));
#26393=CARTESIAN_POINT('Ctrl Pts',(-21.940564418566,-52.2489420082286,-31.4758894508913));
#26394=CARTESIAN_POINT('Ctrl Pts',(-19.1776845993869,-52.8543524310943,
-31.3179409276987));
#26395=CARTESIAN_POINT('Ctrl Pts',(-17.1603731443513,-50.8718083158917,
-31.1599924045063));
#26396=CARTESIAN_POINT('Ctrl Pts',(-17.7176649959856,-48.0988221155217,
-31.0020438813138));
#26397=CARTESIAN_POINT('Ctrl Pts',(-20.3442805816783,-47.0495760812962,
-30.8440953581213));
#26398=CARTESIAN_POINT('Ctrl Pts',(-22.658747434784,-48.6753896810726,-30.6861468349289));
#26399=CARTESIAN_POINT('Ctrl Pts',(-22.5626088509189,-51.5021871708183,
-30.5281983117364));
#26400=CARTESIAN_POINT('Ctrl Pts',(-20.1430307601508,-52.9669972397414,
-30.3702497885439));
#26401=CARTESIAN_POINT('Ctrl Pts',(-17.5937710292379,-51.7417211485313,
-30.2123012653515));
#26402=CARTESIAN_POINT('Ctrl Pts',(-17.2261659239688,-48.9372794640055,
-30.054352742159));
#26403=CARTESIAN_POINT('Ctrl Pts',(-19.3735118130877,-47.0963741682751,
-29.8964042189665));
#26404=CARTESIAN_POINT('Ctrl Pts',(-22.0888754875022,-47.8880981043954,
-29.7384556957741));
#26405=CARTESIAN_POINT('Ctrl Pts',(-22.9103192876763,-50.5946192586408,
-29.5805071725816));
#26406=CARTESIAN_POINT('Ctrl Pts',(-21.0930651030709,-52.7620172156573,
-29.4225586493891));
#26407=CARTESIAN_POINT('Ctrl Pts',(-18.2847620335903,-52.4251781660874,
-29.2646101261966));
#26408=CARTESIAN_POINT('Ctrl Pts',(-17.0316130616351,-49.8895038319974,
-29.1066616030042));
#26409=CARTESIAN_POINT('Ctrl Pts',(-18.4698102473148,-47.454013012425,-28.9487130798117));
#26410=CARTESIAN_POINT('Ctrl Pts',(-21.2953839430823,-47.3268911626317,
-28.7907645566192));
#26411=CARTESIAN_POINT('Ctrl Pts',(-22.9464724150868,-49.6233957950799,
-28.6328160334268));
#26412=CARTESIAN_POINT('Ctrl Pts',(-21.9260839610248,-52.2613560095547,
-28.4748675102343));
#26413=CARTESIAN_POINT('Ctrl Pts',(-19.1593737591251,-52.8490134995825,
-28.3169189870418));
#26414=CARTESIAN_POINT('Ctrl Pts',(-17.1548338024837,-50.85355711154,-28.1589704638494));
#26415=CARTESIAN_POINT('Ctrl Pts',(-17.729919507007,-48.0842064240116,-28.0010219406569));
#26416=CARTESIAN_POINT('Ctrl Pts',(-20.3632181497758,-47.0518475577905,
-27.8430734174644));
#26417=CARTESIAN_POINT('Ctrl Pts',(-22.6671979496393,-48.692488743044,-27.685124894272));
#26418=CARTESIAN_POINT('Ctrl Pts',(-22.5529104743563,-51.5186108255752,
-27.5271763710795));
#26419=CARTESIAN_POINT('Ctrl Pts',(-20.1239767418433,-52.9678542474899,
-27.369227847887));
#26420=CARTESIAN_POINT('Ctrl Pts',(-17.5826370151246,-51.7262353055309,
-27.2112793246945));
#26421=CARTESIAN_POINT('Ctrl Pts',(-17.233046891431,-48.9194896827197,-27.0533308015021));
#26422=CARTESIAN_POINT('Ctrl Pts',(-19.3921687883899,-47.0924131475548,
-26.8953822783096));
#26423=CARTESIAN_POINT('Ctrl Pts',(-22.1023931761822,-47.9015507218836,
-26.7374337551172));
#26424=CARTESIAN_POINT('Ctrl Pts',(-22.9064407812892,-50.6133012921579,
-26.5794852319247));
#26425=CARTESIAN_POINT('Ctrl Pts',(-21.0753085799274,-52.7689646426944,
-26.4215367087322));
#26426=CARTESIAN_POINT('Ctrl Pts',(-18.2692234999564,-52.4141429028396,
-26.2635881855398));
#26427=CARTESIAN_POINT('Ctrl Pts',(-17.0323873883061,-49.8703898293036,
-26.1056396623473));
#26428=CARTESIAN_POINT('Ctrl Pts',(-18.4861823289167,-47.4443521592953,
-25.9476911391548));
#26429=CARTESIAN_POINT('Ctrl Pts',(-21.3125356773786,-47.3350409756728,
-25.7897426159623));
#26430=CARTESIAN_POINT('Ctrl Pts',(-22.9488011980187,-49.6427667095871,
-25.6317940927699));
#26431=CARTESIAN_POINT('Ctrl Pts',(-21.9115807072091,-52.2727922032235,
-25.4738455695774));
#26432=CARTESIAN_POINT('Ctrl Pts',(-19.1409902341146,-52.8453318933313,
-25.3158970463849));
#26433=CARTESIAN_POINT('Ctrl Pts',(-17.1495657595727,-50.8315677962272,
-25.1579485231925));
#26434=CARTESIAN_POINT('Ctrl Pts',(-17.5453386170133,-48.9970000028466,
-25.0526495077308));
#26435=CARTESIAN_POINT('Ctrl Pts',(-18.0865340033349,-48.3640127966251,
-25.));
#26436=CARTESIAN_POINT('Ctrl Pts',(-17.4850545138796,-49.9982392692185,
-39.112583302492));
#26437=CARTESIAN_POINT('Ctrl Pts',(-17.4831412917956,-49.7066909038706,
-39.0941950563712));
#26438=CARTESIAN_POINT('Ctrl Pts',(-17.5300112989184,-49.4157373800817,
-39.0758068102505));
#26439=CARTESIAN_POINT('Ctrl Pts',(-17.6283800884828,-49.143386251485,-39.0574185641297));
#26440=CARTESIAN_POINT('Ctrl Pts',(-17.9100311123284,-48.3635863316678,
-39.0047690563989));
#26441=CARTESIAN_POINT('Ctrl Pts',(-18.6138692516835,-47.736288882693,-38.9521195486681));
#26442=CARTESIAN_POINT('Ctrl Pts',(-19.420804456178,-47.5458496719227,-38.8994700409372));
#26443=CARTESIAN_POINT('Ctrl Pts',(-20.2277396606726,-47.3554104611523,
-38.8468205332064));
#26444=CARTESIAN_POINT('Ctrl Pts',(-21.1377719303066,-47.6018294885863,
-38.7941710254756));
#26445=CARTESIAN_POINT('Ctrl Pts',(-21.7383598786544,-48.1734064793939,
-38.7415215177447));
#26446=CARTESIAN_POINT('Ctrl Pts',(-22.3389478270022,-48.7449834702016,
-38.6888720100139));
#26447=CARTESIAN_POINT('Ctrl Pts',(-22.6300914540638,-49.6417184243828,
-38.6362225022831));
#26448=CARTESIAN_POINT('Ctrl Pts',(-22.4798012527203,-50.4570851407982,
-38.5835729945523));
#26449=CARTESIAN_POINT('Ctrl Pts',(-22.3295110513769,-51.2724518572135,
-38.5309234868215));
#26450=CARTESIAN_POINT('Ctrl Pts',(-21.7377870216284,-52.0064503358631,
-38.4782739790906));
#26451=CARTESIAN_POINT('Ctrl Pts',(-20.9728802492469,-52.3263360634262,
-38.4256244713598));
#26452=CARTESIAN_POINT('Ctrl Pts',(-20.2079734768655,-52.6462217909892,
-38.372974963629));
#26453=CARTESIAN_POINT('Ctrl Pts',(-19.2698839618511,-52.5519947674658,
-38.3203254558982));
#26454=CARTESIAN_POINT('Ctrl Pts',(-18.5838793181283,-52.0863701073861,
-38.2676759481673));
#26455=CARTESIAN_POINT('Ctrl Pts',(-17.9102783689704,-51.6291644370585,
-38.2159783996089));
#26456=CARTESIAN_POINT('Ctrl Pts',(-17.4797287780335,-50.813870240662,-38.1642808510504));
#26457=CARTESIAN_POINT('Ctrl Pts',(-17.4784634893366,-49.9997267145485,
-38.112583302492));
#26458=CARTESIAN_POINT('Origin',(-20.,-50.,-32.));
#26459=CARTESIAN_POINT('Origin',(-20.,50.,-25.));
#26460=CARTESIAN_POINT('Ctrl Pts',(-18.0865340033349,51.6359872033749,-25.));
#26461=CARTESIAN_POINT('Ctrl Pts',(-18.0243833228338,51.5775808249506,-25.));
#26462=CARTESIAN_POINT('Ctrl Pts',(-17.9656072042478,51.5159215542002,-25.));
#26463=CARTESIAN_POINT('Ctrl Pts',(-17.9102180900498,51.4513856299869,-25.));
#26464=CARTESIAN_POINT('Ctrl Pts',(-17.8534757442914,51.3852730051767,-25.));
#26465=CARTESIAN_POINT('Ctrl Pts',(-17.8002874537736,51.3161409574413,-25.));
#26466=CARTESIAN_POINT('Ctrl Pts',(-17.7506954746655,51.2443477068885,-25.));
#26467=CARTESIAN_POINT('Ctrl Pts',(-17.7377283789557,51.2255755189666,-25.));
#26468=CARTESIAN_POINT('Ctrl Pts',(-17.7250073328008,51.2066211684088,-25.));
#26469=CARTESIAN_POINT('Ctrl Pts',(-17.712533469509,51.1874906231763,-25.));
#26470=CARTESIAN_POINT('Ctrl Pts',(-17.7024059324163,51.1719585220211,-25.));
#26471=CARTESIAN_POINT('Ctrl Pts',(-17.6924409292295,51.156309427101,-25.));
#26472=CARTESIAN_POINT('Ctrl Pts',(-17.682647813279,51.1405609613993,-25.));
#26473=CARTESIAN_POINT('Ctrl Pts',(-17.6351885166707,51.0642409108008,-25.));
#26474=CARTESIAN_POINT('Ctrl Pts',(-17.5917126522887,50.9855142151719,-25.));
#26475=CARTESIAN_POINT('Ctrl Pts',(-17.5522554123681,50.9047730795493,-25.));
#26476=CARTESIAN_POINT('Ctrl Pts',(-17.5204203008065,50.8396290637662,-25.));
#26477=CARTESIAN_POINT('Ctrl Pts',(-17.4912016837347,50.7731726244963,-25.));
#26478=CARTESIAN_POINT('Ctrl Pts',(-17.4646351938,50.7055919593486,-25.));
#26479=CARTESIAN_POINT('Ctrl Pts',(-17.4539844043915,50.6784981492764,-25.));
#26480=CARTESIAN_POINT('Ctrl Pts',(-17.4437600743761,50.6512234901344,-25.));
#26481=CARTESIAN_POINT('Ctrl Pts',(-17.4339652711491,50.6237795558022,-25.));
#26482=CARTESIAN_POINT('Ctrl Pts',(-17.4287336556888,50.6091211591182,-25.));
#26483=CARTESIAN_POINT('Ctrl Pts',(-17.4236250235962,50.5944154772993,-25.));
#26484=CARTESIAN_POINT('Ctrl Pts',(-17.41864375021,50.5796764952228,-25.));
#26485=CARTESIAN_POINT('Ctrl Pts',(-17.3890989440111,50.4922570072194,-25.));
#26486=CARTESIAN_POINT('Ctrl Pts',(-17.3639908537199,50.4035567266403,-25.));
#26487=CARTESIAN_POINT('Ctrl Pts',(-17.3433526020187,50.3139730842995,-25.));
#26488=CARTESIAN_POINT('Ctrl Pts',(-17.322396152995,50.223008255434,-25.));
#26489=CARTESIAN_POINT('Ctrl Pts',(-17.3060479349661,50.131131810167,-25.));
#26490=CARTESIAN_POINT('Ctrl Pts',(-17.2943844478798,50.0387266921583,-25.));
#26491=CARTESIAN_POINT('Ctrl Pts',(-17.2828125669698,49.9470473330473,-25.));
#26492=CARTESIAN_POINT('Ctrl Pts',(-17.2758517728664,49.8548466441588,-25.));
#26493=CARTESIAN_POINT('Ctrl Pts',(-17.2736237166568,49.7624794304333,-25.));
#26494=CARTESIAN_POINT('Ctrl Pts',(-17.2725154991996,49.7165367121665,-25.));
#26495=CARTESIAN_POINT('Ctrl Pts',(-17.2725789187574,49.6705525832056,-25.));
#26496=CARTESIAN_POINT('Ctrl Pts',(-17.2738337345407,49.6245700069453,-25.));
#26497=CARTESIAN_POINT('Ctrl Pts',(-17.2742445582872,49.6095154192502,-25.));
#26498=CARTESIAN_POINT('Ctrl Pts',(-17.2747831814028,49.5944594880405,-25.));
#26499=CARTESIAN_POINT('Ctrl Pts',(-17.2754501651331,49.5794084218269,-25.));
#26500=CARTESIAN_POINT('Ctrl Pts',(-17.2796911524576,49.483706865494,-25.));
#26501=CARTESIAN_POINT('Ctrl Pts',(-17.2891006969591,49.3885698423273,-25.));
#26502=CARTESIAN_POINT('Ctrl Pts',(-17.3037432826356,49.294395309891,-25.));
#26503=CARTESIAN_POINT('Ctrl Pts',(-17.3078992671603,49.2676658846328,-25.));
#26504=CARTESIAN_POINT('Ctrl Pts',(-17.3124771127594,49.2410138657042,-25.));
#26505=CARTESIAN_POINT('Ctrl Pts',(-17.3174790132619,49.2144480906985,-25.));
#26506=CARTESIAN_POINT('Ctrl Pts',(-17.3344212204447,49.1244657202194,-25.));
#26507=CARTESIAN_POINT('Ctrl Pts',(-17.3562243822145,49.0354729310092,-25.));
#26508=CARTESIAN_POINT('Ctrl Pts',(-17.3825856673629,48.9477022722757,-25.));
#26509=CARTESIAN_POINT('Ctrl Pts',(-17.4095441942202,48.8579430800576,-25.));
#26510=CARTESIAN_POINT('Ctrl Pts',(-17.441269931108,48.7694613223897,-25.));
#26511=CARTESIAN_POINT('Ctrl Pts',(-17.4774932435503,48.6825093747115,-25.));
#26512=CARTESIAN_POINT('Ctrl Pts',(-17.4899698857142,48.6525599232811,-25.));
#26513=CARTESIAN_POINT('Ctrl Pts',(-17.5029805545828,48.6227920442769,-25.));
#26514=CARTESIAN_POINT('Ctrl Pts',(-17.516515599114,48.59321638808,-25.));
#26515=CARTESIAN_POINT('Ctrl Pts',(-17.5231913782271,48.5786290295058,-25.));
#26516=CARTESIAN_POINT('Ctrl Pts',(-17.529994731303,48.5640884359945,-25.));
#26517=CARTESIAN_POINT('Ctrl Pts',(-17.5369245591161,48.5495959077351,-25.));
#26518=CARTESIAN_POINT('Ctrl Pts',(-17.5430261062936,48.5368355842061,-25.));
#26519=CARTESIAN_POINT('Ctrl Pts',(-17.5492249412562,48.5241142478127,-25.));
#26520=CARTESIAN_POINT('Ctrl Pts',(-17.5555148617866,48.5114432513385,-25.));
#26521=CARTESIAN_POINT('Ctrl Pts',(-17.5983742533158,48.425103337132,-25.));
#26522=CARTESIAN_POINT('Ctrl Pts',(-17.6455227691097,48.3409647245588,-25.));
#26523=CARTESIAN_POINT('Ctrl Pts',(-17.6966178449534,48.2592776638004,-25.));
#26524=CARTESIAN_POINT('Ctrl Pts',(-17.7487226127291,48.175976381616,-25.));
#26525=CARTESIAN_POINT('Ctrl Pts',(-17.8049317736166,48.0952237256181,-25.));
#26526=CARTESIAN_POINT('Ctrl Pts',(-17.8649370191223,48.0172922419165,-25.));
#26527=CARTESIAN_POINT('Ctrl Pts',(-17.9254206661132,47.9387394369082,-25.));
#26528=CARTESIAN_POINT('Ctrl Pts',(-17.989761629997,47.8630521302711,-25.));
#26529=CARTESIAN_POINT('Ctrl Pts',(-18.0576934095421,47.7905288730113,-25.));
#26530=CARTESIAN_POINT('Ctrl Pts',(-18.0946392725352,47.7510858561423,-25.));
#26531=CARTESIAN_POINT('Ctrl Pts',(-18.1326480797102,47.7125791482251,-25.));
#26532=CARTESIAN_POINT('Ctrl Pts',(-18.1716822386029,47.6750605369461,-25.));
#26533=CARTESIAN_POINT('Ctrl Pts',(-18.1843390275069,47.6628951629147,-25.));
#26534=CARTESIAN_POINT('Ctrl Pts',(-18.1971036460433,47.6508336993754,-25.));
#26535=CARTESIAN_POINT('Ctrl Pts',(-18.2099748874407,47.638877986089,-25.));
#26536=CARTESIAN_POINT('Ctrl Pts',(-18.2214598785455,47.6282099194662,-25.));
#26537=CARTESIAN_POINT('Ctrl Pts',(-18.2330243829329,47.6176310982102,-25.));
#26538=CARTESIAN_POINT('Ctrl Pts',(-18.2446619767169,47.6071472907025,-25.));
#26539=CARTESIAN_POINT('Ctrl Pts',(-18.3204767947681,47.5388489832147,-25.));
#26540=CARTESIAN_POINT('Ctrl Pts',(-18.3994577938915,47.4745180356072,-25.));
#26541=CARTESIAN_POINT('Ctrl Pts',(-18.4812785962965,47.4144375027462,-25.));
#26542=CARTESIAN_POINT('Ctrl Pts',(-18.5631717960198,47.3543038089612,-25.));
#26543=CARTESIAN_POINT('Ctrl Pts',(-18.6479104038285,47.2984272169749,-25.));
#26544=CARTESIAN_POINT('Ctrl Pts',(-18.7352121444042,47.2471177279551,-25.));
#26545=CARTESIAN_POINT('Ctrl Pts',(-18.820751629926,47.1968439617712,-25.));
#26546=CARTESIAN_POINT('Ctrl Pts',(-18.9087524795439,47.1509541033334,-25.));
#26547=CARTESIAN_POINT('Ctrl Pts',(-18.998982921958,47.1097758970613,-25.));
#26548=CARTESIAN_POINT('Ctrl Pts',(-19.0364028378792,47.092698678162,-25.));
#26549=CARTESIAN_POINT('Ctrl Pts',(-19.0742065683153,47.0764323013347,-25.));
#26550=CARTESIAN_POINT('Ctrl Pts',(-19.1123789307588,47.0610024423687,-25.));
#26551=CARTESIAN_POINT('Ctrl Pts',(-19.142800661846,47.0487055084058,-25.));
#26552=CARTESIAN_POINT('Ctrl Pts',(-19.1734565434277,47.0369399116326,-25.));
#26553=CARTESIAN_POINT('Ctrl Pts',(-19.2043343151472,47.0257029622097,-25.));
#26554=CARTESIAN_POINT('Ctrl Pts',(-20.7937992825329,47.0307770462543,-25.));
#26555=CARTESIAN_POINT('Ctrl Pts',(-20.8886442187745,47.065471747601,-25.));
#26556=CARTESIAN_POINT('Ctrl Pts',(-20.9814460889928,47.1051547823912,-25.));
#26557=CARTESIAN_POINT('Ctrl Pts',(-21.0719637631512,47.1495064254641,-25.));
#26558=CARTESIAN_POINT('Ctrl Pts',(-21.163746553324,47.1944779471897,-25.));
#26559=CARTESIAN_POINT('Ctrl Pts',(-21.253181519704,47.2442501915546,-25.));
#26560=CARTESIAN_POINT('Ctrl Pts',(-21.3399832517889,47.2985305082219,-25.));
#26561=CARTESIAN_POINT('Ctrl Pts',(-21.3644994122972,47.3138613653821,-25.));
#26562=CARTESIAN_POINT('Ctrl Pts',(-21.3888052755545,47.3295520482463,-25.));
#26563=CARTESIAN_POINT('Ctrl Pts',(-21.4128938145509,47.3455964190897,-25.));
#26564=CARTESIAN_POINT('Ctrl Pts',(-21.4322113128632,47.3584629987829,-25.));
#26565=CARTESIAN_POINT('Ctrl Pts',(-21.4513911411419,47.3715586534343,-25.));
#26566=CARTESIAN_POINT('Ctrl Pts',(-21.470410419303,47.3848664771592,-25.));
#26567=CARTESIAN_POINT('Ctrl Pts',(-21.5531190276758,47.4427378417522,-25.));
#26568=CARTESIAN_POINT('Ctrl Pts',(-21.6328730469962,47.5046694738537,-25.));
#26569=CARTESIAN_POINT('Ctrl Pts',(-21.7094059959913,47.5703647549773,-25.));
#26570=CARTESIAN_POINT('Ctrl Pts',(-21.7684006486615,47.6210053005573,-25.));
#26571=CARTESIAN_POINT('Ctrl Pts',(-21.8254807251055,47.6738830950808,-25.));
#26572=CARTESIAN_POINT('Ctrl Pts',(-21.880506602648,47.7288740485728,-25.));
#26573=CARTESIAN_POINT('Ctrl Pts',(-21.9097988741256,47.758147728711,-25.));
#26574=CARTESIAN_POINT('Ctrl Pts',(-21.9385087463308,47.7880203887706,-25.));
#26575=CARTESIAN_POINT('Ctrl Pts',(-21.9666131342303,47.8184741413986,-25.));
#26576=CARTESIAN_POINT('Ctrl Pts',(-21.9762497481644,47.8289163206757,-25.));
#26577=CARTESIAN_POINT('Ctrl Pts',(-21.9858144352345,47.8394261052524,-25.));
#26578=CARTESIAN_POINT('Ctrl Pts',(-21.9952996346009,47.8499951701003,-25.));
#26579=CARTESIAN_POINT('Ctrl Pts',(-22.0610978805005,47.9233121243291,-25.));
#26580=CARTESIAN_POINT('Ctrl Pts',(-22.1231640295475,47.999575563378,-25.));
#26581=CARTESIAN_POINT('Ctrl Pts',(-22.1812542057559,48.0785076415563,-25.));
#26582=CARTESIAN_POINT('Ctrl Pts',(-22.2388179901799,48.1567244663097,-25.));
#26583=CARTESIAN_POINT('Ctrl Pts',(-22.2924779669419,48.2375625681601,-25.));
#26584=CARTESIAN_POINT('Ctrl Pts',(-22.3419510864935,48.3207739812286,-25.));
#26585=CARTESIAN_POINT('Ctrl Pts',(-22.3900084462906,48.4016041543266,-25.));
#26586=CARTESIAN_POINT('Ctrl Pts',(-22.4341153568532,48.48467444732,-25.));
#26587=CARTESIAN_POINT('Ctrl Pts',(-22.4739645960461,48.5697679270184,-25.));
#26588=CARTESIAN_POINT('Ctrl Pts',(-22.4947696783231,48.6141947939351,-25.));
#26589=CARTESIAN_POINT('Ctrl Pts',(-22.514413373569,48.6591732571786,-25.));
#26590=CARTESIAN_POINT('Ctrl Pts',(-22.5328462651431,48.7046726841286,-25.));
#26591=CARTESIAN_POINT('Ctrl Pts',(-22.5399053146425,48.7220971183659,-25.));
#26592=CARTESIAN_POINT('Ctrl Pts',(-22.5467867474585,48.7395979548892,-25.));
#26593=CARTESIAN_POINT('Ctrl Pts',(-22.5534876260568,48.7571734646438,-25.));
#26594=CARTESIAN_POINT('Ctrl Pts',(-22.5587290601633,48.770921046385,-25.));
#26595=CARTESIAN_POINT('Ctrl Pts',(-22.5638601218329,48.7847148146814,-25.));
#26596=CARTESIAN_POINT('Ctrl Pts',(-22.5688742772034,48.7985392343856,-25.));
#26597=CARTESIAN_POINT('Ctrl Pts',(-22.6005567102338,48.8858901876576,-25.));
#26598=CARTESIAN_POINT('Ctrl Pts',(-22.6276303371176,48.9746044552164,-25.));
#26599=CARTESIAN_POINT('Ctrl Pts',(-22.6498438368096,49.064459151712,-25.));
#26600=CARTESIAN_POINT('Ctrl Pts',(-22.6548287054449,49.0846231900001,-25.));
#26601=CARTESIAN_POINT('Ctrl Pts',(-22.6595686217097,49.1048446984201,-25.));
#26602=CARTESIAN_POINT('Ctrl Pts',(-22.664060384471,49.1251212139915,-25.));
#26603=CARTESIAN_POINT('Ctrl Pts',(-22.6844252492069,49.2170513801367,-25.));
#26604=CARTESIAN_POINT('Ctrl Pts',(-22.699693338023,49.3101125654953,-25.));
#26605=CARTESIAN_POINT('Ctrl Pts',(-22.7099745886613,49.4039125916329,-25.));
#26606=CARTESIAN_POINT('Ctrl Pts',(-22.7207065136441,49.5018243028922,-25.));
#26607=CARTESIAN_POINT('Ctrl Pts',(-22.726004813639,49.6005422870379,-25.));
#26608=CARTESIAN_POINT('Ctrl Pts',(-22.7259370635773,49.6996058630434,-25.));
#26609=CARTESIAN_POINT('Ctrl Pts',(-22.7259105623628,49.7383557181929,-25.));
#26610=CARTESIAN_POINT('Ctrl Pts',(-22.7250624171289,49.777158194654,-25.));
#26611=CARTESIAN_POINT('Ctrl Pts',(-22.7233944482762,49.8159844929349,-25.));
#26612=CARTESIAN_POINT('Ctrl Pts',(-22.7228610319112,49.8284011414003,-25.));
#26613=CARTESIAN_POINT('Ctrl Pts',(-22.7222437741598,49.8408189143377,-25.));
#26614=CARTESIAN_POINT('Ctrl Pts',(-22.7215434366001,49.8532272016926,-25.));
#26615=CARTESIAN_POINT('Ctrl Pts',(-22.7163011026353,49.9461086776959,-25.));
#26616=CARTESIAN_POINT('Ctrl Pts',(-22.7064019888496,50.0386086524861,-25.));
#26617=CARTESIAN_POINT('Ctrl Pts',(-22.6919696691014,50.130354953021,-25.));
#26618=CARTESIAN_POINT('Ctrl Pts',(-22.6775715542487,50.221883812931,-25.));
#26619=CARTESIAN_POINT('Ctrl Pts',(-22.6586612853047,50.3126635132626,-25.));
#26620=CARTESIAN_POINT('Ctrl Pts',(-22.6353128834832,50.4023075767819,-25.));
#26621=CARTESIAN_POINT('Ctrl Pts',(-22.6123616726036,50.4904266618342,-25.));
#26622=CARTESIAN_POINT('Ctrl Pts',(-22.5851215750556,50.5774492051802,-25.));
#26623=CARTESIAN_POINT('Ctrl Pts',(-22.5536224664953,50.6629790188289,-25.));
#26624=CARTESIAN_POINT('Ctrl Pts',(-22.5377791649532,50.7059984784396,-25.));
#26625=CARTESIAN_POINT('Ctrl Pts',(-22.5208577985189,50.748639764913,-25.));
#26626=CARTESIAN_POINT('Ctrl Pts',(-22.5028587517058,50.7908486725183,-25.));
#26627=CARTESIAN_POINT('Ctrl Pts',(-22.4972963290681,50.8038929067832,-25.));
#26628=CARTESIAN_POINT('Ctrl Pts',(-22.4916309664074,50.8168958257194,-25.));
#26629=CARTESIAN_POINT('Ctrl Pts',(-22.4858626342927,50.8298557719296,-25.));
#26630=CARTESIAN_POINT('Ctrl Pts',(-22.4801786518254,50.8426262063587,-25.));
#26631=CARTESIAN_POINT('Ctrl Pts',(-22.4743981603631,50.8553470721618,-25.));
#26632=CARTESIAN_POINT('Ctrl Pts',(-22.4685229752345,50.8680138234556,-25.));
#26633=CARTESIAN_POINT('Ctrl Pts',(-22.4310412018688,50.9488235836377,-25.));
#26634=CARTESIAN_POINT('Ctrl Pts',(-22.3896896687866,51.0274761880601,-25.));
#26635=CARTESIAN_POINT('Ctrl Pts',(-22.3445381491691,51.1036235513123,-25.));
#26636=CARTESIAN_POINT('Ctrl Pts',(-22.3001458590794,51.1784904853093,-25.));
#26637=CARTESIAN_POINT('Ctrl Pts',(-22.2520798483092,51.2509363917474,-25.));
#26638=CARTESIAN_POINT('Ctrl Pts',(-22.2003702290622,51.320596267752,-25.));
#26639=CARTESIAN_POINT('Ctrl Pts',(-22.1502407921192,51.3881274237048,-25.));
#26640=CARTESIAN_POINT('Ctrl Pts',(-22.0966865895448,51.4530406640365,-25.));
#26641=CARTESIAN_POINT('Ctrl Pts',(-22.0397073639147,51.5149631456524,-25.));
#26642=CARTESIAN_POINT('Ctrl Pts',(-22.0187240959256,51.5377668256239,-25.));
#26643=CARTESIAN_POINT('Ctrl Pts',(-21.9972760930074,51.5601644736352,-25.));
#26644=CARTESIAN_POINT('Ctrl Pts',(-21.975362529417,51.5821358538774,-25.));
#26645=CARTESIAN_POINT('Ctrl Pts',(-21.9562846701964,51.6012640480396,-25.));
#26646=CARTESIAN_POINT('Ctrl Pts',(-21.9368539244304,51.6200691348985,-25.));
#26647=CARTESIAN_POINT('Ctrl Pts',(-21.9170804273993,51.6385459961512,-25.));
#26648=CARTESIAN_POINT('Origin',(-20.,50.,-42.2084234471774));
#26649=CARTESIAN_POINT('Ctrl Pts',(-16.9232550353076,50.0019104925463,-39.7084234471775));
#26650=CARTESIAN_POINT('Ctrl Pts',(-16.9223298998565,50.1251796275816,-39.7020198504182));
#26651=CARTESIAN_POINT('Ctrl Pts',(-16.9848354680816,51.261038906527,-39.642966745928));
#26652=CARTESIAN_POINT('Ctrl Pts',(-18.3975849010801,53.2535258762515,-39.5312641337071));
#26653=CARTESIAN_POINT('Ctrl Pts',(-21.848150909044,53.1200739456119,-39.3733156105146));
#26654=CARTESIAN_POINT('Ctrl Pts',(-23.6230224069675,50.158234898072,-39.2153670873222));
#26655=CARTESIAN_POINT('Ctrl Pts',(-22.1130258952668,47.0526834926192,-39.0574185641297));
#26656=CARTESIAN_POINT('Ctrl Pts',(-18.6872049245772,46.6194976592071,-38.8994700409372));
#26657=CARTESIAN_POINT('Ctrl Pts',(-17.0406885958919,48.5578258148839,-38.7831383352865));
#26658=CARTESIAN_POINT('Ctrl Pts',(-16.9238131547401,49.7844436293797,-38.7194561373665));
#26659=CARTESIAN_POINT('Ctrl Pts',(-16.9257449470869,49.9973154802779,-38.7084234471774));
#26660=CARTESIAN_POINT('Ctrl Pts',(-16.9296933173407,49.9966552073599,-39.7915765528225));
#26661=CARTESIAN_POINT('Ctrl Pts',(-16.9347030447108,50.6897748401454,-39.7557520197534));
#26662=CARTESIAN_POINT('Ctrl Pts',(-17.5071823782537,52.4114026146138,-39.6672779789534));
#26663=CARTESIAN_POINT('Ctrl Pts',(-20.3515248609294,53.6086146806686,-39.5261544304226));
#26664=CARTESIAN_POINT('Ctrl Pts',(-23.2138551423641,51.6798054402274,-39.3682059072301));
#26665=CARTESIAN_POINT('Ctrl Pts',(-23.1634851378897,48.2264371018949,-39.2102573840377));
#26666=CARTESIAN_POINT('Ctrl Pts',(-20.2442745178934,46.3818724340551,-39.0523088608451));
#26667=CARTESIAN_POINT('Ctrl Pts',(-17.4694924470354,47.6502488635873,-38.9127485837735));
#26668=CARTESIAN_POINT('Ctrl Pts',(-16.9339705689346,49.3389604585216,-38.8258378144326));
#26669=CARTESIAN_POINT('Ctrl Pts',(-16.9296185387977,50.0021495995983,-38.7915765528225));
#26670=CARTESIAN_POINT('Ctrl Pts',(-21.913465996665,51.635987203375,-40.));
#26671=CARTESIAN_POINT('Ctrl Pts',(-22.4546613829867,51.0029999971535,-39.9473504922692));
#26672=CARTESIAN_POINT('Ctrl Pts',(-22.8504293341544,49.1684270296901,-39.8420514768075));
#26673=CARTESIAN_POINT('Ctrl Pts',(-20.8590122687702,47.1546700385836,-39.6841029536151));
#26674=CARTESIAN_POINT('Ctrl Pts',(-18.0884177969373,47.7272058248279,-39.5261544304226));
#26675=CARTESIAN_POINT('Ctrl Pts',(-17.051198789188,50.3572343043579,-39.3682059072301));
#26676=CARTESIAN_POINT('Ctrl Pts',(-18.6874637997297,52.6649589697292,-39.2102573840377));
#26677=CARTESIAN_POINT('Ctrl Pts',(-21.5138180945235,52.5556486605102,-39.0523088608452));
#26678=CARTESIAN_POINT('Ctrl Pts',(-22.9676131151914,50.1296100067989,-38.8943603376527));
#26679=CARTESIAN_POINT('Ctrl Pts',(-21.7307768639447,47.5858567407415,-38.7364118144603));
#26680=CARTESIAN_POINT('Ctrl Pts',(-18.9246911981855,47.231034767221,-38.5784632912678));
#26681=CARTESIAN_POINT('Ctrl Pts',(-17.0935586692445,49.3866986229546,-38.4205147680753));
#26682=CARTESIAN_POINT('Ctrl Pts',(-17.897606416995,52.0984496625164,-38.2625662448829));
#26683=CARTESIAN_POINT('Ctrl Pts',(-20.6078313299859,52.90758741957,-38.1046177216903));
#26684=CARTESIAN_POINT('Ctrl Pts',(-22.7669536381063,51.0805105191678,-37.9466691984979));
#26685=CARTESIAN_POINT('Ctrl Pts',(-22.4173634487422,48.2737643663635,-37.7887206753054));
#26686=CARTESIAN_POINT('Ctrl Pts',(-19.8760232341734,47.032145182041,-37.630772152113));
#26687=CARTESIAN_POINT('Ctrl Pts',(-17.4470890363398,48.4813888841037,-37.4728236289205));
#26688=CARTESIAN_POINT('Ctrl Pts',(-17.3328015389901,51.3075115071856,-37.3148751057281));
#26689=CARTESIAN_POINT('Ctrl Pts',(-19.6367817806179,52.9481530076165,-37.1569265825355));
#26690=CARTESIAN_POINT('Ctrl Pts',(-22.2700809281698,51.9157939431384,-36.9989780593431));
#26691=CARTESIAN_POINT('Ctrl Pts',(-22.845166742959,49.146442724891,-36.8410295361506));
#26692=CARTESIAN_POINT('Ctrl Pts',(-20.8406264020256,47.1509859542099,-36.6830810129582));
#26693=CARTESIAN_POINT('Ctrl Pts',(-18.0739156697339,47.7386435569461,-36.5251324897657));
#26694=CARTESIAN_POINT('Ctrl Pts',(-17.0535270200547,50.3766042771083,-36.3671839665732));
#26695=CARTESIAN_POINT('Ctrl Pts',(-18.7046158085844,52.6731093498251,-36.2092354433807));
#26696=CARTESIAN_POINT('Ctrl Pts',(-21.5301900460322,52.5459874756549,-36.0512869201883));
#26697=CARTESIAN_POINT('Ctrl Pts',(-22.9683875074239,50.1104961891868,-35.8933383969958));
#26698=CARTESIAN_POINT('Ctrl Pts',(-21.7152382952319,47.5748213689897,-35.7353898738034));
#26699=CARTESIAN_POINT('Ctrl Pts',(-18.9069346873816,47.2379822548464,-35.5774413506109));
#26700=CARTESIAN_POINT('Ctrl Pts',(-17.0896801543967,49.4053806273666,-35.4194928274185));
#26701=CARTESIAN_POINT('Ctrl Pts',(-17.9111241120468,52.1119023004698,-35.2615443042259));
#26702=CARTESIAN_POINT('Ctrl Pts',(-20.626488307014,52.9036263883688,-35.1035957810335));
#26703=CARTESIAN_POINT('Ctrl Pts',(-22.7738346077931,51.062720739725,-34.945647257841));
#26704=CARTESIAN_POINT('Ctrl Pts',(-22.4062294320517,48.2582785175696,-34.7876987346486));
#26705=CARTESIAN_POINT('Ctrl Pts',(-19.8569692124294,47.033002191466,-34.6297502114561));
#26706=CARTESIAN_POINT('Ctrl Pts',(-17.4373906578124,48.4978125412028,-34.4718016882636));
#26707=CARTESIAN_POINT('Ctrl Pts',(-17.341252055517,51.3246105728636,-34.3138531650711));
#26708=CARTESIAN_POINT('Ctrl Pts',(-19.6557193523207,52.9504244843191,-34.1559046418787));
#26709=CARTESIAN_POINT('Ctrl Pts',(-22.2823354415527,51.9011782489466,-33.9979561186862));
#26710=CARTESIAN_POINT('Ctrl Pts',(-22.8396274000236,49.128191516977,-33.8400075954937));
#26711=CARTESIAN_POINT('Ctrl Pts',(-20.8223155582564,47.1456470217079,-33.6820590723012));
#26712=CARTESIAN_POINT('Ctrl Pts',(-18.0594352094154,47.7510575606347,-33.5241105491088));
#26713=CARTESIAN_POINT('Ctrl Pts',(-17.0560059365872,50.3955158108414,-33.3661620259163));
#26714=CARTESIAN_POINT('Ctrl Pts',(-18.7218065435234,52.681371904428,-33.2082135027239));
#26715=CARTESIAN_POINT('Ctrl Pts',(-21.5465062829502,52.5361096425097,-33.0502649795314));
#26716=CARTESIAN_POINT('Ctrl Pts',(-22.9690358104885,50.091433900016,-32.8923164563389));
#26717=CARTESIAN_POINT('Ctrl Pts',(-21.6996308677992,47.5638578212141,-32.7343679331465));
#26718=CARTESIAN_POINT('Ctrl Pts',(-18.8892223092125,47.2450577640023,-32.576419409954));
#26719=CARTESIAN_POINT('Ctrl Pts',(-17.0859221000865,49.424080044389,-32.4184708867615));
#26720=CARTESIAN_POINT('Ctrl Pts',(-17.924727695139,52.1252714327145,-32.2605223635691));
#26721=CARTESIAN_POINT('Ctrl Pts',(-20.645119572455,52.8995438502066,-32.1025738403766));
#26722=CARTESIAN_POINT('Ctrl Pts',(-22.7806011538509,51.0448880443562,-31.9446253171841));
#26723=CARTESIAN_POINT('Ctrl Pts',(-22.3949962372115,48.2428640275214,-31.7866767939916));
#26724=CARTESIAN_POINT('Ctrl Pts',(-19.8379210728103,47.033981756058,-31.6287282707992));
#26725=CARTESIAN_POINT('Ctrl Pts',(-17.4277979422843,48.5142980190097,-31.4707797476067));
#26726=CARTESIAN_POINT('Ctrl Pts',(-17.3498121874998,51.341655082542,-31.3128312244142));
#26727=CARTESIAN_POINT('Ctrl Pts',(-19.6746711204904,52.9525742873284,-31.1548827012218));
#26728=CARTESIAN_POINT('Ctrl Pts',(-22.2944958541018,51.8864841842817,-30.9969341780293));
#26729=CARTESIAN_POINT('Ctrl Pts',(-22.8339709807359,49.1099762461699,-30.8389856548368));
#26730=CARTESIAN_POINT('Ctrl Pts',(-20.8039708104681,47.1404257768069,-30.6810371316443));
#26731=CARTESIAN_POINT('Ctrl Pts',(-18.0450347580157,47.7635642855944,-30.5230886084519));
#26732=CARTESIAN_POINT('Ctrl Pts',(-17.0586062328904,50.4144110385161,-30.3651400852594));
#26733=CARTESIAN_POINT('Ctrl Pts',(-18.7390499779557,52.6895239065569,-30.207191562067));
#26734=CARTESIAN_POINT('Ctrl Pts',(-21.5627587579476,52.5261272466952,-30.0492430388745));
#26735=CARTESIAN_POINT('Ctrl Pts',(-22.9695617012666,50.072367840941,-29.891294515682));
#26736=CARTESIAN_POINT('Ctrl Pts',(-21.6839533651858,47.5529947147765,-29.7333459924895));
#26737=CARTESIAN_POINT('Ctrl Pts',(-18.8715557280134,47.2522468584174,-29.5753974692971));
#26738=CARTESIAN_POINT('Ctrl Pts',(-17.0822841921784,49.4428032064075,-29.4174489461046));
#26739=CARTESIAN_POINT('Ctrl Pts',(-17.9384168409638,52.1385529407526,-29.2595004229121));
#26740=CARTESIAN_POINT('Ctrl Pts',(-20.6637242398626,52.8953417649065,-29.1015518997197));
#26741=CARTESIAN_POINT('Ctrl Pts',(-22.787253056673,51.0270122685761,-28.9436033765272));
#26742=CARTESIAN_POINT('Ctrl Pts',(-22.3836642975977,48.2275219836588,-28.7856548533347));
#26743=CARTESIAN_POINT('Ctrl Pts',(-19.8188796155043,47.0350836083479,-28.6277063301423));
#26744=CARTESIAN_POINT('Ctrl Pts',(-17.4183112780211,48.5308447521454,-28.4697578069498));
#26745=CARTESIAN_POINT('Ctrl Pts',(-17.3584815852165,51.3586442755348,-28.3118092837573));
#26746=CARTESIAN_POINT('Ctrl Pts',(-19.6936363029893,52.9546023581848,-28.1538607605649));
#26747=CARTESIAN_POINT('Ctrl Pts',(-22.3065616631405,51.8717123376796,-27.9959122373724));
#26748=CARTESIAN_POINT('Ctrl Pts',(-22.8281977223296,49.0917976764282,-27.8379637141799));
#26749=CARTESIAN_POINT('Ctrl Pts',(-20.785592906288,47.1353224197833,-27.6800151909875));
#26750=CARTESIAN_POINT('Ctrl Pts',(-18.0307149269819,47.7761632406137,-27.522066667795));
#26751=CARTESIAN_POINT('Ctrl Pts',(-17.0613277662871,50.4332891351524,-27.3641181446025));
#26752=CARTESIAN_POINT('Ctrl Pts',(-18.7563454716562,52.6975651102113,-27.2061696214101));
#26753=CARTESIAN_POINT('Ctrl Pts',(-21.5789466600823,52.5160405210495,-27.0482210982176));
#26754=CARTESIAN_POINT('Ctrl Pts',(-22.9699654385827,50.0532991536051,-26.8902725750251));
#26755=CARTESIAN_POINT('Ctrl Pts',(-21.6682058751988,47.5422317897299,-26.7323240518326));
#26756=CARTESIAN_POINT('Ctrl Pts',(-18.853936784431,47.2595506510657,-26.5743755286402));
#26757=CARTESIAN_POINT('Ctrl Pts',(-17.0787643658711,49.4615465350924,-26.4164270054477));
#26758=CARTESIAN_POINT('Ctrl Pts',(-17.9521953953268,52.151751865176,-26.2584784822553));
#26759=CARTESIAN_POINT('Ctrl Pts',(-20.682292760352,52.8910091782576,-26.1005299590628));
#26760=CARTESIAN_POINT('Ctrl Pts',(-22.7938075288087,51.0091163069545,-25.9425814358703));
#26761=CARTESIAN_POINT('Ctrl Pts',(-22.3721992598072,48.2122088972454,-25.7846329126778));
#26762=CARTESIAN_POINT('Ctrl Pts',(-19.7999149622792,47.0363955599718,-25.6266843894854));
#26763=CARTESIAN_POINT('Ctrl Pts',(-17.4087929877025,48.5472771059899,-25.4687358662929));
#26764=CARTESIAN_POINT('Ctrl Pts',(-17.3675348421714,51.3759259143989,-25.3107873431005));
#26765=CARTESIAN_POINT('Ctrl Pts',(-19.7120663404711,52.9558136087163,-25.1528388199079));
#26766=CARTESIAN_POINT('Ctrl Pts',(-22.3196266734264,51.8582617585154,-24.9948902967155));
#26767=CARTESIAN_POINT('Ctrl Pts',(-22.8200818112517,49.0706994179464,-24.836941773523));
#26768=CARTESIAN_POINT('Ctrl Pts',(-21.4547503964622,47.7830036573307,-24.7316427580614));
#26769=CARTESIAN_POINT('Ctrl Pts',(-20.6501999979751,47.5679131979649,-24.6789932503306));
#26770=CARTESIAN_POINT('Ctrl Pts',(-22.0543315503421,51.7564253212269,-40.1070022498898));
#26771=CARTESIAN_POINT('Ctrl Pts',(-22.6353686625551,51.0768388582481,-40.054352742159));
#26772=CARTESIAN_POINT('Ctrl Pts',(-23.060272261634,49.107208284706,-39.9490537266973));
#26773=CARTESIAN_POINT('Ctrl Pts',(-20.9222510402281,46.9452025167633,-39.7911052035049));
#26774=CARTESIAN_POINT('Ctrl Pts',(-17.9476909243915,47.5598872466888,-39.6331566803124));
#26775=CARTESIAN_POINT('Ctrl Pts',(-16.8341139201763,50.3835331819777,-39.47520815712));
#26776=CARTESIAN_POINT('Ctrl Pts',(-18.5908375001798,52.86114793857,-39.3172596339274));
#26777=CARTESIAN_POINT('Ctrl Pts',(-21.6252623660303,52.7437904222108,-39.159311110735));
#26778=CARTESIAN_POINT('Ctrl Pts',(-23.1860828791167,50.1391516372232,-39.0013625875425));
#26779=CARTESIAN_POINT('Ctrl Pts',(-21.8581932077187,47.4081323247007,-38.84341406435));
#26780=CARTESIAN_POINT('Ctrl Pts',(-18.8455291069827,47.0271890645498,-38.6854655411576));
#26781=CARTESIAN_POINT('Ctrl Pts',(-16.8795922501912,49.341548597713,-38.5275170179651));
#26782=CARTESIAN_POINT('Ctrl Pts',(-17.742832390891,52.2529333450532,-38.3695684947727));
#26783=CARTESIAN_POINT('Ctrl Pts',(-20.6525786612632,53.121638211398,-38.2116199715802));
#26784=CARTESIAN_POINT('Ctrl Pts',(-22.9706512511864,51.1600555504364,-38.0536714483877));
#26785=CARTESIAN_POINT('Ctrl Pts',(-22.5953249287157,48.1466823389155,-37.8957229251952));
#26786=CARTESIAN_POINT('Ctrl Pts',(-19.866896311724,46.8136576244393,-37.7377744020028));
#26787=CARTESIAN_POINT('Ctrl Pts',(-17.2591488184259,48.3695917599147,-37.5798258788103));
#26788=CARTESIAN_POINT('Ctrl Pts',(-17.136447703264,51.4037678988433,-37.4218773556179));
#26789=CARTESIAN_POINT('Ctrl Pts',(-19.6100423790983,53.1651901572008,-37.2639288324253));
#26790=CARTESIAN_POINT('Ctrl Pts',(-22.4371997624713,52.0568308755958,-37.1059803092329));
#26791=CARTESIAN_POINT('Ctrl Pts',(-23.0546222489617,49.0836055391962,-36.9480317860404));
#26792=CARTESIAN_POINT('Ctrl Pts',(-20.9025116426116,46.9412472174394,-36.790083262848));
#26793=CARTESIAN_POINT('Ctrl Pts',(-17.932121179482,47.5721670018534,-36.6321347396555));
#26794=CARTESIAN_POINT('Ctrl Pts',(-16.8366135507598,50.4043291335231,-36.4741862164631));
#26795=CARTESIAN_POINT('Ctrl Pts',(-18.6092522057474,52.8698983334071,-36.3162376932705));
#26796=CARTESIAN_POINT('Ctrl Pts',(-21.6428395879844,52.7334180001784,-36.1582891700781));
#26797=CARTESIAN_POINT('Ctrl Pts',(-23.1869142805623,50.118630698447,-36.0003406468856));
#26798=CARTESIAN_POINT('Ctrl Pts',(-21.8415107205413,47.396284550871,-35.8423921236932));
#26799=CARTESIAN_POINT('Ctrl Pts',(-18.8264653972371,47.0346480123697,-35.6844436005007));
#26800=CARTESIAN_POINT('Ctrl Pts',(-16.8754282068091,49.3616059340618,-35.5264950773083));
#26801=CARTESIAN_POINT('Ctrl Pts',(-17.7573452317156,52.2673763394054,-35.3685465541157));
#26802=CARTESIAN_POINT('Ctrl Pts',(-20.6726091277621,53.117385576973,-35.2105980309233));
#26803=CARTESIAN_POINT('Ctrl Pts',(-22.9780387841496,51.1409561228812,-35.0526495077308));
#26804=CARTESIAN_POINT('Ctrl Pts',(-22.5833712479035,48.1300564527922,-34.8947009845384));
#26805=CARTESIAN_POINT('Ctrl Pts',(-19.8464395708685,46.8145777251907,-34.7367524613459));
#26806=CARTESIAN_POINT('Ctrl Pts',(-17.2487364645975,48.3872244939215,-34.5788039381534));
#26807=CARTESIAN_POINT('Ctrl Pts',(-17.145520329978,51.422125763663,-34.4208554149609));
#26808=CARTESIAN_POINT('Ctrl Pts',(-19.6303740970927,53.1676288554917,-34.2629068917685));
#26809=CARTESIAN_POINT('Ctrl Pts',(-22.4503564287097,52.0411392031225,-34.104958368576));
#26810=CARTESIAN_POINT('Ctrl Pts',(-23.0486751106377,49.0640107137251,-33.9470098453835));
#26811=CARTESIAN_POINT('Ctrl Pts',(-20.8828527910125,46.9355152433656,-33.7890613221911));
#26812=CARTESIAN_POINT('Ctrl Pts',(-17.9165746965303,47.5854948997559,-33.6311127989986));
#26813=CARTESIAN_POINT('Ctrl Pts',(-16.8392749601877,50.4246328966843,-33.4731642758061));
#26814=CARTESIAN_POINT('Ctrl Pts',(-18.6277084883363,52.8787691608149,-33.3152157526137));
#26815=CARTESIAN_POINT('Ctrl Pts',(-21.6603569937506,52.7228129806409,-33.1572672294212));
#26816=CARTESIAN_POINT('Ctrl Pts',(-23.1876103104067,50.0981650815332,-32.9993187062287));
#26817=CARTESIAN_POINT('Ctrl Pts',(-21.8247543054021,47.3845138885554,-32.8413701830363));
#26818=CARTESIAN_POINT('Ctrl Pts',(-18.807449069083,47.0422444064101,-32.6834216598438));
#26819=CARTESIAN_POINT('Ctrl Pts',(-16.8713934920293,49.3816819649028,-32.5254731366513));
#26820=CARTESIAN_POINT('Ctrl Pts',(-17.7719502834869,52.2817296805251,-32.3675246134588));
#26821=CARTESIAN_POINT('Ctrl Pts',(-20.692611989838,53.1130024904866,-32.2095760902664));
#26822=CARTESIAN_POINT('Ctrl Pts',(-22.9853034698444,51.1218106200149,-32.0516275670739));
#26823=CARTESIAN_POINT('Ctrl Pts',(-22.5713110876437,48.1135071787034,-31.8936790438815));
#26824=CARTESIAN_POINT('Ctrl Pts',(-19.8259891451682,46.815629403376,-31.7357305206889));
#26825=CARTESIAN_POINT('Ctrl Pts',(-17.2384375524677,48.4049235997537,-31.5777819974966));
#26826=CARTESIAN_POINT('Ctrl Pts',(-17.1547106418195,51.440425056179,-31.419833474304));
#26827=CARTESIAN_POINT('Ctrl Pts',(-19.6507210566695,53.1699369227146,-31.2618849511116));
#26828=CARTESIAN_POINT('Ctrl Pts',(-22.4634120665983,52.0253633906983,-31.1039364279191));
#26829=CARTESIAN_POINT('Ctrl Pts',(-23.0426022770338,49.0444544709788,-30.9459879047267));
#26830=CARTESIAN_POINT('Ctrl Pts',(-20.8631575394479,46.9299096208195,-30.7880393815342));
#26831=CARTESIAN_POINT('Ctrl Pts',(-17.9011141125945,47.5989223448847,-30.6300908583417));
#26832=CARTESIAN_POINT('Ctrl Pts',(-16.8420666851231,50.4449191533675,-30.4721423351493));
#26833=CARTESIAN_POINT('Ctrl Pts',(-18.6462213500501,52.8875212970958,-30.3141938119568));
#26834=CARTESIAN_POINT('Ctrl Pts',(-21.6778059435708,52.7120957007386,-30.1562452887643));
#26835=CARTESIAN_POINT('Ctrl Pts',(-23.1881749162158,50.0776954171824,-29.9982967655718));
#26836=CARTESIAN_POINT('Ctrl Pts',(-21.8079226562872,47.372851061869,-29.8403482423794));
#26837=CARTESIAN_POINT('Ctrl Pts',(-18.7884819093805,47.0499627476302,-29.6823997191869));
#26838=CARTESIAN_POINT('Ctrl Pts',(-16.8674877685903,49.4017834887991,-29.5244511959944));
#26839=CARTESIAN_POINT('Ctrl Pts',(-17.7866471969486,52.2959889467186,-29.366502672802));
#26840=CARTESIAN_POINT('Ctrl Pts',(-20.7125862957864,53.1084910560403,-29.2085541496095));
#26841=CARTESIAN_POINT('Ctrl Pts',(-22.9924450724969,51.1026188652432,-29.050605626417));
#26842=CARTESIAN_POINT('Ctrl Pts',(-22.559144913217,48.0970356841439,-28.8926571032246));
#26843=CARTESIAN_POINT('Ctrl Pts',(-19.8055458937194,46.8168123718357,-28.7347085800321));
#26844=CARTESIAN_POINT('Ctrl Pts',(-17.2282524988857,48.4226884704099,-28.5767600568396));
#26845=CARTESIAN_POINT('Ctrl Pts',(-17.1640182633205,51.4586649597053,-28.4188115336471));
#26846=CARTESIAN_POINT('Ctrl Pts',(-19.6710824181117,53.1721142961061,-28.2608630104547));
#26847=CARTESIAN_POINT('Ctrl Pts',(-22.4763661364548,52.0095040701854,-28.1029144872622));
#26848=CARTESIAN_POINT('Ctrl Pts',(-23.036404002848,49.0249376311576,-27.9449659640697));
#26849=CARTESIAN_POINT('Ctrl Pts',(-20.843426690584,46.9244305648213,-27.7870174408773));
#26850=CARTESIAN_POINT('Ctrl Pts',(-17.8857400841354,47.6124488098665,-27.6290689176848));
#26851=CARTESIAN_POINT('Ctrl Pts',(-16.8449885723852,50.4651870178593,-27.4711203944923));
#26852=CARTESIAN_POINT('Ctrl Pts',(-18.6647901035319,52.8961544781396,-27.3131718712999));
#26853=CARTESIAN_POINT('Ctrl Pts',(-21.6951855668027,52.7012664104508,-27.1552233481074));
#26854=CARTESIAN_POINT('Ctrl Pts',(-23.1886083758687,50.0572229310833,-26.9972748249149));
#26855=CARTESIAN_POINT('Ctrl Pts',(-21.7910158674676,47.3612957917279,-26.8393263017225));
#26856=CARTESIAN_POINT('Ctrl Pts',(-18.7695658942812,47.057804230939,-26.68137777853));
#26857=CARTESIAN_POINT('Ctrl Pts',(-16.8637088196843,49.4219066639916,-26.5234292553375));
#26858=CARTESIAN_POINT('Ctrl Pts',(-17.8014401010271,52.3101595496564,-26.3654807321451));
#26859=CARTESIAN_POINT('Ctrl Pts',(-20.7325217937523,53.1038395129959,-26.2075322089526));
#26860=CARTESIAN_POINT('Ctrl Pts',(-22.9994820718101,51.0834054385887,-26.0495836857601));
#26861=CARTESIAN_POINT('Ctrl Pts',(-22.5468358421909,48.0805952788235,-25.8916351625677));
#26862=CARTESIAN_POINT('Ctrl Pts',(-19.7851851005152,46.8182209067238,-25.7336866393752));
#26863=CARTESIAN_POINT('Ctrl Pts',(-17.2180334910011,48.4403305413994,-25.5757381161827));
#26864=CARTESIAN_POINT('Ctrl Pts',(-17.1737380030118,51.4772188383851,-25.4177895929903));
#26865=CARTESIAN_POINT('Ctrl Pts',(-19.6908692382271,53.173414716488,-25.2598410697978));
#26866=CARTESIAN_POINT('Ctrl Pts',(-22.4903929667631,51.9950632861863,-25.1018925466053));
#26867=CARTESIAN_POINT('Ctrl Pts',(-23.0276906145693,49.0022861609293,-24.9439440234128));
#26868=CARTESIAN_POINT('Ctrl Pts',(-21.561846221743,47.6197928044311,-24.8386450079512));
#26869=CARTESIAN_POINT('Ctrl Pts',(-20.698066426161,47.3888678140614,-24.7859955002204));
#26870=CARTESIAN_POINT('Ctrl Pts',(-22.1951971040191,51.8768634390788,-40.2140044997796));
#26871=CARTESIAN_POINT('Ctrl Pts',(-22.8160759421236,51.1506777193428,-40.1613549920488));
#26872=CARTESIAN_POINT('Ctrl Pts',(-23.2701151891136,49.0459895397219,-40.0560559765872));
#26873=CARTESIAN_POINT('Ctrl Pts',(-20.9854898116861,46.735734994943,-39.8981074533947));
#26874=CARTESIAN_POINT('Ctrl Pts',(-17.8069640518455,47.3925686685497,-39.7401589302022));
#26875=CARTESIAN_POINT('Ctrl Pts',(-16.6170290511645,50.4098320595973,-39.5822104070097));
#26876=CARTESIAN_POINT('Ctrl Pts',(-18.49421120063,53.0573369074108,-39.4242618838173));
#26877=CARTESIAN_POINT('Ctrl Pts',(-21.7367066375372,52.9319321839113,-39.2663133606248));
#26878=CARTESIAN_POINT('Ctrl Pts',(-23.4045526430421,50.1486932676477,-39.1083648374323));
#26879=CARTESIAN_POINT('Ctrl Pts',(-21.9856095514927,47.2304079086599,-38.9504163142399));
#26880=CARTESIAN_POINT('Ctrl Pts',(-18.76636701578,46.8233433618784,-38.7924677910474));
#26881=CARTESIAN_POINT('Ctrl Pts',(-16.6656258311379,49.2963985724715,-38.6345192678549));
#26882=CARTESIAN_POINT('Ctrl Pts',(-17.5880583647869,52.4074170275899,-38.4765707446625));
#26883=CARTESIAN_POINT('Ctrl Pts',(-20.6973259925406,53.3356890032261,-38.31862222147));
#26884=CARTESIAN_POINT('Ctrl Pts',(-23.1743488642664,51.2396005817052,-38.1606736982775));
#26885=CARTESIAN_POINT('Ctrl Pts',(-22.7732864086894,48.0196003114673,-38.002725175085));
#26886=CARTESIAN_POINT('Ctrl Pts',(-19.8577693892745,46.5951700668379,-37.8447766518926));
#26887=CARTESIAN_POINT('Ctrl Pts',(-17.0712086005119,48.2577946357256,-37.6868281287001));
#26888=CARTESIAN_POINT('Ctrl Pts',(-16.9400938675379,51.500024290501,-37.5288796055076));
#26889=CARTESIAN_POINT('Ctrl Pts',(-19.5833029775787,53.382227306785,-37.3709310823152));
#26890=CARTESIAN_POINT('Ctrl Pts',(-22.6043185967729,52.1978678080534,-37.2129825591227));
#26891=CARTESIAN_POINT('Ctrl Pts',(-23.2640777549644,49.0207683535012,-37.0550340359303));
#26892=CARTESIAN_POINT('Ctrl Pts',(-20.9643968831977,46.731508480669,-36.8970855127378));
#26893=CARTESIAN_POINT('Ctrl Pts',(-17.79032668923,47.4056904467606,-36.7391369895453));
#26894=CARTESIAN_POINT('Ctrl Pts',(-16.619700081465,50.4320539899379,-36.5811884663528));
#26895=CARTESIAN_POINT('Ctrl Pts',(-18.5138886029103,53.066687316989,-36.4232399431604));
#26896=CARTESIAN_POINT('Ctrl Pts',(-21.7554891299366,52.920848524702,-36.2652914199679));
#26897=CARTESIAN_POINT('Ctrl Pts',(-23.4054410537007,50.1267652077072,-36.1073428967755));
#26898=CARTESIAN_POINT('Ctrl Pts',(-21.9677831458506,47.2177477327522,-35.949394373583));
#26899=CARTESIAN_POINT('Ctrl Pts',(-18.7459961070927,46.831313769893,-35.7914458503905));
#26900=CARTESIAN_POINT('Ctrl Pts',(-16.6611762592215,49.317831240757,-35.6334973271981));
#26901=CARTESIAN_POINT('Ctrl Pts',(-17.6035663513843,52.4228503783411,-35.4755488040055));
#26902=CARTESIAN_POINT('Ctrl Pts',(-20.7187299485102,53.3311447655771,-35.3176002808131));
#26903=CARTESIAN_POINT('Ctrl Pts',(-23.1822429605062,51.2191915060373,-35.1596517576206));
#26904=CARTESIAN_POINT('Ctrl Pts',(-22.7605130637554,48.0018343880148,-35.0017032344282));
#26905=CARTESIAN_POINT('Ctrl Pts',(-19.8359099293075,46.5961532589153,-34.8437547112357));
#26906=CARTESIAN_POINT('Ctrl Pts',(-17.0600822713825,48.2766364466403,-34.6858061880432));
#26907=CARTESIAN_POINT('Ctrl Pts',(-16.9497886044391,51.5196409544624,-34.5278576648508));
#26908=CARTESIAN_POINT('Ctrl Pts',(-19.6050288418647,53.3848332266643,-34.3699091416583));
#26909=CARTESIAN_POINT('Ctrl Pts',(-22.6183774158668,52.1811001572986,-34.2119606184659));
#26910=CARTESIAN_POINT('Ctrl Pts',(-23.2577228212518,48.9998299104731,-34.0540120952733));
#26911=CARTESIAN_POINT('Ctrl Pts',(-20.9433900237686,46.7253834650232,-33.8960635720809));
#26912=CARTESIAN_POINT('Ctrl Pts',(-17.7737141836451,47.419932238877,-33.7381150488884));
#26913=CARTESIAN_POINT('Ctrl Pts',(-16.6225439837881,50.4537499825271,-33.580166525696));
#26914=CARTESIAN_POINT('Ctrl Pts',(-18.5336104331491,53.0761664172017,-33.4222180025035));
#26915=CARTESIAN_POINT('Ctrl Pts',(-21.7742077045511,52.909516318772,-33.264269479311));
#26916=CARTESIAN_POINT('Ctrl Pts',(-23.4061848103248,50.1048962630504,-33.1063209561185));
#26917=CARTESIAN_POINT('Ctrl Pts',(-21.9498777430051,47.2051699558967,-32.9483724329261));
#26918=CARTESIAN_POINT('Ctrl Pts',(-18.7256758289536,46.8394310488179,-32.7904239097336));
#26919=CARTESIAN_POINT('Ctrl Pts',(-16.6568648839721,49.3392838854165,-32.6324753865411));
#26920=CARTESIAN_POINT('Ctrl Pts',(-17.6191728718348,52.4381879283357,-32.4745268633487));
#26921=CARTESIAN_POINT('Ctrl Pts',(-20.7401044072209,53.3264611307666,-32.3165783401562));
#26922=CARTESIAN_POINT('Ctrl Pts',(-23.1900057858379,51.1987331956736,-32.1586298169638));
#26923=CARTESIAN_POINT('Ctrl Pts',(-22.747625938076,47.9841503298854,-32.0006812937712));
#26924=CARTESIAN_POINT('Ctrl Pts',(-19.814057217526,46.5972770506939,-31.8427327705788));
#26925=CARTESIAN_POINT('Ctrl Pts',(-17.0490771626511,48.2955491804977,-31.6847842473863));
#26926=CARTESIAN_POINT('Ctrl Pts',(-16.9596090961393,51.539195029816,-31.5268357241939));
#26927=CARTESIAN_POINT('Ctrl Pts',(-19.6267709928486,53.3872995581008,-31.3688872010014));
#26928=CARTESIAN_POINT('Ctrl Pts',(-22.6323282790949,52.1642425971148,-31.2109386778089));
#26929=CARTESIAN_POINT('Ctrl Pts',(-23.2512335733316,48.9789326957879,-31.0529901546164));
#26930=CARTESIAN_POINT('Ctrl Pts',(-20.9223442684278,46.719393464832,-30.895041631424));
#26931=CARTESIAN_POINT('Ctrl Pts',(-17.7571934671733,47.4342804041751,-30.7370931082315));
#26932=CARTESIAN_POINT('Ctrl Pts',(-16.6255271373557,50.4754272682189,-30.5791445850391));
#26933=CARTESIAN_POINT('Ctrl Pts',(-18.5533927221445,53.0855186876348,-30.4211960618465));
#26934=CARTESIAN_POINT('Ctrl Pts',(-21.7928531291939,52.898064154782,-30.2632475386541));
#26935=CARTESIAN_POINT('Ctrl Pts',(-23.4067881311651,50.0830229934237,-30.1052990154616));
#26936=CARTESIAN_POINT('Ctrl Pts',(-21.9318919473886,47.1927074089615,-29.9473504922692));
#26937=CARTESIAN_POINT('Ctrl Pts',(-18.7054080907476,46.8476786368431,-29.7894019690767));
#26938=CARTESIAN_POINT('Ctrl Pts',(-16.6526913450023,49.3607637711907,-29.6314534458842));
#26939=CARTESIAN_POINT('Ctrl Pts',(-17.6348775529335,52.4534249526847,-29.4735049226918));
#26940=CARTESIAN_POINT('Ctrl Pts',(-20.76144835171,53.3216403471741,-29.3155563994993));
#26941=CARTESIAN_POINT('Ctrl Pts',(-23.1976370883209,51.1782254619103,-29.1576078763068));
#26942=CARTESIAN_POINT('Ctrl Pts',(-22.7346255288362,47.9665493846291,-28.9996593531144));
#26943=CARTESIAN_POINT('Ctrl Pts',(-19.7922121719347,46.5985411353234,-28.8417108299219));
#26944=CARTESIAN_POINT('Ctrl Pts',(-17.0381937197502,48.3145321886744,-28.6837623067294));
#26945=CARTESIAN_POINT('Ctrl Pts',(-16.9695549414245,51.5586856438757,-28.525813783537));
#26946=CARTESIAN_POINT('Ctrl Pts',(-19.6485285332341,53.3896262340275,-28.3678652603445));
#26947=CARTESIAN_POINT('Ctrl Pts',(-22.6461706097691,52.1472958026912,-28.209916737152));
#26948=CARTESIAN_POINT('Ctrl Pts',(-23.2446102833664,48.9580775858871,-28.0519682139595));
#26949=CARTESIAN_POINT('Ctrl Pts',(-20.9012604748801,46.7135387098593,-27.8940196907671));
#26950=CARTESIAN_POINT('Ctrl Pts',(-17.7407652412889,47.4487343791192,-27.7360711675746));
#26951=CARTESIAN_POINT('Ctrl Pts',(-16.6286493784833,50.4970849005663,-27.5781226443822));
#26952=CARTESIAN_POINT('Ctrl Pts',(-18.5732347354075,53.0947438460678,-27.4201741211897));
#26953=CARTESIAN_POINT('Ctrl Pts',(-21.8114244735231,52.8864922998521,-27.2622255979972));
#26954=CARTESIAN_POINT('Ctrl Pts',(-23.4072513131546,50.0611467085616,-27.1042770748048));
#26955=CARTESIAN_POINT('Ctrl Pts',(-21.9138258597365,47.1803597937259,-26.9463285516123));
#26956=CARTESIAN_POINT('Ctrl Pts',(-18.6851950041314,46.8560578108122,-26.7883800284198));
#26957=CARTESIAN_POINT('Ctrl Pts',(-16.6486532734975,49.3822667928909,-26.6304315052273));
#26958=CARTESIAN_POINT('Ctrl Pts',(-17.6506848067274,52.4685672341367,-26.4724829820349));
#26959=CARTESIAN_POINT('Ctrl Pts',(-20.7827508271526,53.3166698477343,-26.3145344588424));
#26960=CARTESIAN_POINT('Ctrl Pts',(-23.2051566148114,51.1576945702228,-26.1565859356499));
#26961=CARTESIAN_POINT('Ctrl Pts',(-22.7214724245746,47.9489816604016,-25.9986374124575));
#26962=CARTESIAN_POINT('Ctrl Pts',(-19.7704552387511,46.6000462534758,-25.840688889265));
#26963=CARTESIAN_POINT('Ctrl Pts',(-17.0272739942997,48.3333839768089,-25.6827403660725));
#26964=CARTESIAN_POINT('Ctrl Pts',(-16.9799411638522,51.5785117623713,-25.5247918428801));
#26965=CARTESIAN_POINT('Ctrl Pts',(-19.6696721359831,53.3910158242598,-25.3668433196876));
#26966=CARTESIAN_POINT('Ctrl Pts',(-22.6611592600998,52.1318648138572,-25.2088947964951));
#26967=CARTESIAN_POINT('Ctrl Pts',(-23.2352994178868,48.9338729039122,-25.0509462733027));
#26968=CARTESIAN_POINT('Ctrl Pts',(-21.6689420470237,47.4565819515315,-24.945647257841));
#26969=CARTESIAN_POINT('Ctrl Pts',(-20.7459328543469,47.2098224301578,-24.8929977501102));
#26970=CARTESIAN_POINT('Ctrl Pts',(-22.3360626576961,51.9973015569307,-40.3210067496694));
#26971=CARTESIAN_POINT('Ctrl Pts',(-22.996783221692,51.2245165804374,-40.2683572419386));
#26972=CARTESIAN_POINT('Ctrl Pts',(-23.4799581165932,48.9847707947378,-40.163058226477));
#26973=CARTESIAN_POINT('Ctrl Pts',(-21.0487285831441,46.5262674731227,-40.0051097032845));
#26974=CARTESIAN_POINT('Ctrl Pts',(-17.6662371792997,47.2252500904106,-39.8471611800921));
#26975=CARTESIAN_POINT('Ctrl Pts',(-16.3999441821527,50.4361309372171,-39.6892126568996));
#26976=CARTESIAN_POINT('Ctrl Pts',(-18.3975849010801,53.2535258762515,-39.5312641337071));
#26977=CARTESIAN_POINT('Ctrl Pts',(-21.848150909044,53.1200739456119,-39.3733156105146));
#26978=CARTESIAN_POINT('Ctrl Pts',(-23.6230224069675,50.158234898072,-39.2153670873222));
#26979=CARTESIAN_POINT('Ctrl Pts',(-22.1130258952668,47.0526834926192,-39.0574185641297));
#26980=CARTESIAN_POINT('Ctrl Pts',(-18.6872049245772,46.6194976592071,-38.8994700409372));
#26981=CARTESIAN_POINT('Ctrl Pts',(-16.4516594120846,49.2512485472298,-38.7415215177447));
#26982=CARTESIAN_POINT('Ctrl Pts',(-17.4332843386828,52.5619007101268,-38.5835729945523));
#26983=CARTESIAN_POINT('Ctrl Pts',(-20.7420733238179,53.5497397950539,-38.4256244713598));
#26984=CARTESIAN_POINT('Ctrl Pts',(-23.3780464773465,51.3191456129741,-38.2676759481674));
#26985=CARTESIAN_POINT('Ctrl Pts',(-22.951247888663,47.8925182840191,-38.1097274249748));
#26986=CARTESIAN_POINT('Ctrl Pts',(-19.8486424668251,46.3766825092365,-37.9517789017824));
#26987=CARTESIAN_POINT('Ctrl Pts',(-16.883268382598,48.1459975115365,-37.7938303785899));
#26988=CARTESIAN_POINT('Ctrl Pts',(-16.7437400318118,51.5962806821587,-37.6358818553975));
#26989=CARTESIAN_POINT('Ctrl Pts',(-19.5565635760592,53.5992644563693,-37.477933332205));
#26990=CARTESIAN_POINT('Ctrl Pts',(-22.7714374310744,52.3389047405107,-37.3199848090126));
#26991=CARTESIAN_POINT('Ctrl Pts',(-23.4735332609671,48.9579311678064,-37.16203628582));
#26992=CARTESIAN_POINT('Ctrl Pts',(-21.0262821237837,46.5217697438983,-37.0040877626276));
#26993=CARTESIAN_POINT('Ctrl Pts',(-17.648532198978,47.239213891668,-36.8461392394351));
#26994=CARTESIAN_POINT('Ctrl Pts',(-16.4027866121701,50.4597788463525,-36.6881907162427));
#26995=CARTESIAN_POINT('Ctrl Pts',(-18.4185250000732,53.263476300571,-36.5302421930502));
#26996=CARTESIAN_POINT('Ctrl Pts',(-21.8681386718888,53.1082790492255,-36.3722936698577));
#26997=CARTESIAN_POINT('Ctrl Pts',(-23.6239678268391,50.1348997169674,-36.2143451466652));
#26998=CARTESIAN_POINT('Ctrl Pts',(-22.09405557116,47.0392109146336,-36.0563966234728));
#26999=CARTESIAN_POINT('Ctrl Pts',(-18.6655268169483,46.6279795274162,-35.8984481002803));
#27000=CARTESIAN_POINT('Ctrl Pts',(-16.4469243116338,49.2740565474523,-35.7404995770879));
#27001=CARTESIAN_POINT('Ctrl Pts',(-17.449787471053,52.5783244172767,-35.5825510538954));
#27002=CARTESIAN_POINT('Ctrl Pts',(-20.7648507692583,53.5449039541813,-35.4246025307029));
#27003=CARTESIAN_POINT('Ctrl Pts',(-23.3864471368627,51.2974268891935,-35.2666540075105));
#27004=CARTESIAN_POINT('Ctrl Pts',(-22.9376548796072,47.8736123232374,-35.108705484318));
#27005=CARTESIAN_POINT('Ctrl Pts',(-19.8253802877465,46.3777287926399,-34.9507569611255));
#27006=CARTESIAN_POINT('Ctrl Pts',(-16.8714280781675,48.1660483993591,-34.7928084379331));
#27007=CARTESIAN_POINT('Ctrl Pts',(-16.7540568789002,51.6171561452617,-34.6348599147406));
#27008=CARTESIAN_POINT('Ctrl Pts',(-19.5796835866367,53.602037597837,-34.4769113915481));
#27009=CARTESIAN_POINT('Ctrl Pts',(-22.7863984030238,52.3210611114746,-34.3189628683556));
#27010=CARTESIAN_POINT('Ctrl Pts',(-23.4667705318659,48.935649107221,-34.1610143451632));
#27011=CARTESIAN_POINT('Ctrl Pts',(-21.0039272565248,46.515251686681,-34.0030658219707));
#27012=CARTESIAN_POINT('Ctrl Pts',(-17.6308536707599,47.2543695779982,-33.8451172987782));
#27013=CARTESIAN_POINT('Ctrl Pts',(-16.4058130073886,50.4828670683699,-33.6871687755858));
#27014=CARTESIAN_POINT('Ctrl Pts',(-18.4395123779619,53.2735636735887,-33.5292202523933));
#27015=CARTESIAN_POINT('Ctrl Pts',(-21.8880584153516,53.0962196569031,-33.3712717292008));
#27016=CARTESIAN_POINT('Ctrl Pts',(-23.6247593102429,50.1116274445677,-33.2133232060084));
#27017=CARTESIAN_POINT('Ctrl Pts',(-22.0750011806081,47.025826023238,-33.0553746828159));
#27018=CARTESIAN_POINT('Ctrl Pts',(-18.6439025888241,46.6366176912258,-32.8974261596234));
#27019=CARTESIAN_POINT('Ctrl Pts',(-16.4423362759149,49.2968858059303,-32.7394776364309));
#27020=CARTESIAN_POINT('Ctrl Pts',(-17.4663954601827,52.5946461761462,-32.5815291132385));
#27021=CARTESIAN_POINT('Ctrl Pts',(-20.7875968246039,53.5399197710466,-32.423580590046));
#27022=CARTESIAN_POINT('Ctrl Pts',(-23.3947081018314,51.2756557713323,-32.2656320668536));
#27023=CARTESIAN_POINT('Ctrl Pts',(-22.9239407885082,47.8547934810673,-32.107683543661));
#27024=CARTESIAN_POINT('Ctrl Pts',(-19.8021252898838,46.3789246980118,-31.9497350204686));
#27025=CARTESIAN_POINT('Ctrl Pts',(-16.8597167728345,48.1861747612417,-31.7917864972761));
#27026=CARTESIAN_POINT('Ctrl Pts',(-16.7645075504591,51.637965003453,-31.6338379740837));
#27027=CARTESIAN_POINT('Ctrl Pts',(-19.6028209290277,53.604662193487,-31.4758894508912));
#27028=CARTESIAN_POINT('Ctrl Pts',(-22.8012444915916,52.3031218035313,-31.3179409276987));
#27029=CARTESIAN_POINT('Ctrl Pts',(-23.4598648696293,48.913410920597,-31.1599924045063));
#27030=CARTESIAN_POINT('Ctrl Pts',(-20.9815309974076,46.5088773088445,-31.0020438813138));
#27031=CARTESIAN_POINT('Ctrl Pts',(-17.6132728217522,47.2696384634655,-30.8440953581213));
#27032=CARTESIAN_POINT('Ctrl Pts',(-16.4089875895884,50.5059353830703,-30.6861468349289));
#27033=CARTESIAN_POINT('Ctrl Pts',(-18.460564094239,53.2835160781738,-30.5281983117364));
#27034=CARTESIAN_POINT('Ctrl Pts',(-21.9079003148171,53.0840326088254,-30.3702497885439));
#27035=CARTESIAN_POINT('Ctrl Pts',(-23.6254013461144,50.0883505696652,-30.2123012653514));
#27036=CARTESIAN_POINT('Ctrl Pts',(-22.05586123849,47.0125637560539,-30.054352742159));
#27037=CARTESIAN_POINT('Ctrl Pts',(-18.6223342721148,46.6453945260559,-29.8964042189665));
#27038=CARTESIAN_POINT('Ctrl Pts',(-16.4378949214142,49.3197440535823,-29.738455695774));
#27039=CARTESIAN_POINT('Ctrl Pts',(-17.4831079089184,52.6108609586507,-29.5805071725816));
#27040=CARTESIAN_POINT('Ctrl Pts',(-20.8103104076337,53.5347896383079,-29.4225586493891));
#27041=CARTESIAN_POINT('Ctrl Pts',(-23.4028291041448,51.2538320585774,-29.2646101261967));
#27042=CARTESIAN_POINT('Ctrl Pts',(-22.9101061444555,47.8360630851142,-29.1066616030042));
#27043=CARTESIAN_POINT('Ctrl Pts',(-19.7788784501499,46.3802698988112,-28.9487130798117));
#27044=CARTESIAN_POINT('Ctrl Pts',(-16.8481349406148,48.2063759069389,-28.7907645566192));
#27045=CARTESIAN_POINT('Ctrl Pts',(-16.7750916195284,51.6587063280462,-28.6328160334268));
#27046=CARTESIAN_POINT('Ctrl Pts',(-19.6259746483565,53.6071381719488,-28.4748675102343));
#27047=CARTESIAN_POINT('Ctrl Pts',(-22.8159750830834,52.2850875351969,-28.3169189870418));
#27048=CARTESIAN_POINT('Ctrl Pts',(-23.4528165638848,48.8912175406165,-28.1589704638494));
#27049=CARTESIAN_POINT('Ctrl Pts',(-20.9590942591762,46.5026468548974,-28.0010219406569));
#27050=CARTESIAN_POINT('Ctrl Pts',(-17.5957903984424,47.2850199483718,-27.8430734174645));
#27051=CARTESIAN_POINT('Ctrl Pts',(-16.4123101845813,50.5289827832734,-27.685124894272));
#27052=CARTESIAN_POINT('Ctrl Pts',(-18.4816793672832,53.2933332139959,-27.5271763710795));
#27053=CARTESIAN_POINT('Ctrl Pts',(-21.9276633802435,53.0717181892534,-27.369227847887));
#27054=CARTESIAN_POINT('Ctrl Pts',(-23.6258942504405,50.0650704860399,-27.2112793246945));
#27055=CARTESIAN_POINT('Ctrl Pts',(-22.0366358520053,46.9994237957239,-27.0533308015021));
#27056=CARTESIAN_POINT('Ctrl Pts',(-18.6008241139817,46.6543113906855,-26.8953822783096));
#27057=CARTESIAN_POINT('Ctrl Pts',(-16.4335977273107,49.34262692179,-26.7374337551171));
#27058=CARTESIAN_POINT('Ctrl Pts',(-17.4999295124278,52.6269749186172,-26.5794852319247));
#27059=CARTESIAN_POINT('Ctrl Pts',(-20.8329798605529,53.5295001824726,-26.4215367087322));
#27060=CARTESIAN_POINT('Ctrl Pts',(-23.4108311578128,51.2319837018569,-26.2635881855397));
#27061=CARTESIAN_POINT('Ctrl Pts',(-22.8961090069582,47.8173680419797,-26.1056396623473));
#27062=CARTESIAN_POINT('Ctrl Pts',(-19.7557253769871,46.3818716002278,-25.9476911391548));
#27063=CARTESIAN_POINT('Ctrl Pts',(-16.8365144975983,48.2264374122185,-25.7897426159623));
#27064=CARTESIAN_POINT('Ctrl Pts',(-16.7861443246926,51.6798046863575,-25.6317940927699));
#27065=CARTESIAN_POINT('Ctrl Pts',(-19.6484750337391,53.6086169320315,-25.4738455695774));
#27066=CARTESIAN_POINT('Ctrl Pts',(-22.8319255534364,52.2686663415281,-25.315897046385));
#27067=CARTESIAN_POINT('Ctrl Pts',(-23.4429082212044,48.865459646895,-25.1579485231924));
#27068=CARTESIAN_POINT('Ctrl Pts',(-21.7760378723045,47.2933710986319,-25.0526495077308));
#27069=CARTESIAN_POINT('Ctrl Pts',(-20.7937992825328,47.0307770462543,-25.));
#27070=CARTESIAN_POINT('Ctrl Pts',(-17.4818815371047,49.9978011132584,-38.387416697508));
#27071=CARTESIAN_POINT('Ctrl Pts',(-17.4802992084132,49.8234380468402,-38.3984493876971));
#27072=CARTESIAN_POINT('Ctrl Pts',(-17.4968844920688,49.6493740673602,-38.4094820778862));
#27073=CARTESIAN_POINT('Ctrl Pts',(-17.5327553820264,49.4793798202593,-38.4205147680753));
#27074=CARTESIAN_POINT('Ctrl Pts',(-17.7039361788915,48.6681440043768,-38.4731642758061));
#27075=CARTESIAN_POINT('Ctrl Pts',(-18.3143136885385,47.9495893857989,-38.5258137835369));
#27076=CARTESIAN_POINT('Ctrl Pts',(-19.0871833876552,47.6494490720967,-38.5784632912678));
#27077=CARTESIAN_POINT('Ctrl Pts',(-19.8600530867719,47.3493087583945,-38.6311127989986));
#27078=CARTESIAN_POINT('Ctrl Pts',(-20.7954149753583,47.467582749568,-38.6837623067294));
#27079=CARTESIAN_POINT('Ctrl Pts',(-21.4692352948593,47.950678622831,-38.7364118144603));
#27080=CARTESIAN_POINT('Ctrl Pts',(-22.1430556143602,48.4337744960939,-38.7890613221911));
#27081=CARTESIAN_POINT('Ctrl Pts',(-22.5553343647758,49.2816922514464,-38.8417108299219));
#27082=CARTESIAN_POINT('Ctrl Pts',(-22.5191745698723,50.1099909047412,-38.8943603376527));
#27083=CARTESIAN_POINT('Ctrl Pts',(-22.4830147749687,50.938289558036,-38.9470098453835));
#27084=CARTESIAN_POINT('Ctrl Pts',(-21.9984164347461,51.7469691092731,-38.9996593531144));
#27085=CARTESIAN_POINT('Ctrl Pts',(-21.2850582155025,52.1695272697615,-39.0523088608452));
#27086=CARTESIAN_POINT('Ctrl Pts',(-20.5716999962589,52.5920854302499,-39.104958368576));
#27087=CARTESIAN_POINT('Ctrl Pts',(-19.6295818979943,52.6285221999896,-39.1576078763068));
#27088=CARTESIAN_POINT('Ctrl Pts',(-18.8858120137717,52.2621198072975,-39.2102573840377));
#27089=CARTESIAN_POINT('Ctrl Pts',(-18.1420421295491,51.8957174146055,-39.2629068917685));
#27090=CARTESIAN_POINT('Ctrl Pts',(-17.5966204593686,51.1264758594817,-39.3155563994993));
#27091=CARTESIAN_POINT('Ctrl Pts',(-17.4967794589032,50.3035170019982,-39.3682059072301));
#27092=CARTESIAN_POINT('Ctrl Pts',(-17.4846361068648,50.2034230619036,-39.3746095039894));
#27093=CARTESIAN_POINT('Ctrl Pts',(-17.4790842761961,50.1025344761466,-39.3810131007487));
#27094=CARTESIAN_POINT('Ctrl Pts',(-17.4798420534852,50.0015648820515,-39.387416697508));
#27095=CARTESIAN_POINT('Ctrl Pts',(-19.2062007174672,47.0307770462543,-40.));
#27096=CARTESIAN_POINT('Ctrl Pts',(-18.2239621276955,47.2933710986319,-39.9473504922692));
#27097=CARTESIAN_POINT('Ctrl Pts',(-16.5570907656171,48.8654532317005,-39.8420514768075));
#27098=CARTESIAN_POINT('Ctrl Pts',(-17.16807532845,52.2686690815805,-39.6841029536151));
#27099=CARTESIAN_POINT('Ctrl Pts',(-20.3515248609294,53.6086146806686,-39.5261544304226));
#27100=CARTESIAN_POINT('Ctrl Pts',(-23.2138551423641,51.6798054402274,-39.3682059072301));
#27101=CARTESIAN_POINT('Ctrl Pts',(-23.1634851378897,48.2264371018949,-39.2102573840377));
#27102=CARTESIAN_POINT('Ctrl Pts',(-20.2442745178934,46.3818724340551,-39.0523088608451));
#27103=CARTESIAN_POINT('Ctrl Pts',(-17.103891455686,47.8173681789784,-38.8943603376527));
#27104=CARTESIAN_POINT('Ctrl Pts',(-16.5891692994355,51.231983621924,-38.7364118144602));
#27105=CARTESIAN_POINT('Ctrl Pts',(-19.167020277377,53.5294996249073,-38.5784632912678));
#27106=CARTESIAN_POINT('Ctrl Pts',(-22.5000701187915,52.6269745712345,-38.4205147680753));
#27107=CARTESIAN_POINT('Ctrl Pts',(-23.5664017687871,49.3426270004872,-38.2625662448828));
#27108=CARTESIAN_POINT('Ctrl Pts',(-21.3991756821973,46.6543118776375,-38.1046177216904));
#27109=CARTESIAN_POINT('Ctrl Pts',(-17.9633644414303,46.9994242206471,-37.9466691984979));
#27110=CARTESIAN_POINT('Ctrl Pts',(-16.3741062672361,50.0650704790755,-37.7887206753054));
#27111=CARTESIAN_POINT('Ctrl Pts',(-18.0723368961882,53.0717177485,-37.630772152113));
#27112=CARTESIAN_POINT('Ctrl Pts',(-21.5183204151355,53.2933327434377,-37.4728236289205));
#27113=CARTESIAN_POINT('Ctrl Pts',(-23.5876893022666,50.5289827072374,-37.314875105728));
#27114=CARTESIAN_POINT('Ctrl Pts',(-22.4042092574597,47.2850203370204,-37.1569265825356));
#27115=CARTESIAN_POINT('Ctrl Pts',(-19.0409058781059,46.5026473552099,-36.9989780593431));
#27116=CARTESIAN_POINT('Ctrl Pts',(-16.5471839301236,48.891217699314,-36.8410295361507));
#27117=CARTESIAN_POINT('Ctrl Pts',(-17.1840253198474,52.2850872082152,-36.6830810129582));
#27118=CARTESIAN_POINT('Ctrl Pts',(-20.3740252981191,53.6071376558454,-36.5251324897657));
#27119=CARTESIAN_POINT('Ctrl Pts',(-23.2249079190488,51.6587060907077,-36.3671839665732));
#27120=CARTESIAN_POINT('Ctrl Pts',(-23.1518646084073,48.2063761635784,-36.2092354433808));
#27121=CARTESIAN_POINT('Ctrl Pts',(-20.2211215182128,46.3802704167281,-36.0512869201883));
#27122=CARTESIAN_POINT('Ctrl Pts',(-17.0898942719283,47.8360633947361,-35.8933383969959));
#27123=CARTESIAN_POINT('Ctrl Pts',(-16.5971713827397,51.2538318791758,-35.7353898738033));
#27124=CARTESIAN_POINT('Ctrl Pts',(-19.1896897083071,53.5347891325428,-35.5774413506109));
#27125=CARTESIAN_POINT('Ctrl Pts',(-22.5168917309592,52.6108605850829,-35.4194928274184));
#27126=CARTESIAN_POINT('Ctrl Pts',(-23.562104568912,49.319744150915,-35.261544304226));
#27127=CARTESIAN_POINT('Ctrl Pts',(-21.3776655307659,46.6453950060402,-35.1035957810335));
#27128=CARTESIAN_POINT('Ctrl Pts',(-17.9441390556672,47.0125641835028,-34.945647257841));
#27129=CARTESIAN_POINT('Ctrl Pts',(-16.374599172616,50.0883505570237,-34.7876987346486));
#27130=CARTESIAN_POINT('Ctrl Pts',(-18.0920999581694,53.0840321675552,-34.6297502114561));
#27131=CARTESIAN_POINT('Ctrl Pts',(-21.5394356854951,53.2835156083612,-34.4718016882636));
#27132=CARTESIAN_POINT('Ctrl Pts',(-23.5910118966017,50.50593531068,-34.3138531650712));
#27133=CARTESIAN_POINT('Ctrl Pts',(-22.3867268367498,47.2696388541317,-34.1559046418787));
#27134=CARTESIAN_POINT('Ctrl Pts',(-19.0184691430321,46.5088778083619,-33.9979561186862));
#27135=CARTESIAN_POINT('Ctrl Pts',(-16.5401356254157,48.9134110760685,-33.8400075954937));
#27136=CARTESIAN_POINT('Ctrl Pts',(-17.1987559092166,52.3031214739955,-33.6820590723013));
#27137=CARTESIAN_POINT('Ctrl Pts',(-20.3971790141429,53.6046616777241,-33.5241105491088));
#27138=CARTESIAN_POINT('Ctrl Pts',(-23.2354919865996,51.6379647690895,-33.3661620259163));
#27139=CARTESIAN_POINT('Ctrl Pts',(-23.140282777847,48.1861750207679,-33.2082135027238));
#27140=CARTESIAN_POINT('Ctrl Pts',(-20.1978746818039,46.3789252161231,-33.0502649795314));
#27141=CARTESIAN_POINT('Ctrl Pts',(-17.0760596298556,47.8547937880081,-32.8923164563389));
#27142=CARTESIAN_POINT('Ctrl Pts',(-16.6052923838908,51.2756555888085,-32.7343679331464));
#27143=CARTESIAN_POINT('Ctrl Pts',(-19.2124032880871,53.5399192645472,-32.576419409954));
#27144=CARTESIAN_POINT('Ctrl Pts',(-22.5336041773036,52.5946458048986,-32.4184708867615));
#27145=CARTESIAN_POINT('Ctrl Pts',(-23.5576632150468,49.2968859065335,-32.260522363569));
#27146=CARTESIAN_POINT('Ctrl Pts',(-21.3560972171426,46.6366181724659,-32.1025738403766));
#27147=CARTESIAN_POINT('Ctrl Pts',(-17.9249991162877,47.0258264487893,-31.9446253171841));
#27148=CARTESIAN_POINT('Ctrl Pts',(-16.3752412083956,50.1116274285957,-31.7866767939916));
#27149=CARTESIAN_POINT('Ctrl Pts',(-18.1119418547959,53.0962192138892,-31.6287282707992));
#27150=CARTESIAN_POINT('Ctrl Pts',(-21.56048739876,53.2735632052001,-31.4707797476067));
#27151=CARTESIAN_POINT('Ctrl Pts',(-23.5941864783473,50.4828669992804,-31.3128312244143));
#27152=CARTESIAN_POINT('Ctrl Pts',(-22.3691459902575,47.2543699708491,-31.1548827012218));
#27153=CARTESIAN_POINT('Ctrl Pts',(-18.9960728871194,46.5152521852863,-30.9969341780293));
#27154=CARTESIAN_POINT('Ctrl Pts',(-16.5332299641673,48.9356492595106,-30.8389856548368));
#27155=CARTESIAN_POINT('Ctrl Pts',(-17.2136019956601,52.321060779372,-30.6810371316444));
#27156=CARTESIAN_POINT('Ctrl Pts',(-20.4203163532235,53.6020370824496,-30.5230886084519));
#27157=CARTESIAN_POINT('Ctrl Pts',(-23.2459426566631,51.6171559138756,-30.3651400852594));
#27158=CARTESIAN_POINT('Ctrl Pts',(-23.1285714741897,48.166048661765,-30.207191562067));
#27159=CARTESIAN_POINT('Ctrl Pts',(-20.1746196872686,46.3777293109224,-30.0492430388745));
#27160=CARTESIAN_POINT('Ctrl Pts',(-17.0623455407189,47.8736126274854,-29.891294515682));
#27161=CARTESIAN_POINT('Ctrl Pts',(-16.6135533476775,51.2974267035548,-29.7333459924896));
#27162=CARTESIAN_POINT('Ctrl Pts',(-19.2351493401782,53.5449034469686,-29.5753974692971));
#27163=CARTESIAN_POINT('Ctrl Pts',(-22.5502121640569,52.5783240483645,-29.4174489461047));
#27164=CARTESIAN_POINT('Ctrl Pts',(-23.5530751799844,49.274056651322,-29.2595004229121));
#27165=CARTESIAN_POINT('Ctrl Pts',(-21.3344729921125,46.627980009892,-29.1015518997197));
#27166=CARTESIAN_POINT('Ctrl Pts',(-17.9059447284621,47.0392113382703,-28.9436033765272));
#27167=CARTESIAN_POINT('Ctrl Pts',(-16.3760326916862,50.1348996976644,-28.7856548533347));
#27168=CARTESIAN_POINT('Ctrl Pts',(-18.1318615954084,53.1082786044884,-28.6277063301423));
#27169=CARTESIAN_POINT('Ctrl Pts',(-21.5814747736461,53.2634758336214,-28.4697578069498));
#27170=CARTESIAN_POINT('Ctrl Pts',(-23.5972128731322,50.4597787805748,-28.3118092837574));
#27171=CARTESIAN_POINT('Ctrl Pts',(-22.3514674645701,47.2392142866714,-28.1538607605649));
#27172=CARTESIAN_POINT('Ctrl Pts',(-18.9737180230564,46.5217702416014,-27.9959122373724));
#27173=CARTESIAN_POINT('Ctrl Pts',(-16.5264672360391,48.9579313168502,-27.8379637141799));
#27174=CARTESIAN_POINT('Ctrl Pts',(-17.2285629654577,52.3389044059643,-27.6800151909875));
#27175=CARTESIAN_POINT('Ctrl Pts',(-20.4434363605156,53.599263941172,-27.522066667795));
#27176=CARTESIAN_POINT('Ctrl Pts',(-23.2562595022286,51.5962804541496,-27.3641181446025));
#27177=CARTESIAN_POINT('Ctrl Pts',(-23.1167311715492,48.1459977760775,-27.2061696214101));
#27178=CARTESIAN_POINT('Ctrl Pts',(-20.151357511322,46.3766830290446,-27.0482210982176));
#27179=CARTESIAN_POINT('Ctrl Pts',(-17.0487525340105,47.892518582992,-26.8902725750251));
#27180=CARTESIAN_POINT('Ctrl Pts',(-16.6219540051685,51.3191454290078,-26.7323240518326));
#27181=CARTESIAN_POINT('Ctrl Pts',(-19.2579267840424,53.5497392783032,-26.5743755286402));
#27182=CARTESIAN_POINT('Ctrl Pts',(-22.5667152906276,52.5619003598412,-26.4164270054477));
#27183=CARTESIAN_POINT('Ctrl Pts',(-23.5483400872305,49.251248624616,-26.2584784822553));
#27184=CARTESIAN_POINT('Ctrl Pts',(-21.3127948732631,46.619498196827,-26.1005299590628));
#27185=CARTESIAN_POINT('Ctrl Pts',(-17.8869744362753,47.0526838174963,-25.9425814358703));
#27186=CARTESIAN_POINT('Ctrl Pts',(-16.3769780519003,50.158235047232,-25.7846329126779));
#27187=CARTESIAN_POINT('Ctrl Pts',(-18.1518494766411,53.1200731989091,-25.6266843894854));
#27188=CARTESIAN_POINT('Ctrl Pts',(-21.6024146227446,53.2535259255151,-25.4687358662929));
#27189=CARTESIAN_POINT('Ctrl Pts',(-23.6000558056709,50.4361300140704,-25.3107873431005));
#27190=CARTESIAN_POINT('Ctrl Pts',(-22.3337614586311,47.2252518860991,-25.152838819908));
#27191=CARTESIAN_POINT('Ctrl Pts',(-18.9512736956997,46.5262657145773,-24.9948902967155));
#27192=CARTESIAN_POINT('Ctrl Pts',(-16.520037414612,48.9847755076057,-24.836941773523));
#27193=CARTESIAN_POINT('Ctrl Pts',(-17.003216778308,51.2245165804373,-24.7316427580614));
#27194=CARTESIAN_POINT('Ctrl Pts',(-17.6639373423038,51.9973015569306,-24.6789932503306));
#27195=CARTESIAN_POINT('Ctrl Pts',(-19.2540671456531,47.2098224301578,-40.1070022498898));
#27196=CARTESIAN_POINT('Ctrl Pts',(-18.3310579529763,47.4565819515315,-40.054352742159));
#27197=CARTESIAN_POINT('Ctrl Pts',(-16.7646996300298,48.9338668755566,-39.9490537266973));
#27198=CARTESIAN_POINT('Ctrl Pts',(-17.3388415686086,52.1318673886832,-39.7911052035049));
#27199=CARTESIAN_POINT('Ctrl Pts',(-20.3303277650369,53.391013708655,-39.6331566803124));
#27200=CARTESIAN_POINT('Ctrl Pts',(-23.0200583353412,51.5785124707825,-39.47520815712));
#27201=CARTESIAN_POINT('Ctrl Pts',(-22.9727256631686,48.333383685198,-39.3172596339274));
#27202=CARTESIAN_POINT('Ctrl Pts',(-20.2295446624681,46.600047037023,-39.159311110735));
#27203=CARTESIAN_POINT('Ctrl Pts',(-17.278528010172,47.9489817891393,-39.0013625875425));
#27204=CARTESIAN_POINT('Ctrl Pts',(-16.7948438148646,51.1576944951099,-38.8434140643501));
#27205=CARTESIAN_POINT('Ctrl Pts',(-19.2172493024601,53.3166693237904,-38.6854655411576));
#27206=CARTESIAN_POINT('Ctrl Pts',(-22.3493148467294,52.4685669077014,-38.5275170179651));
#27207=CARTESIAN_POINT('Ctrl Pts',(-23.3513462529859,49.3822668668425,-38.3695684947726));
#27208=CARTESIAN_POINT('Ctrl Pts',(-21.314804804338,46.8560582684008,-38.2116199715802));
#27209=CARTESIAN_POINT('Ctrl Pts',(-18.0861744160049,47.1803601930261,-38.0536714483877));
#27210=CARTESIAN_POINT('Ctrl Pts',(-16.5927491733059,50.0611467020172,-37.8957229251953));
#27211=CARTESIAN_POINT('Ctrl Pts',(-18.1885757862396,52.8864918856763,-37.7377744020028));
#27212=CARTESIAN_POINT('Ctrl Pts',(-21.4267650601314,53.0947434038844,-37.5798258788103));
#27213=CARTESIAN_POINT('Ctrl Pts',(-23.3713501393079,50.4970848291154,-37.4218773556178));
#27214=CARTESIAN_POINT('Ctrl Pts',(-22.2592344353625,47.448734744332,-37.2639288324254));
#27215=CARTESIAN_POINT('Ctrl Pts',(-19.0987396541238,46.7135391800028,-37.1059803092329));
#27216=CARTESIAN_POINT('Ctrl Pts',(-16.7553901808531,48.9580777350151,-36.9480317860405));
#27217=CARTESIAN_POINT('Ctrl Pts',(-17.3538297688648,52.1472954954265,-36.790083262848));
#27218=CARTESIAN_POINT('Ctrl Pts',(-20.3514714164691,53.3896257490454,-36.6321347396555));
#27219=CARTESIAN_POINT('Ctrl Pts',(-23.0304446249768,51.5586854208488,-36.474186216463));
#27220=CARTESIAN_POINT('Ctrl Pts',(-22.961805856466,48.3145324298384,-36.3162376932706));
#27221=CARTESIAN_POINT('Ctrl Pts',(-20.2077877983358,46.5985416220098,-36.1582891700781));
#27222=CARTESIAN_POINT('Ctrl Pts',(-17.2653748624394,47.9665496755805,-36.0003406468856));
#27223=CARTESIAN_POINT('Ctrl Pts',(-16.8023633692043,51.1782252933267,-35.8423921236932));
#27224=CARTESIAN_POINT('Ctrl Pts',(-19.2385517572395,53.3216398719068,-35.6844436005007));
#27225=CARTESIAN_POINT('Ctrl Pts',(-22.3651221086596,52.4534246016432,-35.5264950773082));
#27226=CARTESIAN_POINT('Ctrl Pts',(-23.3473081760575,49.3607638626542,-35.3685465541158));
#27227=CARTESIAN_POINT('Ctrl Pts',(-21.2945917240194,46.8476790878841,-35.2105980309233));
#27228=CARTESIAN_POINT('Ctrl Pts',(-18.0681083290308,47.1927078106349,-35.0526495077308));
#27229=CARTESIAN_POINT('Ctrl Pts',(-16.5932123562856,50.0830229815446,-34.8947009845384));
#27230=CARTESIAN_POINT('Ctrl Pts',(-18.2071471273313,52.8980637401206,-34.7367524613459));
#27231=CARTESIAN_POINT('Ctrl Pts',(-21.4466070708717,53.0855182461522,-34.5788039381534));
#27232=CARTESIAN_POINT('Ctrl Pts',(-23.3744723798173,50.4754272001937,-34.4208554149609));
#27233=CARTESIAN_POINT('Ctrl Pts',(-22.2428062119211,47.434280771284,-34.2629068917685));
#27234=CARTESIAN_POINT('Ctrl Pts',(-19.0776558635433,46.7193939342282,-34.104958368576));
#27235=CARTESIAN_POINT('Ctrl Pts',(-16.7487668918621,48.9789328418844,-33.9470098453835));
#27236=CARTESIAN_POINT('Ctrl Pts',(-17.3676720975443,52.1642422874502,-33.7890613221911));
#27237=CARTESIAN_POINT('Ctrl Pts',(-20.3732289537489,53.3872990734386,-33.6311127989986));
#27238=CARTESIAN_POINT('Ctrl Pts',(-23.0403904688349,51.5391948095847,-33.4731642758062));
#27239=CARTESIAN_POINT('Ctrl Pts',(-22.9509224151245,48.2955494243743,-33.3152157526136));
#27240=CARTESIAN_POINT('Ctrl Pts',(-20.185942755869,46.5972775375629,-33.1572672294212));
#27241=CARTESIAN_POINT('Ctrl Pts',(-17.2523744550604,47.9841506183174,-32.9993187062287));
#27242=CARTESIAN_POINT('Ctrl Pts',(-16.8099946705951,51.1987330241562,-32.8413701830363));
#27243=CARTESIAN_POINT('Ctrl Pts',(-19.2598956986747,53.3264606548093,-32.6834216598438));
#27244=CARTESIAN_POINT('Ctrl Pts',(-22.3808267875112,52.4381875794745,-32.5254731366513));
#27245=CARTESIAN_POINT('Ctrl Pts',(-23.3431346376848,49.3392839799533,-32.3675246134589));
#27246=CARTESIAN_POINT('Ctrl Pts',(-21.2743239887134,46.8394315010391,-32.2095760902664));
#27247=CARTESIAN_POINT('Ctrl Pts',(-18.0501225359877,47.2051703557871,-32.0516275670739));
#27248=CARTESIAN_POINT('Ctrl Pts',(-16.5938156770396,50.1048962480416,-31.8936790438815));
#27249=CARTESIAN_POINT('Ctrl Pts',(-18.2257925493063,52.909515902472,-31.735730520689));
#27250=CARTESIAN_POINT('Ctrl Pts',(-21.4663893570366,53.0761659770572,-31.5777819974965));
#27251=CARTESIAN_POINT('Ctrl Pts',(-23.3774555329581,50.4537499176037,-31.4198334743041));
#27252=CARTESIAN_POINT('Ctrl Pts',(-22.2262854978131,47.4199326080388,-31.2618849511116));
#27253=CARTESIAN_POINT('Ctrl Pts',(-19.0566101112138,46.7253839335625,-31.1039364279191));
#27254=CARTESIAN_POINT('Ctrl Pts',(-16.7422776448703,48.9998300535794,-30.9459879047266));
#27255=CARTESIAN_POINT('Ctrl Pts',(-17.3816229587763,52.1810998452219,-30.7880393815342));
#27256=CARTESIAN_POINT('Ctrl Pts',(-20.3949711016219,53.384832742355,-30.6300908583417));
#27257=CARTESIAN_POINT('Ctrl Pts',(-23.0502109591299,51.5196407370289,-30.4721423351493));
#27258=CARTESIAN_POINT('Ctrl Pts',(-22.9399173079678,48.276636693223,-30.3141938119568));
#27259=CARTESIAN_POINT('Ctrl Pts',(-20.1640900472143,46.5961537459451,-30.1562452887643));
#27260=CARTESIAN_POINT('Ctrl Pts',(-17.2394873312249,48.0018346739166,-29.9982967655719));
#27261=CARTESIAN_POINT('Ctrl Pts',(-16.8177574948161,51.2191913315927,-29.8403482423794));
#27262=CARTESIAN_POINT('Ctrl Pts',(-19.2812701543271,53.3311442889496,-29.6823997191869));
#27263=CARTESIAN_POINT('Ctrl Pts',(-22.3964333057287,52.4228500316744,-29.5244511959944));
#27264=CARTESIAN_POINT('Ctrl Pts',(-23.3388232630524,49.3178313383634,-29.3665026728019));
#27265=CARTESIAN_POINT('Ctrl Pts',(-21.2540037134818,46.8313142232752,-29.2085541496095));
#27266=CARTESIAN_POINT('Ctrl Pts',(-18.0322171357041,47.2177481308435,-29.050605626417));
#27267=CARTESIAN_POINT('Ctrl Pts',(-16.5945594335573,50.1267651895682,-28.8926571032246));
#27268=CARTESIAN_POINT('Ctrl Pts',(-18.2445111212424,52.9208481067826,-28.7347085800321));
#27269=CARTESIAN_POINT('Ctrl Pts',(-21.4861111844538,53.0666868781967,-28.5767600568396));
#27270=CARTESIAN_POINT('Ctrl Pts',(-23.3802994348738,50.4320539281265,-28.4188115336471));
#27271=CARTESIAN_POINT('Ctrl Pts',(-22.2096729946064,47.4056908179454,-28.2608630104547));
#27272=CARTESIAN_POINT('Ctrl Pts',(-19.035603254788,46.7315089483602,-28.1029144872622));
#27273=CARTESIAN_POINT('Ctrl Pts',(-16.7359227120721,49.0207684935577,-27.9449659640697));
#27274=CARTESIAN_POINT('Ctrl Pts',(-17.3956817758482,52.1978674936802,-27.7870174408773));
#27275=CARTESIAN_POINT('Ctrl Pts',(-20.4166969628207,53.3822268226544,-27.6290689176848));
#27276=CARTESIAN_POINT('Ctrl Pts',(-23.0599056946001,51.5000240762409,-27.4711203944924));
#27277=CARTESIAN_POINT('Ctrl Pts',(-22.9287909805204,48.2577948843147,-27.3131718712999));
#27278=CARTESIAN_POINT('Ctrl Pts',(-20.1422305901903,46.5951705553014,-27.1552233481074));
#27279=CARTESIAN_POINT('Ctrl Pts',(-17.2267139884967,48.0196005924119,-26.9972748249149));
#27280=CARTESIAN_POINT('Ctrl Pts',(-16.8256515891527,51.2396004088323,-26.8393263017225));
#27281=CARTESIAN_POINT('Ctrl Pts',(-19.3026741088157,53.3356885176355,-26.68137777853));
#27282=CARTESIAN_POINT('Ctrl Pts',(-22.4119412868763,52.4074166984269,-26.5234292553375));
#27283=CARTESIAN_POINT('Ctrl Pts',(-23.3343736983688,49.2963986451912,-26.3654807321451));
#27284=CARTESIAN_POINT('Ctrl Pts',(-21.2336327942506,46.8233438670796,-26.2075322089526));
#27285=CARTESIAN_POINT('Ctrl Pts',(-18.0143907600572,47.2304082139468,-26.0495836857601));
#27286=CARTESIAN_POINT('Ctrl Pts',(-16.5954477881557,50.1486934078131,-25.8916351625677));
#27287=CARTESIAN_POINT('Ctrl Pts',(-18.263293724891,52.931931482235,-25.7336866393752));
#27288=CARTESIAN_POINT('Ctrl Pts',(-21.5057883519083,53.0573369537037,-25.5757381161827));
#27289=CARTESIAN_POINT('Ctrl Pts',(-23.3829709373934,50.4098311921169,-25.4177895929903));
#27290=CARTESIAN_POINT('Ctrl Pts',(-22.1930346682185,47.3925703559575,-25.2598410697978));
#27291=CARTESIAN_POINT('Ctrl Pts',(-19.0145123297425,46.7357333424386,-25.1018925466053));
#27292=CARTESIAN_POINT('Ctrl Pts',(-16.7298806115618,49.0459939684019,-24.9439440234128));
#27293=CARTESIAN_POINT('Ctrl Pts',(-17.1839240578764,51.1506777193426,-24.8386450079512));
#27294=CARTESIAN_POINT('Ctrl Pts',(-17.8048028959808,51.8768634390787,-24.7859955002204));
#27295=CARTESIAN_POINT('Ctrl Pts',(-19.301933573839,47.3888678140614,-40.2140044997796));
#27296=CARTESIAN_POINT('Ctrl Pts',(-18.438153778257,47.6197928044311,-40.1613549920488));
#27297=CARTESIAN_POINT('Ctrl Pts',(-16.9723084944424,49.0022805194126,-40.0560559765871));
#27298=CARTESIAN_POINT('Ctrl Pts',(-17.5096078087671,51.995065695786,-39.8981074533947));
#27299=CARTESIAN_POINT('Ctrl Pts',(-20.3091306691444,53.1734127366413,-39.7401589302022));
#27300=CARTESIAN_POINT('Ctrl Pts',(-22.8262615283184,51.4772195013377,-39.5822104070098));
#27301=CARTESIAN_POINT('Ctrl Pts',(-22.7819661884474,48.4403302685011,-39.4242618838173));
#27302=CARTESIAN_POINT('Ctrl Pts',(-20.2148148070429,46.8182216399908,-39.2663133606248));
#27303=CARTESIAN_POINT('Ctrl Pts',(-17.4531645646581,48.0805953993001,-39.1083648374324));
#27304=CARTESIAN_POINT('Ctrl Pts',(-17.0005183302937,51.0834053682957,-38.9504163142398));
#27305=CARTESIAN_POINT('Ctrl Pts',(-19.2674783275431,53.1038390226735,-38.7924677910475));
#27306=CARTESIAN_POINT('Ctrl Pts',(-22.1985595746674,52.3101592441684,-38.6345192678549));
#27307=CARTESIAN_POINT('Ctrl Pts',(-23.1362907371846,49.4219067331978,-38.4765707446625));
#27308=CARTESIAN_POINT('Ctrl Pts',(-21.2304339264787,47.0578046591641,-38.31862222147));
#27309=CARTESIAN_POINT('Ctrl Pts',(-18.2089843905794,47.3612961654051,-38.1606736982775));
#27310=CARTESIAN_POINT('Ctrl Pts',(-16.8113920793757,50.0572229249588,-38.002725175085));
#27311=CARTESIAN_POINT('Ctrl Pts',(-18.3048146762911,52.7012660228526,-37.8447766518926));
#27312=CARTESIAN_POINT('Ctrl Pts',(-21.3352097051273,52.896154064331,-37.6868281287001));
#27313=CARTESIAN_POINT('Ctrl Pts',(-23.1550109763493,50.4651869509934,-37.5288796055076));
#27314=CARTESIAN_POINT('Ctrl Pts',(-22.1142596132653,47.6124491516436,-37.3709310823152));
#27315=CARTESIAN_POINT('Ctrl Pts',(-19.1565734301417,46.9244310047958,-37.2129825591227));
#27316=CARTESIAN_POINT('Ctrl Pts',(-16.9635964315826,49.0249377707161,-37.0550340359303));
#27317=CARTESIAN_POINT('Ctrl Pts',(-17.5236342178822,52.0095037826378,-36.8970855127378));
#27318=CARTESIAN_POINT('Ctrl Pts',(-20.328917534819,53.1721138422453,-36.7391369895453));
#27319=CARTESIAN_POINT('Ctrl Pts',(-22.8359813309048,51.45866475099,-36.5811884663528));
#27320=CARTESIAN_POINT('Ctrl Pts',(-22.7717471045247,48.4226886960985,-36.4232399431604));
#27321=CARTESIAN_POINT('Ctrl Pts',(-20.1944540784587,46.8168128272913,-36.2652914199679));
#27322=CARTESIAN_POINT('Ctrl Pts',(-17.4408554529505,48.0970359564251,-36.1073428967755));
#27323=CARTESIAN_POINT('Ctrl Pts',(-17.0075553556689,51.1026187074776,-35.9493943735829));
#27324=CARTESIAN_POINT('Ctrl Pts',(-19.2874138061719,53.1084906112709,-35.7914458503905));
#27325=CARTESIAN_POINT('Ctrl Pts',(-22.21335248636,52.2959886182035,-35.633497327198));
#27326=CARTESIAN_POINT('Ctrl Pts',(-23.132511783203,49.4017835743933,-35.4755488040056));
#27327=CARTESIAN_POINT('Ctrl Pts',(-21.2115179172729,47.049963169728,-35.3176002808131));
#27328=CARTESIAN_POINT('Ctrl Pts',(-18.1920776023944,47.3728514377671,-35.1596517576207));
#27329=CARTESIAN_POINT('Ctrl Pts',(-16.8118255399552,50.0776954060655,-35.0017032344282));
#27330=CARTESIAN_POINT('Ctrl Pts',(-18.3221942964933,52.712095312686,-34.8437547112357));
#27331=CARTESIAN_POINT('Ctrl Pts',(-21.3537784562482,52.8875208839431,-34.6858061880432));
#27332=CARTESIAN_POINT('Ctrl Pts',(-23.1579328630329,50.4449190897075,-34.5278576648507));
#27333=CARTESIAN_POINT('Ctrl Pts',(-22.0988855870924,47.5989226884362,-34.3699091416583));
#27334=CARTESIAN_POINT('Ctrl Pts',(-19.1368425840546,46.9299100600946,-34.2119606184658));
#27335=CARTESIAN_POINT('Ctrl Pts',(-16.9573981583085,49.0444546077003,-34.0540120952734));
#27336=CARTESIAN_POINT('Ctrl Pts',(-17.536588285872,52.0253631009049,-33.8960635720809));
#27337=CARTESIAN_POINT('Ctrl Pts',(-20.3492788933548,53.169936469153,-33.7381150488884));
#27338=CARTESIAN_POINT('Ctrl Pts',(-22.8452889510702,51.44042485008,-33.580166525696));
#27339=CARTESIAN_POINT('Ctrl Pts',(-22.7615620524019,48.4049238279808,-33.4222180025034));
#27340=CARTESIAN_POINT('Ctrl Pts',(-20.1740108299341,46.8156298590027,-33.2642694793111));
#27341=CARTESIAN_POINT('Ctrl Pts',(-17.4286892802651,48.1135074486268,-33.1063209561185));
#27342=CARTESIAN_POINT('Ctrl Pts',(-17.0146969572993,51.1218104595037,-32.9483724329261));
#27343=CARTESIAN_POINT('Ctrl Pts',(-19.3073881092624,53.1130020450714,-32.7904239097336));
#27344=CARTESIAN_POINT('Ctrl Pts',(-22.2280493977188,52.2817293540503,-32.6324753865412));
#27345=CARTESIAN_POINT('Ctrl Pts',(-23.1286060603229,49.3816820533731,-32.4745268633487));
#27346=CARTESIAN_POINT('Ctrl Pts',(-21.1925507602843,47.0422448296122,-32.3165783401562));
#27347=CARTESIAN_POINT('Ctrl Pts',(-18.1752459556877,47.3845142627849,-32.1586298169637));
#27348=CARTESIAN_POINT('Ctrl Pts',(-16.8123901456836,50.0981650674874,-32.0006812937713));
#27349=CARTESIAN_POINT('Ctrl Pts',(-18.3396432438168,52.7228125910548,-31.8427327705788));
#27350=CARTESIAN_POINT('Ctrl Pts',(-21.3722913153132,52.8787687489144,-31.6847842473863));
#27351=CARTESIAN_POINT('Ctrl Pts',(-23.1607245875689,50.424632835927,-31.5268357241939));
#27352=CARTESIAN_POINT('Ctrl Pts',(-22.0834250053688,47.5854952452285,-31.3688872010014));
#27353=CARTESIAN_POINT('Ctrl Pts',(-19.117147335308,46.9355156818388,-31.2109386778089));
#27354=CARTESIAN_POINT('Ctrl Pts',(-16.9513253255734,49.0640108476483,-31.0529901546165));
#27355=CARTESIAN_POINT('Ctrl Pts',(-17.5496439218925,52.0411389110718,-30.895041631424));
#27356=CARTESIAN_POINT('Ctrl Pts',(-20.3696258500203,53.1676284022605,-30.7370931082315));
#27357=CARTESIAN_POINT('Ctrl Pts',(-22.8544792615967,51.4221255601822,-30.579144585039));
#27358=CARTESIAN_POINT('Ctrl Pts',(-22.7512631417458,48.387224724681,-30.4211960618466));
#27359=CARTESIAN_POINT('Ctrl Pts',(-20.1535604071599,46.8145781809679,-30.2632475386541));
#27360=CARTESIAN_POINT('Ctrl Pts',(-17.4166291217309,48.1300567203476,-30.1052990154616));
#27361=CARTESIAN_POINT('Ctrl Pts',(-17.0219616419547,51.1409559596307,-29.9473504922692));
#27362=CARTESIAN_POINT('Ctrl Pts',(-19.3273909684762,53.1173851309305,-29.7894019690767));
#27363=CARTESIAN_POINT('Ctrl Pts',(-22.2426544474004,52.2673760149844,-29.6314534458842));
#27364=CARTESIAN_POINT('Ctrl Pts',(-23.1245713461204,49.3616060254048,-29.4735049226918));
#27365=CARTESIAN_POINT('Ctrl Pts',(-21.1735344348511,47.0346484366585,-29.3155563994993));
#27366=CARTESIAN_POINT('Ctrl Pts',(-18.1584895429461,47.3962849234167,-29.1576078763069));
#27367=CARTESIAN_POINT('Ctrl Pts',(-16.8130861754284,50.1186306814719,-28.9996593531144));
#27368=CARTESIAN_POINT('Ctrl Pts',(-18.3571606470765,52.733417609077,-28.8417108299219));
#27369=CARTESIAN_POINT('Ctrl Pts',(-21.3907475952616,52.869897922772,-28.6837623067294));
#27370=CARTESIAN_POINT('Ctrl Pts',(-23.1633859966154,50.4043290756782,-28.525813783537));
#27371=CARTESIAN_POINT('Ctrl Pts',(-22.0678785246426,47.5721673492192,-28.3678652603445));
#27372=CARTESIAN_POINT('Ctrl Pts',(-19.0974884865195,46.941247655119,-28.209916737152));
#27373=CARTESIAN_POINT('Ctrl Pts',(-16.9453781881051,49.0836056702652,-28.0519682139596));
#27374=CARTESIAN_POINT('Ctrl Pts',(-17.5628005862387,52.0568305813959,-27.8940196907671));
#27375=CARTESIAN_POINT('Ctrl Pts',(-20.3899575651257,53.1651897041368,-27.7360711675746));
#27376=CARTESIAN_POINT('Ctrl Pts',(-22.8635518869715,51.4037676983321,-27.5781226443821));
#27377=CARTESIAN_POINT('Ctrl Pts',(-22.7408507894916,48.3695919925519,-27.4201741211897));
#27378=CARTESIAN_POINT('Ctrl Pts',(-20.1331036690585,46.8136580815583,-27.2622255979972));
#27379=CARTESIAN_POINT('Ctrl Pts',(-17.4046754429829,48.1466826018318,-27.1042770748048));
#27380=CARTESIAN_POINT('Ctrl Pts',(-17.0293491731369,51.1600553886568,-26.9463285516123));
#27381=CARTESIAN_POINT('Ctrl Pts',(-19.3474214335891,53.1216377569678,-26.7883800284198));
#27382=CARTESIAN_POINT('Ctrl Pts',(-22.257167283125,52.2529330370124,-26.6304315052273));
#27383=CARTESIAN_POINT('Ctrl Pts',(-23.120407309507,49.3415486657664,-26.4724829820349));
#27384=CARTESIAN_POINT('Ctrl Pts',(-21.1544707152382,47.0271895373323,-26.3145344588424));
#27385=CARTESIAN_POINT('Ctrl Pts',(-18.1418070838391,47.4081326103973,-26.1565859356499));
#27386=CARTESIAN_POINT('Ctrl Pts',(-16.8139175244112,50.1391517683944,-25.9986374124575));
#27387=CARTESIAN_POINT('Ctrl Pts',(-18.3747379731408,52.7437897655609,-25.840688889265));
#27388=CARTESIAN_POINT('Ctrl Pts',(-21.409162081072,52.8611479818924,-25.6827403660725));
#27389=CARTESIAN_POINT('Ctrl Pts',(-23.1658860691158,50.3835323701632,-25.5247918428801));
#27390=CARTESIAN_POINT('Ctrl Pts',(-22.052307877806,47.5598888258158,-25.3668433196876));
#27391=CARTESIAN_POINT('Ctrl Pts',(-19.0777509637852,46.9452009702999,-25.2088947964951));
#27392=CARTESIAN_POINT('Ctrl Pts',(-16.9397238085116,49.1072124291981,-25.0509462733027));
#27393=CARTESIAN_POINT('Ctrl Pts',(-17.3646313374448,51.076838858248,-24.945647257841));
#27394=CARTESIAN_POINT('Ctrl Pts',(-17.9456684496579,51.7564253212268,-24.8929977501102));
#27395=CARTESIAN_POINT('Ctrl Pts',(-19.3498000020249,47.5679131979649,-40.3210067496694));
#27396=CARTESIAN_POINT('Ctrl Pts',(-18.5452496035378,47.7830036573307,-40.2683572419386));
#27397=CARTESIAN_POINT('Ctrl Pts',(-17.1799173588551,49.0706941632686,-40.163058226477));
#27398=CARTESIAN_POINT('Ctrl Pts',(-17.6803740489257,51.8582640028888,-40.0051097032845));
#27399=CARTESIAN_POINT('Ctrl Pts',(-20.2879335732519,52.9558117646276,-39.847161180092));
#27400=CARTESIAN_POINT('Ctrl Pts',(-22.6324647212955,51.3759265318928,-39.6892126568996));
#27401=CARTESIAN_POINT('Ctrl Pts',(-22.5912067137262,48.5472768518042,-39.5312641337071));
#27402=CARTESIAN_POINT('Ctrl Pts',(-20.2000849516176,47.0363962429587,-39.3733156105146));
#27403=CARTESIAN_POINT('Ctrl Pts',(-17.6278011191441,48.2122090094609,-39.2153670873221));
#27404=CARTESIAN_POINT('Ctrl Pts',(-17.2061928457228,51.0091162414817,-39.0574185641297));
#27405=CARTESIAN_POINT('Ctrl Pts',(-19.3177073526262,52.8910087215565,-38.8994700409372));
#27406=CARTESIAN_POINT('Ctrl Pts',(-22.0478043026054,52.1517515806355,-38.7415215177447));
#27407=CARTESIAN_POINT('Ctrl Pts',(-22.9212352213833,49.461546599553,-38.5835729945523));
#27408=CARTESIAN_POINT('Ctrl Pts',(-21.1460630486194,47.2595510499276,-38.4256244713598));
#27409=CARTESIAN_POINT('Ctrl Pts',(-18.331794365154,47.5422321377839,-38.2676759481673));
#27410=CARTESIAN_POINT('Ctrl Pts',(-17.0300349854455,50.0532991479006,-38.1097274249749));
#27411=CARTESIAN_POINT('Ctrl Pts',(-18.4210535663425,52.5160401600288,-37.9517789017824));
#27412=CARTESIAN_POINT('Ctrl Pts',(-21.2436543501232,52.6975647247778,-37.79383037859));
#27413=CARTESIAN_POINT('Ctrl Pts',(-22.9386718133906,50.4332890728714,-37.6358818553974));
#27414=CARTESIAN_POINT('Ctrl Pts',(-21.969284791168,47.7761635589552,-37.477933332205));
#27415=CARTESIAN_POINT('Ctrl Pts',(-19.2144072061596,47.1353228295887,-37.3199848090125));
#27416=CARTESIAN_POINT('Ctrl Pts',(-17.1718026823121,49.0917978064171,-37.1620362858201));
#27417=CARTESIAN_POINT('Ctrl Pts',(-17.6934386668996,51.8717120698492,-37.0040877626276));
#27418=CARTESIAN_POINT('Ctrl Pts',(-20.306363653169,52.9546019354452,-36.8461392394351));
#27419=CARTESIAN_POINT('Ctrl Pts',(-22.6415180368327,51.3586440811311,-36.6881907162426));
#27420=CARTESIAN_POINT('Ctrl Pts',(-22.5816883525835,48.5308449623585,-36.5302421930502));
#27421=CARTESIAN_POINT('Ctrl Pts',(-20.1811203585817,47.035084032573,-36.3722936698577));
#27422=CARTESIAN_POINT('Ctrl Pts',(-17.6163360434617,48.2275222372696,-36.2143451466653));
#27423=CARTESIAN_POINT('Ctrl Pts',(-17.2127473421335,51.0270121216285,-36.0563966234728));
#27424=CARTESIAN_POINT('Ctrl Pts',(-19.3362758551043,52.8953413506349,-35.8984481002803));
#27425=CARTESIAN_POINT('Ctrl Pts',(-22.0615828640604,52.1385526347637,-35.7404995770878));
#27426=CARTESIAN_POINT('Ctrl Pts',(-22.9177153903485,49.4428032861326,-35.5825510538954));
#27427=CARTESIAN_POINT('Ctrl Pts',(-21.1284441105265,47.2522472515719,-35.4246025307029));
#27428=CARTESIAN_POINT('Ctrl Pts',(-18.3160468757579,47.5529950648994,-35.2666540075104));
#27429=CARTESIAN_POINT('Ctrl Pts',(-17.0304387236248,50.0723678305864,-35.108705484318));
#27430=CARTESIAN_POINT('Ctrl Pts',(-18.4372414656552,52.5261268852514,-34.9507569611255));
#27431=CARTESIAN_POINT('Ctrl Pts',(-21.2609498416249,52.689523521734,-34.792808437933));
#27432=CARTESIAN_POINT('Ctrl Pts',(-22.9413933462485,50.4144109792213,-34.6348599147405));
#27433=CARTESIAN_POINT('Ctrl Pts',(-21.9549649622637,47.7635646055886,-34.4769113915481));
#27434=CARTESIAN_POINT('Ctrl Pts',(-19.1960293045659,47.140426185961,-34.3189628683556));
#27435=CARTESIAN_POINT('Ctrl Pts',(-17.1660294247548,49.1099763735163,-34.1610143451632));
#27436=CARTESIAN_POINT('Ctrl Pts',(-17.7055044741997,51.8864839143595,-34.0030658219707));
#27437=CARTESIAN_POINT('Ctrl Pts',(-20.3253288329608,52.9525738648675,-33.8451172987782));
#27438=CARTESIAN_POINT('Ctrl Pts',(-22.6501874333055,51.3416548905751,-33.6871687755858));
#27439=CARTESIAN_POINT('Ctrl Pts',(-22.5722016896794,48.5142982315872,-33.5292202523932));
#27440=CARTESIAN_POINT('Ctrl Pts',(-20.1620789039991,47.0339821804424,-33.3712717292009));
#27441=CARTESIAN_POINT('Ctrl Pts',(-17.6050041054698,48.2428642789362,-33.2133232060083));
#27442=CARTESIAN_POINT('Ctrl Pts',(-17.2193992440036,51.0448878948513,-33.0553746828159));
#27443=CARTESIAN_POINT('Ctrl Pts',(-19.3548805198501,52.8995434353335,-32.8974261596234));
#27444=CARTESIAN_POINT('Ctrl Pts',(-22.0752720079264,52.1252711286261,-32.739477636431));
#27445=CARTESIAN_POINT('Ctrl Pts',(-22.9140774829609,49.4240801267929,-32.5815291132385));
#27446=CARTESIAN_POINT('Ctrl Pts',(-21.1107775318551,47.2450581581855,-32.423580590046));
#27447=CARTESIAN_POINT('Ctrl Pts',(-18.3003693753878,47.5638581697826,-32.2656320668535));
#27448=CARTESIAN_POINT('Ctrl Pts',(-17.0309646143276,50.0914338869334,-32.1076835436611));
#27449=CARTESIAN_POINT('Ctrl Pts',(-18.4534939383272,52.5361092796376,-31.9497350204686));
#27450=CARTESIAN_POINT('Ctrl Pts',(-21.2781932735898,52.6813715207715,-31.7917864972761));
#27451=CARTESIAN_POINT('Ctrl Pts',(-22.9439936421797,50.3955157542503,-31.6338379740837));
#27452=CARTESIAN_POINT('Ctrl Pts',(-21.9405645129244,47.7510578824183,-31.4758894508912));
#27453=CARTESIAN_POINT('Ctrl Pts',(-19.1776845594024,47.145647430115,-31.3179409276988));
#27454=CARTESIAN_POINT('Ctrl Pts',(-17.1603730062766,49.1281916417172,-31.1599924045062));
#27455=CARTESIAN_POINT('Ctrl Pts',(-17.7176648850087,51.9011779769217,-31.0020438813138));
#27456=CARTESIAN_POINT('Ctrl Pts',(-20.3442805984188,52.9504240621659,-30.8440953581213));
#27457=CARTESIAN_POINT('Ctrl Pts',(-22.6587475640635,51.3246103833355,-30.6861468349288));
#27458=CARTESIAN_POINT('Ctrl Pts',(-22.5626089755239,48.4978127561391,-30.5281983117364));
#27459=CARTESIAN_POINT('Ctrl Pts',(-20.1430307671055,47.0330026159906,-30.3702497885439));
#27460=CARTESIAN_POINT('Ctrl Pts',(-17.5937709122369,48.2582787667788,-30.2123012653514));
#27461=CARTESIAN_POINT('Ctrl Pts',(-17.2261657890932,51.0627205876685,-30.054352742159));
#27462=CARTESIAN_POINT('Ctrl Pts',(-19.3735117826252,52.9036259729115,-29.8964042189665));
#27463=CARTESIAN_POINT('Ctrl Pts',(-22.0888755890722,52.1119019982943,-29.7384556957741));
#27464=CARTESIAN_POINT('Ctrl Pts',(-22.9103194291884,49.4053807124462,-29.5805071725816));
#27465=CARTESIAN_POINT('Ctrl Pts',(-21.0930651562203,47.2379826500416,-29.4225586493891));
#27466=CARTESIAN_POINT('Ctrl Pts',(-18.2847619501882,47.5748217159901,-29.2646101261967));
#27467=CARTESIAN_POINT('Ctrl Pts',(-17.0316129172995,50.1104961733757,-29.1066616030041));
#27468=CARTESIAN_POINT('Ctrl Pts',(-18.4698101729106,52.5459871113712,-28.9487130798117));
#27469=CARTESIAN_POINT('Ctrl Pts',(-21.2953840060693,52.6731089673473,-28.7907645566192));
#27470=CARTESIAN_POINT('Ctrl Pts',(-22.946472558357,50.3766042232299,-28.6328160334268));
#27471=CARTESIAN_POINT('Ctrl Pts',(-21.9260840546788,47.738643880493,-28.4748675102343));
#27472=CARTESIAN_POINT('Ctrl Pts',(-19.159373718251,47.1509863618779,-28.3169189870418));
#27473=CARTESIAN_POINT('Ctrl Pts',(-17.1548336641381,49.1464428469726,-28.1589704638494));
#27474=CARTESIAN_POINT('Ctrl Pts',(-17.7299193966292,51.9157936691118,-28.0010219406569));
#27475=CARTESIAN_POINT('Ctrl Pts',(-20.3632181674306,52.9481525856191,-27.8430734174644));
#27476=CARTESIAN_POINT('Ctrl Pts',(-22.667198079343,51.3075113204235,-27.685124894272));
#27477=CARTESIAN_POINT('Ctrl Pts',(-22.5529105984627,48.4813891007891,-27.5271763710795));
#27478=CARTESIAN_POINT('Ctrl Pts',(-20.1239767479268,47.0321456078151,-27.3692278478871));
#27479=CARTESIAN_POINT('Ctrl Pts',(-17.5826368974691,48.2737646112518,-27.2112793246946));
#27480=CARTESIAN_POINT('Ctrl Pts',(-17.2330467571211,51.0805103684813,-27.0533308015021));
#27481=CARTESIAN_POINT('Ctrl Pts',(-19.3921687583624,52.9075869963002,-26.8953822783096));
#27482=CARTESIAN_POINT('Ctrl Pts',(-22.1023932793737,52.0984493755979,-26.7374337551172));
#27483=CARTESIAN_POINT('Ctrl Pts',(-22.9064409206452,49.3866986863416,-26.5794852319247));
#27484=CARTESIAN_POINT('Ctrl Pts',(-21.0753086362257,47.2310352075848,-26.4215367087322));
#27485=CARTESIAN_POINT('Ctrl Pts',(-18.269223407621,47.5858570068479,-26.2635881855397));
#27486=CARTESIAN_POINT('Ctrl Pts',(-17.0323872606667,50.1296101289755,-26.1056396623473));
#27487=CARTESIAN_POINT('Ctrl Pts',(-18.4861822213906,52.5556480488868,-25.9476911391548));
#27488=CARTESIAN_POINT('Ctrl Pts',(-21.3125358102357,52.6649590100811,-25.7897426159623));
#27489=CARTESIAN_POINT('Ctrl Pts',(-22.9488012008383,50.3572335482097,-25.6317940927699));
#27490=CARTESIAN_POINT('Ctrl Pts',(-21.9115810873935,47.7272072956741,-25.4738455695774));
#27491=CARTESIAN_POINT('Ctrl Pts',(-19.1409895978279,47.1546685981612,-25.3158970463849));
#27492=CARTESIAN_POINT('Ctrl Pts',(-17.1495670054614,49.1684308899942,-25.1579485231925));
#27493=CARTESIAN_POINT('Ctrl Pts',(-17.5453386170133,51.0029999971534,-25.0526495077308));
#27494=CARTESIAN_POINT('Ctrl Pts',(-18.0865340033349,51.6359872033749,-25.));
#27495=CARTESIAN_POINT('Ctrl Pts',(-17.4850543912228,50.0017607343381,-39.112583302492));
#27496=CARTESIAN_POINT('Ctrl Pts',(-17.4831411703387,50.2933091094334,-39.0941950563712));
#27497=CARTESIAN_POINT('Ctrl Pts',(-17.5300111809499,50.5842626429816,-39.0758068102504));
#27498=CARTESIAN_POINT('Ctrl Pts',(-17.6283799757769,50.856613782824,-39.0574185641297));
#27499=CARTESIAN_POINT('Ctrl Pts',(-17.9100310146906,51.63641373484,-39.0047690563988));
#27500=CARTESIAN_POINT('Ctrl Pts',(-18.6138691836584,52.2637112281982,-38.952119548668));
#27501=CARTESIAN_POINT('Ctrl Pts',(-19.4208044264721,52.4541504513905,-38.8994700409372));
#27502=CARTESIAN_POINT('Ctrl Pts',(-20.2277396692859,52.6445896745828,-38.8468205332064));
#27503=CARTESIAN_POINT('Ctrl Pts',(-21.1377719859456,52.3981706276091,-38.7941710254755));
#27504=CARTESIAN_POINT('Ctrl Pts',(-21.7383599640718,51.8265936072752,-38.7415215177447));
#27505=CARTESIAN_POINT('Ctrl Pts',(-22.338947942198,51.2550165869413,-38.6888720100139));
#27506=CARTESIAN_POINT('Ctrl Pts',(-22.6300915817907,50.3582815932472,-38.6362225022831));
#27507=CARTESIAN_POINT('Ctrl Pts',(-22.479801372793,49.5429148381292,-38.5835729945523));
#27508=CARTESIAN_POINT('Ctrl Pts',(-22.3295111637953,48.7275480830112,-38.5309234868215));
#27509=CARTESIAN_POINT('Ctrl Pts',(-21.7377871062073,47.9935495664694,-38.4782739790906));
#27510=CARTESIAN_POINT('Ctrl Pts',(-20.9728802968358,47.6736638228412,-38.4256244713598));
#27511=CARTESIAN_POINT('Ctrl Pts',(-20.2079734874642,47.353778079213,-38.372974963629));
#27512=CARTESIAN_POINT('Ctrl Pts',(-19.2698839263091,47.4480051084985,-38.3203254558981));
#27513=CARTESIAN_POINT('Ctrl Pts',(-18.5838792491135,47.913629791494,-38.2676759481673));
#27514=CARTESIAN_POINT('Ctrl Pts',(-17.9102782670879,48.370835484323,-38.2159783996089));
#27515=CARTESIAN_POINT('Ctrl Pts',(-17.4797286554972,49.1861297197598,-38.1642808510505));
#27516=CARTESIAN_POINT('Ctrl Pts',(-17.4784633668112,50.000273285299,-38.112583302492));
#27517=CARTESIAN_POINT('Origin',(-20.,50.,-32.));
#27518=CARTESIAN_POINT('Origin',(20.,50.,-25.));
#27519=CARTESIAN_POINT('',(17.2889091374855,49.9985242304765,-25.));
#27520=CARTESIAN_POINT('',(20.,50.,-25.));
#27521=CARTESIAN_POINT('Ctrl Pts',(17.2903182801745,49.9970484609529,-25.));
#27522=CARTESIAN_POINT('Ctrl Pts',(17.3003554510133,50.0895165684837,-25.));
#27523=CARTESIAN_POINT('Ctrl Pts',(17.3149872105963,50.1814113532663,-25.));
#27524=CARTESIAN_POINT('Ctrl Pts',(17.3341158855755,50.2723525936389,-25.));
#27525=CARTESIAN_POINT('Ctrl Pts',(17.3530415853084,50.3623288523453,-25.));
#27526=CARTESIAN_POINT('Ctrl Pts',(17.3763697243841,50.451372568364,-25.));
#27527=CARTESIAN_POINT('Ctrl Pts',(17.4040502467771,50.5390918450153,-25.));
#27528=CARTESIAN_POINT('Ctrl Pts',(17.4311163433268,50.6248640128022,-25.));
#27529=CARTESIAN_POINT('Ctrl Pts',(17.462344211455,50.7093705725007,-25.));
#27530=CARTESIAN_POINT('Ctrl Pts',(17.4977230419429,50.7922110937693,-25.));
#27531=CARTESIAN_POINT('Ctrl Pts',(17.5030373595978,50.8046547172202,-25.));
#27532=CARTESIAN_POINT('Ctrl Pts',(17.508445398048,50.8170606740681,-25.));
#27533=CARTESIAN_POINT('Ctrl Pts',(17.5139471830861,50.8294275242323,-25.));
#27534=CARTESIAN_POINT('Ctrl Pts',(17.5197445462543,50.8424587715735,-25.));
#27535=CARTESIAN_POINT('Ctrl Pts',(17.5256427668021,50.855439266843,-25.));
#27536=CARTESIAN_POINT('Ctrl Pts',(17.5316394080788,50.8683630331091,-25.));
#27537=CARTESIAN_POINT('Ctrl Pts',(17.5691316358145,50.949165063062,-25.));
#27538=CARTESIAN_POINT('Ctrl Pts',(17.6104933370969,51.0278095381119,-25.));
#27539=CARTESIAN_POINT('Ctrl Pts',(17.6556548012464,51.1039483466422,-25.));
#27540=CARTESIAN_POINT('Ctrl Pts',(17.7000564873693,51.1788062269566,-25.));
#27541=CARTESIAN_POINT('Ctrl Pts',(17.7481316148364,51.2512427099282,-25.));
#27542=CARTESIAN_POINT('Ctrl Pts',(17.7998501210591,51.3208927635814,-25.));
#27543=CARTESIAN_POINT('Ctrl Pts',(17.8499884667776,51.3884147924337,-25.));
#27544=CARTESIAN_POINT('Ctrl Pts',(17.9035514021835,51.4533185000313,-25.));
#27545=CARTESIAN_POINT('Ctrl Pts',(17.9605392204434,51.5152310005998,-25.));
#27546=CARTESIAN_POINT('Ctrl Pts',(17.9814440127658,51.5379423098947,-25.));
#27547=CARTESIAN_POINT('Ctrl Pts',(18.0028099126018,51.5602506790986,-25.));
#27548=CARTESIAN_POINT('Ctrl Pts',(18.0246377367992,51.5821361070304,-25.));
#27549=CARTESIAN_POINT('Ctrl Pts',(18.0437155989477,51.6012643157499,-25.));
#27550=CARTESIAN_POINT('Ctrl Pts',(18.0631463473053,51.62006941552,-25.));
#27551=CARTESIAN_POINT('Ctrl Pts',(18.0829198466036,51.6385462881155,-25.));
#27552=CARTESIAN_POINT('Origin',(20.,50.,-25.));
#27553=CARTESIAN_POINT('',(22.7115651190295,49.998177688036,-25.));
#27554=CARTESIAN_POINT('',(20.,50.,-25.));
#27555=CARTESIAN_POINT('Ctrl Pts',(22.710630238059,49.9963553760719,-25.));
#27556=CARTESIAN_POINT('Ctrl Pts',(22.7207573802718,49.904718898415,-25.));
#27557=CARTESIAN_POINT('Ctrl Pts',(22.7262776163321,49.8126183039993,-25.));
#27558=CARTESIAN_POINT('Ctrl Pts',(22.7270623951531,49.7204044776374,-25.));
#27559=CARTESIAN_POINT('Ctrl Pts',(22.7273484059302,49.6867973676626,-25.));
#27560=CARTESIAN_POINT('Ctrl Pts',(22.727004959792,49.653175122374,-25.));
#27561=CARTESIAN_POINT('Ctrl Pts',(22.7260241092612,49.6195545302368,-25.));
#27562=CARTESIAN_POINT('Ctrl Pts',(22.7254188474339,49.598807983854,-25.));
#27563=CARTESIAN_POINT('Ctrl Pts',(22.7245703770593,49.578055290145,-25.));
#27564=CARTESIAN_POINT('Ctrl Pts',(22.7234788618636,49.5573357485101,-25.));
#27565=CARTESIAN_POINT('Ctrl Pts',(22.7184418927117,49.46172215333,-25.));
#27566=CARTESIAN_POINT('Ctrl Pts',(22.7082329871324,49.3667044947841,-25.));
#27567=CARTESIAN_POINT('Ctrl Pts',(22.6927840010366,49.2726790977239,-25.));
#27568=CARTESIAN_POINT('Ctrl Pts',(22.6895875629464,49.2532249821753,-25.));
#27569=CARTESIAN_POINT('Ctrl Pts',(22.6861666387365,49.2338132767972,-25.));
#27570=CARTESIAN_POINT('Ctrl Pts',(22.6825203611591,49.2144474008277,-25.));
#27571=CARTESIAN_POINT('Ctrl Pts',(22.6655781463071,49.1244649942471,-25.));
#27572=CARTESIAN_POINT('Ctrl Pts',(22.6437749797271,49.0354721758651,-25.));
#27573=CARTESIAN_POINT('Ctrl Pts',(22.6174136918534,48.9477014940599,-25.));
#27574=CARTESIAN_POINT('Ctrl Pts',(22.590455165839,48.8579422903335,-25.));
#27575=CARTESIAN_POINT('Ctrl Pts',(22.5587294332582,48.7694605271934,-25.));
#27576=CARTESIAN_POINT('Ctrl Pts',(22.5225061276495,48.6825085791675,-25.));
#27577=CARTESIAN_POINT('Ctrl Pts',(22.5100294497312,48.6525590361409,-25.));
#27578=CARTESIAN_POINT('Ctrl Pts',(22.4970187421463,48.6227910672584,-25.));
#27579=CARTESIAN_POINT('Ctrl Pts',(22.4834836559862,48.5932153229631,-25.));
#27580=CARTESIAN_POINT('Ctrl Pts',(22.4768078375194,48.5786278798098,-25.));
#27581=CARTESIAN_POINT('Ctrl Pts',(22.4700044436617,48.5640872024162,-25.));
#27582=CARTESIAN_POINT('Ctrl Pts',(22.4630745736532,48.5495945909901,-25.));
#27583=CARTESIAN_POINT('Ctrl Pts',(22.4569730159819,48.5368342499856,-25.));
#27584=CARTESIAN_POINT('Ctrl Pts',(22.4507741704977,48.5241128967816,-25.));
#27585=CARTESIAN_POINT('Ctrl Pts',(22.4444842391951,48.5114418836784,-25.));
#27586=CARTESIAN_POINT('Ctrl Pts',(22.4016248337138,48.4251019759247,-25.));
#27587=CARTESIAN_POINT('Ctrl Pts',(22.3544763058254,48.3409633756465,-25.));
#27588=CARTESIAN_POINT('Ctrl Pts',(22.3033812187404,48.2592763321126,-25.));
#27589=CARTESIAN_POINT('Ctrl Pts',(22.2512764478704,48.1759750808731,-25.));
#27590=CARTESIAN_POINT('Ctrl Pts',(22.1950672860939,48.095222460128,-25.));
#27591=CARTESIAN_POINT('Ctrl Pts',(22.1350620407109,48.0172910149967,-25.));
#27592=CARTESIAN_POINT('Ctrl Pts',(22.0745784028941,47.9387382606202,-25.));
#27593=CARTESIAN_POINT('Ctrl Pts',(22.0102374503671,47.8630510071298,-25.));
#27594=CARTESIAN_POINT('Ctrl Pts',(21.9423056830507,47.7905278044699,-25.));
#27595=CARTESIAN_POINT('Ctrl Pts',(21.9053598556853,47.7510848482316,-25.));
#27596=CARTESIAN_POINT('Ctrl Pts',(21.8673510860636,47.7125781999077,-25.));
#27597=CARTESIAN_POINT('Ctrl Pts',(21.8283169663557,47.6750596468976,-25.));
#27598=CARTESIAN_POINT('Ctrl Pts',(21.8156599013896,47.662894014204,-25.));
#27599=CARTESIAN_POINT('Ctrl Pts',(21.8028950020426,47.6508322966046,-25.));
#27600=CARTESIAN_POINT('Ctrl Pts',(21.7900234751583,47.6388763339766,-25.));
#27601=CARTESIAN_POINT('Ctrl Pts',(21.7785389308687,47.6282086965192,-25.));
#27602=CARTESIAN_POINT('Ctrl Pts',(21.7669748807076,47.6176302985802,-25.));
#27603=CARTESIAN_POINT('Ctrl Pts',(21.7553377463642,47.6071469065118,-25.));
#27604=CARTESIAN_POINT('Ctrl Pts',(21.6795229583253,47.5388486361528,-25.));
#27605=CARTESIAN_POINT('Ctrl Pts',(21.6005419880646,47.4745177252953,-25.));
#27606=CARTESIAN_POINT('Ctrl Pts',(21.5187212121605,47.4144372276439,-25.));
#27607=CARTESIAN_POINT('Ctrl Pts',(21.4368280436309,47.3543035725284,-25.));
#27608=CARTESIAN_POINT('Ctrl Pts',(21.3520894649761,47.2984270171853,-25.));
#27609=CARTESIAN_POINT('Ctrl Pts',(21.2647877502657,47.2471175615949,-25.));
#27610=CARTESIAN_POINT('Ctrl Pts',(21.1792482856417,47.1968438255531,-25.));
#27611=CARTESIAN_POINT('Ctrl Pts',(21.0912474535113,47.1509539946296,-25.));
#27612=CARTESIAN_POINT('Ctrl Pts',(21.0010170240259,47.1097758121714,-25.));
#27613=CARTESIAN_POINT('Ctrl Pts',(20.9635971819417,47.0926986343979,-25.));
#27614=CARTESIAN_POINT('Ctrl Pts',(20.9257935259626,47.0764322950928,-25.));
#27615=CARTESIAN_POINT('Ctrl Pts',(20.8876212384296,47.0610024698252,-25.));
#27616=CARTESIAN_POINT('Ctrl Pts',(20.8571995126747,47.048705540742,-25.));
#27617=CARTESIAN_POINT('Ctrl Pts',(20.8265436358766,47.0369399483188,-25.));
#27618=CARTESIAN_POINT('Ctrl Pts',(20.7956658684167,47.0257030027424,-25.));
#27619=CARTESIAN_POINT('Ctrl Pts',(19.2062007174671,47.0307770462543,-25.));
#27620=CARTESIAN_POINT('Ctrl Pts',(19.1113557060478,47.0654717751014,-25.));
#27621=CARTESIAN_POINT('Ctrl Pts',(19.0185537598898,47.1051548199859,-25.));
#27622=CARTESIAN_POINT('Ctrl Pts',(18.9280360104757,47.1495064600839,-25.));
#27623=CARTESIAN_POINT('Ctrl Pts',(18.836253198687,47.1944779519955,-25.));
#27624=CARTESIAN_POINT('Ctrl Pts',(18.746818208596,47.2442501473846,-25.));
#27625=CARTESIAN_POINT('Ctrl Pts',(18.6600164517859,47.2985304009372,-25.));
#27626=CARTESIAN_POINT('Ctrl Pts',(18.6355002698107,47.3138612493285,-25.));
#27627=CARTESIAN_POINT('Ctrl Pts',(18.6111943852541,47.3295519227208,-25.));
#27628=CARTESIAN_POINT('Ctrl Pts',(18.5871058251638,47.3455962834916,-25.));
#27629=CARTESIAN_POINT('Ctrl Pts',(18.5677884079412,47.3584627898298,-25.));
#27630=CARTESIAN_POINT('Ctrl Pts',(18.5486086595491,47.3715583683707,-25.));
#27631=CARTESIAN_POINT('Ctrl Pts',(18.5295894598327,47.3848661134958,-25.));
#27632=CARTESIAN_POINT('Ctrl Pts',(18.4468808414566,47.4427373819723,-25.));
#27633=CARTESIAN_POINT('Ctrl Pts',(18.3671268101558,47.5046689052355,-25.));
#27634=CARTESIAN_POINT('Ctrl Pts',(18.2905938480462,47.5703640699442,-25.));
#27635=CARTESIAN_POINT('Ctrl Pts',(18.231599184729,47.6210045262486,-25.));
#27636=CARTESIAN_POINT('Ctrl Pts',(18.1745190969985,47.6738822270316,-25.));
#27637=CARTESIAN_POINT('Ctrl Pts',(18.1194932079197,47.7288730846741,-25.));
#27638=CARTESIAN_POINT('Ctrl Pts',(18.0902009127033,47.7581467313745,-25.));
#27639=CARTESIAN_POINT('Ctrl Pts',(18.0614910173884,47.7880193581185,-25.));
#27640=CARTESIAN_POINT('Ctrl Pts',(18.0333866071095,47.8184730778813,-25.));
#27641=CARTESIAN_POINT('Ctrl Pts',(18.0237499891656,47.8289152419193,-25.));
#27642=CARTESIAN_POINT('Ctrl Pts',(18.0141852981564,47.8394250112168,-25.));
#27643=CARTESIAN_POINT('Ctrl Pts',(18.0047000948839,47.8499940608166,-25.));
#27644=CARTESIAN_POINT('Ctrl Pts',(17.9389018416694,47.9233108872281,-25.));
#27645=CARTESIAN_POINT('Ctrl Pts',(17.8768356848677,47.9995741977793,-25.));
#27646=CARTESIAN_POINT('Ctrl Pts',(17.8187455012205,48.0785061517174,-25.));
#27647=CARTESIAN_POINT('Ctrl Pts',(17.7611817077828,48.1567228555884,-25.));
#27648=CARTESIAN_POINT('Ctrl Pts',(17.707521722539,48.2375608408771,-25.));
#27649=CARTESIAN_POINT('Ctrl Pts',(17.6580485957965,48.3207721465544,-25.));
#27650=CARTESIAN_POINT('Ctrl Pts',(17.6099912397688,48.4016021972458,-25.));
#27651=CARTESIAN_POINT('Ctrl Pts',(17.5658843324267,48.4846723754761,-25.));
#27652=CARTESIAN_POINT('Ctrl Pts',(17.5260350964086,48.5697657528252,-25.));
#27653=CARTESIAN_POINT('Ctrl Pts',(17.5052300089039,48.6141925810086,-25.));
#27654=CARTESIAN_POINT('Ctrl Pts',(17.4855863091861,48.659171009271,-25.));
#27655=CARTESIAN_POINT('Ctrl Pts',(17.4671534140155,48.7046704056706,-25.));
#27656=CARTESIAN_POINT('Ctrl Pts',(17.4600943600105,48.7220948359301,-25.));
#27657=CARTESIAN_POINT('Ctrl Pts',(17.4532129229748,48.7395956691933,-25.));
#27658=CARTESIAN_POINT('Ctrl Pts',(17.4465120404535,48.7571711764424,-25.));
#27659=CARTESIAN_POINT('Ctrl Pts',(17.441270606043,48.7709187489726,-25.));
#27660=CARTESIAN_POINT('Ctrl Pts',(17.4361395441369,48.784712508465,-25.));
#27661=CARTESIAN_POINT('Ctrl Pts',(17.4311253885978,48.798536919806,-25.));
#27662=CARTESIAN_POINT('Ctrl Pts',(17.3994429641943,48.8858877935106,-25.));
#27663=CARTESIAN_POINT('Ctrl Pts',(17.3723693458196,48.9746019981721,-25.));
#27664=CARTESIAN_POINT('Ctrl Pts',(17.3501558549811,49.0644566530551,-25.));
#27665=CARTESIAN_POINT('Ctrl Pts',(17.3451709794145,49.0846207180789,-25.));
#27666=CARTESIAN_POINT('Ctrl Pts',(17.340431057112,49.1048422545129,-25.));
#27667=CARTESIAN_POINT('Ctrl Pts',(17.335939289229,49.1251187994171,-25.));
#27668=CARTESIAN_POINT('Ctrl Pts',(17.3155161680488,49.217311972456,-25.));
#27669=CARTESIAN_POINT('Ctrl Pts',(17.300219006952,49.3106426726263,-25.));
#27670=CARTESIAN_POINT('Ctrl Pts',(17.2899369956297,49.4047153321239,-25.));
#27671=CARTESIAN_POINT('Ctrl Pts',(17.2792457471088,49.5025322037636,-25.));
#27672=CARTESIAN_POINT('Ctrl Pts',(17.2739768612926,49.6011525024422,-25.));
#27673=CARTESIAN_POINT('Ctrl Pts',(17.2740630915786,49.7001168903436,-25.));
#27674=CARTESIAN_POINT('Ctrl Pts',(17.2740904232784,49.731484812998,-25.));
#27675=CARTESIAN_POINT('Ctrl Pts',(17.2746561692793,49.7628871202482,-25.));
#27676=CARTESIAN_POINT('Ctrl Pts',(17.2757593065841,49.7943085770565,-25.));
#27677=CARTESIAN_POINT('Ctrl Pts',(17.2762349624895,49.8078570278432,-25.));
#27678=CARTESIAN_POINT('Ctrl Pts',(17.2768106643348,49.8214115392031,-25.));
#27679=CARTESIAN_POINT('Ctrl Pts',(17.27748594917,49.8349628018775,-25.));
#27680=CARTESIAN_POINT('Ctrl Pts',(17.280185572062,49.889137421273,-25.));
#27681=CARTESIAN_POINT('Ctrl Pts',(17.2844721284628,49.9431903973805,-25.));
#27682=CARTESIAN_POINT('Ctrl Pts',(17.2903182801745,49.9970484609529,-25.));
#27683=CARTESIAN_POINT('',(20.,50.,-25.));
#27684=CARTESIAN_POINT('Origin',(20.,50.,-25.));
#27685=CARTESIAN_POINT('Origin',(20.,50.,-25.));
#27686=CARTESIAN_POINT('',(20.,50.,-25.));
#27687=CARTESIAN_POINT('Ctrl Pts',(21.9134659966651,51.6359872033749,-25.));
#27688=CARTESIAN_POINT('Ctrl Pts',(21.9760669584728,51.57715767109,-25.));
#27689=CARTESIAN_POINT('Ctrl Pts',(22.0352443081274,51.5150279920012,-25.));
#27690=CARTESIAN_POINT('Ctrl Pts',(22.0909852410533,51.449982471831,-25.));
#27691=CARTESIAN_POINT('Ctrl Pts',(22.1343869490307,51.3993359088211,-25.));
#27692=CARTESIAN_POINT('Ctrl Pts',(22.1757048720029,51.346920405304,-25.));
#27693=CARTESIAN_POINT('Ctrl Pts',(22.2149216400472,51.2928987320259,-25.));
#27694=CARTESIAN_POINT('Ctrl Pts',(22.238544542541,51.2603578373004,-25.));
#27695=CARTESIAN_POINT('Ctrl Pts',(22.2614048485299,51.2272338518059,-25.));
#27696=CARTESIAN_POINT('Ctrl Pts',(22.2834967784221,51.1935599636263,-25.));
#27697=CARTESIAN_POINT('Ctrl Pts',(22.2954179674691,51.1753889487401,-25.));
#27698=CARTESIAN_POINT('Ctrl Pts',(22.3071167276197,51.1570553689352,-25.));
#27699=CARTESIAN_POINT('Ctrl Pts',(22.3185794803464,51.1385851146828,-25.));
#27700=CARTESIAN_POINT('Ctrl Pts',(22.3655670889394,51.0628726660144,-25.));
#27701=CARTESIAN_POINT('Ctrl Pts',(22.408638498604,50.9847977644774,-25.));
#27702=CARTESIAN_POINT('Ctrl Pts',(22.4477592672363,50.9047425113829,-25.));
#27703=CARTESIAN_POINT('Ctrl Pts',(22.4825528251087,50.8335422978156,-25.));
#27704=CARTESIAN_POINT('Ctrl Pts',(22.5142211416441,50.7607746036135,-25.));
#27705=CARTESIAN_POINT('Ctrl Pts',(22.5427166787335,50.686684346716,-25.));
#27706=CARTESIAN_POINT('Ctrl Pts',(22.5500219910964,50.667690057611,-25.));
#27707=CARTESIAN_POINT('Ctrl Pts',(22.5571186539646,50.6486087488088,-25.));
#27708=CARTESIAN_POINT('Ctrl Pts',(22.5640056073642,50.6294443637264,-25.));
#27709=CARTESIAN_POINT('Ctrl Pts',(22.5692938298803,50.6147287809691,-25.));
#27710=CARTESIAN_POINT('Ctrl Pts',(22.5744584523851,50.5999638327569,-25.));
#27711=CARTESIAN_POINT('Ctrl Pts',(22.5794944484737,50.5851652200462,-25.));
#27712=CARTESIAN_POINT('Ctrl Pts',(22.6091525619276,50.4980128619004,-25.));
#27713=CARTESIAN_POINT('Ctrl Pts',(22.6343958352894,50.4095773703735,-25.));
#27714=CARTESIAN_POINT('Ctrl Pts',(22.6551922384222,50.3202540828574,-25.));
#27715=CARTESIAN_POINT('Ctrl Pts',(22.6763398077743,50.2294224902284,-25.));
#27716=CARTESIAN_POINT('Ctrl Pts',(22.6928895667938,50.137672075038,-25.));
#27717=CARTESIAN_POINT('Ctrl Pts',(22.704766333404,50.0453852273788,-25.));
#27718=CARTESIAN_POINT('Ctrl Pts',(22.7068675349265,50.0290581182278,-25.));
#27719=CARTESIAN_POINT('Ctrl Pts',(22.7088223589801,50.012714154031,-25.));
#27720=CARTESIAN_POINT('Ctrl Pts',(22.710630238059,49.9963553760719,-25.));
#27721=CARTESIAN_POINT('Origin',(20.,50.,-42.2084234471774));
#27722=CARTESIAN_POINT('Ctrl Pts',(23.0767446582541,50.0019103494728,-39.7084234471775));
#27723=CARTESIAN_POINT('Ctrl Pts',(23.0776698137548,50.1251794436804,-39.7020198504182));
#27724=CARTESIAN_POINT('Ctrl Pts',(23.0151644123476,51.2610383915795,-39.642966745928));
#27725=CARTESIAN_POINT('Ctrl Pts',(21.6024147148416,53.2535259157778,-39.5312641337071));
#27726=CARTESIAN_POINT('Ctrl Pts',(18.1518494020808,53.1200733432643,-39.3733156105146));
#27727=CARTESIAN_POINT('Ctrl Pts',(16.376977963313,50.1582350183397,-39.2153670873222));
#27728=CARTESIAN_POINT('Ctrl Pts',(17.8869743722217,47.0526837548,-39.0574185641297));
#27729=CARTESIAN_POINT('Ctrl Pts',(21.3127949123184,46.6194980929628,-38.8994700409373));
#27730=CARTESIAN_POINT('Ctrl Pts',(22.9593110635881,48.5578259751719,-38.7831383352865));
#27731=CARTESIAN_POINT('Ctrl Pts',(23.076186491933,49.7844436463546,-38.7194561373665));
#27732=CARTESIAN_POINT('Ctrl Pts',(23.074254699799,49.9973154728993,-38.7084234471775));
#27733=CARTESIAN_POINT('Ctrl Pts',(23.0703066071761,49.9966560053347,-39.7915765528225));
#27734=CARTESIAN_POINT('Ctrl Pts',(23.0652969469962,50.6897753512944,-39.7557520197534));
#27735=CARTESIAN_POINT('Ctrl Pts',(22.4928178620874,52.4114019306593,-39.6672779789534));
#27736=CARTESIAN_POINT('Ctrl Pts',(19.6484751064271,53.6086153775441,-39.5261544304226));
#27737=CARTESIAN_POINT('Ctrl Pts',(16.7861446928906,51.6798052066136,-39.3682059072302));
#27738=CARTESIAN_POINT('Ctrl Pts',(16.8365147494583,48.2264371981741,-39.2102573840376));
#27739=CARTESIAN_POINT('Ctrl Pts',(19.7557254495835,46.3818721760905,-39.0523088608452));
#27740=CARTESIAN_POINT('Ctrl Pts',(22.5305076755622,47.6502487962456,-38.9127485837735));
#27741=CARTESIAN_POINT('Ctrl Pts',(23.0660295697572,49.3389604422763,-38.8258378144326));
#27742=CARTESIAN_POINT('Ctrl Pts',(23.0703815974152,50.0021496035415,-38.7915765528225));
#27743=CARTESIAN_POINT('Ctrl Pts',(18.086534003335,51.635987203375,-40.));
#27744=CARTESIAN_POINT('Ctrl Pts',(17.5453386170133,51.0029999971535,-39.9473504922692));
#27745=CARTESIAN_POINT('Ctrl Pts',(17.1495677130931,49.1684301437675,-39.8420514768075));
#27746=CARTESIAN_POINT('Ctrl Pts',(19.1409892366488,47.1546688770413,-39.6841029536151));
#27747=CARTESIAN_POINT('Ctrl Pts',(21.9115813032277,47.7272070111674,-39.5261544304226));
#27748=CARTESIAN_POINT('Ctrl Pts',(22.9488012025699,50.3572336945348,-39.3682059072301));
#27749=CARTESIAN_POINT('Ctrl Pts',(21.3125358856723,52.6649590021054,-39.2102573840377));
#27750=CARTESIAN_POINT('Ctrl Pts',(18.4861821603183,52.5556481671279,-39.0523088608452));
#27751=CARTESIAN_POINT('Ctrl Pts',(17.0323871881049,50.1296101053101,-38.8943603376527));
#27752=CARTESIAN_POINT('Ctrl Pts',(18.2692233551548,47.5858569554934,-38.7364118144602));
#27753=CARTESIAN_POINT('Ctrl Pts',(21.0753086682159,47.2310351225099,-38.5784632912678));
#27754=CARTESIAN_POINT('Ctrl Pts',(22.9064409998485,49.3866986741128,-38.4205147680753));
#27755=CARTESIAN_POINT('Ctrl Pts',(22.102393338019,52.098449431005,-38.2625662448829));
#27756=CARTESIAN_POINT('Ctrl Pts',(19.3921687412977,52.9075870780541,-38.1046177216904));
#27757=CARTESIAN_POINT('Ctrl Pts',(17.2330466807883,51.0805103975822,-37.9466691984979));
#27758=CARTESIAN_POINT('Ctrl Pts',(17.5826368306021,48.2737645639559,-37.7887206753054));
#27759=CARTESIAN_POINT('Ctrl Pts',(20.123976751384,47.0321455255811,-37.630772152113));
#27760=CARTESIAN_POINT('Ctrl Pts',(22.5529106689962,48.4813890589392,-37.4728236289205));
#27761=CARTESIAN_POINT('Ctrl Pts',(22.6671981530575,51.3075113564941,-37.314875105728));
#27762=CARTESIAN_POINT('Ctrl Pts',(20.3632181774645,52.948152667123,-37.1569265825356));
#27763=CARTESIAN_POINT('Ctrl Pts',(17.7299193338982,51.9157937220368,-36.9989780593431));
#27764=CARTESIAN_POINT('Ctrl Pts',(17.154833585512,49.1464428233941,-36.8410295361507));
#27765=CARTESIAN_POINT('Ctrl Pts',(19.159373695021,47.1509862831415,-36.6830810129581));
#27766=CARTESIAN_POINT('Ctrl Pts',(21.9260841079052,47.7386438180038,-36.5251324897658));
#27767=CARTESIAN_POINT('Ctrl Pts',(22.9464726397818,50.3766042336357,-36.3671839665732));
#27768=CARTESIAN_POINT('Ctrl Pts',(21.2953840418668,52.6731090412184,-36.2092354433808));
#27769=CARTESIAN_POINT('Ctrl Pts',(18.4698101306244,52.5459871817283,-36.0512869201882));
#27770=CARTESIAN_POINT('Ctrl Pts',(17.0316128352692,50.1104961764295,-35.8933383969959));
#27771=CARTESIAN_POINT('Ctrl Pts',(18.2847619027881,47.574821648971,-35.7353898738033));
#27772=CARTESIAN_POINT('Ctrl Pts',(21.0930651864267,47.2379825737144,-35.5774413506109));
#27773=CARTESIAN_POINT('Ctrl Pts',(22.910319509614,49.4053806960139,-35.4194928274184));
#27774=CARTESIAN_POINT('Ctrl Pts',(22.0888756467976,52.1119020566559,-35.261544304226));
#27775=CARTESIAN_POINT('Ctrl Pts',(19.3735117653125,52.9036260531522,-35.1035957810335));
#27776=CARTESIAN_POINT('Ctrl Pts',(17.2261657124394,51.0627206170365,-34.945647257841));
#27777=CARTESIAN_POINT('Ctrl Pts',(17.5937708457415,48.258278718647,-34.7876987346485));
#27778=CARTESIAN_POINT('Ctrl Pts',(20.143030771058,47.0330025339987,-34.6297502114561));
#27779=CARTESIAN_POINT('Ctrl Pts',(22.5626090463406,48.4978127146266,-34.4718016882636));
#27780=CARTESIAN_POINT('Ctrl Pts',(22.6587476375371,51.3246104199406,-34.3138531650712));
#27781=CARTESIAN_POINT('Ctrl Pts',(20.3442806079329,52.9504241436998,-34.1559046418787));
#27782=CARTESIAN_POINT('Ctrl Pts',(17.7176648219373,51.9011780294602,-33.9979561186862));
#27783=CARTESIAN_POINT('Ctrl Pts',(17.1603729278045,49.1281916176252,-33.8400075954937));
#27784=CARTESIAN_POINT('Ctrl Pts',(19.1776845366779,47.145647351236,-33.6820590723013));
#27785=CARTESIAN_POINT('Ctrl Pts',(21.9405645665512,47.7510578202695,-33.5241105491088));
#27786=CARTESIAN_POINT('Ctrl Pts',(22.9439937235359,50.3955157651801,-33.3661620259163));
#27787=CARTESIAN_POINT('Ctrl Pts',(21.2781933089123,52.6813715948702,-33.2082135027239));
#27788=CARTESIAN_POINT('Ctrl Pts',(18.4534938955901,52.5361093497221,-33.0502649795314));
#27789=CARTESIAN_POINT('Ctrl Pts',(17.0309645322794,50.0914338894602,-32.8923164563389));
#27790=CARTESIAN_POINT('Ctrl Pts',(18.300369328419,47.5638581024608,-32.7343679331465));
#27791=CARTESIAN_POINT('Ctrl Pts',(21.1107775625509,47.2450580820535,-32.576419409954));
#27792=CARTESIAN_POINT('Ctrl Pts',(22.9140775634904,49.4240801108775,-32.4184708867615));
#27793=CARTESIAN_POINT('Ctrl Pts',(22.0752720652759,52.1252711873571,-32.260522363569));
#27794=CARTESIAN_POINT('Ctrl Pts',(19.3548805020225,52.8995435154614,-32.1025738403766));
#27795=CARTESIAN_POINT('Ctrl Pts',(17.2193991671627,51.0448879237265,-31.9446253171841));
#27796=CARTESIAN_POINT('Ctrl Pts',(17.605004039285,48.2428642303784,-31.7866767939917));
#27797=CARTESIAN_POINT('Ctrl Pts',(20.162078908478,47.0339820984776,-31.6287282707991));
#27798=CARTESIAN_POINT('Ctrl Pts',(22.5722017607613,48.5142981905304,-31.4707797476067));
#27799=CARTESIAN_POINT('Ctrl Pts',(22.6501875065425,51.3416549276512,-31.3128312244142));
#27800=CARTESIAN_POINT('Ctrl Pts',(20.3253288419512,52.9525739464609,-31.1548827012218));
#27801=CARTESIAN_POINT('Ctrl Pts',(17.7055044107922,51.8864839664918,-30.9969341780293));
#27802=CARTESIAN_POINT('Ctrl Pts',(17.1660293464391,49.1099763489209,-30.8389856548369));
#27803=CARTESIAN_POINT('Ctrl Pts',(19.1960292823484,47.1404261069377,-30.6810371316443));
#27804=CARTESIAN_POINT('Ctrl Pts',(21.9549650162884,47.7635645437854,-30.5230886084519));
#27805=CARTESIAN_POINT('Ctrl Pts',(22.9413934275329,50.4144109906734,-30.3651400852594));
#27806=CARTESIAN_POINT('Ctrl Pts',(21.2609498764708,52.6895235960579,-30.207191562067));
#27807=CARTESIAN_POINT('Ctrl Pts',(18.437241422469,52.5261269550601,-30.0492430388745));
#27808=CARTESIAN_POINT('Ctrl Pts',(17.030438641562,50.0723678325863,-29.891294515682));
#27809=CARTESIAN_POINT('Ctrl Pts',(18.3160468292225,47.5529949972773,-29.7333459924896));
#27810=CARTESIAN_POINT('Ctrl Pts',(21.1284441417105,47.2522471756388,-29.5753974692971));
#27811=CARTESIAN_POINT('Ctrl Pts',(22.9177154709785,49.4428032707346,-29.4174489461046));
#27812=CARTESIAN_POINT('Ctrl Pts',(22.0615829210316,52.1385526938618,-29.2595004229121));
#27813=CARTESIAN_POINT('Ctrl Pts',(19.3362758367626,52.8953414306466,-29.1015518997197));
#27814=CARTESIAN_POINT('Ctrl Pts',(17.2127472651087,51.0270121500097,-28.9436033765272));
#27815=CARTESIAN_POINT('Ctrl Pts',(17.61633597759,48.2275221882877,-28.7856548533347));
#27816=CARTESIAN_POINT('Ctrl Pts',(20.1811203635866,47.0350839506389,-28.6277063301423));
#27817=CARTESIAN_POINT('Ctrl Pts',(22.5816884239278,48.5308449217582,-28.4697578069498));
#27818=CARTESIAN_POINT('Ctrl Pts',(22.6415181098295,51.358644118678,-28.3118092837574));
#27819=CARTESIAN_POINT('Ctrl Pts',(20.3063636616365,52.9546020170924,-28.1538607605649));
#27820=CARTESIAN_POINT('Ctrl Pts',(17.6934386031563,51.8717121215775,-27.9959122373724));
#27821=CARTESIAN_POINT('Ctrl Pts',(17.1718026041603,49.0917977813112,-27.8379637141799));
#27822=CARTESIAN_POINT('Ctrl Pts',(19.2144071844416,47.1353227504398,-27.6800151909875));
#27823=CARTESIAN_POINT('Ctrl Pts',(21.9692848456041,47.7761634974712,-27.522066667795));
#27824=CARTESIAN_POINT('Ctrl Pts',(22.9386718945708,50.4332890849004,-27.3641181446025));
#27825=CARTESIAN_POINT('Ctrl Pts',(21.2436543845446,52.6975647992193,-27.2061696214101));
#27826=CARTESIAN_POINT('Ctrl Pts',(18.421053522611,52.5160402297565,-27.0482210982176));
#27827=CARTESIAN_POINT('Ctrl Pts',(17.03003490355,50.053299149001,-26.8902725750251));
#27828=CARTESIAN_POINT('Ctrl Pts',(18.3317943187318,47.5422320705639,-26.7323240518327));
#27829=CARTESIAN_POINT('Ctrl Pts',(21.1460630808652,47.2595509728877,-26.5743755286402));
#27830=CARTESIAN_POINT('Ctrl Pts',(22.9212353010978,49.4615465871111,-26.4164270054477));
#27831=CARTESIAN_POINT('Ctrl Pts',(22.0478043609502,52.1517516355771,-26.2584784822553));
#27832=CARTESIAN_POINT('Ctrl Pts',(19.3177073307994,52.8910088097876,-26.1005299590628));
#27833=CARTESIAN_POINT('Ctrl Pts',(17.206192773396,51.0091162540841,-25.9425814358703));
#27834=CARTESIAN_POINT('Ctrl Pts',(17.6278010459406,48.2122089878618,-25.7846329126778));
#27835=CARTESIAN_POINT('Ctrl Pts',(20.2000849682644,47.0363961109221,-25.6266843894854));
#27836=CARTESIAN_POINT('Ctrl Pts',(22.5912067713758,48.5472769011073,-25.4687358662929));
#27837=CARTESIAN_POINT('Ctrl Pts',(22.6324648056073,51.3759264122866,-25.3107873431004));
#27838=CARTESIAN_POINT('Ctrl Pts',(20.287933589965,52.9558121213478,-25.152838819908));
#27839=CARTESIAN_POINT('Ctrl Pts',(17.6803739092466,51.8582635684763,-24.9948902967155));
#27840=CARTESIAN_POINT('Ctrl Pts',(17.1799175193219,49.0706951790677,-24.836941773523));
#27841=CARTESIAN_POINT('Ctrl Pts',(18.5452496035378,47.7830036573307,-24.7316427580614));
#27842=CARTESIAN_POINT('Ctrl Pts',(19.3498000020249,47.5679131979649,-24.6789932503306));
#27843=CARTESIAN_POINT('Ctrl Pts',(17.9456684496579,51.7564253212269,-40.1070022498898));
#27844=CARTESIAN_POINT('Ctrl Pts',(17.3646313374449,51.0768388582481,-40.054352742159));
#27845=CARTESIAN_POINT('Ctrl Pts',(16.9397245682378,49.1072116280355,-39.9490537266973));
#27846=CARTESIAN_POINT('Ctrl Pts',(19.0777505760168,46.9452012697107,-39.7911052035049));
#27847=CARTESIAN_POINT('Ctrl Pts',(22.0523081095296,47.5598885203642,-39.6331566803124));
#27848=CARTESIAN_POINT('Ctrl Pts',(23.1658860709749,50.3835325272606,-39.47520815712));
#27849=CARTESIAN_POINT('Ctrl Pts',(21.4091621620621,52.8611479733296,-39.3172596339275));
#27850=CARTESIAN_POINT('Ctrl Pts',(18.3747379075725,52.7437898925067,-39.159311110735));
#27851=CARTESIAN_POINT('Ctrl Pts',(16.8139174465076,50.1391517429866,-39.0013625875426));
#27852=CARTESIAN_POINT('Ctrl Pts',(18.1418070275104,47.4081325552623,-38.84341406435));
#27853=CARTESIAN_POINT('Ctrl Pts',(21.1544707495834,47.0271894459942,-38.6854655411577));
#27854=CARTESIAN_POINT('Ctrl Pts',(23.1204073945411,49.3415486526373,-38.5275170179651));
#27855=CARTESIAN_POINT('Ctrl Pts',(22.2571673460876,52.2529330964984,-38.3695684947727));
#27856=CARTESIAN_POINT('Ctrl Pts',(19.3474214152682,53.1216378447405,-38.2116199715801));
#27857=CARTESIAN_POINT('Ctrl Pts',(17.0293490911846,51.1600554199,-38.0536714483878));
#27858=CARTESIAN_POINT('Ctrl Pts',(17.4046753711933,48.1466825510542,-37.8957229251952));
#27859=CARTESIAN_POINT('Ctrl Pts',(20.1331036727703,46.8136579932703,-37.7377744020028));
#27860=CARTESIAN_POINT('Ctrl Pts',(22.7408508652176,48.3695919476212,-37.5798258788103));
#27861=CARTESIAN_POINT('Ctrl Pts',(22.8635519661128,51.4037677370582,-37.4218773556178));
#27862=CARTESIAN_POINT('Ctrl Pts',(20.3899575758982,53.1651897916408,-37.2639288324254));
#27863=CARTESIAN_POINT('Ctrl Pts',(17.5628005188895,52.0568306382172,-37.1059803092329));
#27864=CARTESIAN_POINT('Ctrl Pts',(16.9453781036908,49.0836056449508,-36.9480317860405));
#27865=CARTESIAN_POINT('Ctrl Pts',(19.0974884615793,46.9412475705864,-36.790083262848));
#27866=CARTESIAN_POINT('Ctrl Pts',(22.0678785817874,47.5721672821295,-36.6321347396555));
#27867=CARTESIAN_POINT('Ctrl Pts',(23.1633860840345,50.4043290868502,-36.474186216463));
#27868=CARTESIAN_POINT('Ctrl Pts',(21.3907476336944,52.8698980020813,-36.3162376932706));
#27869=CARTESIAN_POINT('Ctrl Pts',(18.3571606016773,52.7334176846136,-36.1582891700781));
#27870=CARTESIAN_POINT('Ctrl Pts',(16.8130860873592,50.1186306847505,-36.0003406468856));
#27871=CARTESIAN_POINT('Ctrl Pts',(18.1584894920566,47.396284851464,-35.8423921236932));
#27872=CARTESIAN_POINT('Ctrl Pts',(21.1735344672812,47.034648354712,-35.6844436005007));
#27873=CARTESIAN_POINT('Ctrl Pts',(23.1245714324667,49.3616060077629,-35.5264950773082));
#27874=CARTESIAN_POINT('Ctrl Pts',(22.2426545093755,52.2673760776425,-35.3685465541158));
#27875=CARTESIAN_POINT('Ctrl Pts',(19.3273909498889,53.1173852170784,-35.2105980309233));
#27876=CARTESIAN_POINT('Ctrl Pts',(17.0219615596577,51.1409559911606,-35.0526495077308));
#27877=CARTESIAN_POINT('Ctrl Pts',(17.4166290503403,48.1300566686725,-34.8947009845384));
#27878=CARTESIAN_POINT('Ctrl Pts',(20.1535604114034,46.8145780929399,-34.7367524613459));
#27879=CARTESIAN_POINT('Ctrl Pts',(22.7512632177759,48.3872246801124,-34.5788039381534));
#27880=CARTESIAN_POINT('Ctrl Pts',(22.8544793404793,51.4221255994822,-34.420855414961));
#27881=CARTESIAN_POINT('Ctrl Pts',(20.3696258602349,53.1676284897966,-34.2629068917685));
#27882=CARTESIAN_POINT('Ctrl Pts',(17.5496438541779,52.0411389674781,-34.104958368576));
#27883=CARTESIAN_POINT('Ctrl Pts',(16.9513252413244,49.0640108217826,-33.9470098453835));
#27884=CARTESIAN_POINT('Ctrl Pts',(19.1171473109107,46.9355155971529,-33.7890613221911));
#27885=CARTESIAN_POINT('Ctrl Pts',(22.0834250629434,47.5854951785045,-33.6311127989986));
#27886=CARTESIAN_POINT('Ctrl Pts',(23.1607246749144,50.4246328476615,-33.4731642758061));
#27887=CARTESIAN_POINT('Ctrl Pts',(21.3722913532361,52.8787688284681,-33.3152157526137));
#27888=CARTESIAN_POINT('Ctrl Pts',(18.3396431979335,52.7228126662988,-33.1572672294212));
#27889=CARTESIAN_POINT('Ctrl Pts',(16.8123900575951,50.0981650702003,-32.9993187062287));
#27890=CARTESIAN_POINT('Ctrl Pts',(18.1752459052613,47.3845141905069,-32.8413701830363));
#27891=CARTESIAN_POINT('Ctrl Pts',(21.1925507932399,47.0422447478757,-32.6834216598438));
#27892=CARTESIAN_POINT('Ctrl Pts',(23.1286061467808,49.381682036286,-32.5254731366513));
#27893=CARTESIAN_POINT('Ctrl Pts',(22.2280494592902,52.281729417105,-32.3675246134589));
#27894=CARTESIAN_POINT('Ctrl Pts',(19.3073880901224,53.1130021310981,-32.2095760902664));
#27895=CARTESIAN_POINT('Ctrl Pts',(17.0146968748016,51.1218104905046,-32.0516275670739));
#27896=CARTESIAN_POINT('Ctrl Pts',(17.4286892092078,48.1135073964944,-31.8936790438815));
#27897=CARTESIAN_POINT('Ctrl Pts',(20.1740108347427,46.8156297710037,-31.735730520689));
#27898=CARTESIAN_POINT('Ctrl Pts',(22.7615621287167,48.4049237839014,-31.5777819974965));
#27899=CARTESIAN_POINT('Ctrl Pts',(22.8452890296988,51.4404248898854,-31.4198334743041));
#27900=CARTESIAN_POINT('Ctrl Pts',(20.3492789030071,53.1699365567532,-31.2618849511116));
#27901=CARTESIAN_POINT('Ctrl Pts',(17.5365882177965,52.025363156875,-31.1039364279191));
#27902=CARTESIAN_POINT('Ctrl Pts',(16.9573980742272,49.0444545812943,-30.9459879047267));
#27903=CARTESIAN_POINT('Ctrl Pts',(19.1368425602015,46.9299099752538,-30.7880393815342));
#27904=CARTESIAN_POINT('Ctrl Pts',(22.0988856450943,47.5989226220833,-30.6300908583417));
#27905=CARTESIAN_POINT('Ctrl Pts',(23.1579329503013,50.4449191020027,-30.4721423351493));
#27906=CARTESIAN_POINT('Ctrl Pts',(21.3537784936595,52.8875209637386,-30.3141938119568));
#27907=CARTESIAN_POINT('Ctrl Pts',(18.3221942501278,52.7120953876339,-30.1562452887643));
#27908=CARTESIAN_POINT('Ctrl Pts',(16.8118254518511,50.0776954082126,-29.9982967655718));
#27909=CARTESIAN_POINT('Ctrl Pts',(18.192077552433,47.372851365167,-29.8403482423794));
#27910=CARTESIAN_POINT('Ctrl Pts',(21.2115179507527,47.0499630882047,-29.6823997191869));
#27911=CARTESIAN_POINT('Ctrl Pts',(23.1325118697688,49.4017835578618,-29.5244511959945));
#27912=CARTESIAN_POINT('Ctrl Pts',(22.2133525475253,52.2959886816523,-29.3665026728019));
#27913=CARTESIAN_POINT('Ctrl Pts',(19.2874137864799,53.1084906971728,-29.2085541496095));
#27914=CARTESIAN_POINT('Ctrl Pts',(17.0075552729738,51.1026187379482,-29.050605626417));
#27915=CARTESIAN_POINT('Ctrl Pts',(17.4408553822296,48.0970359038373,-28.8926571032246));
#27916=CARTESIAN_POINT('Ctrl Pts',(20.1944540838321,46.8168127393254,-28.7347085800321));
#27917=CARTESIAN_POINT('Ctrl Pts',(22.7717471811213,48.4226886525094,-28.5767600568397));
#27918=CARTESIAN_POINT('Ctrl Pts',(22.8359814092754,51.4586647913009,-28.4188115336471));
#27919=CARTESIAN_POINT('Ctrl Pts',(20.3289175439099,53.1721139299031,-28.2608630104547));
#27920=CARTESIAN_POINT('Ctrl Pts',(17.5236341494462,52.0095038381744,-28.1029144872622));
#27921=CARTESIAN_POINT('Ctrl Pts',(16.9635963476774,49.024937743762,-27.9449659640698));
#27922=CARTESIAN_POINT('Ctrl Pts',(19.1565734068249,46.9244309198201,-27.7870174408773));
#27923=CARTESIAN_POINT('Ctrl Pts',(22.1142596717088,47.6124490856331,-27.6290689176848));
#27924=CARTESIAN_POINT('Ctrl Pts',(23.1550110635058,50.4651869639081,-27.4711203944923));
#27925=CARTESIAN_POINT('Ctrl Pts',(21.3352097420827,52.8961541442528,-27.3131718712999));
#27926=CARTESIAN_POINT('Ctrl Pts',(18.3048146293401,52.7012660977134,-27.1552233481074));
#27927=CARTESIAN_POINT('Ctrl Pts',(16.8113919914512,50.0572229261403,-26.9972748249149));
#27928=CARTESIAN_POINT('Ctrl Pts',(18.2089843407397,47.3612960932364,-26.8393263017225));
#27929=CARTESIAN_POINT('Ctrl Pts',(21.2304339610984,47.0578045764528,-26.68137777853));
#27930=CARTESIAN_POINT('Ctrl Pts',(23.1362908227675,49.4219067198399,-26.5234292553375));
#27931=CARTESIAN_POINT('Ctrl Pts',(22.1985596373075,52.3101593031548,-26.3654807321451));
#27932=CARTESIAN_POINT('Ctrl Pts',(19.2674783041096,53.1038391173999,-26.2075322089526));
#27933=CARTESIAN_POINT('Ctrl Pts',(17.0005182526424,51.083405381826,-26.0495836857601));
#27934=CARTESIAN_POINT('Ctrl Pts',(17.4531644860655,48.0805953761109,-25.8916351625676));
#27935=CARTESIAN_POINT('Ctrl Pts',(20.2148148249151,46.818221498234,-25.7336866393752));
#27936=CARTESIAN_POINT('Ctrl Pts',(22.7819662503411,48.4403303214338,-25.5757381161827));
#27937=CARTESIAN_POINT('Ctrl Pts',(22.8262616188369,51.4772193729263,-25.4177895929902));
#27938=CARTESIAN_POINT('Ctrl Pts',(20.3091306870879,53.1734131196224,-25.2598410697978));
#27939=CARTESIAN_POINT('Ctrl Pts',(17.5096076588051,51.995065229393,-25.1018925466053));
#27940=CARTESIAN_POINT('Ctrl Pts',(16.9723086667225,49.0022816099927,-24.9439440234128));
#27941=CARTESIAN_POINT('Ctrl Pts',(18.438153778257,47.6197928044311,-24.8386450079512));
#27942=CARTESIAN_POINT('Ctrl Pts',(19.301933573839,47.3888678140614,-24.7859955002204));
#27943=CARTESIAN_POINT('Ctrl Pts',(17.8048028959809,51.8768634390788,-40.2140044997796));
#27944=CARTESIAN_POINT('Ctrl Pts',(17.1839240578764,51.1506777193428,-40.1613549920488));
#27945=CARTESIAN_POINT('Ctrl Pts',(16.7298814233824,49.0459931123036,-40.0560559765871));
#27946=CARTESIAN_POINT('Ctrl Pts',(19.0145119153848,46.7357336623799,-39.8981074533947));
#27947=CARTESIAN_POINT('Ctrl Pts',(22.1930349158314,47.392570029561,-39.7401589302022));
#27948=CARTESIAN_POINT('Ctrl Pts',(23.3829709393799,50.4098313599865,-39.5822104070097));
#27949=CARTESIAN_POINT('Ctrl Pts',(21.5057884384518,53.0573369445537,-39.4242618838173));
#27950=CARTESIAN_POINT('Ctrl Pts',(18.2632936548267,52.9319316178855,-39.2663133606248));
#27951=CARTESIAN_POINT('Ctrl Pts',(16.5954477049103,50.1486933806631,-39.1083648374324));
#27952=CARTESIAN_POINT('Ctrl Pts',(18.014390699866,47.2304081550311,-38.9504163142398));
#27953=CARTESIAN_POINT('Ctrl Pts',(21.2336328309509,46.8233437694785,-38.7924677910474));
#27954=CARTESIAN_POINT('Ctrl Pts',(23.3343737892337,49.2963986311619,-38.6345192678549));
#27955=CARTESIAN_POINT('Ctrl Pts',(22.4119413541563,52.4074167619917,-38.4765707446625));
#27956=CARTESIAN_POINT('Ctrl Pts',(19.3026740892386,53.3356886114267,-38.31862222147));
#27957=CARTESIAN_POINT('Ctrl Pts',(16.8256515015809,51.2396004422179,-38.1606736982775));
#27958=CARTESIAN_POINT('Ctrl Pts',(17.2267139117844,48.0196005381524,-38.0027251750851));
#27959=CARTESIAN_POINT('Ctrl Pts',(20.1422305941565,46.5951704609596,-37.8447766518926));
#27960=CARTESIAN_POINT('Ctrl Pts',(22.9287910614389,48.257794836303,-37.6868281287001));
#27961=CARTESIAN_POINT('Ctrl Pts',(23.0599057791681,51.5000241176224,-37.5288796055076));
#27962=CARTESIAN_POINT('Ctrl Pts',(20.4166969743319,53.3822269161586,-37.3709310823152));
#27963=CARTESIAN_POINT('Ctrl Pts',(17.3956817038809,52.1978675543976,-37.2129825591227));
#27964=CARTESIAN_POINT('Ctrl Pts',(16.7359226218695,49.0207684665076,-37.0550340359303));
#27965=CARTESIAN_POINT('Ctrl Pts',(19.0356032281376,46.7315088580311,-36.8970855127378));
#27966=CARTESIAN_POINT('Ctrl Pts',(22.2096730556696,47.4056907462554,-36.7391369895453));
#27967=CARTESIAN_POINT('Ctrl Pts',(23.3802995282873,50.4320539400645,-36.5811884663528));
#27968=CARTESIAN_POINT('Ctrl Pts',(21.486111225522,53.0666869629442,-36.4232399431604));
#27969=CARTESIAN_POINT('Ctrl Pts',(18.2445110727302,52.9208481874989,-36.2652914199679));
#27970=CARTESIAN_POINT('Ctrl Pts',(16.5945593394492,50.1267651930716,-36.1073428967755));
#27971=CARTESIAN_POINT('Ctrl Pts',(18.0322170813251,47.2177480539569,-35.949394373583));
#27972=CARTESIAN_POINT('Ctrl Pts',(21.2540037481356,46.8313141357098,-35.7914458503905));
#27973=CARTESIAN_POINT('Ctrl Pts',(23.3388233553195,49.3178313195118,-35.6334973271981));
#27974=CARTESIAN_POINT('Ctrl Pts',(22.3964333719533,52.422850098629,-35.4755488040055));
#27975=CARTESIAN_POINT('Ctrl Pts',(19.2812701344654,53.3311443810046,-35.3176002808131));
#27976=CARTESIAN_POINT('Ctrl Pts',(16.817757406876,51.2191913652847,-35.1596517576206));
#27977=CARTESIAN_POINT('Ctrl Pts',(17.2394872549391,48.0018346186981,-35.0017032344282));
#27978=CARTESIAN_POINT('Ctrl Pts',(20.1640900517487,46.596153651881,-34.8437547112357));
#27979=CARTESIAN_POINT('Ctrl Pts',(22.9399173892113,48.2766366455985,-34.6858061880432));
#27980=CARTESIAN_POINT('Ctrl Pts',(23.0502110434214,51.5196407790236,-34.5278576648508));
#27981=CARTESIAN_POINT('Ctrl Pts',(20.3949711125369,53.3848328358937,-34.3699091416583));
#27982=CARTESIAN_POINT('Ctrl Pts',(17.3816228864185,52.1810999054958,-34.2119606184658));
#27983=CARTESIAN_POINT('Ctrl Pts',(16.7422775548443,48.9998300259402,-34.0540120952734));
#27984=CARTESIAN_POINT('Ctrl Pts',(19.0566100851434,46.7253838430697,-33.8960635720809));
#27985=CARTESIAN_POINT('Ctrl Pts',(22.2262855593357,47.4199325367396,-33.7381150488884));
#27986=CARTESIAN_POINT('Ctrl Pts',(23.3774556262928,50.4537499301427,-33.580166525696));
#27987=CARTESIAN_POINT('Ctrl Pts',(21.4663893975598,53.0761660620659,-33.4222180025035));
#27988=CARTESIAN_POINT('Ctrl Pts',(18.2257925002768,52.9095159828755,-33.264269479311));
#27989=CARTESIAN_POINT('Ctrl Pts',(16.5938155829109,50.1048962509405,-33.1063209561186));
#27990=CARTESIAN_POINT('Ctrl Pts',(18.0501224821035,47.205170278553,-32.9483724329261));
#27991=CARTESIAN_POINT('Ctrl Pts',(21.2743240239289,46.8394314136979,-32.7904239097336));
#27992=CARTESIAN_POINT('Ctrl Pts',(23.3431347300711,49.3392839616946,-32.6324753865411));
#27993=CARTESIAN_POINT('Ctrl Pts',(22.3808268533046,52.4381876468528,-32.4745268633487));
#27994=CARTESIAN_POINT('Ctrl Pts',(19.2598956782223,53.3264607467349,-32.3165783401562));
#27995=CARTESIAN_POINT('Ctrl Pts',(16.8099945824404,51.1987330572828,-32.1586298169637));
#27996=CARTESIAN_POINT('Ctrl Pts',(17.2523743791307,47.9841505626103,-32.0006812937713));
#27997=CARTESIAN_POINT('Ctrl Pts',(20.1859427610074,46.5972774435298,-31.8427327705788));
#27998=CARTESIAN_POINT('Ctrl Pts',(22.9509224966721,48.2955493772724,-31.6847842473863));
#27999=CARTESIAN_POINT('Ctrl Pts',(23.040390552855,51.5391948521197,-31.5268357241939));
#28000=CARTESIAN_POINT('Ctrl Pts',(20.373228964063,53.3872991670454,-31.3688872010014));
#28001=CARTESIAN_POINT('Ctrl Pts',(17.3676720248009,52.1642423472583,-31.210938677809));
#28002=CARTESIAN_POINT('Ctrl Pts',(16.7487668020154,48.9789328136677,-31.0529901546164));
#28003=CARTESIAN_POINT('Ctrl Pts',(19.0776558380546,46.7193938435699,-30.895041631424));
#28004=CARTESIAN_POINT('Ctrl Pts',(22.2428062739001,47.4342807003812,-30.7370931082315));
#28005=CARTESIAN_POINT('Ctrl Pts',(23.3744724730697,50.4754272133319,-30.5791445850391));
#28006=CARTESIAN_POINT('Ctrl Pts',(21.4466071108482,53.0855183314193,-30.4211960618466));
#28007=CARTESIAN_POINT('Ctrl Pts',(18.2071470777866,52.8980638202076,-30.2632475386541));
#28008=CARTESIAN_POINT('Ctrl Pts',(16.5932122621402,50.0830229838389,-30.1052990154616));
#28009=CARTESIAN_POINT('Ctrl Pts',(18.0681082756436,47.1927077330565,-29.9473504922692));
#28010=CARTESIAN_POINT('Ctrl Pts',(21.2945917597949,46.8476790007708,-29.7894019690767));
#28011=CARTESIAN_POINT('Ctrl Pts',(23.3473082685591,49.3607638449891,-29.6314534458843));
#28012=CARTESIAN_POINT('Ctrl Pts',(22.365122174019,52.4534246694427,-29.4735049226918));
#28013=CARTESIAN_POINT('Ctrl Pts',(19.2385517361972,53.3216399636991,-29.3155563994993));
#28014=CARTESIAN_POINT('Ctrl Pts',(16.8023632808387,51.1782253258867,-29.1576078763069));
#28015=CARTESIAN_POINT('Ctrl Pts',(17.2653747868691,47.9665496193868,-28.9996593531143));
#28016=CARTESIAN_POINT('Ctrl Pts',(20.2077878040777,46.598541528012,-28.8417108299219));
#28017=CARTESIAN_POINT('Ctrl Pts',(22.9618059383148,48.3145323832604,-28.6837623067294));
#28018=CARTESIAN_POINT('Ctrl Pts',(23.0304447087213,51.5586854639238,-28.525813783537));
#28019=CARTESIAN_POINT('Ctrl Pts',(20.3514714261833,53.3896258427139,-28.3678652603445));
#28020=CARTESIAN_POINT('Ctrl Pts',(17.3538296957362,52.1472955547711,-28.209916737152));
#28021=CARTESIAN_POINT('Ctrl Pts',(16.7553900911946,48.9580777062127,-28.0519682139596));
#28022=CARTESIAN_POINT('Ctrl Pts',(19.0987396292081,46.7135390892003,-27.8940196907671));
#28023=CARTESIAN_POINT('Ctrl Pts',(22.2592344978135,47.4487346737953,-27.7360711675746));
#28024=CARTESIAN_POINT('Ctrl Pts',(23.3713502324408,50.4970848429156,-27.5781226443821));
#28025=CARTESIAN_POINT('Ctrl Pts',(21.4267650996209,53.0947434892864,-27.4201741211897));
#28026=CARTESIAN_POINT('Ctrl Pts',(18.1885757360692,52.8864919656703,-27.2622255979972));
#28027=CARTESIAN_POINT('Ctrl Pts',(16.5927490793524,50.0611467032797,-27.1042770748047));
#28028=CARTESIAN_POINT('Ctrl Pts',(18.0861743627476,47.1803601159088,-26.9463285516123));
#28029=CARTESIAN_POINT('Ctrl Pts',(21.3148048413315,46.8560581800179,-26.7883800284198));
#28030=CARTESIAN_POINT('Ctrl Pts',(23.3513463444372,49.3822668525686,-26.6304315052273));
#28031=CARTESIAN_POINT('Ctrl Pts',(22.3493149136648,52.4685669707326,-26.4724829820349));
#28032=CARTESIAN_POINT('Ctrl Pts',(19.2172492774196,53.3166694250122,-26.3145344588424));
#28033=CARTESIAN_POINT('Ctrl Pts',(16.7948437318888,51.1576945095679,-26.1565859356499));
#28034=CARTESIAN_POINT('Ctrl Pts',(17.2785279261903,47.94898176436,-25.9986374124574));
#28035=CARTESIAN_POINT('Ctrl Pts',(20.2295446815659,46.6000468855458,-25.840688889265));
#28036=CARTESIAN_POINT('Ctrl Pts',(22.9727257293063,48.3333837417603,-25.6827403660725));
#28037=CARTESIAN_POINT('Ctrl Pts',(23.0200584320667,51.578512333566,-25.5247918428801));
#28038=CARTESIAN_POINT('Ctrl Pts',(20.3303277842108,53.3910141178971,-25.3668433196876));
#28039=CARTESIAN_POINT('Ctrl Pts',(17.3388414083637,52.1318668903096,-25.2088947964951));
#28040=CARTESIAN_POINT('Ctrl Pts',(16.7646998141231,48.9338680409178,-25.0509462733026));
#28041=CARTESIAN_POINT('Ctrl Pts',(18.3310579529763,47.4565819515315,-24.945647257841));
#28042=CARTESIAN_POINT('Ctrl Pts',(19.2540671456531,47.2098224301578,-24.8929977501102));
#28043=CARTESIAN_POINT('Ctrl Pts',(17.6639373423039,51.9973015569307,-40.3210067496694));
#28044=CARTESIAN_POINT('Ctrl Pts',(17.003216778308,51.2245165804374,-40.2683572419386));
#28045=CARTESIAN_POINT('Ctrl Pts',(16.520038278527,48.9847745965717,-40.163058226477));
#28046=CARTESIAN_POINT('Ctrl Pts',(18.9512732547528,46.5262660550493,-40.0051097032845));
#28047=CARTESIAN_POINT('Ctrl Pts',(22.3337617221332,47.2252515387578,-39.847161180092));
#28048=CARTESIAN_POINT('Ctrl Pts',(23.6000558077849,50.4361301927122,-39.6892126568996));
#28049=CARTESIAN_POINT('Ctrl Pts',(21.6024147148416,53.2535259157778,-39.5312641337071));
#28050=CARTESIAN_POINT('Ctrl Pts',(18.1518494020808,53.1200733432643,-39.3733156105146));
#28051=CARTESIAN_POINT('Ctrl Pts',(16.376977963313,50.1582350183397,-39.2153670873222));
#28052=CARTESIAN_POINT('Ctrl Pts',(17.8869743722217,47.0526837548,-39.0574185641297));
#28053=CARTESIAN_POINT('Ctrl Pts',(21.3127949123184,46.6194980929628,-38.8994700409373));
#28054=CARTESIAN_POINT('Ctrl Pts',(23.5483401839262,49.2512486096866,-38.7415215177447));
#28055=CARTESIAN_POINT('Ctrl Pts',(22.566715362225,52.561900427485,-38.5835729945523));
#28056=CARTESIAN_POINT('Ctrl Pts',(19.257926763209,53.5497393781131,-38.4256244713598));
#28057=CARTESIAN_POINT('Ctrl Pts',(16.6219539119773,51.3191454645357,-38.2676759481674));
#28058=CARTESIAN_POINT('Ctrl Pts',(17.0487524523756,47.8925185252508,-38.1097274249749));
#28059=CARTESIAN_POINT('Ctrl Pts',(20.1513575155428,46.3766829286487,-37.9517789017824));
#28060=CARTESIAN_POINT('Ctrl Pts',(23.1167312576603,48.1459977249851,-37.79383037859));
#28061=CARTESIAN_POINT('Ctrl Pts',(23.2562595922233,51.5962804981864,-37.6358818553975));
#28062=CARTESIAN_POINT('Ctrl Pts',(20.4434363727656,53.5992640406764,-37.477933332205));
#28063=CARTESIAN_POINT('Ctrl Pts',(17.2285628888723,52.338904470578,-37.3199848090125));
#28064=CARTESIAN_POINT('Ctrl Pts',(16.5264671400482,48.9579312880643,-37.1620362858201));
#28065=CARTESIAN_POINT('Ctrl Pts',(18.9737179946959,46.5217701454759,-37.0040877626275));
#28066=CARTESIAN_POINT('Ctrl Pts',(22.3514675295518,47.2392142103812,-36.8461392394352));
#28067=CARTESIAN_POINT('Ctrl Pts',(23.59721297254,50.4597787932788,-36.6881907162426));
#28068=CARTESIAN_POINT('Ctrl Pts',(21.5814748173496,53.2634759238072,-36.5302421930502));
#28069=CARTESIAN_POINT('Ctrl Pts',(18.1318615437831,53.1082786903842,-36.3722936698577));
#28070=CARTESIAN_POINT('Ctrl Pts',(16.3760325915391,50.1348997013926,-36.2143451466653));
#28071=CARTESIAN_POINT('Ctrl Pts',(17.9059446705936,47.0392112564499,-36.0563966234728));
#28072=CARTESIAN_POINT('Ctrl Pts',(21.3344730289901,46.6279799167075,-35.8984481002803));
#28073=CARTESIAN_POINT('Ctrl Pts',(23.5530752781723,49.2740566312607,-35.7404995770878));
#28074=CARTESIAN_POINT('Ctrl Pts',(22.5502122345312,52.5783241196155,-35.5825510538954));
#28075=CARTESIAN_POINT('Ctrl Pts',(19.2351493190419,53.5449035449308,-35.4246025307029));
#28076=CARTESIAN_POINT('Ctrl Pts',(16.6135532540943,51.2974267394088,-35.2666540075105));
#28077=CARTESIAN_POINT('Ctrl Pts',(17.0623454595379,47.8736125687236,-35.108705484318));
#28078=CARTESIAN_POINT('Ctrl Pts',(20.1746196920941,46.3777292108223,-34.9507569611255));
#28079=CARTESIAN_POINT('Ctrl Pts',(23.1285715606466,48.1660486110843,-34.792808437933));
#28080=CARTESIAN_POINT('Ctrl Pts',(23.2459427463636,51.6171559585651,-34.6348599147406));
#28081=CARTESIAN_POINT('Ctrl Pts',(20.4203163648388,53.6020371819906,-34.4769113915481));
#28082=CARTESIAN_POINT('Ctrl Pts',(17.2136019186591,52.3210608435138,-34.3189628683557));
#28083=CARTESIAN_POINT('Ctrl Pts',(16.5332298683643,48.9356492300977,-34.1610143451631));
#28084=CARTESIAN_POINT('Ctrl Pts',(18.9960728593762,46.5152520889867,-34.0030658219707));
#28085=CARTESIAN_POINT('Ctrl Pts',(22.3691460557279,47.2543698949745,-33.8451172987782));
#28086=CARTESIAN_POINT('Ctrl Pts',(23.5941865776713,50.4828670126241,-33.6871687755858));
#28087=CARTESIAN_POINT('Ctrl Pts',(21.5604874418836,53.2735632956638,-33.5292202523933));
#28088=CARTESIAN_POINT('Ctrl Pts',(18.1119418026202,53.0962192994522,-33.3712717292008));
#28089=CARTESIAN_POINT('Ctrl Pts',(16.3752411082267,50.1116274316806,-33.2133232060084));
#28090=CARTESIAN_POINT('Ctrl Pts',(17.9249990589457,47.0258263665991,-33.0553746828159));
#28091=CARTESIAN_POINT('Ctrl Pts',(21.3560972546178,46.63661807952,-32.8974261596234));
#28092=CARTESIAN_POINT('Ctrl Pts',(23.5576633133616,49.2968858871031,-32.739477636431));
#28093=CARTESIAN_POINT('Ctrl Pts',(22.5336042473189,52.5946458766007,-32.5815291132385));
#28094=CARTESIAN_POINT('Ctrl Pts',(19.2124032663222,53.5399193623716,-32.423580590046));
#28095=CARTESIAN_POINT('Ctrl Pts',(16.6052922900793,51.2756556240609,-32.2656320668535));
#28096=CARTESIAN_POINT('Ctrl Pts',(17.0760595490536,47.8547937287262,-32.1076835436611));
#28097=CARTESIAN_POINT('Ctrl Pts',(20.197874687272,46.378925116056,-31.9497350204686));
#28098=CARTESIAN_POINT('Ctrl Pts',(23.1402828646275,48.1861749706435,-31.7917864972762));
#28099=CARTESIAN_POINT('Ctrl Pts',(23.2354920760113,51.637964814354,-31.6338379740837));
#28100=CARTESIAN_POINT('Ctrl Pts',(20.397179025119,53.6046617773376,-31.4758894508912));
#28101=CARTESIAN_POINT('Ctrl Pts',(17.1987558318052,52.3031215376416,-31.3179409276987));
#28102=CARTESIAN_POINT('Ctrl Pts',(16.5401355298036,48.913411046041,-31.1599924045062));
#28103=CARTESIAN_POINT('Ctrl Pts',(19.0184691159077,46.508877711886,-31.0020438813138));
#28104=CARTESIAN_POINT('Ctrl Pts',(22.3867269027061,47.2696387786791,-30.8440953581213));
#28105=CARTESIAN_POINT('Ctrl Pts',(23.591011995838,50.5059353246612,-30.6861468349289));
#28106=CARTESIAN_POINT('Ctrl Pts',(21.5394357280369,53.2835156991,-30.5281983117364));
#28107=CARTESIAN_POINT('Ctrl Pts',(18.0920999054453,53.0840322527814,-30.370249788544));
#28108=CARTESIAN_POINT('Ctrl Pts',(16.3745990724293,50.0883505594653,-30.2123012653514));
#28109=CARTESIAN_POINT('Ctrl Pts',(17.9441389988542,47.012564100946,-30.054352742159));
#28110=CARTESIAN_POINT('Ctrl Pts',(21.3776655688371,46.6453949133369,-29.8964042189665));
#28111=CARTESIAN_POINT('Ctrl Pts',(23.5621046673495,49.3197441321162,-29.7384556957741));
#28112=CARTESIAN_POINT('Ctrl Pts',(22.5168918005126,52.6108606572331,-29.5805071725816));
#28113=CARTESIAN_POINT('Ctrl Pts',(19.1896896859145,53.5347892302254,-29.4225586493891));
#28114=CARTESIAN_POINT('Ctrl Pts',(16.5971712887038,51.2538319138251,-29.2646101261966));
#28115=CARTESIAN_POINT('Ctrl Pts',(17.0898941915086,47.8360633349363,-29.1066616030042));
#28116=CARTESIAN_POINT('Ctrl Pts',(20.2211215243232,46.3802703166986,-28.9487130798117));
#28117=CARTESIAN_POINT('Ctrl Pts',(23.1518646955083,48.2063761140114,-28.7907645566193));
#28118=CARTESIAN_POINT('Ctrl Pts',(23.2249080081672,51.6587061365469,-28.6328160334268));
#28119=CARTESIAN_POINT('Ctrl Pts',(20.3740253084567,53.6071377555246,-28.4748675102343));
#28120=CARTESIAN_POINT('Ctrl Pts',(17.1840252420261,52.2850872713679,-28.3169189870418));
#28121=CARTESIAN_POINT('Ctrl Pts',(16.5471838347117,48.8912176686634,-28.1589704638494));
#28122=CARTESIAN_POINT('Ctrl Pts',(19.0409058515914,46.5026472585805,-28.0010219406569));
#28123=CARTESIAN_POINT('Ctrl Pts',(22.4042093239182,47.2850202619573,-27.8430734174644));
#28124=CARTESIAN_POINT('Ctrl Pts',(23.5876894013757,50.5289827219232,-27.685124894272));
#28125=CARTESIAN_POINT('Ctrl Pts',(21.518320457159,53.29333283432,-27.5271763710795));
#28126=CARTESIAN_POINT('Ctrl Pts',(18.0723368427983,53.0717178336273,-27.369227847887));
#28127=CARTESIAN_POINT('Ctrl Pts',(16.3741061672535,50.0650704804189,-27.2112793246946));
#28128=CARTESIAN_POINT('Ctrl Pts',(17.9633643847556,46.9994241385813,-27.0533308015021));
#28129=CARTESIAN_POINT('Ctrl Pts',(21.3991757215647,46.654311783583,-26.8953822783096));
#28130=CARTESIAN_POINT('Ctrl Pts',(23.5664018661069,49.3426269852974,-26.7374337551172));
#28131=CARTESIAN_POINT('Ctrl Pts',(22.5000701900221,52.6269746383103,-26.5794852319247));
#28132=CARTESIAN_POINT('Ctrl Pts',(19.1670202507297,53.5294997326245,-26.4215367087322));
#28133=CARTESIAN_POINT('Ctrl Pts',(16.5891692111351,51.2319836373097,-26.2635881855398));
#28134=CARTESIAN_POINT('Ctrl Pts',(17.1038913663152,47.8173681526091,-26.1056396623473));
#28135=CARTESIAN_POINT('Ctrl Pts',(20.2442745382167,46.3818722728576,-25.9476911391548));
#28136=CARTESIAN_POINT('Ctrl Pts',(23.1634852082715,48.2264371620868,-25.7897426159623));
#28137=CARTESIAN_POINT('Ctrl Pts',(23.2138552452965,51.6798052942057,-25.6317940927699));
#28138=CARTESIAN_POINT('Ctrl Pts',(20.3515248813337,53.6086151161717,-25.4738455695774));
#28139=CARTESIAN_POINT('Ctrl Pts',(17.1680751579223,52.2686685512262,-25.3158970463849));
#28140=CARTESIAN_POINT('Ctrl Pts',(16.5570909615237,48.8654544718428,-25.1579485231925));
#28141=CARTESIAN_POINT('Ctrl Pts',(18.2239621276955,47.2933710986319,-25.0526495077308));
#28142=CARTESIAN_POINT('Ctrl Pts',(19.2062007174672,47.0307770462543,-25.));
#28143=CARTESIAN_POINT('Ctrl Pts',(22.51811817366,49.9978011072146,-38.387416697508));
#28144=CARTESIAN_POINT('Ctrl Pts',(22.5197005021771,49.8234380607443,-38.3984493876971));
#28145=CARTESIAN_POINT('Ctrl Pts',(22.5031152203389,49.6493741016012,-38.4094820778862));
#28146=CARTESIAN_POINT('Ctrl Pts',(22.4672443342715,49.4793798749943,-38.4205147680753));
#28147=CARTESIAN_POINT('Ctrl Pts',(22.296063555971,48.6681441569118,-38.4731642758061));
#28148=CARTESIAN_POINT('Ctrl Pts',(21.6856861120934,47.9495896397109,-38.525813783537));
#28149=CARTESIAN_POINT('Ctrl Pts',(20.9128165046445,47.6494493532743,-38.5784632912678));
#28150=CARTESIAN_POINT('Ctrl Pts',(20.1399468971955,47.3493090668377,-38.6311127989986));
#28151=CARTESIAN_POINT('Ctrl Pts',(19.2045851261751,47.4675830111656,-38.6837623067294));
#28152=CARTESIAN_POINT('Ctrl Pts',(18.53076487949,47.9506788416322,-38.7364118144602));
#28153=CARTESIAN_POINT('Ctrl Pts',(17.8569446328048,48.4337746720989,-38.7890613221911));
#28154=CARTESIAN_POINT('Ctrl Pts',(17.4446659104548,49.2816923887045,-38.8417108299219));
#28155=CARTESIAN_POINT('Ctrl Pts',(17.4808257113154,50.1099909239769,-38.8943603376527));
#28156=CARTESIAN_POINT('Ctrl Pts',(17.516985512176,50.9382894592493,-38.9470098453835));
#28157=CARTESIAN_POINT('Ctrl Pts',(18.0015838362472,51.7469688131886,-38.9996593531144));
#28158=CARTESIAN_POINT('Ctrl Pts',(18.7149419525084,52.1695269626545,-39.0523088608452));
#28159=CARTESIAN_POINT('Ctrl Pts',(19.4283000687697,52.5920851121204,-39.104958368576));
#28160=CARTESIAN_POINT('Ctrl Pts',(20.370417977221,52.6285220571129,-39.1576078763068));
#28161=CARTESIAN_POINT('Ctrl Pts',(21.1141878175962,52.2621196450141,-39.2102573840377));
#28162=CARTESIAN_POINT('Ctrl Pts',(21.8579576579715,51.8957172329152,-39.2629068917685));
#28163=CARTESIAN_POINT('Ctrl Pts',(22.4033794302707,51.126475463725,-39.3155563994993));
#28164=CARTESIAN_POINT('Ctrl Pts',(22.5032203331966,50.3035167985687,-39.3682059072301));
#28165=CARTESIAN_POINT('Ctrl Pts',(22.5153636733716,50.2034228818663,-39.3746095039894));
#28166=CARTESIAN_POINT('Ctrl Pts',(22.5209154892233,50.1025343255133,-39.3810131007487));
#28167=CARTESIAN_POINT('Ctrl Pts',(22.5201576955115,50.0015647648602,-39.387416697508));
#28168=CARTESIAN_POINT('Ctrl Pts',(20.7937992825328,47.0307770462543,-40.));
#28169=CARTESIAN_POINT('Ctrl Pts',(21.7760378723045,47.2933710986319,-39.9473504922692));
#28170=CARTESIAN_POINT('Ctrl Pts',(23.4429089208816,48.865455216316,-39.8420514768075));
#28171=CARTESIAN_POINT('Ctrl Pts',(22.8319249444368,52.2686682330012,-39.6841029536151));
#28172=CARTESIAN_POINT('Ctrl Pts',(19.6484751064271,53.6086153775441,-39.5261544304226));
#28173=CARTESIAN_POINT('Ctrl Pts',(16.7861446928906,51.6798052066136,-39.3682059072302));
#28174=CARTESIAN_POINT('Ctrl Pts',(16.8365147494583,48.2264371981741,-39.2102573840376));
#28175=CARTESIAN_POINT('Ctrl Pts',(19.7557254495835,46.3818721760905,-39.0523088608452));
#28176=CARTESIAN_POINT('Ctrl Pts',(22.8961086873501,47.8173681367529,-38.8943603376527));
#28177=CARTESIAN_POINT('Ctrl Pts',(23.4108308418939,51.2319836465612,-38.7364118144603));
#28178=CARTESIAN_POINT('Ctrl Pts',(20.8329797652707,53.529499797304,-38.5784632912678));
#28179=CARTESIAN_POINT('Ctrl Pts',(17.4999297672036,52.6269746785947,-38.4205147680753));
#28180=CARTESIAN_POINT('Ctrl Pts',(16.4335980754498,49.3426269761734,-38.2625662448828));
#28181=CARTESIAN_POINT('Ctrl Pts',(18.6008242547947,46.6543117271026,-38.1046177216904));
#28182=CARTESIAN_POINT('Ctrl Pts',(22.0366356492785,46.9994240892982,-37.9466691984979));
#28183=CARTESIAN_POINT('Ctrl Pts',(23.6258938927882,50.065070481226,-37.7887206753055));
#28184=CARTESIAN_POINT('Ctrl Pts',(21.9276631892634,53.0717178847477,-37.6307721521129));
#28185=CARTESIAN_POINT('Ctrl Pts',(18.4816795176051,53.2933328888968,-37.4728236289205));
#28186=CARTESIAN_POINT('Ctrl Pts',(16.4123105391071,50.5289827307422,-37.314875105728));
#28187=CARTESIAN_POINT('Ctrl Pts',(17.595790636172,47.2850202168804,-37.1569265825356));
#28188=CARTESIAN_POINT('Ctrl Pts',(20.959094164331,46.5026472005525,-36.9989780593431));
#28189=CARTESIAN_POINT('Ctrl Pts',(23.4528162225852,48.891217650257,-36.8410295361507));
#28190=CARTESIAN_POINT('Ctrl Pts',(22.8159748047073,52.2850873092924,-36.6830810129581));
#28191=CARTESIAN_POINT('Ctrl Pts',(19.6259746853353,53.6071378153842,-36.5251324897657));
#28192=CARTESIAN_POINT('Ctrl Pts',(16.7750919383154,51.6587061640742,-36.3671839665732));
#28193=CARTESIAN_POINT('Ctrl Pts',(16.8481352521856,48.2063760842456,-36.2092354433807));
#28194=CARTESIAN_POINT('Ctrl Pts',(19.7788784720074,46.3802702566287,-36.0512869201883));
#28195=CARTESIAN_POINT('Ctrl Pts',(22.910105856785,47.8360632990252,-35.8933383969958));
#28196=CARTESIAN_POINT('Ctrl Pts',(23.4028287677669,51.2538319346328,-35.7353898738033));
#28197=CARTESIAN_POINT('Ctrl Pts',(20.8103103275328,53.5347892888857,-35.5774413506109));
#28198=CARTESIAN_POINT('Ctrl Pts',(17.4831081577191,52.610860700561,-35.4194928274184));
#28199=CARTESIAN_POINT('Ctrl Pts',(16.4378952735367,49.3197441208273,-35.2615443042259));
#28200=CARTESIAN_POINT('Ctrl Pts',(18.6223344083003,46.6453948576666,-35.1035957810335));
#28201=CARTESIAN_POINT('Ctrl Pts',(22.0558610352632,47.012564051369,-34.945647257841));
#28202=CARTESIAN_POINT('Ctrl Pts',(23.6254009877349,50.0883505609314,-34.7876987346485));
#28203=CARTESIAN_POINT('Ctrl Pts',(21.9079001262167,53.0840323039615,-34.6297502114561));
#28204=CARTESIAN_POINT('Ctrl Pts',(18.4605642464159,53.2835157535905,-34.4718016882636));
#28205=CARTESIAN_POINT('Ctrl Pts',(16.4089879445684,50.5059353330574,-34.3138531650712));
#28206=CARTESIAN_POINT('Ctrl Pts',(17.6132730576857,47.2696387333682,-34.1559046418787));
#28207=CARTESIAN_POINT('Ctrl Pts',(20.9815309003809,46.5088776539501,-33.9979561186862));
#28208=CARTESIAN_POINT('Ctrl Pts',(23.4598645276135,48.9134110280088,-33.8400075954937));
#28209=CARTESIAN_POINT('Ctrl Pts',(22.801244214682,52.3031215758622,-33.6820590723013));
#28210=CARTESIAN_POINT('Ctrl Pts',(19.6028209682899,53.6046618371577,-33.5241105491088));
#28211=CARTESIAN_POINT('Ctrl Pts',(16.7645078702952,51.6379648415364,-33.3661620259164));
#28212=CARTESIAN_POINT('Ctrl Pts',(16.8597170832589,48.1861749405428,-33.2082135027238));
#28213=CARTESIAN_POINT('Ctrl Pts',(19.8021253094441,46.3789250559636,-33.0502649795314));
#28214=CARTESIAN_POINT('Ctrl Pts',(22.9239404994698,47.854793693126,-32.8923164563389));
#28215=CARTESIAN_POINT('Ctrl Pts',(23.3947077662565,51.2756556452305,-32.7343679331465));
#28216=CARTESIAN_POINT('Ctrl Pts',(20.7875967467482,53.5399194211172,-32.5764194099539));
#28217=CARTESIAN_POINT('Ctrl Pts',(17.4663957106355,52.5946459196594,-32.4184708867616));
#28218=CARTESIAN_POINT('Ctrl Pts',(16.4423366275984,49.2968858754349,-32.260522363569));
#28219=CARTESIAN_POINT('Ctrl Pts',(18.6439027228774,46.6366180237041,-32.1025738403766));
#28220=CARTESIAN_POINT('Ctrl Pts',(22.0750009754893,47.0258263172421,-31.9446253171841));
#28221=CARTESIAN_POINT('Ctrl Pts',(23.6247589519268,50.111627433533,-31.7866767939916));
#28222=CARTESIAN_POINT('Ctrl Pts',(21.8880582287126,53.0962193508344,-31.6287282707992));
#28223=CARTESIAN_POINT('Ctrl Pts',(18.4395125322199,53.2735633499893,-31.4707797476067));
#28224=CARTESIAN_POINT('Ctrl Pts',(16.4058133626825,50.4828670206375,-31.3128312244142));
#28225=CARTESIAN_POINT('Ctrl Pts',(17.6308539049556,47.2543698494103,-31.1548827012218));
#28226=CARTESIAN_POINT('Ctrl Pts',(21.0039271572841,46.5152520311566,-30.9969341780293));
#28227=CARTESIAN_POINT('Ctrl Pts',(23.4667701891674,48.9356492124344,-30.8389856548368));
#28228=CARTESIAN_POINT('Ctrl Pts',(22.7863981275818,52.3210608820322,-30.6810371316443));
#28229=CARTESIAN_POINT('Ctrl Pts',(19.5796836281861,53.602037241767,-30.5230886084519));
#28230=CARTESIAN_POINT('Ctrl Pts',(16.7540571997694,51.6171559854022,-30.3651400852594));
#28231=CARTESIAN_POINT('Ctrl Pts',(16.8714283874341,48.1660485806496,-30.207191562067));
#28232=CARTESIAN_POINT('Ctrl Pts',(19.825380305008,46.3777291507101,-30.0492430388745));
#28233=CARTESIAN_POINT('Ctrl Pts',(22.937654589213,47.8736125334356,-29.891294515682));
#28234=CARTESIAN_POINT('Ctrl Pts',(23.3864468021045,51.2974267609398,-29.7333459924896));
#28235=CARTESIAN_POINT('Ctrl Pts',(20.7648506936511,53.5449036037592,-29.5753974692971));
#28236=CARTESIAN_POINT('Ctrl Pts',(17.4497877231476,52.5783241624032,-29.4174489461046));
#28237=CARTESIAN_POINT('Ctrl Pts',(16.4469246628638,49.2740566192138,-29.2595004229122));
#28238=CARTESIAN_POINT('Ctrl Pts',(18.665526948864,46.6279798607482,-29.1015518997197));
#28239=CARTESIAN_POINT('Ctrl Pts',(22.0940553641576,47.0392112073149,-28.9436033765272));
#28240=CARTESIAN_POINT('Ctrl Pts',(23.6239674686013,50.1348997036314,-28.7856548533348));
#28241=CARTESIAN_POINT('Ctrl Pts',(21.868138487219,53.1082787419663,-28.6277063301423));
#28242=CARTESIAN_POINT('Ctrl Pts',(18.4185251564057,53.2634759779658,-28.4697578069498));
#28243=CARTESIAN_POINT('Ctrl Pts',(16.4027869677635,50.4597788009081,-28.3118092837573));
#28244=CARTESIAN_POINT('Ctrl Pts',(17.6485324314252,47.2392141645673,-28.1538607605649));
#28245=CARTESIAN_POINT('Ctrl Pts',(21.026282022335,46.5217700877505,-27.9959122373724));
#28246=CARTESIAN_POINT('Ctrl Pts',(23.4735329175963,48.9579312707775,-27.83796371418));
#28247=CARTESIAN_POINT('Ctrl Pts',(22.771437157119,52.3389045093798,-27.6800151909875));
#28248=CARTESIAN_POINT('Ctrl Pts',(19.5565636198783,53.5992641004309,-27.522066667795));
#28249=CARTESIAN_POINT('Ctrl Pts',(16.743740353733,51.5962805246318,-27.3641181446025));
#28250=CARTESIAN_POINT('Ctrl Pts',(16.8832686906281,48.1459976943029,-27.2061696214101));
#28251=CARTESIAN_POINT('Ctrl Pts',(19.8486424819224,46.3766828683592,-27.0482210982176));
#28252=CARTESIAN_POINT('Ctrl Pts',(22.9512475966477,47.8925184905753,-26.8902725750252));
#28253=CARTESIAN_POINT('Ctrl Pts',(23.3780461439863,51.3191454858715,-26.7323240518326));
#28254=CARTESIAN_POINT('Ctrl Pts',(20.7420732493018,53.5497394380497,-26.5743755286402));
#28255=CARTESIAN_POINT('Ctrl Pts',(17.4332845947801,52.5619004681089,-26.4164270054477));
#28256=CARTESIAN_POINT('Ctrl Pts',(16.4516597580046,49.2512486007173,-26.2584784822552));
#28257=CARTESIAN_POINT('Ctrl Pts',(18.6872050642303,46.6194980305971,-26.1005299590628));
#28258=CARTESIAN_POINT('Ctrl Pts',(22.113025666239,47.0526837171379,-25.9425814358703));
#28259=CARTESIAN_POINT('Ctrl Pts',(23.6230220898943,50.1582350010085,-25.7846329126779));
#28260=CARTESIAN_POINT('Ctrl Pts',(21.8481506426783,53.1200734299207,-25.6266843894854));
#28261=CARTESIAN_POINT('Ctrl Pts',(18.3975852298821,53.2535259099818,-25.4687358662929));
#28262=CARTESIAN_POINT('Ctrl Pts',(16.3999441908908,50.4361302999107,-25.3107873431005));
#28263=CARTESIAN_POINT('Ctrl Pts',(17.6662381197281,47.2252513302932,-25.1528388199079));
#28264=CARTESIAN_POINT('Ctrl Pts',(21.0487270098574,46.5262662593188,-24.9948902967155));
#28265=CARTESIAN_POINT('Ctrl Pts',(23.4799612028624,48.9847740496603,-24.836941773523));
#28266=CARTESIAN_POINT('Ctrl Pts',(22.996783221692,51.2245165804373,-24.7316427580614));
#28267=CARTESIAN_POINT('Ctrl Pts',(22.3360626576962,51.9973015569306,-24.6789932503306));
#28268=CARTESIAN_POINT('Ctrl Pts',(20.7459328543469,47.2098224301578,-40.1070022498898));
#28269=CARTESIAN_POINT('Ctrl Pts',(21.6689420470237,47.4565819515315,-40.054352742159));
#28270=CARTESIAN_POINT('Ctrl Pts',(23.2353000753732,48.9338687404989,-39.9490537266973));
#28271=CARTESIAN_POINT('Ctrl Pts',(22.6611586878231,52.1318665912736,-39.7911052035049));
#28272=CARTESIAN_POINT('Ctrl Pts',(19.669672204288,53.3910143635086,-39.6331566803124));
#28273=CARTESIAN_POINT('Ctrl Pts',(16.9799415098477,51.5785122512557,-39.4752081571199));
#28274=CARTESIAN_POINT('Ctrl Pts',(17.0272742309725,48.3333837756716,-39.3172596339275));
#28275=CARTESIAN_POINT('Ctrl Pts',(19.7704553069699,46.6000467946138,-39.159311110735));
#28276=CARTESIAN_POINT('Ctrl Pts',(22.7214721242389,47.9489817494599,-39.0013625875425));
#28277=CARTESIAN_POINT('Ctrl Pts',(23.2051563179425,51.1576945182614,-38.8434140643501));
#28278=CARTESIAN_POINT('Ctrl Pts',(20.782750737616,53.3166694857916,-38.6854655411576));
#28279=CARTESIAN_POINT('Ctrl Pts',(17.6506850461402,52.4685670085878,-38.5275170179651));
#28280=CARTESIAN_POINT('Ctrl Pts',(16.6486536006437,49.3822668439948,-38.3695684947727));
#28281=CARTESIAN_POINT('Ctrl Pts',(18.6851951364534,46.8560581269433,-38.2116199715802));
#28282=CARTESIAN_POINT('Ctrl Pts',(21.9138256692342,47.1803600695975,-38.0536714483877));
#28283=CARTESIAN_POINT('Ctrl Pts',(23.4072509770689,50.0611467040381,-37.8957229251952));
#28284=CARTESIAN_POINT('Ctrl Pts',(21.8114242940591,52.8864920137083,-37.7377744020028));
#28285=CARTESIAN_POINT('Ctrl Pts',(18.573234876665,53.0947435405722,-37.5798258788103));
#28286=CARTESIAN_POINT('Ctrl Pts',(16.628649711631,50.4970848512028,-37.4218773556178));
#28287=CARTESIAN_POINT('Ctrl Pts',(17.7407654646833,47.4487346314366,-37.2639288324254));
#28288=CARTESIAN_POINT('Ctrl Pts',(20.9012603857541,46.7135390346713,-37.1059803092329));
#28289=CARTESIAN_POINT('Ctrl Pts',(23.2446099626473,48.9580776889162,-36.9480317860404));
#28290=CARTESIAN_POINT('Ctrl Pts',(22.6461703481792,52.1472955904087,-36.790083262848));
#28291=CARTESIAN_POINT('Ctrl Pts',(19.6485285679831,53.3896258989639,-36.6321347396555));
#28292=CARTESIAN_POINT('Ctrl Pts',(16.9695552409884,51.5586854897913,-36.474186216463));
#28293=CARTESIAN_POINT('Ctrl Pts',(17.0381940125332,48.3145323552894,-36.3162376932706));
#28294=CARTESIAN_POINT('Ctrl Pts',(19.7922121924742,46.5985414715644,-36.1582891700781));
#28295=CARTESIAN_POINT('Ctrl Pts',(22.7346252585124,47.9665495856411,-36.0003406468857));
#28296=CARTESIAN_POINT('Ctrl Pts',(23.1976367722267,51.1782253454396,-35.8423921236931));
#28297=CARTESIAN_POINT('Ctrl Pts',(20.7614482764392,53.3216400188223,-35.6844436005007));
#28298=CARTESIAN_POINT('Ctrl Pts',(17.6348777867315,52.4534247101578,-35.5264950773082));
#28299=CARTESIAN_POINT('Ctrl Pts',(16.6526916758916,49.3607638343807,-35.3685465541157));
#28300=CARTESIAN_POINT('Ctrl Pts',(18.7054082187211,46.8476789484576,-35.2105980309233));
#28301=CARTESIAN_POINT('Ctrl Pts',(21.9318917564165,47.1927076864689,-35.0526495077308));
#28302=CARTESIAN_POINT('Ctrl Pts',(23.406787794396,50.0830229852167,-34.8947009845383));
#28303=CARTESIAN_POINT('Ctrl Pts',(21.7928529519662,52.8980638683015,-34.7367524613459));
#28304=CARTESIAN_POINT('Ctrl Pts',(18.5533928651451,53.0855183826241,-34.5788039381534));
#28305=CARTESIAN_POINT('Ctrl Pts',(16.6255274709304,50.4754272212218,-34.4208554149609));
#28306=CARTESIAN_POINT('Ctrl Pts',(17.75719368888,47.4342806578026,-34.2629068917685));
#28307=CARTESIAN_POINT('Ctrl Pts',(20.9223441772518,46.7193937891277,-34.104958368576));
#28308=CARTESIAN_POINT('Ctrl Pts',(23.2512332519394,48.9789327967227,-33.9470098453835));
#28309=CARTESIAN_POINT('Ctrl Pts',(22.6323280188832,52.1642423831742,-33.7890613221911));
#28310=CARTESIAN_POINT('Ctrl Pts',(19.6267710297432,53.3872992232582,-33.6311127989986));
#28311=CARTESIAN_POINT('Ctrl Pts',(16.9596093966892,51.539194877663,-33.4731642758061));
#28312=CARTESIAN_POINT('Ctrl Pts',(17.0490774543567,48.2955493489868,-33.3152157526137));
#28313=CARTESIAN_POINT('Ctrl Pts',(19.8140572359068,46.597277387061,-33.1572672294212));
#28314=CARTESIAN_POINT('Ctrl Pts',(22.7476256664666,47.9841505291569,-32.9993187062288));
#28315=CARTESIAN_POINT('Ctrl Pts',(23.1900054704983,51.1987330771759,-32.8413701830363));
#28316=CARTESIAN_POINT('Ctrl Pts',(20.74010433406,53.3264608019381,-32.6834216598438));
#28317=CARTESIAN_POINT('Ctrl Pts',(17.6191731071852,52.4381876873151,-32.5254731366513));
#28318=CARTESIAN_POINT('Ctrl Pts',(16.6568652144489,49.3392839507299,-32.3675246134589));
#28319=CARTESIAN_POINT('Ctrl Pts',(18.7256759549234,46.8394313612477,-32.2095760902664));
#28320=CARTESIAN_POINT('Ctrl Pts',(21.949877550255,47.2051702321722,-32.0516275670739));
#28321=CARTESIAN_POINT('Ctrl Pts',(23.4061844736153,50.1048962526811,-31.8936790438814));
#28322=CARTESIAN_POINT('Ctrl Pts',(21.7742075291666,52.9095160311594,-31.735730520689));
#28323=CARTESIAN_POINT('Ctrl Pts',(18.5336105781053,53.0761661131155,-31.5777819974965));
#28324=CARTESIAN_POINT('Ctrl Pts',(16.6225443176576,50.4537499376729,-31.419833474304));
#28325=CARTESIAN_POINT('Ctrl Pts',(17.7737144037186,47.4199324939229,-31.2618849511116));
#28326=CARTESIAN_POINT('Ctrl Pts',(20.9433899305122,46.7253837887268,-31.1039364279191));
#28327=CARTESIAN_POINT('Ctrl Pts',(23.2577224992181,48.9998300093421,-30.9459879047267));
#28328=CARTESIAN_POINT('Ctrl Pts',(22.6183771570341,52.1810999416916,-30.7880393815342));
#28329=CARTESIAN_POINT('Ctrl Pts',(19.6050288809086,53.3848328920656,-30.6300908583417));
#28330=CARTESIAN_POINT('Ctrl Pts',(16.9497889059598,51.5196408042424,-30.4721423351492));
#28331=CARTESIAN_POINT('Ctrl Pts',(17.0600825620002,48.276636616999,-30.3141938119568));
#28332=CARTESIAN_POINT('Ctrl Pts',(19.8359099455281,46.5961535953936,-30.1562452887643));
#28333=CARTESIAN_POINT('Ctrl Pts',(22.7605127908721,48.001834585538,-29.9982967655718));
#28334=CARTESIAN_POINT('Ctrl Pts',(23.182242645934,51.2191913855173,-29.8403482423794));
#28335=CARTESIAN_POINT('Ctrl Pts',(20.7187298774621,53.3311444362856,-29.6823997191869));
#28336=CARTESIAN_POINT('Ctrl Pts',(17.6035665882775,52.4228501388366,-29.5244511959944));
#28337=CARTESIAN_POINT('Ctrl Pts',(16.6611765892721,49.3178313081912,-29.366502672802));
#28338=CARTESIAN_POINT('Ctrl Pts',(18.7459962310538,46.8313140831249,-29.2085541496095));
#28339=CARTESIAN_POINT('Ctrl Pts',(21.9677829513306,47.2177480077848,-29.050605626417));
#28340=CARTESIAN_POINT('Ctrl Pts',(23.4054407170648,50.1267651951753,-28.8926571032246));
#28341=CARTESIAN_POINT('Ctrl Pts',(21.7554889564025,52.9208482359706,-28.7347085800321));
#28342=CARTESIAN_POINT('Ctrl Pts',(18.5138887498158,53.0666870138371,-28.5767600568396));
#28343=CARTESIAN_POINT('Ctrl Pts',(16.619700415616,50.4320539472337,-28.4188115336471));
#28344=CARTESIAN_POINT('Ctrl Pts',(17.7903269076605,47.4056907032041,-28.2608630104547));
#28345=CARTESIAN_POINT('Ctrl Pts',(20.9643967878664,46.7315088037866,-28.1029144872622));
#28346=CARTESIAN_POINT('Ctrl Pts',(23.264077432299,49.0207684502632,-27.9449659640697));
#28347=CARTESIAN_POINT('Ctrl Pts',(22.6043183393371,52.1978675908597,-27.7870174408773));
#28348=CARTESIAN_POINT('Ctrl Pts',(19.5833030187556,53.3822269723099,-27.6290689176848));
#28349=CARTESIAN_POINT('Ctrl Pts',(16.9400941700472,51.5000241424731,-27.4711203944923));
#28350=CARTESIAN_POINT('Ctrl Pts',(17.0712088899677,48.2577948074711,-27.3131718712999));
#28351=CARTESIAN_POINT('Ctrl Pts',(19.8577694034615,46.5951704043054,-27.1552233481074));
#28352=CARTESIAN_POINT('Ctrl Pts',(22.7732861342827,48.019600505568,-26.997274824915));
#28353=CARTESIAN_POINT('Ctrl Pts',(23.174348551008,51.2396004622671,-26.8393263017225));
#28354=CARTESIAN_POINT('Ctrl Pts',(20.6973259225178,53.3356886677492,-26.68137777853));
#28355=CARTESIAN_POINT('Ctrl Pts',(17.5880586054414,52.407416800166,-26.5234292553375));
#28356=CARTESIAN_POINT('Ctrl Pts',(16.6656261561987,49.2963986227336,-26.365480732145));
#28357=CARTESIAN_POINT('Ctrl Pts',(18.766367147012,46.8233437108734,-26.2075322089526));
#28358=CARTESIAN_POINT('Ctrl Pts',(21.9856093362754,47.2304081196401,-26.0495836857601));
#28359=CARTESIAN_POINT('Ctrl Pts',(23.4045523450886,50.148693364377,-25.8916351625677));
#28360=CARTESIAN_POINT('Ctrl Pts',(21.7367063872335,52.9319316993164,-25.7336866393752));
#28361=CARTESIAN_POINT('Ctrl Pts',(18.4942115096051,53.0573369391072,-25.5757381161827));
#28362=CARTESIAN_POINT('Ctrl Pts',(16.6170290593757,50.4098314607207,-25.4177895929903));
#28363=CARTESIAN_POINT('Ctrl Pts',(17.8069649355658,47.392569833667,-25.2598410697978));
#28364=CARTESIAN_POINT('Ctrl Pts',(20.9854883332692,46.7357338543319,-25.1018925466053));
#28365=CARTESIAN_POINT('Ctrl Pts',(23.2701180892795,49.0459925983713,-24.9439440234128));
#28366=CARTESIAN_POINT('Ctrl Pts',(22.8160759421236,51.1506777193426,-24.8386450079512));
#28367=CARTESIAN_POINT('Ctrl Pts',(22.1951971040192,51.8768634390787,-24.7859955002204));
#28368=CARTESIAN_POINT('Ctrl Pts',(20.698066426161,47.3888678140614,-40.2140044997796));
#28369=CARTESIAN_POINT('Ctrl Pts',(21.561846221743,47.6197928044311,-40.1613549920488));
#28370=CARTESIAN_POINT('Ctrl Pts',(23.0276912298648,49.0022822646818,-40.0560559765871));
#28371=CARTESIAN_POINT('Ctrl Pts',(22.4903924312093,51.9950649495461,-39.8981074533947));
#28372=CARTESIAN_POINT('Ctrl Pts',(19.6908693021489,53.1734133494731,-39.7401589302022));
#28373=CARTESIAN_POINT('Ctrl Pts',(17.1737383268048,51.4772192958978,-39.5822104070098));
#28374=CARTESIAN_POINT('Ctrl Pts',(17.2180337124866,48.4403303531691,-39.4242618838172));
#28375=CARTESIAN_POINT('Ctrl Pts',(19.7851851643563,46.818221413137,-39.2663133606248));
#28376=CARTESIAN_POINT('Ctrl Pts',(22.5468355611278,48.0805953621669,-39.1083648374323));
#28377=CARTESIAN_POINT('Ctrl Pts',(22.9994817939913,51.0834053899617,-38.9504163142399));
#28378=CARTESIAN_POINT('Ctrl Pts',(20.7325217099613,53.103839174279,-38.7924677910474));
#28379=CARTESIAN_POINT('Ctrl Pts',(17.8014403250768,52.3101593385808,-38.6345192678549));
#28380=CARTESIAN_POINT('Ctrl Pts',(16.8637091258375,49.4219067118163,-38.4765707446625));
#28381=CARTESIAN_POINT('Ctrl Pts',(18.7695660181121,47.0578045267839,-38.31862222147));
#28382=CARTESIAN_POINT('Ctrl Pts',(21.7910156891898,47.3612960498969,-38.1606736982775));
#28383=CARTESIAN_POINT('Ctrl Pts',(23.1886080613495,50.0572229268501,-38.0027251750851));
#28384=CARTESIAN_POINT('Ctrl Pts',(21.6951853988549,52.7012661426686,-37.8447766518926));
#28385=CARTESIAN_POINT('Ctrl Pts',(18.6647902357249,52.8961541922478,-37.6868281287002));
#28386=CARTESIAN_POINT('Ctrl Pts',(16.8449888841548,50.4651869716634,-37.5288796055076));
#28387=CARTESIAN_POINT('Ctrl Pts',(17.8857402931946,47.6124490459927,-37.3709310823153));
#28388=CARTESIAN_POINT('Ctrl Pts',(20.8434266071773,46.9244308687901,-37.2129825591227));
#28389=CARTESIAN_POINT('Ctrl Pts',(23.0364037027094,49.0249377275755,-37.0550340359303));
#28390=CARTESIAN_POINT('Ctrl Pts',(22.4763658916511,52.0095038715251,-36.8970855127378));
#28391=CARTESIAN_POINT('Ctrl Pts',(19.6710824506308,53.1721139825436,-36.7391369895453));
#28392=CARTESIAN_POINT('Ctrl Pts',(17.1640185436614,51.4586648155085,-36.5811884663528));
#28393=CARTESIAN_POINT('Ctrl Pts',(17.2282527728808,48.4226886263332,-36.4232399431604));
#28394=CARTESIAN_POINT('Ctrl Pts',(19.805545912941,46.8168126865001,-36.2652914199679));
#28395=CARTESIAN_POINT('Ctrl Pts',(22.5591446602398,48.097035872257,-36.1073428967755));
#28396=CARTESIAN_POINT('Ctrl Pts',(22.9924447766865,51.1026187562464,-35.9493943735829));
#28397=CARTESIAN_POINT('Ctrl Pts',(20.7125862253456,53.1084907487588,-35.7914458503905));
#28398=CARTESIAN_POINT('Ctrl Pts',(17.7866474157438,52.2959887197547,-35.633497327198));
#28399=CARTESIAN_POINT('Ctrl Pts',(16.8674880782465,49.4017835479343,-35.4755488040056));
#28400=CARTESIAN_POINT('Ctrl Pts',(18.7884820291419,47.0499630392484,-35.3176002808131));
#28401=CARTESIAN_POINT('Ctrl Pts',(21.8079224775697,47.3728513215688,-35.1596517576206));
#28402=CARTESIAN_POINT('Ctrl Pts',(23.1881746010572,50.077695409502,-35.0017032344282));
#28403=CARTESIAN_POINT('Ctrl Pts',(21.6778057777158,52.7120954326415,-34.8437547112357));
#28404=CARTESIAN_POINT('Ctrl Pts',(18.6462214838744,52.8875210116576,-34.6858061880433));
#28405=CARTESIAN_POINT('Ctrl Pts',(16.8420669972922,50.4449191093862,-34.5278576648507));
#28406=CARTESIAN_POINT('Ctrl Pts',(17.9011143200743,47.5989225822371,-34.3699091416583));
#28407=CARTESIAN_POINT('Ctrl Pts',(20.8631574541227,46.9299099243051,-34.2119606184658));
#28408=CARTESIAN_POINT('Ctrl Pts',(23.0426019762653,49.0444545654367,-34.0540120952734));
#28409=CARTESIAN_POINT('Ctrl Pts',(22.4634118230843,52.0253631904863,-33.8960635720809));
#28410=CARTESIAN_POINT('Ctrl Pts',(19.6507210911966,53.1699366093588,-33.7381150488884));
#28411=CARTESIAN_POINT('Ctrl Pts',(17.1547109230832,51.4404249137897,-33.5801665256959));
#28412=CARTESIAN_POINT('Ctrl Pts',(17.2384378254546,48.4049237574308,-33.4222180025035));
#28413=CARTESIAN_POINT('Ctrl Pts',(19.8259891623695,46.8156297181585,-33.264269479311));
#28414=CARTESIAN_POINT('Ctrl Pts',(22.5713108334635,48.1135073651876,-33.1063209561185));
#28415=CARTESIAN_POINT('Ctrl Pts',(22.9853031747401,51.1218105091212,-32.9483724329261));
#28416=CARTESIAN_POINT('Ctrl Pts',(20.6926119213717,53.113002182759,-32.7904239097336));
#28417=CARTESIAN_POINT('Ctrl Pts',(17.7719505037349,52.2817294549708,-32.6324753865412));
#28418=CARTESIAN_POINT('Ctrl Pts',(16.8713938012994,49.381682026025,-32.4745268633487));
#28419=CARTESIAN_POINT('Ctrl Pts',(18.8074491869694,47.0422446987913,-32.3165783401562));
#28420=CARTESIAN_POINT('Ctrl Pts',(21.8247541250208,47.3845141471024,-32.1586298169637));
#28421=CARTESIAN_POINT('Ctrl Pts',(23.1876099953038,50.0981650718293,-32.0006812937713));
#28422=CARTESIAN_POINT('Ctrl Pts',(21.6603568296206,52.7228127114843,-31.8427327705788));
#28423=CARTESIAN_POINT('Ctrl Pts',(18.6277086239906,52.8787688762418,-31.6847842473863));
#28424=CARTESIAN_POINT('Ctrl Pts',(16.8392752726328,50.4246328547084,-31.5268357241939));
#28425=CARTESIAN_POINT('Ctrl Pts',(17.9165749024817,47.5854951384354,-31.3688872010014));
#28426=CARTESIAN_POINT('Ctrl Pts',(20.8828527037404,46.9355155462971,-31.2109386778089));
#28427=CARTESIAN_POINT('Ctrl Pts',(23.0486748092689,49.0640108062497,-31.0529901546164));
#28428=CARTESIAN_POINT('Ctrl Pts',(22.4503561864863,52.0411390013511,-30.895041631424));
#28429=CARTESIAN_POINT('Ctrl Pts',(19.6303741336312,53.1676285423641,-30.7370931082315));
#28430=CARTESIAN_POINT('Ctrl Pts',(17.1455206121502,51.4221256230826,-30.5791445850391));
#28431=CARTESIAN_POINT('Ctrl Pts',(17.2487367365663,48.3872246533482,-30.4211960618466));
#28432=CARTESIAN_POINT('Ctrl Pts',(19.8464395860482,46.8145780400772,-30.2632475386541));
#28433=CARTESIAN_POINT('Ctrl Pts',(22.5833709925312,48.1300566376404,-30.1052990154616));
#28434=CARTESIAN_POINT('Ctrl Pts',(22.9780384897635,51.1409560100949,-29.9473504922692));
#28435=CARTESIAN_POINT('Ctrl Pts',(20.6726090612732,53.117385268812,-29.7894019690767));
#28436=CARTESIAN_POINT('Ctrl Pts',(17.7573454534073,52.2673761152701,-29.6314534458842));
#28437=CARTESIAN_POINT('Ctrl Pts',(16.8754285156804,49.3616059971687,-29.4735049226918));
#28438=CARTESIAN_POINT('Ctrl Pts',(18.8264655132437,47.0346483055016,-29.3155563994993));
#28439=CARTESIAN_POINT('Ctrl Pts',(21.8415105385036,47.3962848082547,-29.1576078763068));
#28440=CARTESIAN_POINT('Ctrl Pts',(23.1869139655283,50.1186306867194,-28.9996593531144));
#28441=CARTESIAN_POINT('Ctrl Pts',(21.642839425586,52.7334177299748,-28.8417108299219));
#28442=CARTESIAN_POINT('Ctrl Pts',(18.609252343226,52.8698980497084,-28.6837623067294));
#28443=CARTESIAN_POINT('Ctrl Pts',(16.8366138634684,50.4043290935593,-28.5258137835369));
#28444=CARTESIAN_POINT('Ctrl Pts',(17.9321213838958,47.5721672418409,-28.3678652603445));
#28445=CARTESIAN_POINT('Ctrl Pts',(20.9025115533977,46.9412475198227,-28.209916737152));
#28446=CARTESIAN_POINT('Ctrl Pts',(23.0546219470018,49.0836056297488,-28.0519682139596));
#28447=CARTESIAN_POINT('Ctrl Pts',(22.4371995215552,52.0568306723395,-27.8940196907671));
#28448=CARTESIAN_POINT('Ctrl Pts',(19.6100424176328,53.1651898441889,-27.7360711675746));
#28449=CARTESIAN_POINT('Ctrl Pts',(17.1364479863613,51.4037677603142,-27.5781226443821));
#28450=CARTESIAN_POINT('Ctrl Pts',(17.2591490893073,48.3695919206393,-27.4201741211897));
#28451=CARTESIAN_POINT('Ctrl Pts',(19.8668963250006,46.8136579402516,-27.2622255979972));
#28452=CARTESIAN_POINT('Ctrl Pts',(22.5953246719178,48.1466825205607,-27.1042770748048));
#28453=CARTESIAN_POINT('Ctrl Pts',(22.9706509580297,51.1600554386627,-26.9463285516123));
#28454=CARTESIAN_POINT('Ctrl Pts',(20.6525785957338,53.1216378974487,-26.7883800284198));
#28455=CARTESIAN_POINT('Ctrl Pts',(17.7428326161027,52.252933132223,-26.6304315052274));
#28456=CARTESIAN_POINT('Ctrl Pts',(16.8795925543929,49.3415486447498,-26.4724829820348));
#28457=CARTESIAN_POINT('Ctrl Pts',(18.8455292297936,47.0271893911498,-26.3145344588424));
#28458=CARTESIAN_POINT('Ctrl Pts',(21.8581930063119,47.4081325221422,-26.1565859356499));
#28459=CARTESIAN_POINT('Ctrl Pts',(23.1860826002829,50.1391517277455,-25.9986374124575));
#28460=CARTESIAN_POINT('Ctrl Pts',(21.6252621317886,52.7437899687123,-25.840688889265));
#28461=CARTESIAN_POINT('Ctrl Pts',(18.590837789328,52.8611479682325,-25.6827403660725));
#28462=CARTESIAN_POINT('Ctrl Pts',(16.8341139278605,50.3835326215309,-25.5247918428801));
#28463=CARTESIAN_POINT('Ctrl Pts',(17.9476917514034,47.5598883370406,-25.3668433196876));
#28464=CARTESIAN_POINT('Ctrl Pts',(20.9222496566812,46.945201449345,-25.2088947964952));
#28465=CARTESIAN_POINT('Ctrl Pts',(23.0602749756965,49.1072111470821,-25.0509462733026));
#28466=CARTESIAN_POINT('Ctrl Pts',(22.6353686625552,51.076838858248,-24.945647257841));
#28467=CARTESIAN_POINT('Ctrl Pts',(22.0543315503421,51.7564253212268,-24.8929977501102));
#28468=CARTESIAN_POINT('Ctrl Pts',(20.6501999979751,47.5679131979649,-40.3210067496694));
#28469=CARTESIAN_POINT('Ctrl Pts',(21.4547503964622,47.7830036573307,-40.2683572419386));
#28470=CARTESIAN_POINT('Ctrl Pts',(22.8200823843564,49.0706957888647,-40.1630582264769));
#28471=CARTESIAN_POINT('Ctrl Pts',(22.3196261745956,51.8582633078185,-40.0051097032845));
#28472=CARTESIAN_POINT('Ctrl Pts',(19.7120664000098,52.9558123354376,-39.847161180092));
#28473=CARTESIAN_POINT('Ctrl Pts',(17.3675351437619,51.37592634054,-39.6892126568996));
#28474=CARTESIAN_POINT('Ctrl Pts',(17.4087931940007,48.5472769306665,-39.5312641337071));
#28475=CARTESIAN_POINT('Ctrl Pts',(19.7999150217428,47.0363960316603,-39.3733156105147));
#28476=CARTESIAN_POINT('Ctrl Pts',(22.3721989980166,48.212208974874,-39.2153670873221));
#28477=CARTESIAN_POINT('Ctrl Pts',(22.79380727004,51.0091162616619,-39.0574185641297));
#28478=CARTESIAN_POINT('Ctrl Pts',(20.6822926823065,52.8910088627665,-38.8994700409372));
#28479=CARTESIAN_POINT('Ctrl Pts',(17.9521956040134,52.151751668574,-38.7415215177447));
#28480=CARTESIAN_POINT('Ctrl Pts',(17.0787646510314,49.4615465796377,-38.5835729945523));
#28481=CARTESIAN_POINT('Ctrl Pts',(18.8539368997708,47.2595509266246,-38.4256244713598));
#28482=CARTESIAN_POINT('Ctrl Pts',(21.6682057091455,47.5422320301962,-38.2676759481674));
#28483=CARTESIAN_POINT('Ctrl Pts',(22.9699651456302,50.0532991496622,-38.1097274249748));
#28484=CARTESIAN_POINT('Ctrl Pts',(21.5789465036507,52.5160402716292,-37.9517789017824));
#28485=CARTESIAN_POINT('Ctrl Pts',(18.7563455947847,52.6975648439231,-37.7938303785899));
#28486=CARTESIAN_POINT('Ctrl Pts',(17.0613280566787,50.4332890921241,-37.6358818553975));
#28487=CARTESIAN_POINT('Ctrl Pts',(18.0307151217059,47.7761634605487,-37.477933332205));
#28488=CARTESIAN_POINT('Ctrl Pts',(20.7855928286004,47.135322702909,-37.3199848090125));
#28489=CARTESIAN_POINT('Ctrl Pts',(22.8281974427715,49.0917977662346,-37.1620362858201));
#28490=CARTESIAN_POINT('Ctrl Pts',(22.306561435123,51.8717121526415,-37.0040877626276));
#28491=CARTESIAN_POINT('Ctrl Pts',(19.6936363332786,52.9546020661232,-36.8461392394351));
#28492=CARTESIAN_POINT('Ctrl Pts',(17.3584818463344,51.3586441412256,-36.6881907162427));
#28493=CARTESIAN_POINT('Ctrl Pts',(17.4183115332283,48.5308448973769,-36.5302421930502));
#28494=CARTESIAN_POINT('Ctrl Pts',(19.8188796334077,47.0350839014358,-36.3722936698577));
#28495=CARTESIAN_POINT('Ctrl Pts',(22.3836640619672,48.2275221588729,-36.2143451466653));
#28496=CARTESIAN_POINT('Ctrl Pts',(22.7872527811463,51.0270121670532,-36.0563966234728));
#28497=CARTESIAN_POINT('Ctrl Pts',(20.663724174252,52.8953414786953,-35.8984481002803));
#28498=CARTESIAN_POINT('Ctrl Pts',(17.9384170447561,52.1385527293516,-35.7404995770879));
#28499=CARTESIAN_POINT('Ctrl Pts',(17.0822844806015,49.4428032614878,-35.5825510538953));
#28500=CARTESIAN_POINT('Ctrl Pts',(18.8715558395627,47.2522471300393,-35.4246025307029));
#28501=CARTESIAN_POINT('Ctrl Pts',(21.683953198723,47.5529949566688,-35.2666540075104));
#28502=CARTESIAN_POINT('Ctrl Pts',(22.9695614077184,50.0723678337872,-35.108705484318));
#28503=CARTESIAN_POINT('Ctrl Pts',(21.5627586034653,52.5261269969816,-34.9507569611255));
#28504=CARTESIAN_POINT('Ctrl Pts',(18.7390501026036,52.6895236406911,-34.7928084379331));
#28505=CARTESIAN_POINT('Ctrl Pts',(17.0586065236542,50.4144109975506,-34.6348599147405));
#28506=CARTESIAN_POINT('Ctrl Pts',(18.0450349512685,47.7635645066714,-34.4769113915481));
#28507=CARTESIAN_POINT('Ctrl Pts',(20.8039707309936,47.1404260594826,-34.3189628683556));
#28508=CARTESIAN_POINT('Ctrl Pts',(22.8339707005912,49.1099763341506,-34.1610143451632));
#28509=CARTESIAN_POINT('Ctrl Pts',(22.2944956272855,51.8864839977984,-34.0030658219707));
#28510=CARTESIAN_POINT('Ctrl Pts',(19.67467115265,52.9525739954594,-33.8451172987782));
#28511=CARTESIAN_POINT('Ctrl Pts',(17.3498124494772,51.3416549499163,-33.6871687755857));
#28512=CARTESIAN_POINT('Ctrl Pts',(17.4277981965525,48.5142981658749,-33.5292202523933));
#28513=CARTESIAN_POINT('Ctrl Pts',(19.8379210888321,47.0339820492559,-33.3712717292008));
#28514=CARTESIAN_POINT('Ctrl Pts',(22.3949960004604,48.2428642012184,-33.2133232060084));
#28515=CARTESIAN_POINT('Ctrl Pts',(22.7806008789819,51.0448879410665,-33.0553746828159));
#28516=CARTESIAN_POINT('Ctrl Pts',(20.6451195086835,52.8995435635799,-32.8974261596234));
#28517=CARTESIAN_POINT('Ctrl Pts',(17.9247279002847,52.1252712226264,-32.7394776364309));
#28518=CARTESIAN_POINT('Ctrl Pts',(17.0859223881499,49.4240801013201,-32.5815291132385));
#28519=CARTESIAN_POINT('Ctrl Pts',(18.8892224190154,47.2450580363348,-32.423580590046));
#28520=CARTESIAN_POINT('Ctrl Pts',(21.6996306997866,47.5638580620325,-32.2656320668536));
#28521=CARTESIAN_POINT('Ctrl Pts',(22.9690355169923,50.0914338909774,-32.1076835436611));
#28522=CARTESIAN_POINT('Ctrl Pts',(21.5465061300745,52.5361093918092,-31.9497350204686));
#28523=CARTESIAN_POINT('Ctrl Pts',(18.721806669876,52.6813716393681,-31.7917864972762));
#28524=CARTESIAN_POINT('Ctrl Pts',(17.056006227608,50.3955157717439,-31.6338379740837));
#28525=CARTESIAN_POINT('Ctrl Pts',(18.0594354012447,47.7510577829479,-31.4758894508912));
#28526=CARTESIAN_POINT('Ctrl Pts',(20.8223154769685,47.1456473038675,-31.3179409276987));
#28527=CARTESIAN_POINT('Ctrl Pts',(22.8396271193197,49.1281916031572,-31.1599924045063));
#28528=CARTESIAN_POINT('Ctrl Pts',(22.2823352159385,51.9011780610106,-31.0020438813138));
#28529=CARTESIAN_POINT('Ctrl Pts',(19.6557193863538,52.9504241926626,-30.8440953581213));
#28530=CARTESIAN_POINT('Ctrl Pts',(17.3412523183405,51.3246104419229,-30.6861468349288));
#28531=CARTESIAN_POINT('Ctrl Pts',(17.4373909111324,48.4978126896975,-30.5281983117364));
#28532=CARTESIAN_POINT('Ctrl Pts',(19.8569692265682,47.0330024847609,-30.370249788544));
#28533=CARTESIAN_POINT('Ctrl Pts',(22.4062291941903,48.2582786897427,-30.2123012653514));
#28534=CARTESIAN_POINT('Ctrl Pts',(22.773834333593,51.0627206346725,-30.054352742159));
#28535=CARTESIAN_POINT('Ctrl Pts',(20.6264882450843,52.9036261013384,-29.8964042189665));
#28536=CARTESIAN_POINT('Ctrl Pts',(17.9111243185372,52.1119020917034,-29.738455695774));
#28537=CARTESIAN_POINT('Ctrl Pts',(17.0896804420887,49.4053806861463,-29.5805071725816));
#28538=CARTESIAN_POINT('Ctrl Pts',(18.9069347954335,47.2379825278782,-29.4225586493891));
#28539=CARTESIAN_POINT('Ctrl Pts',(21.7152381256765,47.5748216087247,-29.2646101261967));
#28540=CARTESIAN_POINT('Ctrl Pts',(22.9683872139918,50.1104961782632,-29.1066616030042));
#28541=CARTESIAN_POINT('Ctrl Pts',(21.5301898947694,52.5459872239793,-28.9487130798117));
#28542=CARTESIAN_POINT('Ctrl Pts',(18.7046159366362,52.6731090855795,-28.7907645566193));
#28543=CARTESIAN_POINT('Ctrl Pts',(17.0535273113208,50.3766042398849,-28.6328160334267));
#28544=CARTESIAN_POINT('Ctrl Pts',(18.0739158601312,47.7386437804777,-28.4748675102343));
#28545=CARTESIAN_POINT('Ctrl Pts',(20.840626318929,47.1509862358588,-28.3169189870418));
#28546=CARTESIAN_POINT('Ctrl Pts',(22.8451664617045,49.1464428092345,-28.1589704638493));
#28547=CARTESIAN_POINT('Ctrl Pts',(22.2700807037733,51.9157937538193,-28.0010219406569));
#28548=CARTESIAN_POINT('Ctrl Pts',(19.6367818165101,52.9481527160679,-27.8430734174644));
#28549=CARTESIAN_POINT('Ctrl Pts',(17.3328018026754,51.3075113781554,-27.685124894272));
#28550=CARTESIAN_POINT('Ctrl Pts',(17.4470892886469,48.4813890338076,-27.5271763710795));
#28551=CARTESIAN_POINT('Ctrl Pts',(19.8760232465397,47.0321454761979,-27.369227847887));
#28552=CARTESIAN_POINT('Ctrl Pts',(22.4173632095528,48.2737645355534,-27.2112793246945));
#28553=CARTESIAN_POINT('Ctrl Pts',(22.7669533650514,51.0805104150582,-27.0533308015021));
#28554=CARTESIAN_POINT('Ctrl Pts',(20.6078312689498,52.9075871271482,-26.8953822783096));
#28555=CARTESIAN_POINT('Ctrl Pts',(17.897606626764,52.0984494642799,-26.7374337551172));
#28556=CARTESIAN_POINT('Ctrl Pts',(17.0935589525871,49.3866986667662,-26.5794852319246));
#28557=CARTESIAN_POINT('Ctrl Pts',(18.9246913125752,47.2310350714261,-26.4215367087322));
#28558=CARTESIAN_POINT('Ctrl Pts',(21.7307766763484,47.5858569246444,-26.2635881855397));
#28559=CARTESIAN_POINT('Ctrl Pts',(22.9676128554771,50.129610091114,-26.1056396623473));
#28560=CARTESIAN_POINT('Ctrl Pts',(21.5138178763438,52.5556482381081,-25.9476911391548));
#28561=CARTESIAN_POINT('Ctrl Pts',(18.687464069051,52.6649589973579,-25.7897426159623));
#28562=CARTESIAN_POINT('Ctrl Pts',(17.0511987963454,50.3572337823409,-25.6317940927699));
#28563=CARTESIAN_POINT('Ctrl Pts',(18.0884185672411,47.7272068404143,-25.4738455695774));
#28564=CARTESIAN_POINT('Ctrl Pts',(20.859010980093,47.1546690443582,-25.3158970463849));
#28565=CARTESIAN_POINT('Ctrl Pts',(22.8504318621136,49.168429695793,-25.1579485231925));
#28566=CARTESIAN_POINT('Ctrl Pts',(22.4546613829867,51.0029999971534,-25.0526495077308));
#28567=CARTESIAN_POINT('Ctrl Pts',(21.9134659966651,51.6359872033749,-25.));
#28568=CARTESIAN_POINT('Ctrl Pts',(22.5149457203491,50.0017607375679,-39.112583302492));
#28569=CARTESIAN_POINT('Ctrl Pts',(22.5168589401434,50.2933091215384,-39.0941950563712));
#28570=CARTESIAN_POINT('Ctrl Pts',(22.4699889263606,50.5842626639725,-39.0758068102504));
#28571=CARTESIAN_POINT('Ctrl Pts',(22.3716201267472,50.856613814048,-39.0574185641297));
#28572=CARTESIAN_POINT('Ctrl Pts',(22.0899690741288,51.6364137953635,-39.0047690563988));
#28573=CARTESIAN_POINT('Ctrl Pts',(21.3861308782177,52.263711329065,-38.952119548668));
#28574=CARTESIAN_POINT('Ctrl Pts',(20.5791956005466,52.4541505635503,-38.8994700409372));
#28575=CARTESIAN_POINT('Ctrl Pts',(19.7722603228755,52.6445897980356,-38.8468205332064));
#28576=CARTESIAN_POINT('Ctrl Pts',(18.8622279634444,52.3981707333048,-38.7941710254756));
#28577=CARTESIAN_POINT('Ctrl Pts',(18.2616399582319,51.8265936861167,-38.7415215177447));
#28578=CARTESIAN_POINT('Ctrl Pts',(17.6610519530194,51.2550166389285,-38.6888720100139));
#28579=CARTESIAN_POINT('Ctrl Pts',(17.3699083020254,50.3582816092831,-38.6362225022831));
#28580=CARTESIAN_POINT('Ctrl Pts',(17.520198517985,49.5429148189582,-38.5835729945523));
#28581=CARTESIAN_POINT('Ctrl Pts',(17.6704887339445,48.7275480286333,-38.5309234868215));
#28582=CARTESIAN_POINT('Ctrl Pts',(18.2622128168577,47.993549477629,-38.4782739790906));
#28583=CARTESIAN_POINT('Ctrl Pts',(19.0271196598767,47.6736637193888,-38.4256244713598));
#28584=CARTESIAN_POINT('Ctrl Pts',(19.7920265028957,47.3537779611485,-38.372974963629));
#28585=CARTESIAN_POINT('Ctrl Pts',(20.7301161060206,47.4480049956724,-38.3203254558982));
#28586=CARTESIAN_POINT('Ctrl Pts',(21.4161208136638,47.913629699512,-38.2676759481674));
#28587=CARTESIAN_POINT('Ctrl Pts',(22.0897218255865,48.3708354128081,-38.2159783996089));
#28588=CARTESIAN_POINT('Ctrl Pts',(22.520271455965,49.1861296837586,-38.1642808510504));
#28589=CARTESIAN_POINT('Ctrl Pts',(22.5215367446411,50.0002732851607,-38.112583302492));
#28590=CARTESIAN_POINT('Origin',(20.,50.,-32.));
#28591=CARTESIAN_POINT('',(20.,47.4825,-24.3199761284063));
#28592=CARTESIAN_POINT('Ctrl Pts',(17.4825,50.,-25.));
#28593=CARTESIAN_POINT('Ctrl Pts',(17.4825,49.6777819917977,-25.));
#28594=CARTESIAN_POINT('Ctrl Pts',(17.5480817994189,49.3379042845386,-24.965994767533));
#28595=CARTESIAN_POINT('Ctrl Pts',(17.8069078640769,48.7191330360028,-24.8434341672334));
#28596=CARTESIAN_POINT('Ctrl Pts',(17.9998598225217,48.439857534204,-24.75619390213));
#28597=CARTESIAN_POINT('Ctrl Pts',(18.4404784589042,47.9992388978215,-24.5883213994305));
#28598=CARTESIAN_POINT('Ctrl Pts',(18.7195457648911,47.8067418484832,-24.4956547875015));
#28599=CARTESIAN_POINT('Ctrl Pts',(19.3374025937984,47.5482850278898,-24.3600905047278));
#28600=CARTESIAN_POINT('Ctrl Pts',(19.6768725637946,47.4825,-24.3199761284063));
#28601=CARTESIAN_POINT('Ctrl Pts',(20.,47.4825,-24.3199761284063));
#28602=CARTESIAN_POINT('Ctrl Pts',(20.,47.4825,-24.3199761284063));
#28603=CARTESIAN_POINT('Ctrl Pts',(20.3231274362054,47.4825,-24.3199761284063));
#28604=CARTESIAN_POINT('Ctrl Pts',(20.6625974062016,47.5482850278898,-24.3600905047278));
#28605=CARTESIAN_POINT('Ctrl Pts',(21.2804542351089,47.8067418484832,-24.4956547875015));
#28606=CARTESIAN_POINT('Ctrl Pts',(21.5595215410957,47.9992388978215,-24.5883213994305));
#28607=CARTESIAN_POINT('Ctrl Pts',(22.0001401774783,48.439857534204,-24.75619390213));
#28608=CARTESIAN_POINT('Ctrl Pts',(22.1930921359231,48.7191330360027,-24.8434341672334));
#28609=CARTESIAN_POINT('Ctrl Pts',(22.4519182005811,49.3379042845385,-24.965994767533));
#28610=CARTESIAN_POINT('Ctrl Pts',(22.5175,49.6777819917977,-25.));
#28611=CARTESIAN_POINT('Ctrl Pts',(22.5175,50.,-25.));
#28612=CARTESIAN_POINT('Origin',(20.,-50.,-25.));
#28613=CARTESIAN_POINT('',(17.2889091698078,-50.0014754277217,-25.));
#28614=CARTESIAN_POINT('',(20.,-50.,-25.));
#28615=CARTESIAN_POINT('Ctrl Pts',(17.2903183448191,-50.0029508554434,-25.));
#28616=CARTESIAN_POINT('Ctrl Pts',(17.3003555066451,-49.9104827882475,-25.));
#28617=CARTESIAN_POINT('Ctrl Pts',(17.314987256537,-49.8185880473882,-25.));
#28618=CARTESIAN_POINT('Ctrl Pts',(17.3341159214449,-49.7276468529595,-25.));
#28619=CARTESIAN_POINT('Ctrl Pts',(17.3530416128693,-49.6376706318372,-25.));
#28620=CARTESIAN_POINT('Ctrl Pts',(17.3763697440335,-49.548626955546,-25.));
#28621=CARTESIAN_POINT('Ctrl Pts',(17.4040502591901,-49.4609077193442,-25.));
#28622=CARTESIAN_POINT('Ctrl Pts',(17.4311163521567,-49.3751355800408,-25.));
#28623=CARTESIAN_POINT('Ctrl Pts',(17.4623442184204,-49.2906290498442,-25.));
#28624=CARTESIAN_POINT('Ctrl Pts',(17.4977230490407,-49.2077885578907,-25.));
#28625=CARTESIAN_POINT('Ctrl Pts',(17.5030373904386,-49.1953448832951,-25.));
#28626=CARTESIAN_POINT('Ctrl Pts',(17.5084454535136,-49.1829388756344,-25.));
#28627=CARTESIAN_POINT('Ctrl Pts',(17.5139472640597,-49.1705719750047,-25.));
#28628=CARTESIAN_POINT('Ctrl Pts',(17.5197445971897,-49.1575408024235,-25.));
#28629=CARTESIAN_POINT('Ctrl Pts',(17.5256427865735,-49.1445603815785,-25.));
#28630=CARTESIAN_POINT('Ctrl Pts',(17.5316393957237,-49.1316366890192,-25.));
#28631=CARTESIAN_POINT('Ctrl Pts',(17.5691316190762,-49.0508346964552,-25.));
#28632=CARTESIAN_POINT('Ctrl Pts',(17.6104933170903,-48.9721902576076,-25.));
#28633=CARTESIAN_POINT('Ctrl Pts',(17.6556547793454,-48.8960514827779,-25.));
#28634=CARTESIAN_POINT('Ctrl Pts',(17.7000564683813,-48.8211936275458,-25.));
#28635=CARTESIAN_POINT('Ctrl Pts',(17.7481316008788,-48.7487571677604,-25.));
#28636=CARTESIAN_POINT('Ctrl Pts',(17.7998501145092,-48.6791071342385,-25.));
#28637=CARTESIAN_POINT('Ctrl Pts',(17.8499884747111,-48.6115851150686,-25.));
#28638=CARTESIAN_POINT('Ctrl Pts',(17.9035514278317,-48.5466814150452,-25.));
#28639=CARTESIAN_POINT('Ctrl Pts',(17.9605392673115,-48.4847689190164,-25.));
#28640=CARTESIAN_POINT('Ctrl Pts',(17.9814440129101,-48.4620576706049,-25.));
#28641=CARTESIAN_POINT('Ctrl Pts',(18.0028098640902,-48.439749359775,-25.));
#28642=CARTESIAN_POINT('Ctrl Pts',(18.0246376377076,-48.4178639875036,-25.));
#28643=CARTESIAN_POINT('Ctrl Pts',(18.0437154987664,-48.3987357842003,-25.));
#28644=CARTESIAN_POINT('Ctrl Pts',(18.0631462461595,-48.3799306892336,-25.));
#28645=CARTESIAN_POINT('Ctrl Pts',(18.082919744614,-48.3614538208575,-25.));
#28646=CARTESIAN_POINT('Origin',(20.,-50.,-25.));
#28647=CARTESIAN_POINT('',(22.7115649000387,-50.0018225476882,-25.));
#28648=CARTESIAN_POINT('',(20.,-50.,-25.));
#28649=CARTESIAN_POINT('Ctrl Pts',(22.7106298000774,-50.0036450953763,-25.));
#28650=CARTESIAN_POINT('Ctrl Pts',(22.7207569197221,-50.0952816165228,-25.));
#28651=CARTESIAN_POINT('Ctrl Pts',(22.7262771338965,-50.1873822523437,-25.));
#28652=CARTESIAN_POINT('Ctrl Pts',(22.7270618926046,-50.2795961166426,-25.));
#28653=CARTESIAN_POINT('Ctrl Pts',(22.7273478963458,-50.3132032750016,-25.));
#28654=CARTESIAN_POINT('Ctrl Pts',(22.7270044421126,-50.3468255682447,-25.));
#28655=CARTESIAN_POINT('Ctrl Pts',(22.7260235824556,-50.3804462077869,-25.));
#28656=CARTESIAN_POINT('Ctrl Pts',(22.7254183178835,-50.4011926844725,-25.));
#28657=CARTESIAN_POINT('Ctrl Pts',(22.72456984669,-50.4219453082198,-25.));
#28658=CARTESIAN_POINT('Ctrl Pts',(22.723478332626,-50.4426647798907,-25.));
#28659=CARTESIAN_POINT('Ctrl Pts',(22.7184413506502,-50.5382783947722,-25.));
#28660=CARTESIAN_POINT('Ctrl Pts',(22.7082324366332,-50.6332960684915,-25.));
#28661=CARTESIAN_POINT('Ctrl Pts',(22.6927834477001,-50.7273214749238,-25.));
#28662=CARTESIAN_POINT('Ctrl Pts',(22.6895870066842,-50.7467756066445,-25.));
#28663=CARTESIAN_POINT('Ctrl Pts',(22.6861660794599,-50.7661873278843,-25.));
#28664=CARTESIAN_POINT('Ctrl Pts',(22.6825197987883,-50.7855532193863,-25.));
#28665=CARTESIAN_POINT('Ctrl Pts',(22.665577577038,-50.8755356584169,-25.));
#28666=CARTESIAN_POINT('Ctrl Pts',(22.6437744061299,-50.964528503021,-25.));
#28667=CARTESIAN_POINT('Ctrl Pts',(22.6174131158025,-51.0522992055656,-25.));
#28668=CARTESIAN_POINT('Ctrl Pts',(22.590454590549,-51.1420584196133,-25.));
#28669=CARTESIAN_POINT('Ctrl Pts',(22.558728861846,-51.2305401876501,-25.));
#28670=CARTESIAN_POINT('Ctrl Pts',(22.5225055623892,-51.3174921359681,-25.));
#28671=CARTESIAN_POINT('Ctrl Pts',(22.5100288523632,-51.3474417612542,-25.));
#28672=CARTESIAN_POINT('Ctrl Pts',(22.4970181100108,-51.3772098108535,-25.));
#28673=CARTESIAN_POINT('Ctrl Pts',(22.4834829864678,-51.4067856342665,-25.));
#28674=CARTESIAN_POINT('Ctrl Pts',(22.4768071327121,-51.4213731532634,-25.));
#28675=CARTESIAN_POINT('Ctrl Pts',(22.4700037022852,-51.4359139058754,-25.));
#28676=CARTESIAN_POINT('Ctrl Pts',(22.4630737944401,-51.4504065918778,-25.));
#28677=CARTESIAN_POINT('Ctrl Pts',(22.4569722275614,-51.4631669481296,-25.));
#28678=CARTESIAN_POINT('Ctrl Pts',(22.4507733728518,-51.4758883159868,-25.));
#28679=CARTESIAN_POINT('Ctrl Pts',(22.4444834321049,-51.4885593435834,-25.));
#28680=CARTESIAN_POINT('Ctrl Pts',(22.4016240141549,-51.5748992455749,-25.));
#28681=CARTESIAN_POINT('Ctrl Pts',(22.3544754754652,-51.6590378348422,-25.));
#28682=CARTESIAN_POINT('Ctrl Pts',(22.303380378344,-51.7407248629369,-25.));
#28683=CARTESIAN_POINT('Ctrl Pts',(22.2512756047644,-51.8240260864021,-25.));
#28684=CARTESIAN_POINT('Ctrl Pts',(22.1950664422593,-51.9047786755034,-25.));
#28685=CARTESIAN_POINT('Ctrl Pts',(22.1350611970561,-51.9827100860122,-25.));
#28686=CARTESIAN_POINT('Ctrl Pts',(22.0745775675633,-52.0612627949147,-25.));
#28687=CARTESIAN_POINT('Ctrl Pts',(22.0102366253224,-52.1369500006744,-25.));
#28688=CARTESIAN_POINT('Ctrl Pts',(21.9423048690762,-52.2094731543011,-25.));
#28689=CARTESIAN_POINT('Ctrl Pts',(21.9053590736893,-52.2489160561597,-25.));
#28690=CARTESIAN_POINT('Ctrl Pts',(21.8673503377721,-52.2874226510328,-25.));
#28691=CARTESIAN_POINT('Ctrl Pts',(21.8283162532303,-52.3249411517793,-25.));
#28692=CARTESIAN_POINT('Ctrl Pts',(21.815658940581,-52.3371070165525,-25.));
#28693=CARTESIAN_POINT('Ctrl Pts',(21.80289378929,-52.3491689621023,-25.));
#28694=CARTESIAN_POINT('Ctrl Pts',(21.7900220062658,-52.361125148447,-25.));
#28695=CARTESIAN_POINT('Ctrl Pts',(21.7785378626427,-52.3717924010652,-25.));
#28696=CARTESIAN_POINT('Ctrl Pts',(21.7669742197933,-52.3823704194089,-25.));
#28697=CARTESIAN_POINT('Ctrl Pts',(21.755337497437,-52.3928534389456,-25.));
#28698=CARTESIAN_POINT('Ctrl Pts',(21.6795227363725,-52.4611516759468,-25.));
#28699=CARTESIAN_POINT('Ctrl Pts',(21.6005417920538,-52.5254825537856,-25.));
#28700=CARTESIAN_POINT('Ctrl Pts',(21.5187210399691,-52.5855630198017,-25.));
#28701=CARTESIAN_POINT('Ctrl Pts',(21.4368278994846,-52.6456966401667,-25.));
#28702=CARTESIAN_POINT('Ctrl Pts',(21.3520893470422,-52.7015731625802,-25.));
#28703=CARTESIAN_POINT('Ctrl Pts',(21.2647876555901,-52.7528825881287,-25.));
#28704=CARTESIAN_POINT('Ctrl Pts',(21.1792482097518,-52.8031562970879,-25.));
#28705=CARTESIAN_POINT('Ctrl Pts',(21.0912473933424,-52.8490461032894,-25.));
#28706=CARTESIAN_POINT('Ctrl Pts',(21.0010169754817,-52.8902242643499,-25.));
#28707=CARTESIAN_POINT('Ctrl Pts',(20.9635971996838,-52.9073014051988,-25.));
#28708=CARTESIAN_POINT('Ctrl Pts',(20.9257936105469,-52.9235677108145,-25.));
#28709=CARTESIAN_POINT('Ctrl Pts',(20.8876213902621,-52.9389975058256,-25.));
#28710=CARTESIAN_POINT('Ctrl Pts',(20.8571996693011,-52.9512944305214,-25.));
#28711=CARTESIAN_POINT('Ctrl Pts',(20.8265437968036,-52.9630600190333,-25.));
#28712=CARTESIAN_POINT('Ctrl Pts',(20.7956660331737,-52.9742969611506,-25.));
#28713=CARTESIAN_POINT('Ctrl Pts',(19.2062007174671,-52.9692229537457,-25.));
#28714=CARTESIAN_POINT('Ctrl Pts',(19.1113557340264,-52.9345282351333,-25.));
#28715=CARTESIAN_POINT('Ctrl Pts',(19.0185538161309,-52.8948451940055,-25.));
#28716=CARTESIAN_POINT('Ctrl Pts',(18.9280360947249,-52.8504935528002,-25.));
#28717=CARTESIAN_POINT('Ctrl Pts',(18.8362532909695,-52.8055220497869,-25.));
#28718=CARTESIAN_POINT('Ctrl Pts',(18.7468183096923,-52.7557498361634,-25.));
#28719=CARTESIAN_POINT('Ctrl Pts',(18.6600165620743,-52.7014695591135,-25.));
#28720=CARTESIAN_POINT('Ctrl Pts',(18.6355003880952,-52.6861387074624,-25.));
#28721=CARTESIAN_POINT('Ctrl Pts',(18.6111945114723,-52.670448030549,-25.));
#28722=CARTESIAN_POINT('Ctrl Pts',(18.5871059592391,-52.6544036660335,-25.));
#28723=CARTESIAN_POINT('Ctrl Pts',(18.5677885117881,-52.6415371323618,-25.));
#28724=CARTESIAN_POINT('Ctrl Pts',(18.5486087336159,-52.6284415254607,-25.));
#28725=CARTESIAN_POINT('Ctrl Pts',(18.529589504657,-52.6151337510479,-25.));
#28726=CARTESIAN_POINT('Ctrl Pts',(18.4468808900083,-52.5572624467948,-25.));
#28727=CARTESIAN_POINT('Ctrl Pts',(18.3671268631708,-52.4953308830207,-25.));
#28728=CARTESIAN_POINT('Ctrl Pts',(18.290593905947,-52.4296356749819,-25.));
#28729=CARTESIAN_POINT('Ctrl Pts',(18.2315992466026,-52.3789951854543,-25.));
#28730=CARTESIAN_POINT('Ctrl Pts',(18.1745191630826,-52.3261174497872,-25.));
#28731=CARTESIAN_POINT('Ctrl Pts',(18.119493278307,-52.2711265564765,-25.));
#28732=CARTESIAN_POINT('Ctrl Pts',(18.0902009918943,-52.2418528972976,-25.));
#28733=CARTESIAN_POINT('Ctrl Pts',(18.0614911051503,-52.2119802581191,-25.));
#28734=CARTESIAN_POINT('Ctrl Pts',(18.0333867031721,-52.1815265260884,-25.));
#28735=CARTESIAN_POINT('Ctrl Pts',(18.0237500866723,-52.1710843563246,-25.));
#28736=CARTESIAN_POINT('Ctrl Pts',(18.0141853970817,-52.1605745812859,-25.));
#28737=CARTESIAN_POINT('Ctrl Pts',(18.0047001952164,-52.1500055259558,-25.));
#28738=CARTESIAN_POINT('Ctrl Pts',(17.938901944737,-52.0766886519643,-25.));
#28739=CARTESIAN_POINT('Ctrl Pts',(17.8768357908346,-52.0004252935808,-25.));
#28740=CARTESIAN_POINT('Ctrl Pts',(17.8187456099699,-51.9214932933958,-25.));
#28741=CARTESIAN_POINT('Ctrl Pts',(17.7611818199286,-51.8432765445658,-25.));
#28742=CARTESIAN_POINT('Ctrl Pts',(17.7075218378801,-51.7624385159295,-25.));
#28743=CARTESIAN_POINT('Ctrl Pts',(17.6580487138489,-51.6792271703209,-25.));
#28744=CARTESIAN_POINT('Ctrl Pts',(17.6099913564333,-51.5983970740766,-25.));
#28745=CARTESIAN_POINT('Ctrl Pts',(17.5658844479073,-51.5153268531393,-25.));
#28746=CARTESIAN_POINT('Ctrl Pts',(17.5260352107221,-51.4302334377047,-25.));
#28747=CARTESIAN_POINT('Ctrl Pts',(17.5052301251829,-51.3858065951351,-25.));
#28748=CARTESIAN_POINT('Ctrl Pts',(17.4855864271477,-51.340828153884,-25.));
#28749=CARTESIAN_POINT('Ctrl Pts',(17.4671535333325,-51.2953287461456,-25.));
#28750=CARTESIAN_POINT('Ctrl Pts',(17.4600944809444,-51.2779043142537,-25.));
#28751=CARTESIAN_POINT('Ctrl Pts',(17.4532130454223,-51.2604034796238,-25.));
#28752=CARTESIAN_POINT('Ctrl Pts',(17.4465121643074,-51.2428279712876,-25.));
#28753=CARTESIAN_POINT('Ctrl Pts',(17.441270730006,-51.2290803953082,-25.));
#28754=CARTESIAN_POINT('Ctrl Pts',(17.4361396681845,-51.2152866325184,-25.));
#28755=CARTESIAN_POINT('Ctrl Pts',(17.4311255127051,-51.2014622180439,-25.));
#28756=CARTESIAN_POINT('Ctrl Pts',(17.3994430851164,-51.1141113147183,-25.));
#28757=CARTESIAN_POINT('Ctrl Pts',(17.3723694636016,-51.0253970866411,-25.));
#28758=CARTESIAN_POINT('Ctrl Pts',(17.3501559694963,-50.9355424162655,-25.));
#28759=CARTESIAN_POINT('Ctrl Pts',(17.3451710965855,-50.9153783614734,-25.));
#28760=CARTESIAN_POINT('Ctrl Pts',(17.3404311765996,-50.8951568357486,-25.));
#28761=CARTESIAN_POINT('Ctrl Pts',(17.3359394106852,-50.874880302046,-25.));
#28762=CARTESIAN_POINT('Ctrl Pts',(17.3155162874091,-50.7826871300692,-25.));
#28763=CARTESIAN_POINT('Ctrl Pts',(17.3002191225768,-50.6893564399051,-25.));
#28764=CARTESIAN_POINT('Ctrl Pts',(17.2899371061862,-50.5952837977441,-25.));
#28765=CARTESIAN_POINT('Ctrl Pts',(17.2792458523533,-50.4974669437472,-25.));
#28766=CARTESIAN_POINT('Ctrl Pts',(17.2739769598257,-50.3988466706342,-25.));
#28767=CARTESIAN_POINT('Ctrl Pts',(17.2740631823385,-50.2998823144491,-25.));
#28768=CARTESIAN_POINT('Ctrl Pts',(17.274090511577,-50.2685143990752,-25.));
#28769=CARTESIAN_POINT('Ctrl Pts',(17.274656255105,-50.2371120997174,-25.));
#28770=CARTESIAN_POINT('Ctrl Pts',(17.275759389936,-50.2056906513608,-25.));
#28771=CARTESIAN_POINT('Ctrl Pts',(17.2762350449305,-50.1921421997773,-25.));
#28772=CARTESIAN_POINT('Ctrl Pts',(17.2768107459306,-50.1785876877151,-25.));
#28773=CARTESIAN_POINT('Ctrl Pts',(17.2774860299861,-50.1650364244566,-25.));
#28774=CARTESIAN_POINT('Ctrl Pts',(17.2801856482179,-50.1108618336893,-25.));
#28775=CARTESIAN_POINT('Ctrl Pts',(17.2844721992041,-50.0568088877183,-25.));
#28776=CARTESIAN_POINT('Ctrl Pts',(17.2903183448191,-50.0029508554434,-25.));
#28777=CARTESIAN_POINT('',(20.,-50.,-25.));
#28778=CARTESIAN_POINT('Origin',(20.,-50.,-25.));
#28779=CARTESIAN_POINT('Origin',(20.,-50.,-25.));
#28780=CARTESIAN_POINT('',(20.,-50.,-25.));
#28781=CARTESIAN_POINT('Ctrl Pts',(21.9134659966651,-48.3640127966251,-25.));
#28782=CARTESIAN_POINT('Ctrl Pts',(21.9760669288874,-48.422842301107,-25.));
#28783=CARTESIAN_POINT('Ctrl Pts',(22.0352442468464,-48.4849719549136,-25.));
#28784=CARTESIAN_POINT('Ctrl Pts',(22.0909851470911,-48.5500174517208,-25.));
#28785=CARTESIAN_POINT('Ctrl Pts',(22.1343868534266,-48.6006640243179,-25.));
#28786=CARTESIAN_POINT('Ctrl Pts',(22.1757047718733,-48.6530795405248,-25.));
#28787=CARTESIAN_POINT('Ctrl Pts',(22.2149215330014,-48.7071012290448,-25.));
#28788=CARTESIAN_POINT('Ctrl Pts',(22.2385444426018,-48.7396421484798,-25.));
#28789=CARTESIAN_POINT('Ctrl Pts',(22.2614047541017,-48.7727661601668,-25.));
#28790=CARTESIAN_POINT('Ctrl Pts',(22.2834966880046,-48.8064400758587,-25.));
#28791=CARTESIAN_POINT('Ctrl Pts',(22.2954178781671,-48.8246111039924,-25.));
#28792=CARTESIAN_POINT('Ctrl Pts',(22.3071166390413,-48.8429446974121,-25.));
#28793=CARTESIAN_POINT('Ctrl Pts',(22.3185793921054,-48.8614149655927,-25.));
#28794=CARTESIAN_POINT('Ctrl Pts',(22.3655669620942,-48.9371274069235,-25.));
#28795=CARTESIAN_POINT('Ctrl Pts',(22.4086383333277,-49.0152023023888,-25.));
#28796=CARTESIAN_POINT('Ctrl Pts',(22.4477590648795,-49.0952575499459,-25.));
#28797=CARTESIAN_POINT('Ctrl Pts',(22.4825526073179,-49.1664577944914,-25.));
#28798=CARTESIAN_POINT('Ctrl Pts',(22.5142209063364,-49.2392255216741,-25.));
#28799=CARTESIAN_POINT('Ctrl Pts',(22.5427164245852,-49.3133158126709,-25.));
#28800=CARTESIAN_POINT('Ctrl Pts',(22.5500217400807,-49.3323101312216,-25.));
#28801=CARTESIAN_POINT('Ctrl Pts',(22.5571184055396,-49.3513914697327,-25.));
#28802=CARTESIAN_POINT('Ctrl Pts',(22.5640053609969,-49.37055588476,-25.));
#28803=CARTESIAN_POINT('Ctrl Pts',(22.5692935788638,-49.3852714731768,-25.));
#28804=CARTESIAN_POINT('Ctrl Pts',(22.5744581966978,-49.4000364270766,-25.));
#28805=CARTESIAN_POINT('Ctrl Pts',(22.5794941881025,-49.414835045487,-25.));
#28806=CARTESIAN_POINT('Ctrl Pts',(22.6091522636753,-49.5019874069421,-25.));
#28807=CARTESIAN_POINT('Ctrl Pts',(22.6343955017318,-49.5904229013513,-25.));
#28808=CARTESIAN_POINT('Ctrl Pts',(22.6551918733353,-49.6797461904936,-25.));
#28809=CARTESIAN_POINT('Ctrl Pts',(22.6763394154917,-49.7705778056766,-25.));
#28810=CARTESIAN_POINT('Ctrl Pts',(22.6928891491029,-49.8623282425449,-25.));
#28811=CARTESIAN_POINT('Ctrl Pts',(22.7047658933192,-49.9546151098704,-25.));
#28812=CARTESIAN_POINT('Ctrl Pts',(22.706867096187,-49.9709422637395,-25.));
#28813=CARTESIAN_POINT('Ctrl Pts',(22.7088219209409,-49.9872862726765,-25.));
#28814=CARTESIAN_POINT('Ctrl Pts',(22.7106298000774,-50.0036450953763,-25.));
#28815=CARTESIAN_POINT('Origin',(20.,-50.,-42.2084234471774));
#28816=CARTESIAN_POINT('Ctrl Pts',(23.0767447721987,-49.9980895972329,-39.7084234471774));
#28817=CARTESIAN_POINT('Ctrl Pts',(23.0776699202316,-49.8748204878272,-39.7020198504181));
#28818=CARTESIAN_POINT('Ctrl Pts',(23.0151644566962,-48.7389614167051,-39.642966745928));
#28819=CARTESIAN_POINT('Ctrl Pts',(21.6024148578293,-46.7464740991412,-39.5312641337071));
#28820=CARTESIAN_POINT('Ctrl Pts',(18.1518492862868,-46.8799264325519,-39.3733156105146));
#28821=CARTESIAN_POINT('Ctrl Pts',(16.3769778256201,-49.8417650264767,-39.2153670873222));
#28822=CARTESIAN_POINT('Ctrl Pts',(17.8869742727072,-52.9473163426722,-39.0574185641297));
#28823=CARTESIAN_POINT('Ctrl Pts',(21.3127949729971,-53.3805020684052,-38.8994700409372));
#28824=CARTESIAN_POINT('Ctrl Pts',(22.9593111902465,-51.4421740844442,-38.7831383352865));
#28825=CARTESIAN_POINT('Ctrl Pts',(23.0761866233546,-50.2155563599539,-38.7194561373666));
#28826=CARTESIAN_POINT('Ctrl Pts',(23.0742548311415,-50.0026845243509,-38.7084234471775));
#28827=CARTESIAN_POINT('Ctrl Pts',(23.0703065393339,-50.0033432771247,-39.7915765528225));
#28828=CARTESIAN_POINT('Ctrl Pts',(23.0652969395396,-49.3102241888876,-39.7557520197534));
#28829=CARTESIAN_POINT('Ctrl Pts',(22.4928180780877,-47.5885986835485,-39.6672779789534));
#28830=CARTESIAN_POINT('Ctrl Pts',(19.6484750771286,-46.3913839963408,-39.5261544304226));
#28831=CARTESIAN_POINT('Ctrl Pts',(16.7861445447059,-48.3201950030769,-39.3682059072301));
#28832=CARTESIAN_POINT('Ctrl Pts',(16.8365146481096,-51.7735627154933,-39.2102573840377));
#28833=CARTESIAN_POINT('Ctrl Pts',(19.7557254203512,-53.6181280557829,-39.0523088608451));
#28834=CARTESIAN_POINT('Ctrl Pts',(22.5305077858237,-52.349751264392,-38.9127485837735));
#28835=CARTESIAN_POINT('Ctrl Pts',(23.0660296945049,-50.6610395723575,-38.8258378144326));
#28836=CARTESIAN_POINT('Ctrl Pts',(23.0703817199364,-49.9978503929169,-38.7915765528226));
#28837=CARTESIAN_POINT('Ctrl Pts',(18.086534003335,-48.364012796625,-40.));
#28838=CARTESIAN_POINT('Ctrl Pts',(17.5453386170133,-48.9970000028465,-39.9473504922692));
#28839=CARTESIAN_POINT('Ctrl Pts',(17.1495688120533,-50.8315710151824,-39.8420514768075));
#28840=CARTESIAN_POINT('Ctrl Pts',(19.1409886760425,-52.8453306902491,-39.684102953615));
#28841=CARTESIAN_POINT('Ctrl Pts',(21.9115816382771,-52.2727934305225,-39.5261544304226));
#28842=CARTESIAN_POINT('Ctrl Pts',(22.9488012054458,-49.6427660783584,-39.3682059072301));
#28843=CARTESIAN_POINT('Ctrl Pts',(21.3125360027934,-47.3350410101149,-39.2102573840377));
#28844=CARTESIAN_POINT('Ctrl Pts',(18.4861820654716,-47.4443516492433,-39.0523088608452));
#28845=CARTESIAN_POINT('Ctrl Pts',(17.0323870753209,-49.8703899313991,-38.8943603376527));
#28846=CARTESIAN_POINT('Ctrl Pts',(18.2692232736426,-52.4141431243459,-38.7364118144602));
#28847=CARTESIAN_POINT('Ctrl Pts',(21.0753087179177,-52.7689650096666,-38.5784632912678));
#28848=CARTESIAN_POINT('Ctrl Pts',(22.9064411229281,-50.6133013449025,-38.4205147680753));
#28849=CARTESIAN_POINT('Ctrl Pts',(22.1023934291463,-47.9015504828899,-38.2625662448829));
#28850=CARTESIAN_POINT('Ctrl Pts',(19.3921687147818,-47.0924127949112,-38.1046177216903));
#28851=CARTESIAN_POINT('Ctrl Pts',(17.233046562173,-48.9194895571954,-37.9466691984979));
#28852=CARTESIAN_POINT('Ctrl Pts',(17.5826367266969,-51.7262355095391,-37.7887206753054));
#28853=CARTESIAN_POINT('Ctrl Pts',(20.1239767567563,-52.9678546022029,-37.630772152113));
#28854=CARTESIAN_POINT('Ctrl Pts',(22.5529107785992,-51.518611006092,-37.4728236289205));
#28855=CARTESIAN_POINT('Ctrl Pts',(22.6671982676034,-48.692488587455,-37.314875105728));
#28856=CARTESIAN_POINT('Ctrl Pts',(20.3632181930562,-47.0518472062269,-37.1569265825356));
#28857=CARTESIAN_POINT('Ctrl Pts',(17.7299192364194,-48.0842061957224,-36.9989780593431));
#28858=CARTESIAN_POINT('Ctrl Pts',(17.154833463334,-50.853557213245,-36.8410295361506));
#28859=CARTESIAN_POINT('Ctrl Pts',(19.1593736589235,-52.8490138392078,-36.6830810129582));
#28860=CARTESIAN_POINT('Ctrl Pts',(21.9260841906145,-52.2613562790991,-36.5251324897657));
#28861=CARTESIAN_POINT('Ctrl Pts',(22.9464727663089,-49.6233957501942,-36.3671839665733));
#28862=CARTESIAN_POINT('Ctrl Pts',(21.2953840974929,-47.3268908439923,-36.2092354433807));
#28863=CARTESIAN_POINT('Ctrl Pts',(18.4698100649153,-47.4540127089428,-36.0512869201883));
#28864=CARTESIAN_POINT('Ctrl Pts',(17.0316127078011,-49.8895038188253,-35.8933383969958));
#28865=CARTESIAN_POINT('Ctrl Pts',(18.2847618291327,-52.4251784551708,-35.7353898738034));
#28866=CARTESIAN_POINT('Ctrl Pts',(21.0930652333649,-52.7620175448917,-35.5774413506109));
#28867=CARTESIAN_POINT('Ctrl Pts',(22.9103196345885,-50.5946193295201,-35.4194928274184));
#28868=CARTESIAN_POINT('Ctrl Pts',(22.0888757364977,-47.8880978526551,-35.2615443042259));
#28869=CARTESIAN_POINT('Ctrl Pts',(19.3735117384099,-47.0963738221607,-35.1035957810335));
#28870=CARTESIAN_POINT('Ctrl Pts',(17.2261655933258,-48.9372793373283,-34.945647257841));
#28871=CARTESIAN_POINT('Ctrl Pts',(17.5937707424136,-51.7417213561457,-34.7876987346485));
#28872=CARTESIAN_POINT('Ctrl Pts',(20.1430307772,-52.9669975934097,-34.6297502114561));
#28873=CARTESIAN_POINT('Ctrl Pts',(22.5626091563838,-51.5021873498801,-34.4718016882636));
#28874=CARTESIAN_POINT('Ctrl Pts',(22.6587477517086,-48.6753895231782,-34.3138531650711));
#28875=CARTESIAN_POINT('Ctrl Pts',(20.344280622717,-47.0495757296036,-34.1559046418787));
#28876=CARTESIAN_POINT('Ctrl Pts',(17.7176647239296,-48.0988218888997,-33.9979561186862));
#28877=CARTESIAN_POINT('Ctrl Pts',(17.1603728058656,-50.8718084198119,-33.8400075954937));
#28878=CARTESIAN_POINT('Ctrl Pts',(19.1776845013661,-52.8543527713352,-33.6820590723013));
#28879=CARTESIAN_POINT('Ctrl Pts',(21.9405646498826,-52.2489422763042,-33.5241105491088));
#28880=CARTESIAN_POINT('Ctrl Pts',(22.9439938499564,-49.6044842178357,-33.3661620259164));
#28881=CARTESIAN_POINT('Ctrl Pts',(21.2781933638003,-47.3186282899868,-33.2082135027238));
#28882=CARTESIAN_POINT('Ctrl Pts',(18.4534938291803,-47.4638905413727,-33.0502649795314));
#28883=CARTESIAN_POINT('Ctrl Pts',(17.0309644047835,-49.9085661066135,-32.8923164563389));
#28884=CARTESIAN_POINT('Ctrl Pts',(18.3003692554337,-52.4361420021517,-32.7343679331465));
#28885=CARTESIAN_POINT('Ctrl Pts',(21.1107776102498,-52.7549420362487,-32.576419409954));
#28886=CARTESIAN_POINT('Ctrl Pts',(22.9140776886262,-50.5759199138536,-32.4184708867615));
#28887=CARTESIAN_POINT('Ctrl Pts',(22.0752721543919,-47.8747287213798,-32.260522363569));
#28888=CARTESIAN_POINT('Ctrl Pts',(19.3548804743199,-47.1004563600269,-32.1025738403766));
#28889=CARTESIAN_POINT('Ctrl Pts',(17.2193990477586,-48.9551120314041,-31.9446253171841));
#28890=CARTESIAN_POINT('Ctrl Pts',(17.6050039364394,-51.7571358450762,-31.7866767939917));
#28891=CARTESIAN_POINT('Ctrl Pts',(20.162078915438,-52.9660180288887,-31.6287282707991));
#28892=CARTESIAN_POINT('Ctrl Pts',(22.5722018712164,-51.4857018732685,-31.4707797476068));
#28893=CARTESIAN_POINT('Ctrl Pts',(22.6501876203464,-48.6583450147357,-31.3128312244142));
#28894=CARTESIAN_POINT('Ctrl Pts',(20.3253288559214,-47.0474259267501,-31.1548827012218));
#28895=CARTESIAN_POINT('Ctrl Pts',(17.7055043122623,-48.1135159524991,-30.9969341780293));
#28896=CARTESIAN_POINT('Ctrl Pts',(17.1660292247431,-50.8900236892983,-30.8389856548368));
#28897=CARTESIAN_POINT('Ctrl Pts',(19.1960292478244,-52.8595740158577,-30.6810371316444));
#28898=CARTESIAN_POINT('Ctrl Pts',(21.9549651002382,-52.2364355522512,-30.5230886084519));
#28899=CARTESIAN_POINT('Ctrl Pts',(22.9413935538417,-49.5855889915311,-30.3651400852594));
#28900=CARTESIAN_POINT('Ctrl Pts',(21.2609499306183,-47.310476288449,-30.207191562067));
#28901=CARTESIAN_POINT('Ctrl Pts',(18.4372413553613,-47.4738729364634,-30.0492430388745));
#28902=CARTESIAN_POINT('Ctrl Pts',(17.0304385140436,-49.9276321643062,-29.8912945156821));
#28903=CARTESIAN_POINT('Ctrl Pts',(18.3160467569104,-52.4470051078016,-29.7333459924895));
#28904=CARTESIAN_POINT('Ctrl Pts',(21.128444190168,-52.7477529423549,-29.5753974692971));
#28905=CARTESIAN_POINT('Ctrl Pts',(22.9177155962706,-50.5571967531925,-29.4174489461046));
#28906=CARTESIAN_POINT('Ctrl Pts',(22.0615830095597,-47.8614472143047,-29.2595004229122));
#28907=CARTESIAN_POINT('Ctrl Pts',(19.3362758082611,-47.1046584450221,-29.1015518997197));
#28908=CARTESIAN_POINT('Ctrl Pts',(17.2127471454189,-48.9729878058884,-28.9436033765272));
#28909=CARTESIAN_POINT('Ctrl Pts',(17.6163358752312,-51.7724778878259,-28.7856548533347));
#28910=CARTESIAN_POINT('Ctrl Pts',(20.181120371364,-52.9649161766797,-28.6277063301423));
#28911=CARTESIAN_POINT('Ctrl Pts',(22.5816885347909,-51.4691551413309,-28.4697578069498));
#28912=CARTESIAN_POINT('Ctrl Pts',(22.6415182232601,-48.6413558229776,-28.3118092837573));
#28913=CARTESIAN_POINT('Ctrl Pts',(20.3063636747943,-47.045397856035,-28.1538607605649));
#28914=CARTESIAN_POINT('Ctrl Pts',(17.6934385041046,-48.1282877980411,-27.9959122373724));
#28915=CARTESIAN_POINT('Ctrl Pts',(17.1718024827192,-50.9082022577011,-27.8379637141799));
#28916=CARTESIAN_POINT('Ctrl Pts',(19.2144071506939,-52.8646773725511,-27.6800151909875));
#28917=CARTESIAN_POINT('Ctrl Pts',(21.969284930193,-52.2238365980696,-27.522066667795));
#28918=CARTESIAN_POINT('Ctrl Pts',(22.9386720207179,-49.5667108964077,-27.3641181446025));
#28919=CARTESIAN_POINT('Ctrl Pts',(21.2436544380323,-47.3024350851045,-27.2061696214101));
#28920=CARTESIAN_POINT('Ctrl Pts',(18.4210534546561,-47.4839596618936,-27.0482210982176));
#28921=CARTESIAN_POINT('Ctrl Pts',(17.0300347762909,-49.9467008492878,-26.8902725750251));
#28922=CARTESIAN_POINT('Ctrl Pts',(18.3317942465966,-52.4577680338926,-26.7323240518326));
#28923=CARTESIAN_POINT('Ctrl Pts',(21.146063130971,-52.7404491468214,-26.5743755286402));
#28924=CARTESIAN_POINT('Ctrl Pts',(22.9212354249696,-50.5384534322301,-26.4164270054477));
#28925=CARTESIAN_POINT('Ctrl Pts',(22.0478044516093,-47.8482482790349,-26.2584784822553));
#28926=CARTESIAN_POINT('Ctrl Pts',(19.3177072968886,-47.1089910531324,-26.1005299590628));
#28927=CARTESIAN_POINT('Ctrl Pts',(17.2061926609974,-48.9908837262921,-25.9425814358703));
#28928=CARTESIAN_POINT('Ctrl Pts',(17.6278009322015,-51.7877910457717,-25.7846329126779));
#28929=CARTESIAN_POINT('Ctrl Pts',(20.2000849941159,-52.9636040941318,-25.6266843894854));
#28930=CARTESIAN_POINT('Ctrl Pts',(22.5912068609734,-51.4527230224798,-25.4687358662929));
#28931=CARTESIAN_POINT('Ctrl Pts',(22.63246493662,-48.6240737732433,-25.3107873431004));
#28932=CARTESIAN_POINT('Ctrl Pts',(20.2879336158885,-47.044187324869,-25.152838819908));
#28933=CARTESIAN_POINT('Ctrl Pts',(17.6803736923545,-48.1417371056711,-24.9948902967155));
#28934=CARTESIAN_POINT('Ctrl Pts',(17.1799177684998,-50.9293032433429,-24.836941773523));
#28935=CARTESIAN_POINT('Ctrl Pts',(18.5452496035378,-52.2169963426693,-24.7316427580614));
#28936=CARTESIAN_POINT('Ctrl Pts',(19.3498000020249,-52.4320868020351,-24.6789932503306));
#28937=CARTESIAN_POINT('Ctrl Pts',(17.9456684496579,-48.2435746787731,-40.1070022498898));
#28938=CARTESIAN_POINT('Ctrl Pts',(17.3646313374449,-48.9231611417519,-40.054352742159));
#28939=CARTESIAN_POINT('Ctrl Pts',(16.9397257481012,-50.8927896162339,-39.9490537266974));
#28940=CARTESIAN_POINT('Ctrl Pts',(19.0777499741398,-53.0547982657246,-39.7911052035049));
#28941=CARTESIAN_POINT('Ctrl Pts',(22.0523084692446,-52.4401119538419,-39.6331566803124));
#28942=CARTESIAN_POINT('Ctrl Pts',(23.1658860740626,-49.6164672289135,-39.4752081571199));
#28943=CARTESIAN_POINT('Ctrl Pts',(21.4091622878053,-47.1388520397903,-39.3172596339275));
#28944=CARTESIAN_POINT('Ctrl Pts',(18.3747378057433,-47.2562099103462,-39.159311110735));
#28945=CARTESIAN_POINT('Ctrl Pts',(16.8139173254206,-49.8608482964249,-39.0013625875425));
#28946=CARTESIAN_POINT('Ctrl Pts',(18.1418069399974,-52.5918675304547,-38.8434140643501));
#28947=CARTESIAN_POINT('Ctrl Pts',(21.1544708029442,-52.9728106959128,-38.6854655411576));
#28948=CARTESIAN_POINT('Ctrl Pts',(23.1204075266815,-50.6584513677779,-38.5275170179651));
#28949=CARTESIAN_POINT('Ctrl Pts',(22.2571674439236,-47.7470668110575,-38.3695684947727));
#28950=CARTESIAN_POINT('Ctrl Pts',(19.3474213868002,-46.878362018873,-38.2116199715802));
#28951=CARTESIAN_POINT('Ctrl Pts',(17.0293489638371,-48.8399445315482,-38.0536714483877));
#28952=CARTESIAN_POINT('Ctrl Pts',(17.4046752596388,-51.8533175278514,-37.8957229251952));
#28953=CARTESIAN_POINT('Ctrl Pts',(20.133103678538,-53.1863421439208,-37.7377744020028));
#28954=CARTESIAN_POINT('Ctrl Pts',(22.7408509828893,-51.6304081221977,-37.5798258788103));
#28955=CARTESIAN_POINT('Ctrl Pts',(22.8635520890914,-48.5962322027645,-37.4218773556178));
#28956=CARTESIAN_POINT('Ctrl Pts',(20.3899575926377,-46.8348100723855,-37.2639288324254));
#28957=CARTESIAN_POINT('Ctrl Pts',(17.5628004142346,-47.9431692734875,-37.1059803092329));
#28958=CARTESIAN_POINT('Ctrl Pts',(16.9453779725182,-50.9163943943856,-36.9480317860404));
#28959=CARTESIAN_POINT('Ctrl Pts',(19.0974884228245,-53.0587525607701,-36.790083262848));
#28960=CARTESIAN_POINT('Ctrl Pts',(22.0678786705856,-52.4278328221218,-36.6321347396554));
#28961=CARTESIAN_POINT('Ctrl Pts',(23.1633862198763,-49.5956708957895,-36.4741862164631));
#28962=CARTESIAN_POINT('Ctrl Pts',(21.3907476934156,-47.1301018746788,-36.3162376932706));
#28963=CARTESIAN_POINT('Ctrl Pts',(18.3571605311308,-47.266582198009,-36.1582891700781));
#28964=CARTESIAN_POINT('Ctrl Pts',(16.8130859505072,-49.881369310155,-36.0003406468856));
#28965=CARTESIAN_POINT('Ctrl Pts',(18.1584894129788,-52.6037152603445,-35.8423921236932));
#28966=CARTESIAN_POINT('Ctrl Pts',(21.1735345176749,-52.9653517726256,-35.6844436005007));
#28967=CARTESIAN_POINT('Ctrl Pts',(23.1245715666416,-50.6383940196509,-35.5264950773083));
#28968=CARTESIAN_POINT('Ctrl Pts',(22.2426546056792,-47.7326238249923,-35.3685465541157));
#28969=CARTESIAN_POINT('Ctrl Pts',(19.3273909210059,-46.8826146490553,-35.2105980309233));
#28970=CARTESIAN_POINT('Ctrl Pts',(17.0219614317752,-48.8590439598447,-35.0526495077308));
#28971=CARTESIAN_POINT('Ctrl Pts',(17.4166289394056,-51.8699434116262,-34.8947009845384));
#28972=CARTESIAN_POINT('Ctrl Pts',(20.1535604179975,-53.1854220438481,-34.7367524613459));
#28973=CARTESIAN_POINT('Ctrl Pts',(22.7512633359202,-51.6127753891431,-34.5788039381534));
#28974=CARTESIAN_POINT('Ctrl Pts',(22.8544794630559,-48.5778743394492,-34.420855414961));
#28975=CARTESIAN_POINT('Ctrl Pts',(20.3696258761073,-46.8323713741795,-34.2629068917684));
#28976=CARTESIAN_POINT('Ctrl Pts',(17.5496437489551,-47.9588609448717,-34.104958368576));
#28977=CARTESIAN_POINT('Ctrl Pts',(16.9513251104087,-50.9359892184104,-33.9470098453835));
#28978=CARTESIAN_POINT('Ctrl Pts',(19.1171472729993,-53.0644845344418,-33.7890613221911));
#28979=CARTESIAN_POINT('Ctrl Pts',(22.0834251524095,-52.4145049251787,-33.6311127989986));
#28980=CARTESIAN_POINT('Ctrl Pts',(23.1607248106417,-49.575367134104,-33.4731642758061));
#28981=CARTESIAN_POINT('Ctrl Pts',(21.3722914121648,-47.1212310479123,-33.3152157526137));
#28982=CARTESIAN_POINT('Ctrl Pts',(18.3396431266347,-47.2771872167786,-33.1572672294212));
#28983=CARTESIAN_POINT('Ctrl Pts',(16.8123899207133,-49.9018349255842,-32.9993187062287));
#28984=CARTESIAN_POINT('Ctrl Pts',(18.1752458269029,-52.6154859218069,-32.8413701830363));
#28985=CARTESIAN_POINT('Ctrl Pts',(21.1925508444502,-52.9577553791357,-32.6834216598438));
#28986=CARTESIAN_POINT('Ctrl Pts',(23.1286062811288,-50.6183179902657,-32.5254731366514));
#28987=CARTESIAN_POINT('Ctrl Pts',(22.2280495549668,-47.7182704849133,-32.3675246134588));
#28988=CARTESIAN_POINT('Ctrl Pts',(19.3073880603804,-46.8869977352239,-32.2095760902664));
#28989=CARTESIAN_POINT('Ctrl Pts',(17.0146967466071,-48.8781894613227,-32.0516275670739));
#28990=CARTESIAN_POINT('Ctrl Pts',(17.428689098791,-51.8864926845151,-31.8936790438815));
#28991=CARTESIAN_POINT('Ctrl Pts',(20.1740108422151,-53.184370365739,-31.735730520689));
#28992=CARTESIAN_POINT('Ctrl Pts',(22.7615622473033,-51.5950762845941,-31.5777819974966));
#28993=CARTESIAN_POINT('Ctrl Pts',(22.8452891518807,-48.55957504826,-31.419833474304));
#28994=CARTESIAN_POINT('Ctrl Pts',(20.3492789180058,-46.830063307124,-31.2618849511116));
#28995=CARTESIAN_POINT('Ctrl Pts',(17.5365881120131,-47.9746367561522,-31.1039364279191));
#28996=CARTESIAN_POINT('Ctrl Pts',(16.9573979435723,-50.9555454597386,-30.9459879047267));
#28997=CARTESIAN_POINT('Ctrl Pts',(19.1368425231359,-53.0700901565815,-30.7880393815342));
#28998=CARTESIAN_POINT('Ctrl Pts',(22.0988857352243,-52.4010774810233,-30.6300908583417));
#28999=CARTESIAN_POINT('Ctrl Pts',(23.1579330859087,-49.5550808788918,-30.4721423351492));
#29000=CARTESIAN_POINT('Ctrl Pts',(21.3537785517932,-47.1124789122659,-30.3141938119568));
#29001=CARTESIAN_POINT('Ctrl Pts',(18.3221941780797,-47.2879044959038,-30.1562452887643));
#29002=CARTESIAN_POINT('Ctrl Pts',(16.811825314945,-49.922304588451,-29.9982967655719));
#29003=CARTESIAN_POINT('Ctrl Pts',(18.1920774747975,-52.6271487476477,-29.8403482423793));
#29004=CARTESIAN_POINT('Ctrl Pts',(21.2115180027775,-52.9500370384753,-29.6823997191869));
#29005=CARTESIAN_POINT('Ctrl Pts',(23.1325120042847,-50.5982164678267,-29.5244511959944));
#29006=CARTESIAN_POINT('Ctrl Pts',(22.2133526425706,-47.7040112197537,-29.366502672802));
#29007=CARTESIAN_POINT('Ctrl Pts',(19.2874137558802,-46.8915091693428,-29.2085541496095));
#29008=CARTESIAN_POINT('Ctrl Pts',(17.0075551444725,-48.8973812147032,-29.050605626417));
#29009=CARTESIAN_POINT('Ctrl Pts',(17.4408552723353,-51.9029641778798,-28.8926571032246));
#29010=CARTESIAN_POINT('Ctrl Pts',(20.194454092182,-53.183187397366,-28.7347085800321));
#29011=CARTESIAN_POINT('Ctrl Pts',(22.7717473001459,-51.5773114152244,-28.5767600568396));
#29012=CARTESIAN_POINT('Ctrl Pts',(22.8359815310565,-48.5413351460594,-28.4188115336471));
#29013=CARTESIAN_POINT('Ctrl Pts',(20.3289175580364,-46.8278859338841,-28.2608630104547));
#29014=CARTESIAN_POINT('Ctrl Pts',(17.5236340431025,-47.9904960755269,-28.1029144872622));
#29015=CARTESIAN_POINT('Ctrl Pts',(16.9635962172961,-50.9750622981224,-27.9449659640698));
#29016=CARTESIAN_POINT('Ctrl Pts',(19.1565733705927,-53.0755692122251,-27.7870174408773));
#29017=CARTESIAN_POINT('Ctrl Pts',(22.1142597625249,-52.3875510169411,-27.6290689176848));
#29018=CARTESIAN_POINT('Ctrl Pts',(23.1550111989396,-49.534813016024,-27.4711203944923));
#29019=CARTESIAN_POINT('Ctrl Pts',(21.335209799508,-47.1038457315552,-27.3131718712999));
#29020=CARTESIAN_POINT('Ctrl Pts',(18.3048145563825,-47.29873378596,-27.1552233481074));
#29021=CARTESIAN_POINT('Ctrl Pts',(16.8113918548235,-49.9427770720226,-26.997274824915));
#29022=CARTESIAN_POINT('Ctrl Pts',(18.208984263294,-52.63870401891,-26.8393263017224));
#29023=CARTESIAN_POINT('Ctrl Pts',(21.2304340148929,-52.9421955520691,-26.68137777853));
#29024=CARTESIAN_POINT('Ctrl Pts',(23.1362909557585,-50.5780933009252,-26.5234292553375));
#29025=CARTESIAN_POINT('Ctrl Pts',(22.1985597346407,-47.6898406051712,-26.3654807321451));
#29026=CARTESIAN_POINT('Ctrl Pts',(19.2674782677023,-46.8961607354285,-26.2075322089526));
#29027=CARTESIAN_POINT('Ctrl Pts',(17.0005181319692,-48.9165945971056,-26.0495836857601));
#29028=CARTESIAN_POINT('Ctrl Pts',(17.4531643639531,-51.9194046599987,-25.8916351625677));
#29029=CARTESIAN_POINT('Ctrl Pts',(20.2148148526698,-53.1817787219156,-25.7336866393752));
#29030=CARTESIAN_POINT('Ctrl Pts',(22.7819663465347,-51.5596695965279,-25.5757381161827));
#29031=CARTESIAN_POINT('Ctrl Pts',(22.8262617594946,-48.522780826262,-25.4177895929903));
#29032=CARTESIAN_POINT('Ctrl Pts',(20.3091307149198,-46.8265862858259,-25.2598410697978));
#29033=CARTESIAN_POINT('Ctrl Pts',(17.5096074259459,-48.0049354943838,-25.1018925466053));
#29034=CARTESIAN_POINT('Ctrl Pts',(16.9723089342444,-50.9977166962789,-24.9439440234128));
#29035=CARTESIAN_POINT('Ctrl Pts',(18.438153778257,-52.3802071955689,-24.8386450079512));
#29036=CARTESIAN_POINT('Ctrl Pts',(19.301933573839,-52.6111321859386,-24.7859955002204));
#29037=CARTESIAN_POINT('Ctrl Pts',(17.8048028959809,-48.1231365609212,-40.2140044997796));
#29038=CARTESIAN_POINT('Ctrl Pts',(17.1839240578764,-48.8493222806572,-40.1613549920488));
#29039=CARTESIAN_POINT('Ctrl Pts',(16.7298826841491,-50.9540082172854,-40.0560559765871));
#29040=CARTESIAN_POINT('Ctrl Pts',(19.014511272237,-53.2642658412,-39.8981074533947));
#29041=CARTESIAN_POINT('Ctrl Pts',(22.1930353002121,-52.6074304771614,-39.7401589302022));
#29042=CARTESIAN_POINT('Ctrl Pts',(23.3829709426793,-49.5901683794686,-39.5822104070097));
#29043=CARTESIAN_POINT('Ctrl Pts',(21.5057885728173,-46.9426630694658,-39.4242618838173));
#29044=CARTESIAN_POINT('Ctrl Pts',(18.2632935460151,-47.068068171449,-39.2663133606248));
#29045=CARTESIAN_POINT('Ctrl Pts',(16.5954475755204,-49.8513066614508,-39.1083648374323));
#29046=CARTESIAN_POINT('Ctrl Pts',(18.0143906063523,-52.7695919365634,-38.9504163142399));
#29047=CARTESIAN_POINT('Ctrl Pts',(21.2336328879706,-53.176656382159,-38.7924677910474));
#29048=CARTESIAN_POINT('Ctrl Pts',(23.334373930435,-50.7036013906531,-38.6345192678549));
#29049=CARTESIAN_POINT('Ctrl Pts',(22.4119414587009,-47.5925831392253,-38.4765707446625));
#29050=CARTESIAN_POINT('Ctrl Pts',(19.3026740588186,-46.6643112428346,-38.31862222147));
#29051=CARTESIAN_POINT('Ctrl Pts',(16.8256513655012,-48.7603995059013,-38.1606736982775));
#29052=CARTESIAN_POINT('Ctrl Pts',(17.2267137925807,-51.9803995461637,-38.002725175085));
#29053=CARTESIAN_POINT('Ctrl Pts',(20.1422306003197,-53.4048296856387,-37.8447766518926));
#29054=CARTESIAN_POINT('Ctrl Pts',(22.9287911871795,-51.7422052383032,-37.6868281287001));
#29055=CARTESIAN_POINT('Ctrl Pts',(23.0599059105793,-48.499975818074,-37.5288796055077));
#29056=CARTESIAN_POINT('Ctrl Pts',(20.4166969922192,-46.6177729385439,-37.3709310823152));
#29057=CARTESIAN_POINT('Ctrl Pts',(17.3956815920498,-47.8021323512527,-37.2129825591227));
#29058=CARTESIAN_POINT('Ctrl Pts',(16.7359224817024,-50.9792315755262,-37.0550340359303));
#29059=CARTESIAN_POINT('Ctrl Pts',(19.0356031867254,-53.2684912823324,-36.8970855127378));
#29060=CARTESIAN_POINT('Ctrl Pts',(22.2096731505566,-52.5943093651446,-36.7391369895453));
#29061=CARTESIAN_POINT('Ctrl Pts',(23.3802996734437,-49.5679460413847,-36.5811884663528));
#29062=CARTESIAN_POINT('Ctrl Pts',(21.4861112893383,-46.9333129053653,-36.4232399431604));
#29063=CARTESIAN_POINT('Ctrl Pts',(18.2445109973463,-47.0791516870751,-36.2652914199679));
#29064=CARTESIAN_POINT('Ctrl Pts',(16.5945591932132,-49.8732348014845,-36.1073428967754));
#29065=CARTESIAN_POINT('Ctrl Pts',(18.0322169968249,-52.7822520655183,-35.949394373583));
#29066=CARTESIAN_POINT('Ctrl Pts',(21.2540038019849,-53.1686860003594,-35.7914458503905));
#29067=CARTESIAN_POINT('Ctrl Pts',(23.3388234986948,-50.6821687097818,-35.633497327198));
#29068=CARTESIAN_POINT('Ctrl Pts',(22.3964334748606,-47.5771497973294,-35.4755488040056));
#29069=CARTESIAN_POINT('Ctrl Pts',(19.2812701036018,-46.6688554759499,-35.3176002808131));
#29070=CARTESIAN_POINT('Ctrl Pts',(16.8177572702246,-48.780808582361,-35.1596517576206));
#29071=CARTESIAN_POINT('Ctrl Pts',(17.2394871363976,-51.9981654671068,-35.0017032344282));
#29072=CARTESIAN_POINT('Ctrl Pts',(20.1640900587951,-53.4038464942864,-34.8437547112357));
#29073=CARTESIAN_POINT('Ctrl Pts',(22.9399175154567,-51.723363428406,-34.6858061880432));
#29074=CARTESIAN_POINT('Ctrl Pts',(23.0502111744031,-48.4803591557203,-34.5278576648508));
#29075=CARTESIAN_POINT('Ctrl Pts',(20.3949711294977,-46.6151670187554,-34.3699091416583));
#29076=CARTESIAN_POINT('Ctrl Pts',(17.3816227739805,-47.8189000008437,-34.2119606184658));
#29077=CARTESIAN_POINT('Ctrl Pts',(16.7422774149517,-51.000170017009,-34.0540120952733));
#29078=CARTESIAN_POINT('Ctrl Pts',(19.0566100446325,-53.2746162975484,-33.8960635720809));
#29079=CARTESIAN_POINT('Ctrl Pts',(22.2262856549365,-52.5800675740533,-33.7381150488884));
#29080=CARTESIAN_POINT('Ctrl Pts',(23.377455771327,-49.5462500503724,-33.5801665256959));
#29081=CARTESIAN_POINT('Ctrl Pts',(21.4663894605293,-46.9238338058378,-33.4222180025035));
#29082=CARTESIAN_POINT('Ctrl Pts',(18.2257924240891,-47.0904838921846,-33.264269479311));
#29083=CARTESIAN_POINT('Ctrl Pts',(16.5938154366431,-49.8951037445551,-33.1063209561186));
#29084=CARTESIAN_POINT('Ctrl Pts',(18.0501223983721,-52.7948298414622,-32.9483724329261));
#29085=CARTESIAN_POINT('Ctrl Pts',(21.2743240786507,-53.1605687220227,-32.7904239097336));
#29086=CARTESIAN_POINT('Ctrl Pts',(23.3431348736315,-50.6607160666778,-32.6324753865412));
#29087=CARTESIAN_POINT('Ctrl Pts',(22.3808269555417,-47.5618122484469,-32.4745268633486));
#29088=CARTESIAN_POINT('Ctrl Pts',(19.2598956464409,-46.6735391104208,-32.3165783401562));
#29089=CARTESIAN_POINT('Ctrl Pts',(16.8099944454557,-48.8012668912414,-32.1586298169637));
#29090=CARTESIAN_POINT('Ctrl Pts',(17.2523742611426,-52.015849523954,-32.0006812937713));
#29091=CARTESIAN_POINT('Ctrl Pts',(20.1859427689921,-53.4027227025893,-31.8427327705787));
#29092=CARTESIAN_POINT('Ctrl Pts',(22.9509226233902,-51.7044506959199,-31.6847842473864));
#29093=CARTESIAN_POINT('Ctrl Pts',(23.040390683415,-48.4608050817844,-31.5268357241939));
#29094=CARTESIAN_POINT('Ctrl Pts',(20.3732289800902,-46.6127006874977,-31.3688872010014));
#29095=CARTESIAN_POINT('Ctrl Pts',(17.3676719117639,-47.8357575598052,-31.2109386778089));
#29096=CARTESIAN_POINT('Ctrl Pts',(16.7487666624015,-51.0210672301788,-31.0529901546165));
#29097=CARTESIAN_POINT('Ctrl Pts',(19.0776557984475,-53.2806062973054,-30.895041631424));
#29098=CARTESIAN_POINT('Ctrl Pts',(22.2428063702104,-52.5657194097955,-30.7370931082315));
#29099=CARTESIAN_POINT('Ctrl Pts',(23.3744726179757,-49.5245727662524,-30.579144585039));
#29100=CARTESIAN_POINT('Ctrl Pts',(21.4466071729682,-46.9144815360828,-30.4211960618466));
#29101=CARTESIAN_POINT('Ctrl Pts',(18.2071470007981,-47.1019360553443,-30.2632475386541));
#29102=CARTESIAN_POINT('Ctrl Pts',(16.5932121158465,-49.9169770125958,-30.1052990154617));
#29103=CARTESIAN_POINT('Ctrl Pts',(18.0681081926846,-52.8072923874939,-29.9473504922691));
#29104=CARTESIAN_POINT('Ctrl Pts',(21.2945918153871,-53.1523211345956,-29.7894019690767));
#29105=CARTESIAN_POINT('Ctrl Pts',(23.3473084122988,-50.639236182461,-29.6314534458842));
#29106=CARTESIAN_POINT('Ctrl Pts',(22.3651222755816,-47.5465752252027,-29.4735049226918));
#29107=CARTESIAN_POINT('Ctrl Pts',(19.2385517034993,-46.6783598936636,-29.3155563994993));
#29108=CARTESIAN_POINT('Ctrl Pts',(16.8023631435262,-48.821774623518,-29.1576078763068));
#29109=CARTESIAN_POINT('Ctrl Pts',(17.2653746694394,-52.0334504679336,-28.9996593531144));
#29110=CARTESIAN_POINT('Ctrl Pts',(20.2077878130001,-53.4014586180524,-28.8417108299219));
#29111=CARTESIAN_POINT('Ctrl Pts',(22.9618060655009,-51.6854676891177,-28.6837623067294));
#29112=CARTESIAN_POINT('Ctrl Pts',(23.030444838853,-48.4413144691413,-28.5258137835369));
#29113=CARTESIAN_POINT('Ctrl Pts',(20.3514714412784,-46.6103740117332,-28.3678652603445));
#29114=CARTESIAN_POINT('Ctrl Pts',(17.3538295821005,-47.8527043530126,-28.209916737152));
#29115=CARTESIAN_POINT('Ctrl Pts',(16.755389951873,-51.0419223385436,-28.0519682139596));
#29116=CARTESIAN_POINT('Ctrl Pts',(19.0987395904915,-53.2864610518992,-27.8940196907671));
#29117=CARTESIAN_POINT('Ctrl Pts',(22.259234594857,-52.5512654358125,-27.7360711675746));
#29118=CARTESIAN_POINT('Ctrl Pts',(23.3713503771613,-49.5029151356404,-27.5781226443821));
#29119=CARTESIAN_POINT('Ctrl Pts',(21.4267651609838,-46.9052563780058,-27.4201741211897));
#29120=CARTESIAN_POINT('Ctrl Pts',(18.1885756581089,-47.1135079100266,-27.2622255979972));
#29121=CARTESIAN_POINT('Ctrl Pts',(16.5927489333562,-49.9388532947573,-27.1042770748048));
#29122=CARTESIAN_POINT('Ctrl Pts',(18.0861742799915,-52.8196400039275,-26.9463285516122));
#29123=CARTESIAN_POINT('Ctrl Pts',(21.3148048988148,-53.1439419573167,-26.7883800284198));
#29124=CARTESIAN_POINT('Ctrl Pts',(23.3513464865473,-50.6177331696203,-26.6304315052273));
#29125=CARTESIAN_POINT('Ctrl Pts',(22.3493150176721,-47.5314329313073,-26.4724829820349));
#29126=CARTESIAN_POINT('Ctrl Pts',(19.2172492385159,-46.6833304177247,-26.3145344588424));
#29127=CARTESIAN_POINT('Ctrl Pts',(16.794843602941,-48.8423054679189,-26.1565859356499));
#29128=CARTESIAN_POINT('Ctrl Pts',(17.2785277957047,-52.0510182742257,-25.9986374124575));
#29129=CARTESIAN_POINT('Ctrl Pts',(20.2295447112238,-53.3999533496994,-25.840688889265));
#29130=CARTESIAN_POINT('Ctrl Pts',(22.9727258320959,-51.6666161705761,-25.6827403660725));
#29131=CARTESIAN_POINT('Ctrl Pts',(23.0200585823692,-48.4214878792807,-25.52479184288));
#29132=CARTESIAN_POINT('Ctrl Pts',(20.3303278139511,-46.6089852467828,-25.3668433196876));
#29133=CARTESIAN_POINT('Ctrl Pts',(17.3388411595373,-47.8681338830967,-25.2088947964951));
#29134=CARTESIAN_POINT('Ctrl Pts',(16.764700099989,-51.0661301492147,-25.0509462733027));
#29135=CARTESIAN_POINT('Ctrl Pts',(18.3310579529763,-52.5434180484685,-24.945647257841));
#29136=CARTESIAN_POINT('Ctrl Pts',(19.2540671456531,-52.7901775698422,-24.8929977501102));
#29137=CARTESIAN_POINT('Ctrl Pts',(17.6639373423039,-48.0026984430693,-40.3210067496694));
#29138=CARTESIAN_POINT('Ctrl Pts',(17.003216778308,-48.7754834195626,-40.2683572419386));
#29139=CARTESIAN_POINT('Ctrl Pts',(16.520039620197,-51.0152268183369,-40.163058226477));
#29140=CARTESIAN_POINT('Ctrl Pts',(18.9512725703343,-53.4737334166756,-40.0051097032844));
#29141=CARTESIAN_POINT('Ctrl Pts',(22.3337621311796,-52.7747490004808,-39.8471611800921));
#29142=CARTESIAN_POINT('Ctrl Pts',(23.600055811296,-49.5638695300238,-39.6892126568995));
#29143=CARTESIAN_POINT('Ctrl Pts',(21.6024148578293,-46.7464740991412,-39.5312641337071));
#29144=CARTESIAN_POINT('Ctrl Pts',(18.1518492862868,-46.8799264325519,-39.3733156105146));
#29145=CARTESIAN_POINT('Ctrl Pts',(16.3769778256201,-49.8417650264767,-39.2153670873222));
#29146=CARTESIAN_POINT('Ctrl Pts',(17.8869742727072,-52.9473163426722,-39.0574185641297));
#29147=CARTESIAN_POINT('Ctrl Pts',(21.3127949729971,-53.3805020684052,-38.8994700409372));
#29148=CARTESIAN_POINT('Ctrl Pts',(23.5483403341885,-50.7487514135285,-38.7415215177447));
#29149=CARTESIAN_POINT('Ctrl Pts',(22.5667154734781,-47.438099467393,-38.5835729945523));
#29150=CARTESIAN_POINT('Ctrl Pts',(19.257926730837,-46.4502604667964,-38.4256244713598));
#29151=CARTESIAN_POINT('Ctrl Pts',(16.6219537671653,-48.6808544802542,-38.2676759481673));
#29152=CARTESIAN_POINT('Ctrl Pts',(17.0487523255225,-52.107481564476,-38.1097274249749));
#29153=CARTESIAN_POINT('Ctrl Pts',(20.1513575221015,-53.6233172273567,-37.9517789017824));
#29154=CARTESIAN_POINT('Ctrl Pts',(23.1167313914696,-51.8540023544087,-37.7938303785899));
#29155=CARTESIAN_POINT('Ctrl Pts',(23.2562597320672,-48.4037194333835,-37.6358818553975));
#29156=CARTESIAN_POINT('Ctrl Pts',(20.4434363918007,-46.4007358047025,-37.477933332205));
#29157=CARTESIAN_POINT('Ctrl Pts',(17.228562769865,-47.6610954290179,-37.3199848090125));
#29158=CARTESIAN_POINT('Ctrl Pts',(16.5264669908866,-51.0420687566668,-37.1620362858201));
#29159=CARTESIAN_POINT('Ctrl Pts',(18.9737179506262,-53.4782300038948,-37.0040877626276));
#29160=CARTESIAN_POINT('Ctrl Pts',(22.3514676305278,-52.7607859081673,-36.8461392394351));
#29161=CARTESIAN_POINT('Ctrl Pts',(23.5972131270111,-49.5402211869799,-36.6881907162427));
#29162=CARTESIAN_POINT('Ctrl Pts',(21.581474885261,-46.7365239360518,-36.5302421930502));
#29163=CARTESIAN_POINT('Ctrl Pts',(18.1318614635619,-46.8917211761413,-36.3722936698578));
#29164=CARTESIAN_POINT('Ctrl Pts',(16.3760324359193,-49.8651002928142,-36.2143451466652));
#29165=CARTESIAN_POINT('Ctrl Pts',(17.905944580671,-52.960788870692,-36.0563966234728));
#29166=CARTESIAN_POINT('Ctrl Pts',(21.3344730862948,-53.3720202280932,-35.8984481002803));
#29167=CARTESIAN_POINT('Ctrl Pts',(23.5530754307479,-50.7259433999127,-35.7404995770879));
#29168=CARTESIAN_POINT('Ctrl Pts',(22.550212344042,-47.4216757696665,-35.5825510538954));
#29169=CARTESIAN_POINT('Ctrl Pts',(19.2351492861978,-46.4550963028444,-35.4246025307029));
#29170=CARTESIAN_POINT('Ctrl Pts',(16.613553108674,-48.7025732048773,-35.2666540075104));
#29171=CARTESIAN_POINT('Ctrl Pts',(17.0623453333896,-52.1263875225874,-35.108705484318));
#29172=CARTESIAN_POINT('Ctrl Pts',(20.1746196995926,-53.6222709447248,-34.9507569611255));
#29173=CARTESIAN_POINT('Ctrl Pts',(23.1285716949932,-51.833951467669,-34.792808437933));
#29174=CARTESIAN_POINT('Ctrl Pts',(23.2459428857504,-48.3828439719913,-34.6348599147406));
#29175=CARTESIAN_POINT('Ctrl Pts',(20.420316382888,-46.3979626633313,-34.4769113915481));
#29176=CARTESIAN_POINT('Ctrl Pts',(17.213601799006,-47.6789390568155,-34.3189628683557));
#29177=CARTESIAN_POINT('Ctrl Pts',(16.5332297194947,-51.0643508156075,-34.1610143451632));
#29178=CARTESIAN_POINT('Ctrl Pts',(18.9960728162657,-53.4847480606549,-34.0030658219707));
#29179=CARTESIAN_POINT('Ctrl Pts',(22.3691461574634,-52.7456302229279,-33.8451172987783));
#29180=CARTESIAN_POINT('Ctrl Pts',(23.5941867320123,-49.5171329666407,-33.6871687755858));
#29181=CARTESIAN_POINT('Ctrl Pts',(21.5604875088938,-46.7264365637634,-33.5292202523933));
#29182=CARTESIAN_POINT('Ctrl Pts',(18.1119417215434,-46.9037805675905,-33.3712717292008));
#29183=CARTESIAN_POINT('Ctrl Pts',(16.3752409525729,-49.8883725635259,-33.2133232060083));
#29184=CARTESIAN_POINT('Ctrl Pts',(17.9249989698413,-52.9741737611174,-33.0553746828159));
#29185=CARTESIAN_POINT('Ctrl Pts',(21.3560973128511,-53.3633820649098,-32.8974261596234));
#29186=CARTESIAN_POINT('Ctrl Pts',(23.5576634661342,-50.7031141430899,-32.7394776364309));
#29187=CARTESIAN_POINT('Ctrl Pts',(22.5336043561166,-47.4053540119805,-32.5815291132385));
#29188=CARTESIAN_POINT('Ctrl Pts',(19.2124032325014,-46.4600804856177,-32.4235805900461));
#29189=CARTESIAN_POINT('Ctrl Pts',(16.6052921443043,-48.7243443211601,-32.2656320668535));
#29190=CARTESIAN_POINT('Ctrl Pts',(17.0760594234942,-52.145206363393,-32.1076835436611));
#29191=CARTESIAN_POINT('Ctrl Pts',(20.1978746957691,-53.6210750394396,-31.9497350204685));
#29192=CARTESIAN_POINT('Ctrl Pts',(23.1402829994771,-51.8138251072455,-31.7917864972762));
#29193=CARTESIAN_POINT('Ctrl Pts',(23.2354922149493,-48.3620351153088,-31.6338379740836));
#29194=CARTESIAN_POINT('Ctrl Pts',(20.3971790421746,-46.3953380678715,-31.4758894508912));
#29195=CARTESIAN_POINT('Ctrl Pts',(17.1987557115146,-47.6968783634582,-31.3179409276987));
#29196=CARTESIAN_POINT('Ctrl Pts',(16.5401353812306,-51.0865890006191,-31.1599924045063));
#29197=CARTESIAN_POINT('Ctrl Pts',(19.018469073759,-53.4911224380292,-31.0020438813138));
#29198=CARTESIAN_POINT('Ctrl Pts',(22.3867270051965,-52.7303613385677,-30.8440953581213));
#29199=CARTESIAN_POINT('Ctrl Pts',(23.5910121500427,-49.494064653613,-30.6861468349289));
#29200=CARTESIAN_POINT('Ctrl Pts',(21.5394357941431,-46.7164841598999,-30.5281983117364));
#29201=CARTESIAN_POINT('Ctrl Pts',(18.0920998235166,-46.9159676147846,-30.3702497885439));
#29202=CARTESIAN_POINT('Ctrl Pts',(16.3745989167479,-49.9116494367408,-30.2123012653515));
#29203=CARTESIAN_POINT('Ctrl Pts',(17.9441389105717,-52.98743602734,-30.054352742159));
#29204=CARTESIAN_POINT('Ctrl Pts',(21.3776656279966,-53.354605230716,-29.8964042189665));
#29205=CARTESIAN_POINT('Ctrl Pts',(23.5621048203129,-50.6802558970953,-29.738455695774));
#29206=CARTESIAN_POINT('Ctrl Pts',(22.5168919085926,-47.3891392306516,-29.5805071725816));
#29207=CARTESIAN_POINT('Ctrl Pts',(19.1896896511183,-46.4652106179844,-29.4225586493891));
#29208=CARTESIAN_POINT('Ctrl Pts',(16.5971711425799,-48.7461680323328,-29.2646101261967));
#29209=CARTESIAN_POINT('Ctrl Pts',(17.0898940665435,-52.1639367579875,-29.1066616030041));
#29210=CARTESIAN_POINT('Ctrl Pts',(20.2211215338182,-53.6197298387387,-28.9487130798117));
#29211=CARTESIAN_POINT('Ctrl Pts',(23.1518648308559,-51.7936239630112,-28.7907645566192));
#29212=CARTESIAN_POINT('Ctrl Pts',(23.2249081466494,-48.341293792223,-28.6328160334268));
#29213=CARTESIAN_POINT('Ctrl Pts',(20.3740253245205,-46.3928620895824,-28.4748675102343));
#29214=CARTESIAN_POINT('Ctrl Pts',(17.1840251210985,-47.7149126304983,-28.3169189870418));
#29215=CARTESIAN_POINT('Ctrl Pts',(16.5471836864498,-51.1087823789649,-28.1589704638494));
#29216=CARTESIAN_POINT('Ctrl Pts',(19.0409058103903,-53.4973528915733,-28.0010219406569));
#29217=CARTESIAN_POINT('Ctrl Pts',(22.4042094271889,-52.714979854684,-27.8430734174644));
#29218=CARTESIAN_POINT('Ctrl Pts',(23.587689555383,-49.4710172552568,-27.685124894272));
#29219=CARTESIAN_POINT('Ctrl Pts',(21.5183205224596,-46.7066670244563,-27.5271763710795));
#29220=CARTESIAN_POINT('Ctrl Pts',(18.0723367598354,-46.9282820340933,-27.369227847887));
#29221=CARTESIAN_POINT('Ctrl Pts',(16.3741060118888,-49.934929517492,-27.2112793246946));
#29222=CARTESIAN_POINT('Ctrl Pts',(17.963364296689,-53.000575988945,-27.053330801502));
#29223=CARTESIAN_POINT('Ctrl Pts',(21.3991757827366,-53.3456883625643,-26.8953822783096));
#29224=CARTESIAN_POINT('Ctrl Pts',(23.5664020173362,-50.6573730383154,-26.7374337551172));
#29225=CARTESIAN_POINT('Ctrl Pts',(22.5000703007035,-47.3730252574435,-26.5794852319247));
#29226=CARTESIAN_POINT('Ctrl Pts',(19.1670202093295,-46.4705001000209,-26.4215367087323));
#29227=CARTESIAN_POINT('Ctrl Pts',(16.5891690739128,-48.7680163387323,-26.2635881855397));
#29228=CARTESIAN_POINT('Ctrl Pts',(17.1038912274563,-52.1826318884526,-26.1056396623473));
#29229=CARTESIAN_POINT('Ctrl Pts',(20.2442745697777,-53.6181279774832,-25.9476911391548));
#29230=CARTESIAN_POINT('Ctrl Pts',(23.1634853176571,-51.7735627446242,-25.7897426159623));
#29231=CARTESIAN_POINT('Ctrl Pts',(23.2138554052439,-48.3201949322993,-25.6317940927699));
#29232=CARTESIAN_POINT('Ctrl Pts',(20.3515249129824,-46.3913842077397,-25.4738455695774));
#29233=CARTESIAN_POINT('Ctrl Pts',(17.1680748931287,-47.7313322718094,-25.315897046385));
#29234=CARTESIAN_POINT('Ctrl Pts',(16.5570912657335,-51.1345436021507,-25.1579485231925));
#29235=CARTESIAN_POINT('Ctrl Pts',(18.2239621276955,-52.7066289013681,-25.0526495077308));
#29236=CARTESIAN_POINT('Ctrl Pts',(19.2062007174672,-52.9692229537457,-25.));
#29237=CARTESIAN_POINT('Ctrl Pts',(22.5181182812424,-50.0021988905331,-38.387416697508));
#29238=CARTESIAN_POINT('Ctrl Pts',(22.5197006098244,-50.176561944423,-38.3984493876971));
#29239=CARTESIAN_POINT('Ctrl Pts',(22.5031153273103,-50.3506259111307,-38.4094820778862));
#29240=CARTESIAN_POINT('Ctrl Pts',(22.4672444397961,-50.5206201453611,-38.4205147680753));
#29241=CARTESIAN_POINT('Ctrl Pts',(22.2960636545913,-51.3318558998239,-38.4731642758061));
#29242=CARTESIAN_POINT('Ctrl Pts',(21.6856861862545,-52.0504104547452,-38.525813783537));
#29243=CARTESIAN_POINT('Ctrl Pts',(20.9128165447069,-52.3505507513191,-38.5784632912678));
#29244=CARTESIAN_POINT('Ctrl Pts',(20.1399469031593,-52.650691047893,-38.6311127989986));
#29245=CARTESIAN_POINT('Ctrl Pts',(19.2045850884009,-52.5324170861195,-38.6837623067294));
#29246=CARTESIAN_POINT('Ctrl Pts',(18.5307648146348,-52.0493212397415,-38.7364118144603));
#29247=CARTESIAN_POINT('Ctrl Pts',(17.8569445408687,-51.5662253933636,-38.7890613221911));
#29248=CARTESIAN_POINT('Ctrl Pts',(17.4446658080948,-50.7183076623813,-38.8417108299219));
#29249=CARTESIAN_POINT('Ctrl Pts',(17.4808256067329,-49.8900090831976,-38.8943603376527));
#29250=CARTESIAN_POINT('Ctrl Pts',(17.5169854053711,-49.0617105040138,-38.9470098453835));
#29251=CARTESIAN_POINT('Ctrl Pts',(18.0015837354214,-48.2530310766285,-38.9996593531144));
#29252=CARTESIAN_POINT('Ctrl Pts',(18.7149418900001,-47.8304729230812,-39.0523088608452));
#29253=CARTESIAN_POINT('Ctrl Pts',(19.4283000445789,-47.4079147695338,-39.104958368576));
#29254=CARTESIAN_POINT('Ctrl Pts',(20.3704180236861,-47.3714778898244,-39.1576078763068));
#29255=CARTESIAN_POINT('Ctrl Pts',(21.1141878803485,-47.7378802946769,-39.2102573840377));
#29256=CARTESIAN_POINT('Ctrl Pts',(21.8579577370108,-48.1042826995294,-39.2629068917685));
#29257=CARTESIAN_POINT('Ctrl Pts',(22.4033794712283,-48.8735243889439,-39.3155563994993));
#29258=CARTESIAN_POINT('Ctrl Pts',(22.5032204104756,-49.6964831256785,-39.3682059072301));
#29259=CARTESIAN_POINT('Ctrl Pts',(22.5153637550683,-49.7965770510867,-39.3746095039894));
#29260=CARTESIAN_POINT('Ctrl Pts',(22.5209155764383,-49.8974656183845,-39.3810131007487));
#29261=CARTESIAN_POINT('Ctrl Pts',(22.5201577888434,-49.9984351914864,-39.387416697508));
#29262=CARTESIAN_POINT('Ctrl Pts',(20.7937992825328,-52.9692229537457,-40.));
#29263=CARTESIAN_POINT('Ctrl Pts',(21.7760378723045,-52.7066289013681,-39.9473504922692));
#29264=CARTESIAN_POINT('Ctrl Pts',(23.4429086391268,-51.1345429997358,-39.8420514768075));
#29265=CARTESIAN_POINT('Ctrl Pts',(22.831925189682,-47.7313325290799,-39.6841029536151));
#29266=CARTESIAN_POINT('Ctrl Pts',(19.6484750771286,-46.3913839963408,-39.5261544304226));
#29267=CARTESIAN_POINT('Ctrl Pts',(16.7861445447059,-48.3201950030769,-39.3682059072301));
#29268=CARTESIAN_POINT('Ctrl Pts',(16.8365146481096,-51.7735627154933,-39.2102573840377));
#29269=CARTESIAN_POINT('Ctrl Pts',(19.7557254203512,-53.6181280557829,-39.0523088608451));
#29270=CARTESIAN_POINT('Ctrl Pts',(22.8961088159911,-52.1826319013229,-38.8943603376528));
#29271=CARTESIAN_POINT('Ctrl Pts',(23.4108309690293,-48.7680163312232,-38.7364118144603));
#29272=CARTESIAN_POINT('Ctrl Pts',(20.8329798036235,-46.4705000476597,-38.5784632912678));
#29273=CARTESIAN_POINT('Ctrl Pts',(17.4999296646635,-47.373025224819,-38.4205147680753));
#29274=CARTESIAN_POINT('Ctrl Pts',(16.4335979353407,-50.6573730457065,-38.2625662448828));
#29275=CARTESIAN_POINT('Ctrl Pts',(18.600824198122,-53.3456884082951,-38.1046177216904));
#29276=CARTESIAN_POINT('Ctrl Pts',(22.0366357308683,-53.0005760288509,-37.9466691984979));
#29277=CARTESIAN_POINT('Ctrl Pts',(23.6258940367278,-49.9349295168378,-37.7887206753055));
#29278=CARTESIAN_POINT('Ctrl Pts',(21.9276632661251,-46.9282819927009,-37.630772152113));
#29279=CARTESIAN_POINT('Ctrl Pts',(18.4816794571067,-46.7066669802649,-37.4728236289205));
#29280=CARTESIAN_POINT('Ctrl Pts',(16.4123103964255,-49.471017248116,-37.314875105728));
#29281=CARTESIAN_POINT('Ctrl Pts',(17.5957905404958,-52.7149798911831,-37.1569265825356));
#29282=CARTESIAN_POINT('Ctrl Pts',(20.9590942025022,-53.497352938559,-36.9989780593431));
#29283=CARTESIAN_POINT('Ctrl Pts',(23.4528163599439,-51.1087823938688,-36.8410295361506));
#29284=CARTESIAN_POINT('Ctrl Pts',(22.815974916742,-47.7149125997905,-36.6830810129582));
#29285=CARTESIAN_POINT('Ctrl Pts',(19.625974670453,-46.3928620411136,-36.5251324897657));
#29286=CARTESIAN_POINT('Ctrl Pts',(16.775091810017,-48.3412937699339,-36.3671839665732));
#29287=CARTESIAN_POINT('Ctrl Pts',(16.8481351267915,-51.7936239871129,-36.2092354433808));
#29288=CARTESIAN_POINT('Ctrl Pts',(19.7788784632106,-53.6197298873777,-36.0512869201883));
#29289=CARTESIAN_POINT('Ctrl Pts',(22.9101059725603,-52.163936787065,-35.8933383969958));
#29290=CARTESIAN_POINT('Ctrl Pts',(23.4028289031449,-48.7461680154847,-35.7353898738033));
#29291=CARTESIAN_POINT('Ctrl Pts',(20.81031035977,-46.4652105704865,-35.5774413506109));
#29292=CARTESIAN_POINT('Ctrl Pts',(17.4831080575873,-47.3891391955688,-35.4194928274184));
#29293=CARTESIAN_POINT('Ctrl Pts',(16.4378951318222,-50.6802559062359,-35.261544304226));
#29294=CARTESIAN_POINT('Ctrl Pts',(18.6223343534913,-53.3546052757928,-35.1035957810335));
#29295=CARTESIAN_POINT('Ctrl Pts',(22.0558611170534,-52.9874360674829,-34.945647257841));
#29296=CARTESIAN_POINT('Ctrl Pts',(23.6254011319675,-49.9116494355537,-34.7876987346486));
#29297=CARTESIAN_POINT('Ctrl Pts',(21.9079002021205,-46.9159675733437,-34.6297502114561));
#29298=CARTESIAN_POINT('Ctrl Pts',(18.4605641851711,-46.7164841157783,-34.4718016882636));
#29299=CARTESIAN_POINT('Ctrl Pts',(16.4089878017039,-49.4940646468145,-34.3138531650711));
#29300=CARTESIAN_POINT('Ctrl Pts',(17.6132729627324,-52.7303613752562,-34.1559046418787));
#29301=CARTESIAN_POINT('Ctrl Pts',(20.98153093943,-53.4911224849404,-33.9979561186862));
#29302=CARTESIAN_POINT('Ctrl Pts',(23.4598646652605,-51.08658901522,-33.8400075954937));
#29303=CARTESIAN_POINT('Ctrl Pts',(22.8012443261265,-47.6968783325106,-33.6820590723013));
#29304=CARTESIAN_POINT('Ctrl Pts',(19.6028209524885,-46.3953380194348,-33.5241105491088));
#29305=CARTESIAN_POINT('Ctrl Pts',(16.7645077415746,-48.362035093299,-33.3661620259164));
#29306=CARTESIAN_POINT('Ctrl Pts',(16.8597169583261,-51.8138251316183,-33.2082135027239));
#29307=CARTESIAN_POINT('Ctrl Pts',(19.8021253015719,-53.621075088097,-33.0502649795314));
#29308=CARTESIAN_POINT('Ctrl Pts',(22.9239406157955,-52.1452063922187,-32.8923164563389));
#29309=CARTESIAN_POINT('Ctrl Pts',(23.3947079013113,-48.7243443040189,-32.7343679331465));
#29310=CARTESIAN_POINT('Ctrl Pts',(20.7875967780819,-46.4600804380509,-32.576419409954));
#29311=CARTESIAN_POINT('Ctrl Pts',(17.4663956098388,-47.4053539771154,-32.4184708867615));
#29312=CARTESIAN_POINT('Ctrl Pts',(16.4423364860605,-50.7031141525378,-32.2605223635691));
#29313=CARTESIAN_POINT('Ctrl Pts',(18.6439026689266,-53.3633821101044,-32.1025738403766));
#29314=CARTESIAN_POINT('Ctrl Pts',(22.0750010580409,-52.9741738010823,-31.9446253171841));
#29315=CARTESIAN_POINT('Ctrl Pts',(23.624759096134,-49.888372562026,-31.7866767939916));
#29316=CARTESIAN_POINT('Ctrl Pts',(21.888058303827,-46.9037805259858,-31.6287282707992));
#29317=CARTESIAN_POINT('Ctrl Pts',(18.4395124701376,-46.7264365197756,-31.4707797476067));
#29318=CARTESIAN_POINT('Ctrl Pts',(16.4058132196916,-49.5171329601522,-31.3128312244143));
#29319=CARTESIAN_POINT('Ctrl Pts',(17.6308538107017,-52.7456302598216,-31.1548827012217));
#29320=CARTESIAN_POINT('Ctrl Pts',(21.0039271972243,-53.4847481074805,-30.9969341780293));
#29321=CARTESIAN_POINT('Ctrl Pts',(23.4667703270891,-51.0643508299095,-30.8389856548368));
#29322=CARTESIAN_POINT('Ctrl Pts',(22.7863982384356,-47.6789390256271,-30.6810371316444));
#29323=CARTESIAN_POINT('Ctrl Pts',(19.5796836114642,-46.3979626149297,-30.5230886084519));
#29324=CARTESIAN_POINT('Ctrl Pts',(16.7540570706331,-48.3828439502611,-30.3651400852594));
#29325=CARTESIAN_POINT('Ctrl Pts',(16.8714282629673,-51.8339514923121,-30.207191562067));
#29326=CARTESIAN_POINT('Ctrl Pts',(19.8253802980609,-53.6222709933982,-30.0492430388745));
#29327=CARTESIAN_POINT('Ctrl Pts',(22.9376547060844,-52.1263875511603,-29.891294515682));
#29328=CARTESIAN_POINT('Ctrl Pts',(23.3864469368306,-48.7025731874435,-29.7333459924896));
#29329=CARTESIAN_POINT('Ctrl Pts',(20.7648507240798,-46.4550962552107,-29.5753974692971));
#29330=CARTESIAN_POINT('Ctrl Pts',(17.4497876216902,-47.4216757350208,-29.4174489461046));
#29331=CARTESIAN_POINT('Ctrl Pts',(16.4469245215085,-50.7259434096673,-29.2595004229122));
#29332=CARTESIAN_POINT('Ctrl Pts',(18.6655268957734,-53.3720202734039,-29.1015518997197));
#29333=CARTESIAN_POINT('Ctrl Pts',(22.0940554474673,-52.960788910477,-28.9436033765272));
#29334=CARTESIAN_POINT('Ctrl Pts',(23.6239676127769,-49.8651002910015,-28.7856548533348));
#29335=CARTESIAN_POINT('Ctrl Pts',(21.8681385615409,-46.8917211343748,-28.6277063301423));
#29336=CARTESIAN_POINT('Ctrl Pts',(18.4185250934885,-46.7365238921992,-28.4697578069498));
#29337=CARTESIAN_POINT('Ctrl Pts',(16.4027868246521,-49.5402211808024,-28.3118092837573));
#29338=CARTESIAN_POINT('Ctrl Pts',(17.648532337875,-52.7607859452632,-28.1538607605649));
#29339=CARTESIAN_POINT('Ctrl Pts',(21.0262820631638,-53.4782300506355,-27.9959122373724));
#29340=CARTESIAN_POINT('Ctrl Pts',(23.4735330557886,-51.042068770664,-27.8379637141799));
#29341=CARTESIAN_POINT('Ctrl Pts',(22.7714372673746,-47.6610953975998,-27.6800151909874));
#29342=CARTESIAN_POINT('Ctrl Pts',(19.556563602243,-46.4007357563187,-27.522066667795));
#29343=CARTESIAN_POINT('Ctrl Pts',(16.7437402241732,-48.4037194119704,-27.3641181446025));
#29344=CARTESIAN_POINT('Ctrl Pts',(16.883268566659,-51.8540023792524,-27.2061696214101));
#29345=CARTESIAN_POINT('Ctrl Pts',(19.8486424758461,-53.6233172761733,-27.0482210982176));
#29346=CARTESIAN_POINT('Ctrl Pts',(22.9512477141718,-52.1074815925537,-26.8902725750252));
#29347=CARTESIAN_POINT('Ctrl Pts',(23.3780462781492,-48.6808544629774,-26.7323240518326));
#29348=CARTESIAN_POINT('Ctrl Pts',(20.7420732792926,-46.4502604182672,-26.5743755286402));
#29349=CARTESIAN_POINT('Ctrl Pts',(17.4332844917096,-47.4380994344961,-26.4164270054477));
#29350=CARTESIAN_POINT('Ctrl Pts',(16.4516596187905,-50.7487514207967,-26.2584784822553));
#29351=CARTESIAN_POINT('Ctrl Pts',(18.6872050080179,-53.3805021188932,-26.1005299590628));
#29352=CARTESIAN_POINT('Ctrl Pts',(22.1130257584277,-52.9473163731849,-25.9425814358703));
#29353=CARTESIAN_POINT('Ctrl Pts',(23.6230222174753,-49.8417650404807,-25.7846329126778));
#29354=CARTESIAN_POINT('Ctrl Pts',(21.8481507499307,-46.8799263624337,-25.6266843894854));
#29355=CARTESIAN_POINT('Ctrl Pts',(18.3975850974581,-46.7464741037567,-25.4687358662929));
#29356=CARTESIAN_POINT('Ctrl Pts',(16.3999441875489,-49.5638694433452,-25.3107873431005));
#29357=CARTESIAN_POINT('Ctrl Pts',(17.6662377409256,-52.7747491690934,-25.152838819908));
#29358=CARTESIAN_POINT('Ctrl Pts',(21.0487276436386,-53.4737332515659,-24.9948902967155));
#29359=CARTESIAN_POINT('Ctrl Pts',(23.4799599601655,-51.0152272608972,-24.836941773523));
#29360=CARTESIAN_POINT('Ctrl Pts',(22.996783221692,-48.7754834195627,-24.7316427580614));
#29361=CARTESIAN_POINT('Ctrl Pts',(22.3360626576962,-48.0026984430694,-24.6789932503306));
#29362=CARTESIAN_POINT('Ctrl Pts',(20.7459328543469,-52.7901775698422,-40.1070022498898));
#29363=CARTESIAN_POINT('Ctrl Pts',(21.6689420470237,-52.5434180484685,-40.054352742159));
#29364=CARTESIAN_POINT('Ctrl Pts',(23.2352998106083,-51.0661295831258,-39.9490537266973));
#29365=CARTESIAN_POINT('Ctrl Pts',(22.6611589182799,-47.8681341248537,-39.7911052035049));
#29366=CARTESIAN_POINT('Ctrl Pts',(19.6696721767562,-46.6089850481313,-39.6331566803124));
#29367=CARTESIAN_POINT('Ctrl Pts',(16.9799413705986,-48.4214879457904,-39.4752081571199));
#29368=CARTESIAN_POINT('Ctrl Pts',(17.0272741357351,-51.6666161432018,-39.3172596339275));
#29369=CARTESIAN_POINT('Ctrl Pts',(19.7704552795004,-53.3999534232776,-39.159311110735));
#29370=CARTESIAN_POINT('Ctrl Pts',(22.7214722451228,-52.0510182863199,-39.0013625875425));
#29371=CARTESIAN_POINT('Ctrl Pts',(23.2051564374117,-48.8423054608625,-38.84341406435));
#29372=CARTESIAN_POINT('Ctrl Pts',(20.7827507736561,-46.683330368521,-38.6854655411576));
#29373=CARTESIAN_POINT('Ctrl Pts',(17.6506849497833,-47.5314329006501,-38.5275170179651));
#29374=CARTESIAN_POINT('Ctrl Pts',(16.6486534689832,-50.6177331765657,-38.3695684947727));
#29375=CARTESIAN_POINT('Ctrl Pts',(18.6851950831981,-53.1439420002899,-38.2116199715802));
#29376=CARTESIAN_POINT('Ctrl Pts',(21.9138257459041,-52.8196400414271,-38.0536714483878));
#29377=CARTESIAN_POINT('Ctrl Pts',(23.4072511123288,-49.9388532941425,-37.8957229251952));
#29378=CARTESIAN_POINT('Ctrl Pts',(21.8114243662861,-47.1135078711303,-37.7377744020028));
#29379=CARTESIAN_POINT('Ctrl Pts',(18.5732348198147,-46.905256336479,-37.5798258788103));
#29380=CARTESIAN_POINT('Ctrl Pts',(16.6286495775531,-49.5029151289302,-37.4218773556178));
#29381=CARTESIAN_POINT('Ctrl Pts',(17.7407653747764,-52.5512654701108,-37.2639288324254));
#29382=CARTESIAN_POINT('Ctrl Pts',(20.9012604216236,-53.2864610960517,-37.1059803092329));
#29383=CARTESIAN_POINT('Ctrl Pts',(23.2446100917232,-51.0419223525488,-36.9480317860405));
#29384=CARTESIAN_POINT('Ctrl Pts',(22.6461704534581,-47.8527043241565,-36.790083262848));
#29385=CARTESIAN_POINT('Ctrl Pts',(19.6485285539981,-46.6103739661872,-36.6321347396555));
#29386=CARTESIAN_POINT('Ctrl Pts',(16.9695551204265,-48.4413144481962,-36.474186216463));
#29387=CARTESIAN_POINT('Ctrl Pts',(17.0381938947004,-51.6854677117661,-36.3162376932706));
#29388=CARTESIAN_POINT('Ctrl Pts',(19.7922121842078,-53.4014586637584,-36.1582891700781));
#29389=CARTESIAN_POINT('Ctrl Pts',(22.7346253673064,-52.0334504952578,-36.0003406468857));
#29390=CARTESIAN_POINT('Ctrl Pts',(23.1976368994413,-48.8217746076858,-35.8423921236931));
#29391=CARTESIAN_POINT('Ctrl Pts',(20.7614483067326,-46.67835984903,-35.6844436005007));
#29392=CARTESIAN_POINT('Ctrl Pts',(17.6348776926376,-47.5465751922353,-35.5264950773082));
#29393=CARTESIAN_POINT('Ctrl Pts',(16.6526915427226,-50.6392361910505,-35.3685465541158));
#29394=CARTESIAN_POINT('Ctrl Pts',(18.7054081672171,-53.1523211769542,-35.2105980309233));
#29395=CARTESIAN_POINT('Ctrl Pts',(21.9318918332747,-52.8072924252161,-35.0526495077308));
#29396=CARTESIAN_POINT('Ctrl Pts',(23.4067879299314,-49.9169770114804,-34.8947009845384));
#29397=CARTESIAN_POINT('Ctrl Pts',(21.7928530232929,-47.1019360164021,-34.7367524613459));
#29398=CARTESIAN_POINT('Ctrl Pts',(18.5533928075934,-46.9144814946219,-34.5788039381534));
#29399=CARTESIAN_POINT('Ctrl Pts',(16.6255273366806,-49.5245727598638,-34.420855414961));
#29400=CARTESIAN_POINT('Ctrl Pts',(17.7571935996524,-52.5657194442717,-34.2629068917685));
#29401=CARTESIAN_POINT('Ctrl Pts',(20.9223442139462,-53.2806063413878,-34.104958368576));
#29402=CARTESIAN_POINT('Ctrl Pts',(23.2512333812862,-51.0210672438993,-33.9470098453835));
#29403=CARTESIAN_POINT('Ctrl Pts',(22.6323281236075,-47.8357575307237,-33.7890613221911));
#29404=CARTESIAN_POINT('Ctrl Pts',(19.6267710148948,-46.6127006419817,-33.6311127989986));
#29405=CARTESIAN_POINT('Ctrl Pts',(16.9596092757305,-48.4608050611018,-33.4731642758062));
#29406=CARTESIAN_POINT('Ctrl Pts',(17.0490773369575,-51.7044507188229,-33.3152157526136));
#29407=CARTESIAN_POINT('Ctrl Pts',(19.8140572285093,-53.4027227483126,-33.1572672294212));
#29408=CARTESIAN_POINT('Ctrl Pts',(22.7476257757779,-52.0158495510415,-32.9993187062287));
#29409=CARTESIAN_POINT('Ctrl Pts',(23.1900055974093,-48.8012668751339,-32.8413701830363));
#29410=CARTESIAN_POINT('Ctrl Pts',(20.7401043635042,-46.6735390657223,-32.6834216598438));
#29411=CARTESIAN_POINT('Ctrl Pts',(17.6191730124666,-47.5618122156842,-32.5254731366514));
#29412=CARTESIAN_POINT('Ctrl Pts',(16.6568650814459,-50.6607160755559,-32.3675246134588));
#29413=CARTESIAN_POINT('Ctrl Pts',(18.7256759042258,-53.1605687644921,-32.2095760902664));
#29414=CARTESIAN_POINT('Ctrl Pts',(21.9498776278288,-52.7948298790171,-32.0516275670739));
#29415=CARTESIAN_POINT('Ctrl Pts',(23.4061846091267,-49.8951037431457,-31.8936790438815));
#29416=CARTESIAN_POINT('Ctrl Pts',(21.7742075997515,-47.0904838530887,-31.735730520689));
#29417=CARTESIAN_POINT('Ctrl Pts',(18.5336105197666,-46.9238337645025,-31.5777819974966));
#29418=CARTESIAN_POINT('Ctrl Pts',(16.6225441832892,-49.5462500442751,-31.419833474304));
#29419=CARTESIAN_POINT('Ctrl Pts',(17.7737143151483,-52.5800676087223,-31.2618849511116));
#29420=CARTESIAN_POINT('Ctrl Pts',(20.943389968044,-53.2746163415502,-31.1039364279191));
#29421=CARTESIAN_POINT('Ctrl Pts',(23.2577226288231,-51.0001700304486,-30.9459879047267));
#29422=CARTESIAN_POINT('Ctrl Pts',(22.6183772612034,-47.8188999715357,-30.7880393815342));
#29423=CARTESIAN_POINT('Ctrl Pts',(19.6050288651951,-46.6151669732725,-30.6300908583417));
#29424=CARTESIAN_POINT('Ctrl Pts',(16.9497887846104,-48.4803591353003,-30.4721423351492));
#29425=CARTESIAN_POINT('Ctrl Pts',(17.0600824450388,-51.7233634515632,-30.3141938119568));
#29426=CARTESIAN_POINT('Ctrl Pts',(19.8359099389999,-53.4038465400247,-30.1562452887643));
#29427=CARTESIAN_POINT('Ctrl Pts',(22.7605129006961,-51.9981654939569,-29.9982967655718));
#29428=CARTESIAN_POINT('Ctrl Pts',(23.1822427725361,-48.7808085659784,-29.8403482423793));
#29429=CARTESIAN_POINT('Ctrl Pts',(20.718729906056,-46.6688554311885,-29.6823997191869));
#29430=CARTESIAN_POINT('Ctrl Pts',(17.603566492938,-47.5771497647728,-29.5244511959944));
#29431=CARTESIAN_POINT('Ctrl Pts',(16.6611764564406,-50.6821687189482,-29.366502672802));
#29432=CARTESIAN_POINT('Ctrl Pts',(18.7459961811647,-53.1686860429378,-29.2085541496095));
#29433=CARTESIAN_POINT('Ctrl Pts',(21.9677830296167,-52.7822521029042,-29.050605626417));
#29434=CARTESIAN_POINT('Ctrl Pts',(23.4054408525466,-49.8732347997812,-28.8926571032246));
#29435=CARTESIAN_POINT('Ctrl Pts',(21.7554890262427,-47.0791516478272,-28.7347085800321));
#29436=CARTESIAN_POINT('Ctrl Pts',(18.5138886906926,-46.933312864157,-28.5767600568396));
#29437=CARTESIAN_POINT('Ctrl Pts',(16.6197002811342,-49.5679460355797,-28.4188115336471));
#29438=CARTESIAN_POINT('Ctrl Pts',(17.7903268197514,-52.5943094000035,-28.2608630104547));
#29439=CARTESIAN_POINT('Ctrl Pts',(20.9643968262331,-53.2684913262547,-28.1029144872623));
#29440=CARTESIAN_POINT('Ctrl Pts',(23.2640775621583,-50.9792315886794,-27.9449659640697));
#29441=CARTESIAN_POINT('Ctrl Pts',(22.6043184429442,-47.8021323217292,-27.7870174408773));
#29442=CARTESIAN_POINT('Ctrl Pts',(19.5833030021837,-46.6177728930778,-27.6290689176848));
#29443=CARTESIAN_POINT('Ctrl Pts',(16.9400940482998,-48.4999757979521,-27.4711203944923));
#29444=CARTESIAN_POINT('Ctrl Pts',(17.071208773474,-51.7422052616489,-27.3131718712999));
#29445=CARTESIAN_POINT('Ctrl Pts',(19.8577693977516,-53.4048297315116,-27.1552233481074));
#29446=CARTESIAN_POINT('Ctrl Pts',(22.7732862447201,-51.9803995725483,-26.997274824915));
#29447=CARTESIAN_POINT('Ctrl Pts',(23.1743486770808,-48.7603994896662,-26.8393263017224));
#29448=CARTESIAN_POINT('Ctrl Pts',(20.6973259507001,-46.6643111972318,-26.68137777853));
#29449=CARTESIAN_POINT('Ctrl Pts',(17.5880585085861,-47.5925831083121,-26.5234292553375));
#29450=CARTESIAN_POINT('Ctrl Pts',(16.6656260253793,-50.7036013974831,-26.3654807321451));
#29451=CARTESIAN_POINT('Ctrl Pts',(18.7663670941892,-53.1766564296025,-26.2075322089526));
#29452=CARTESIAN_POINT('Ctrl Pts',(21.9856094229051,-52.7695919652361,-26.0495836857601));
#29453=CARTESIAN_POINT('Ctrl Pts',(23.4045524649764,-49.8513066746105,-25.8916351625676));
#29454=CARTESIAN_POINT('Ctrl Pts',(21.7367064880185,-47.0680681055589,-25.7336866393752));
#29455=CARTESIAN_POINT('Ctrl Pts',(18.4942113851663,-46.942663073803,-25.5757381161827));
#29456=CARTESIAN_POINT('Ctrl Pts',(16.6170290562352,-49.5901682980168,-25.4177895929903));
#29457=CARTESIAN_POINT('Ctrl Pts',(17.8069645796052,-52.6074306356065,-25.2598410697978));
#29458=CARTESIAN_POINT('Ctrl Pts',(20.9854889288333,-53.2642656860466,-25.1018925466053));
#29459=CARTESIAN_POINT('Ctrl Pts',(23.2701169215177,-50.9540086331591,-24.9439440234129));
#29460=CARTESIAN_POINT('Ctrl Pts',(22.8160759421236,-48.8493222806574,-24.8386450079512));
#29461=CARTESIAN_POINT('Ctrl Pts',(22.1951971040192,-48.1231365609213,-24.7859955002204));
#29462=CARTESIAN_POINT('Ctrl Pts',(20.698066426161,-52.6111321859386,-40.2140044997796));
#29463=CARTESIAN_POINT('Ctrl Pts',(21.561846221743,-52.3802071955689,-40.1613549920488));
#29464=CARTESIAN_POINT('Ctrl Pts',(23.0276909820899,-50.9977161665157,-40.0560559765871));
#29465=CARTESIAN_POINT('Ctrl Pts',(22.4903926468778,-48.0049357206273,-39.8981074533947));
#29466=CARTESIAN_POINT('Ctrl Pts',(19.6908692763838,-46.8265860999219,-39.7401589302022));
#29467=CARTESIAN_POINT('Ctrl Pts',(17.1737381964913,-48.5227808885037,-39.5822104070097));
#29468=CARTESIAN_POINT('Ctrl Pts',(17.2180336233606,-51.5596695709103,-39.4242618838173));
#29469=CARTESIAN_POINT('Ctrl Pts',(19.7851851386495,-53.1817787907722,-39.2663133606248));
#29470=CARTESIAN_POINT('Ctrl Pts',(22.5468356742545,-51.9194046713169,-39.1083648374324));
#29471=CARTESIAN_POINT('Ctrl Pts',(22.9994819057941,-48.9165945905019,-38.9504163142399));
#29472=CARTESIAN_POINT('Ctrl Pts',(20.7325217436886,-46.8961606893823,-38.7924677910474));
#29473=CARTESIAN_POINT('Ctrl Pts',(17.8014402349031,-47.6898405764811,-38.634519267855));
#29474=CARTESIAN_POINT('Ctrl Pts',(16.8637090026257,-50.5780933074249,-38.4765707446625));
#29475=CARTESIAN_POINT('Ctrl Pts',(18.7695659682742,-52.9421955922846,-38.31862222147));
#29476=CARTESIAN_POINT('Ctrl Pts',(21.7910157609398,-52.6387040540034,-38.1606736982776));
#29477=CARTESIAN_POINT('Ctrl Pts',(23.1886081879298,-49.9427770714472,-38.002725175085));
#29478=CARTESIAN_POINT('Ctrl Pts',(21.6951854664471,-47.2987337495597,-37.8447766518926));
#29479=CARTESIAN_POINT('Ctrl Pts',(18.6647901825227,-47.1038456926932,-37.6868281287001));
#29480=CARTESIAN_POINT('Ctrl Pts',(16.8449887586807,-49.5348130097445,-37.5288796055077));
#29481=CARTESIAN_POINT('Ctrl Pts',(17.8857402090571,-52.3875510490384,-37.3709310823152));
#29482=CARTESIAN_POINT('Ctrl Pts',(20.8434266407449,-53.0755692535444,-37.2129825591227));
#29483=CARTESIAN_POINT('Ctrl Pts',(23.0364038235026,-50.9750623112288,-37.0550340359302));
#29484=CARTESIAN_POINT('Ctrl Pts',(22.4763659901743,-47.9904960485225,-36.8970855127378));
#29485=CARTESIAN_POINT('Ctrl Pts',(19.6710824375433,-46.8278858912607,-36.7391369895453));
#29486=CARTESIAN_POINT('Ctrl Pts',(17.164018430836,-48.5413351264584,-36.5811884663529));
#29487=CARTESIAN_POINT('Ctrl Pts',(17.2282526626093,-51.5773114364193,-36.4232399431604));
#29488=CARTESIAN_POINT('Ctrl Pts',(19.8055459052051,-53.1831874401391,-36.2652914199679));
#29489=CARTESIAN_POINT('Ctrl Pts',(22.5591447620525,-51.9029642034506,-36.1073428967754));
#29490=CARTESIAN_POINT('Ctrl Pts',(22.9924448957378,-48.897381199887,-35.949394373583));
#29491=CARTESIAN_POINT('Ctrl Pts',(20.7125862536951,-46.8915091275734,-35.7914458503905));
#29492=CARTESIAN_POINT('Ctrl Pts',(17.786647327688,-47.7040111889018,-35.633497327198));
#29493=CARTESIAN_POINT('Ctrl Pts',(16.8674879536229,-50.5982164758651,-35.4755488040056));
#29494=CARTESIAN_POINT('Ctrl Pts',(18.788481980943,-52.9500370781157,-35.3176002808131));
#29495=CARTESIAN_POINT('Ctrl Pts',(21.8079225494959,-52.6271487829494,-35.1596517576206));
#29496=CARTESIAN_POINT('Ctrl Pts',(23.1881747278953,-49.9223045874071,-35.0017032344282));
#29497=CARTESIAN_POINT('Ctrl Pts',(21.6778058444655,-47.2879044594606,-34.8437547112357));
#29498=CARTESIAN_POINT('Ctrl Pts',(18.6462214300157,-47.1124788734655,-34.6858061880432));
#29499=CARTESIAN_POINT('Ctrl Pts',(16.8420668716573,-49.5550808729132,-34.5278576648508));
#29500=CARTESIAN_POINT('Ctrl Pts',(17.9011142365724,-52.4010775132872,-34.3699091416583));
#29501=CARTESIAN_POINT('Ctrl Pts',(20.8631574884625,-53.0700901978351,-34.2119606184659));
#29502=CARTESIAN_POINT('Ctrl Pts',(23.0426020973119,-50.9555454725786,-34.0540120952733));
#29503=CARTESIAN_POINT('Ctrl Pts',(22.4634119210885,-47.9746367289368,-33.8960635720809));
#29504=CARTESIAN_POINT('Ctrl Pts',(19.650721077301,-46.8300632645287,-33.7381150488884));
#29505=CARTESIAN_POINT('Ctrl Pts',(17.1547108098864,-48.5595750289046,-33.580166525696));
#29506=CARTESIAN_POINT('Ctrl Pts',(17.2384377155889,-51.5950763060275,-33.4222180025035));
#29507=CARTESIAN_POINT('Ctrl Pts',(19.8259891554466,-53.1843704085283,-33.264269479311));
#29508=CARTESIAN_POINT('Ctrl Pts',(22.5713109357603,-51.8864927098645,-33.1063209561185));
#29509=CARTESIAN_POINT('Ctrl Pts',(22.9853032935072,-48.8781894462487,-32.9483724329261));
#29510=CARTESIAN_POINT('Ctrl Pts',(20.6926119489265,-46.8869976933937,-32.7904239097336));
#29511=CARTESIAN_POINT('Ctrl Pts',(17.7719504150944,-47.718270454253,-32.6324753865412));
#29512=CARTESIAN_POINT('Ctrl Pts',(16.8713936768312,-50.6183179985742,-32.4745268633487));
#29513=CARTESIAN_POINT('Ctrl Pts',(18.8074491395251,-52.9577554188798,-32.3165783401562));
#29514=CARTESIAN_POINT('Ctrl Pts',(21.8247541976167,-52.615485956952,-32.1586298169637));
#29515=CARTESIAN_POINT('Ctrl Pts',(23.1876101221194,-49.9018349242652,-32.0006812937713));
#29516=CARTESIAN_POINT('Ctrl Pts',(21.6603568956761,-47.2771871801915,-31.8427327705788));
#29517=CARTESIAN_POINT('Ctrl Pts',(18.6277085693955,-47.1212310092294,-31.6847842473863));
#29518=CARTESIAN_POINT('Ctrl Pts',(16.8392751468868,-49.575367128398,-31.5268357241939));
#29519=CARTESIAN_POINT('Ctrl Pts',(17.9165748195948,-52.414504957623,-31.3688872010014));
#29520=CARTESIAN_POINT('Ctrl Pts',(20.8828527388637,-53.0644845756201,-31.2109386778089));
#29521=CARTESIAN_POINT('Ctrl Pts',(23.0486749305571,-50.9359892309876,-31.0529901546165));
#29522=CARTESIAN_POINT('Ctrl Pts',(22.4503562839711,-47.9588609174444,-30.895041631424));
#29523=CARTESIAN_POINT('Ctrl Pts',(19.6303741189261,-46.8323713316152,-30.7370931082315));
#29524=CARTESIAN_POINT('Ctrl Pts',(17.1455204985878,-48.5778743203397,-30.579144585039));
#29525=CARTESIAN_POINT('Ctrl Pts',(17.2487366271103,-51.6127754108142,-30.4211960618466));
#29526=CARTESIAN_POINT('Ctrl Pts',(19.8464395799389,-53.1854220866514,-30.2632475386541));
#29527=CARTESIAN_POINT('Ctrl Pts',(22.5833710953078,-51.8699434367532,-30.1052990154617));
#29528=CARTESIAN_POINT('Ctrl Pts',(22.9780386082415,-48.8590439445134,-29.9473504922691));
#29529=CARTESIAN_POINT('Ctrl Pts',(20.6726090880323,-46.8826146071662,-29.7894019690767));
#29530=CARTESIAN_POINT('Ctrl Pts',(17.7573453641857,-47.7326237945248,-29.6314534458842));
#29531=CARTESIAN_POINT('Ctrl Pts',(16.8754283913727,-50.6383940282292,-29.4735049226918));
#29532=CARTESIAN_POINT('Ctrl Pts',(18.8264654665559,-52.9653518124717,-29.3155563994993));
#29533=CARTESIAN_POINT('Ctrl Pts',(21.8415106117661,-52.6037152953314,-29.1576078763068));
#29534=CARTESIAN_POINT('Ctrl Pts',(23.1869140923162,-49.8813693085608,-28.9996593531144));
#29535=CARTESIAN_POINT('Ctrl Pts',(21.6428394909445,-47.2665821612795,-28.8417108299219));
#29536=CARTESIAN_POINT('Ctrl Pts',(18.6092522878967,-47.1301018361149,-28.6837623067294));
#29537=CARTESIAN_POINT('Ctrl Pts',(16.8366137376164,-49.5956708903569,-28.525813783537));
#29538=CARTESIAN_POINT('Ctrl Pts',(17.9321213016278,-52.4278328547439,-28.3678652603445));
#29539=CARTESIAN_POINT('Ctrl Pts',(20.9025115893025,-53.0587526018739,-28.209916737152));
#29540=CARTESIAN_POINT('Ctrl Pts',(23.0546220685279,-50.9163944066948,-28.0519682139595));
#29541=CARTESIAN_POINT('Ctrl Pts',(22.4371996185138,-47.9431692458585,-27.8940196907671));
#29542=CARTESIAN_POINT('Ctrl Pts',(19.6100424021244,-46.8348100298369,-27.7360711675746));
#29543=CARTESIAN_POINT('Ctrl Pts',(17.1364478724265,-48.5962321839338,-27.5781226443822));
#29544=CARTESIAN_POINT('Ctrl Pts',(17.259148980289,-51.6304081440452,-27.4201741211897));
#29545=CARTESIAN_POINT('Ctrl Pts',(19.8668963196571,-53.1863421868501,-27.2622255979972));
#29546=CARTESIAN_POINT('Ctrl Pts',(22.5953247752684,-51.8533175525428,-27.1042770748048));
#29547=CARTESIAN_POINT('Ctrl Pts',(22.9706510760124,-48.8399445163551,-26.9463285516123));
#29548=CARTESIAN_POINT('Ctrl Pts',(20.6525786221077,-46.8783619761964,-26.7883800284198));
#29549=CARTESIAN_POINT('Ctrl Pts',(17.7428325254625,-47.747066782128,-26.6304315052274));
#29550=CARTESIAN_POINT('Ctrl Pts',(16.8795924319682,-50.6584513741695,-26.4724829820349));
#29551=CARTESIAN_POINT('Ctrl Pts',(18.8455291803604,-52.9728107403119,-26.3145344588424));
#29552=CARTESIAN_POINT('Ctrl Pts',(21.8581930873826,-52.5918675572875,-26.1565859356499));
#29553=CARTESIAN_POINT('Ctrl Pts',(23.1860827124775,-49.8608483087402,-25.9986374124575));
#29554=CARTESIAN_POINT('Ctrl Pts',(21.6252622261063,-47.2562098486842,-25.840688889265));
#29555=CARTESIAN_POINT('Ctrl Pts',(18.5908376728745,-47.1388520438493,-25.6827403660725));
#29556=CARTESIAN_POINT('Ctrl Pts',(16.8341139249216,-49.6164671526884,-25.5247918428801));
#29557=CARTESIAN_POINT('Ctrl Pts',(17.9476914182848,-52.4401121021197,-25.3668433196876));
#29558=CARTESIAN_POINT('Ctrl Pts',(20.9222502140279,-53.0547981205273,-25.2088947964951));
#29559=CARTESIAN_POINT('Ctrl Pts',(23.0602738828699,-50.892790005421,-25.0509462733027));
#29560=CARTESIAN_POINT('Ctrl Pts',(22.6353686625552,-48.923161141752,-24.945647257841));
#29561=CARTESIAN_POINT('Ctrl Pts',(22.0543315503421,-48.2435746787732,-24.8929977501102));
#29562=CARTESIAN_POINT('Ctrl Pts',(20.6501999979751,-52.4320868020351,-40.3210067496694));
#29563=CARTESIAN_POINT('Ctrl Pts',(21.4547503964622,-52.2169963426693,-40.2683572419386));
#29564=CARTESIAN_POINT('Ctrl Pts',(22.8200821535714,-50.9293027499057,-40.1630582264769));
#29565=CARTESIAN_POINT('Ctrl Pts',(22.3196263754757,-48.141737316401,-40.0051097032845));
#29566=CARTESIAN_POINT('Ctrl Pts',(19.7120663760114,-47.0441871517124,-39.847161180092));
#29567=CARTESIAN_POINT('Ctrl Pts',(17.367535022384,-48.6240738312172,-39.6892126568995));
#29568=CARTESIAN_POINT('Ctrl Pts',(17.4087931109861,-51.4527229986188,-39.5312641337071));
#29569=CARTESIAN_POINT('Ctrl Pts',(19.7999149977987,-52.9636041582669,-39.3733156105146));
#29570=CARTESIAN_POINT('Ctrl Pts',(22.3721991033862,-51.7877910563139,-39.2153670873222));
#29571=CARTESIAN_POINT('Ctrl Pts',(22.7938073741765,-48.9908837201412,-39.0574185641296));
#29572=CARTESIAN_POINT('Ctrl Pts',(20.6822927137212,-47.1089910102435,-38.8994700409372));
#29573=CARTESIAN_POINT('Ctrl Pts',(17.9521955200229,-47.8482482523122,-38.7415215177447));
#29574=CARTESIAN_POINT('Ctrl Pts',(17.0787645362682,-50.5384534382841,-38.5835729945523));
#29575=CARTESIAN_POINT('Ctrl Pts',(18.8539368533503,-52.7404491842795,-38.4256244713598));
#29576=CARTESIAN_POINT('Ctrl Pts',(21.6682057759756,-52.4577680665795,-38.2676759481674));
#29577=CARTESIAN_POINT('Ctrl Pts',(22.9699652635309,-49.946700848752,-38.1097274249748));
#29578=CARTESIAN_POINT('Ctrl Pts',(21.5789465666081,-47.4839596279891,-37.9517789017824));
#29579=CARTESIAN_POINT('Ctrl Pts',(18.7563455452306,-47.3024350489073,-37.7938303785899));
#29580=CARTESIAN_POINT('Ctrl Pts',(17.0613279398084,-49.5667108905587,-37.6358818553975));
#29581=CARTESIAN_POINT('Ctrl Pts',(18.0307150433377,-52.223836627966,-37.477933332205));
#29582=CARTESIAN_POINT('Ctrl Pts',(20.7855928598664,-52.8646774110371,-37.3199848090125));
#29583=CARTESIAN_POINT('Ctrl Pts',(22.8281975552819,-50.9082022699088,-37.1620362858201));
#29584=CARTESIAN_POINT('Ctrl Pts',(22.3065615268905,-48.1282877728884,-37.0040877626276));
#29585=CARTESIAN_POINT('Ctrl Pts',(19.6936363210884,-47.0453978163343,-36.8461392394351));
#29586=CARTESIAN_POINT('Ctrl Pts',(17.3584817412455,-48.6413558047206,-36.6881907162427));
#29587=CARTESIAN_POINT('Ctrl Pts',(17.4183114305182,-51.4691551610726,-36.5302421930502));
#29588=CARTESIAN_POINT('Ctrl Pts',(19.8188796262023,-52.9649162165198,-36.3722936698577));
#29589=CARTESIAN_POINT('Ctrl Pts',(22.3836641567986,-51.7724779116434,-36.2143451466652));
#29590=CARTESIAN_POINT('Ctrl Pts',(22.7872528920342,-48.9729877920881,-36.0563966234728));
#29591=CARTESIAN_POINT('Ctrl Pts',(20.6637242006576,-47.1046584061167,-35.8984481002803));
#29592=CARTESIAN_POINT('Ctrl Pts',(17.9384169627383,-47.8614471855684,-35.7404995770878));
#29593=CARTESIAN_POINT('Ctrl Pts',(17.0822843645233,-50.5571967606797,-35.5825510538954));
#29594=CARTESIAN_POINT('Ctrl Pts',(18.8715557946688,-52.7477529792771,-35.4246025307029));
#29595=CARTESIAN_POINT('Ctrl Pts',(21.6839532657172,-52.4470051406827,-35.2666540075104));
#29596=CARTESIAN_POINT('Ctrl Pts',(22.9695615258592,-49.9276321633338,-35.108705484318));
#29597=CARTESIAN_POINT('Ctrl Pts',(21.562758665638,-47.4738729025192,-34.9507569611255));
#29598=CARTESIAN_POINT('Ctrl Pts',(18.739050052438,-47.3104762523091,-34.792808437933));
#29599=CARTESIAN_POINT('Ctrl Pts',(17.058606406634,-49.5855889859624,-34.6348599147405));
#29600=CARTESIAN_POINT('Ctrl Pts',(18.0450348734924,-52.2364355823028,-34.4769113915481));
#29601=CARTESIAN_POINT('Ctrl Pts',(20.8039707629787,-52.8595740542826,-34.3189628683556));
#29602=CARTESIAN_POINT('Ctrl Pts',(22.8339708133377,-50.8900237012579,-34.1610143451632));
#29603=CARTESIAN_POINT('Ctrl Pts',(22.2944957185695,-48.11351592715,-34.0030658219707));
#29604=CARTESIAN_POINT('Ctrl Pts',(19.6746711397071,-47.0474258870756,-33.8451172987782));
#29605=CARTESIAN_POINT('Ctrl Pts',(17.3498123440423,-48.6583449967074,-33.6871687755857));
#29606=CARTESIAN_POINT('Ctrl Pts',(17.4277980942202,-51.4857018932322,-33.5292202523933));
#29607=CARTESIAN_POINT('Ctrl Pts',(19.837921082384,-52.9660180687438,-33.3712717292008));
#29608=CARTESIAN_POINT('Ctrl Pts',(22.3949960957427,-51.7571358686874,-33.2133232060084));
#29609=CARTESIAN_POINT('Ctrl Pts',(22.7806009896051,-48.9551120173637,-33.0553746828159));
#29610=CARTESIAN_POINT('Ctrl Pts',(20.6451195343488,-47.100456321065,-32.8974261596234));
#29611=CARTESIAN_POINT('Ctrl Pts',(17.9247278177222,-47.8747286928219,-32.7394776364309));
#29612=CARTESIAN_POINT('Ctrl Pts',(17.0859222722165,-50.5759199215923,-32.5815291132385));
#29613=CARTESIAN_POINT('Ctrl Pts',(18.8892223748244,-52.7549420732675,-32.423580590046));
#29614=CARTESIAN_POINT('Ctrl Pts',(21.6996307674046,-52.4361420348868,-32.2656320668536));
#29615=CARTESIAN_POINT('Ctrl Pts',(22.9690356351122,-49.9085661053849,-32.107683543661));
#29616=CARTESIAN_POINT('Ctrl Pts',(21.5465061916006,-47.4638905072944,-31.9497350204686));
#29617=CARTESIAN_POINT('Ctrl Pts',(18.7218066190244,-47.3186282539564,-31.7917864972761));
#29618=CARTESIAN_POINT('Ctrl Pts',(17.0560061104844,-49.6044842125209,-31.6338379740837));
#29619=CARTESIAN_POINT('Ctrl Pts',(18.0594353240415,-52.2489423065238,-31.4758894508912));
#29620=CARTESIAN_POINT('Ctrl Pts',(20.8223155096835,-52.8543528096899,-31.3179409276987));
#29621=CARTESIAN_POINT('Ctrl Pts',(22.8396272322911,-50.8718084315267,-31.1599924045063));
#29622=CARTESIAN_POINT('Ctrl Pts',(22.2823353067388,-48.0988218633531,-31.0020438813138));
#29623=CARTESIAN_POINT('Ctrl Pts',(19.655719372657,-47.049575689958,-30.8440953581213));
#29624=CARTESIAN_POINT('Ctrl Pts',(17.3412522125651,-48.6753895053789,-30.6861468349288));
#29625=CARTESIAN_POINT('Ctrl Pts',(17.4373908091818,-51.5021873700654,-30.5281983117364));
#29626=CARTESIAN_POINT('Ctrl Pts',(19.8569692208779,-52.9669976332779,-30.3702497885439));
#29627=CARTESIAN_POINT('Ctrl Pts',(22.4062292899195,-51.7417213795498,-30.2123012653515));
#29628=CARTESIAN_POINT('Ctrl Pts',(22.773834443947,-48.9372793230483,-30.054352742159));
#29629=CARTESIAN_POINT('Ctrl Pts',(20.6264882700084,-47.096373783144,-29.8964042189665));
#29630=CARTESIAN_POINT('Ctrl Pts',(17.9111242354336,-47.8880978242769,-29.738455695774));
#29631=CARTESIAN_POINT('Ctrl Pts',(17.0896803263047,-50.5946193375101,-29.5805071725816));
#29632=CARTESIAN_POINT('Ctrl Pts',(18.9069347519471,-52.7620175820056,-29.4225586493891));
#29633=CARTESIAN_POINT('Ctrl Pts',(21.7152381939154,-52.4251784877586,-29.2646101261966));
#29634=CARTESIAN_POINT('Ctrl Pts',(22.9683873320859,-49.8895038173406,-29.1066616030042));
#29635=CARTESIAN_POINT('Ctrl Pts',(21.5301899556464,-47.4540126747319,-28.9487130798117));
#29636=CARTESIAN_POINT('Ctrl Pts',(18.7046158851008,-47.3268908080728,-28.7907645566192));
#29637=CARTESIAN_POINT('Ctrl Pts',(17.0535271940985,-49.6233957451342,-28.6328160334268));
#29638=CARTESIAN_POINT('Ctrl Pts',(18.0739157835043,-52.2613563094843,-28.4748675102343));
#29639=CARTESIAN_POINT('Ctrl Pts',(20.8406263523719,-52.8490138774931,-28.3169189870418));
#29640=CARTESIAN_POINT('Ctrl Pts',(22.8451665748976,-50.8535572247102,-28.1589704638494));
#29641=CARTESIAN_POINT('Ctrl Pts',(22.2700807940834,-48.0842061699878,-28.0010219406569));
#29642=CARTESIAN_POINT('Ctrl Pts',(19.636781802065,-47.0518471665959,-27.8430734174644));
#29643=CARTESIAN_POINT('Ctrl Pts',(17.3328016965531,-48.6924885699155,-27.685124894272));
#29644=CARTESIAN_POINT('Ctrl Pts',(17.447089187104,-51.5186110264415,-27.5271763710795));
#29645=CARTESIAN_POINT('Ctrl Pts',(19.8760232415626,-52.9678546421884,-27.369227847887));
#29646=CARTESIAN_POINT('Ctrl Pts',(22.4173633058167,-51.7262355325375,-27.2112793246946));
#29647=CARTESIAN_POINT('Ctrl Pts',(22.7669534749441,-48.9194895430439,-27.0533308015021));
#29648=CARTESIAN_POINT('Ctrl Pts',(20.6078312935152,-47.0924127551611,-26.8953822783097));
#29649=CARTESIAN_POINT('Ctrl Pts',(17.897606542339,-47.901550455944,-26.7374337551171));
#29650=CARTESIAN_POINT('Ctrl Pts',(17.093558838557,-50.6133013508559,-26.5794852319247));
#29651=CARTESIAN_POINT('Ctrl Pts',(18.9246912665317,-52.7689650510212,-26.4215367087322));
#29652=CARTESIAN_POINT('Ctrl Pts',(21.73077675186,-52.4141431493388,-26.2635881855398));
#29653=CARTESIAN_POINT('Ctrl Pts',(22.9676129599786,-49.8703899428698,-26.1056396623473));
#29654=CARTESIAN_POINT('Ctrl Pts',(21.5138179641941,-47.4443515918095,-25.9476911391548));
#29655=CARTESIAN_POINT('Ctrl Pts',(18.6874639605827,-47.3350410138954,-25.7897426159623));
#29656=CARTESIAN_POINT('Ctrl Pts',(17.051198793608,-49.6427660073601,-25.6317940927699));
#29657=CARTESIAN_POINT('Ctrl Pts',(18.0884182569644,-52.2727935686328,-25.4738455695774));
#29658=CARTESIAN_POINT('Ctrl Pts',(20.8590114992225,-52.8453305550081,-25.3158970463849));
#29659=CARTESIAN_POINT('Ctrl Pts',(22.8504308442221,-50.8315713776829,-25.1579485231925));
#29660=CARTESIAN_POINT('Ctrl Pts',(22.4546613829867,-48.9970000028466,-25.0526495077308));
#29661=CARTESIAN_POINT('Ctrl Pts',(21.9134659966651,-48.3640127966251,-25.));
#29662=CARTESIAN_POINT('Ctrl Pts',(22.514945820706,-49.9982392595312,-39.112583302492));
#29663=CARTESIAN_POINT('Ctrl Pts',(22.5168590395215,-49.7066908675705,-39.0941950563712));
#29664=CARTESIAN_POINT('Ctrl Pts',(22.4699890228872,-49.4157373171367,-39.0758068102504));
#29665=CARTESIAN_POINT('Ctrl Pts',(22.3716202189689,-49.1433861578537,-39.0574185641297));
#29666=CARTESIAN_POINT('Ctrl Pts',(22.0899691540247,-48.3635861501753,-39.0047690563988));
#29667=CARTESIAN_POINT('Ctrl Pts',(21.386130933873,-47.7362885802094,-38.952119548668));
#29668=CARTESIAN_POINT('Ctrl Pts',(20.5791956248474,-47.5458493355713,-38.8994700409372));
#29669=CARTESIAN_POINT('Ctrl Pts',(19.7722603158218,-47.3554100909331,-38.8468205332064));
#29670=CARTESIAN_POINT('Ctrl Pts',(18.8622279179223,-47.6018291716227,-38.7941710254756));
#29671=CARTESIAN_POINT('Ctrl Pts',(18.2616398883468,-48.1734062429628,-38.7415215177447));
#29672=CARTESIAN_POINT('Ctrl Pts',(17.6610518587713,-48.7449833143029,-38.6888720100139));
#29673=CARTESIAN_POINT('Ctrl Pts',(17.3699081975197,-49.6417183762935,-38.6362225022831));
#29674=CARTESIAN_POINT('Ctrl Pts',(17.520198419741,-50.457085198288,-38.5835729945523));
#29675=CARTESIAN_POINT('Ctrl Pts',(17.6704886419622,-51.2724520202826,-38.5309234868215));
#29676=CARTESIAN_POINT('Ctrl Pts',(18.2622127476563,-52.006450602281,-38.4782739790906));
#29677=CARTESIAN_POINT('Ctrl Pts',(19.0271196209408,-52.3263363736636,-38.4256244713598));
#29678=CARTESIAN_POINT('Ctrl Pts',(19.7920264942254,-52.6462221450461,-38.372974963629));
#29679=CARTESIAN_POINT('Ctrl Pts',(20.7301161351005,-52.5519951058128,-38.3203254558982));
#29680=CARTESIAN_POINT('Ctrl Pts',(21.4161208701306,-52.0863703832249,-38.2676759481673));
#29681=CARTESIAN_POINT('Ctrl Pts',(22.0897219089449,-51.6291646515194,-38.2159783996089));
#29682=CARTESIAN_POINT('Ctrl Pts',(22.5202715562231,-50.8138703486238,-38.1642808510504));
#29683=CARTESIAN_POINT('Ctrl Pts',(22.5215368448905,-49.9997267149633,-38.112583302492));
#29684=CARTESIAN_POINT('Origin',(20.,-50.,-32.));
#29685=CARTESIAN_POINT('',(20.,-52.5175,-24.3199761284063));
#29686=CARTESIAN_POINT('Ctrl Pts',(17.4825,-50.,-25.));
#29687=CARTESIAN_POINT('Ctrl Pts',(17.4825,-50.3222180082023,-25.));
#29688=CARTESIAN_POINT('Ctrl Pts',(17.5480817994189,-50.6620957154614,-24.965994767533));
#29689=CARTESIAN_POINT('Ctrl Pts',(17.8069078640769,-51.2808669639972,-24.8434341672334));
#29690=CARTESIAN_POINT('Ctrl Pts',(17.9998598225217,-51.560142465796,-24.75619390213));
#29691=CARTESIAN_POINT('Ctrl Pts',(18.4404784589042,-52.0007611021785,-24.5883213994305));
#29692=CARTESIAN_POINT('Ctrl Pts',(18.719545764891,-52.1932581515168,-24.4956547875015));
#29693=CARTESIAN_POINT('Ctrl Pts',(19.3374025937983,-52.4517149721102,-24.3600905047278));
#29694=CARTESIAN_POINT('Ctrl Pts',(19.6768725637946,-52.5175,-24.3199761284063));
#29695=CARTESIAN_POINT('Ctrl Pts',(20.,-52.5175,-24.3199761284063));
#29696=CARTESIAN_POINT('Ctrl Pts',(20.,-52.5175,-24.3199761284063));
#29697=CARTESIAN_POINT('Ctrl Pts',(20.3231274362054,-52.5175,-24.3199761284063));
#29698=CARTESIAN_POINT('Ctrl Pts',(20.6625974062016,-52.4517149721102,-24.3600905047278));
#29699=CARTESIAN_POINT('Ctrl Pts',(21.2804542351089,-52.1932581515168,-24.4956547875015));
#29700=CARTESIAN_POINT('Ctrl Pts',(21.5595215410957,-52.0007611021785,-24.5883213994305));
#29701=CARTESIAN_POINT('Ctrl Pts',(22.0001401774783,-51.560142465796,-24.75619390213));
#29702=CARTESIAN_POINT('Ctrl Pts',(22.1930921359231,-51.2808669639972,-24.8434341672334));
#29703=CARTESIAN_POINT('Ctrl Pts',(22.4519182005811,-50.6620957154615,-24.965994767533));
#29704=CARTESIAN_POINT('Ctrl Pts',(22.5175,-50.3222180082023,-25.));
#29705=CARTESIAN_POINT('Ctrl Pts',(22.5175,-50.,-25.));
#29706=CARTESIAN_POINT('Origin',(20.,-50.,-32.));
#29707=CARTESIAN_POINT('Origin',(-20.,-50.,-24.));
#29708=CARTESIAN_POINT('Origin',(-20.,50.,-24.));
#29709=CARTESIAN_POINT('Origin',(20.,50.,-32.));
#29710=CARTESIAN_POINT('Origin',(20.,66.,25.));
#29711=CARTESIAN_POINT('Ctrl Pts',(19.2300979593296,64.5225674811446,25.));
#29712=CARTESIAN_POINT('Ctrl Pts',(19.281839231255,64.4874948330505,25.));
#29713=CARTESIAN_POINT('Ctrl Pts',(19.3355569853841,64.4556772697649,25.));
#29714=CARTESIAN_POINT('Ctrl Pts',(19.3909199227331,64.4270507505591,25.));
#29715=CARTESIAN_POINT('Ctrl Pts',(19.426030142418,64.4088963059748,25.));
#29716=CARTESIAN_POINT('Ctrl Pts',(19.4618029278252,64.3920259076849,25.));
#29717=CARTESIAN_POINT('Ctrl Pts',(19.4981613804728,64.3764304346951,25.));
#29718=CARTESIAN_POINT('Ctrl Pts',(19.5229472314038,64.365798874753,25.));
#29719=CARTESIAN_POINT('Ctrl Pts',(19.5480053751662,64.3557599229072,25.));
#29720=CARTESIAN_POINT('Ctrl Pts',(19.5733126916688,64.3463122740479,25.));
#29721=CARTESIAN_POINT('Ctrl Pts',(19.5868015745102,64.3412766461662,25.));
#29722=CARTESIAN_POINT('Ctrl Pts',(19.6003611975298,64.336409177933,25.));
#29723=CARTESIAN_POINT('Ctrl Pts',(19.6139743572948,64.33171419315,25.));
#29724=CARTESIAN_POINT('Ctrl Pts',(19.6763387771318,64.3102055935898,25.));
#29725=CARTESIAN_POINT('Ctrl Pts',(19.7398944948615,64.2922866657573,25.));
#29726=CARTESIAN_POINT('Ctrl Pts',(19.8042916188756,64.2779108681233,25.));
#29727=CARTESIAN_POINT('Ctrl Pts',(19.850744007574,64.267540992919,25.));
#29728=CARTESIAN_POINT('Ctrl Pts',(19.897635109279,64.2590155593061,25.));
#29729=CARTESIAN_POINT('Ctrl Pts',(19.9448427078687,64.2523311286925,25.));
#29730=CARTESIAN_POINT('Ctrl Pts',(19.9577423603646,64.2505045830807,25.));
#29731=CARTESIAN_POINT('Ctrl Pts',(19.9706656780993,64.2488155711042,25.));
#29732=CARTESIAN_POINT('Ctrl Pts',(19.9836102341249,64.247264183342,25.));
#29733=CARTESIAN_POINT('Ctrl Pts',(19.9969403079863,64.2456665917817,25.));
#29734=CARTESIAN_POINT('Ctrl Pts',(20.0102849815179,64.2442159339093,25.));
#29735=CARTESIAN_POINT('Ctrl Pts',(20.0236360018045,64.2429122860894,25.));
#29736=CARTESIAN_POINT('Ctrl Pts',(20.0911671831916,64.2363182673923,25.));
#29737=CARTESIAN_POINT('Ctrl Pts',(20.1589020463386,64.2334766424509,25.));
#29738=CARTESIAN_POINT('Ctrl Pts',(20.2264859165014,64.2343394624463,25.));
#29739=CARTESIAN_POINT('Ctrl Pts',(20.295048342074,64.2352147753216,25.));
#29740=CARTESIAN_POINT('Ctrl Pts',(20.3634563804349,64.239902250275,25.));
#29741=CARTESIAN_POINT('Ctrl Pts',(20.4313612181172,64.2484001199632,25.));
#29742=CARTESIAN_POINT('Ctrl Pts',(20.4734290714963,64.2536646511553,25.));
#29743=CARTESIAN_POINT('Ctrl Pts',(20.5153041663473,64.2603925631682,25.));
#29744=CARTESIAN_POINT('Ctrl Pts',(20.5569049437151,64.2685933800542,25.));
#29745=CARTESIAN_POINT('Ctrl Pts',(20.5909685471161,64.2753083837547,25.));
#29746=CARTESIAN_POINT('Ctrl Pts',(20.6248482693332,64.2830110591366,25.));
#29747=CARTESIAN_POINT('Ctrl Pts',(20.6584989914886,64.2917106170954,25.));
#29748=CARTESIAN_POINT('Ctrl Pts',(20.6722821250041,64.2952739037411,25.));
#29749=CARTESIAN_POINT('Ctrl Pts',(20.6860293036811,64.2990053184497,25.));
#29750=CARTESIAN_POINT('Ctrl Pts',(20.6997141699917,64.3028986531347,25.));
#29751=CARTESIAN_POINT('Ctrl Pts',(20.767509458307,64.3221863642084,25.));
#29752=CARTESIAN_POINT('Ctrl Pts',(20.8338951499891,64.3454732746142,25.));
#29753=CARTESIAN_POINT('Ctrl Pts',(20.8985085156353,64.3727406748912,25.));
#29754=CARTESIAN_POINT('Ctrl Pts',(20.9056752429655,64.3757650959352,25.));
#29755=CARTESIAN_POINT('Ctrl Pts',(20.912820174029,64.3788385395555,25.));
#29756=CARTESIAN_POINT('Ctrl Pts',(20.9199428180022,64.381961019588,25.));
#29757=CARTESIAN_POINT('Ctrl Pts',(20.9816953861963,64.4090325904643,25.));
#29758=CARTESIAN_POINT('Ctrl Pts',(21.0417735205151,64.4397857609011,25.));
#29759=CARTESIAN_POINT('Ctrl Pts',(21.1000352843316,64.4739103291622,25.));
#29760=CARTESIAN_POINT('Ctrl Pts',(21.1627111717192,64.5106202990872,25.));
#29761=CARTESIAN_POINT('Ctrl Pts',(21.2232860382956,64.5512318872835,25.));
#29762=CARTESIAN_POINT('Ctrl Pts',(21.2815632966598,64.5954199888185,25.));
#29763=CARTESIAN_POINT('Ctrl Pts',(21.2920884895073,64.6034006025823,25.));
#29764=CARTESIAN_POINT('Ctrl Pts',(21.3025386647321,64.6114980246855,25.));
#29765=CARTESIAN_POINT('Ctrl Pts',(21.3129125592066,64.6197105288189,25.));
#29766=CARTESIAN_POINT('Ctrl Pts',(21.3220886651644,64.6269748024524,25.));
#29767=CARTESIAN_POINT('Ctrl Pts',(21.3311980890197,64.6343235975034,25.));
#29768=CARTESIAN_POINT('Ctrl Pts',(21.3402381792021,64.641753616724,25.));
#29769=CARTESIAN_POINT('Ctrl Pts',(21.3951413928709,64.6868783803714,25.));
#29770=CARTESIAN_POINT('Ctrl Pts',(21.4475124849223,64.7350138905591,25.));
#29771=CARTESIAN_POINT('Ctrl Pts',(21.4972014371838,64.7858101432121,25.));
#29772=CARTESIAN_POINT('Ctrl Pts',(21.54793815392,64.8376775093934,25.));
#29773=CARTESIAN_POINT('Ctrl Pts',(21.5958791893217,64.8923195535381,25.));
#29774=CARTESIAN_POINT('Ctrl Pts',(21.6408446258094,64.9494149499861,25.));
#29775=CARTESIAN_POINT('Ctrl Pts',(21.686082829692,65.00685669607,25.));
#29776=CARTESIAN_POINT('Ctrl Pts',(21.7283100119046,65.0667823784968,25.));
#29777=CARTESIAN_POINT('Ctrl Pts',(21.7673110082825,65.1289063303553,25.));
#29778=CARTESIAN_POINT('Ctrl Pts',(21.7769380340976,65.1442410382814,25.));
#29779=CARTESIAN_POINT('Ctrl Pts',(21.7863683037242,65.1597098543281,25.));
#29780=CARTESIAN_POINT('Ctrl Pts',(21.7955981964646,65.1753087874189,25.));
#29781=CARTESIAN_POINT('Ctrl Pts',(21.8028478722767,65.1875610650027,25.));
#29782=CARTESIAN_POINT('Ctrl Pts',(21.8099746659192,65.199895168117,25.));
#29783=CARTESIAN_POINT('Ctrl Pts',(21.8169663572284,65.212290083603,25.));
#29784=CARTESIAN_POINT('Ctrl Pts',(21.8539815854589,65.2779109191527,25.));
#29785=CARTESIAN_POINT('Ctrl Pts',(21.8872827332467,65.3453487040639,25.));
#29786=CARTESIAN_POINT('Ctrl Pts',(21.9166890670406,65.4142571139814,25.));
#29787=CARTESIAN_POINT('Ctrl Pts',(21.9461274772774,65.4832406892256,25.));
#29788=CARTESIAN_POINT('Ctrl Pts',(21.9716633369393,65.5536989287888,25.));
#29789=CARTESIAN_POINT('Ctrl Pts',(21.9930795831037,65.625322085145,25.));
#29790=CARTESIAN_POINT('Ctrl Pts',(22.014008595814,65.6953157683622,25.));
#29791=CARTESIAN_POINT('Ctrl Pts',(22.0310038676764,65.7664228433862,25.));
#29792=CARTESIAN_POINT('Ctrl Pts',(22.0438192119979,65.8383774372798,25.));
#29793=CARTESIAN_POINT('Ctrl Pts',(22.0465680662148,65.8538114891385,25.));
#29794=CARTESIAN_POINT('Ctrl Pts',(22.0491244257846,65.8692845939399,25.));
#29795=CARTESIAN_POINT('Ctrl Pts',(22.0514855533718,65.8847942120883,25.));
#29796=CARTESIAN_POINT('Ctrl Pts',(22.0534987458236,65.8980183370176,25.));
#29797=CARTESIAN_POINT('Ctrl Pts',(22.0553700032061,65.9112690075299,25.));
#29798=CARTESIAN_POINT('Ctrl Pts',(22.0571001530702,65.9245445252814,25.));
#29799=CARTESIAN_POINT('Ctrl Pts',(21.8174278887594,66.9586205879594,25.));
#29800=CARTESIAN_POINT('Ctrl Pts',(21.7765814107043,67.0211003513439,25.));
#29801=CARTESIAN_POINT('Ctrl Pts',(21.7321382448712,67.0810293930508,25.));
#29802=CARTESIAN_POINT('Ctrl Pts',(21.6844272397568,67.1382579399872,25.));
#29803=CARTESIAN_POINT('Ctrl Pts',(21.637967675109,67.1939854051645,25.));
#29804=CARTESIAN_POINT('Ctrl Pts',(21.5884084550957,67.2471523904015,25.));
#29805=CARTESIAN_POINT('Ctrl Pts',(21.5360271611327,67.2975829314462,25.));
#29806=CARTESIAN_POINT('Ctrl Pts',(21.5243354888859,67.3088391894062,25.));
#29807=CARTESIAN_POINT('Ctrl Pts',(21.5125015557441,67.3199604168664,25.));
#29808=CARTESIAN_POINT('Ctrl Pts',(21.5005334335621,67.3309397166112,25.));
#29809=CARTESIAN_POINT('Ctrl Pts',(21.4456122493378,67.3813232383342,25.));
#29810=CARTESIAN_POINT('Ctrl Pts',(21.3879773343812,67.4286222799669,25.));
#29811=CARTESIAN_POINT('Ctrl Pts',(21.3279448353606,67.4726643541928,25.));
#29812=CARTESIAN_POINT('Ctrl Pts',(21.2858003429978,67.5035831213795,25.));
#29813=CARTESIAN_POINT('Ctrl Pts',(21.2424735350058,67.5328958196392,25.));
#29814=CARTESIAN_POINT('Ctrl Pts',(21.1980684694414,67.5605283676983,25.));
#29815=CARTESIAN_POINT('Ctrl Pts',(21.1811930594238,67.5710296601162,25.));
#29816=CARTESIAN_POINT('Ctrl Pts',(21.1641618931168,67.5812881669686,25.));
#29817=CARTESIAN_POINT('Ctrl Pts',(21.1469806065534,67.5912993349929,25.));
#29818=CARTESIAN_POINT('Ctrl Pts',(21.1305958626812,67.6008463746361,25.));
#29819=CARTESIAN_POINT('Ctrl Pts',(21.1140692794188,67.6101712136826,25.));
#29820=CARTESIAN_POINT('Ctrl Pts',(21.0974353366829,67.6192539953179,25.));
#29821=CARTESIAN_POINT('Ctrl Pts',(21.0337183685953,67.6540459455365,25.));
#29822=CARTESIAN_POINT('Ctrl Pts',(20.9683624441582,67.6853307441412,25.));
#29823=CARTESIAN_POINT('Ctrl Pts',(20.9016592645668,67.712946755633,25.));
#29824=CARTESIAN_POINT('Ctrl Pts',(20.8363884218304,67.7399697604452,25.));
#29825=CARTESIAN_POINT('Ctrl Pts',(20.7698266382456,67.7634800022219,25.));
#29826=CARTESIAN_POINT('Ctrl Pts',(20.7022386209724,67.7832777771816,25.));
#29827=CARTESIAN_POINT('Ctrl Pts',(20.6361329278297,67.8026413521051,25.));
#29828=CARTESIAN_POINT('Ctrl Pts',(20.5690447597529,67.8184536274702,25.));
#29829=CARTESIAN_POINT('Ctrl Pts',(20.5012257200427,67.8304791677269,25.));
#29830=CARTESIAN_POINT('Ctrl Pts',(20.479165553528,67.8343908335604,25.));
#29831=CARTESIAN_POINT('Ctrl Pts',(20.4570281345296,67.8379014394019,25.));
#29832=CARTESIAN_POINT('Ctrl Pts',(20.4348224165778,67.8410017088834,25.));
#29833=CARTESIAN_POINT('Ctrl Pts',(20.4223379067786,67.8427447439344,25.));
#29834=CARTESIAN_POINT('Ctrl Pts',(20.4098305231907,67.844358118475,25.));
#29835=CARTESIAN_POINT('Ctrl Pts',(20.3973195611165,67.8458383045697,25.));
#29836=CARTESIAN_POINT('Ctrl Pts',(20.3294889065971,67.85386342614,25.));
#29837=CARTESIAN_POINT('Ctrl Pts',(20.2614347205481,67.857995328394,25.));
#29838=CARTESIAN_POINT('Ctrl Pts',(20.1934027269559,67.8580559708634,25.));
#29839=CARTESIAN_POINT('Ctrl Pts',(20.1836058007518,67.8580647036635,25.));
#29840=CARTESIAN_POINT('Ctrl Pts',(20.1738093409654,67.8579889211747,25.));
#29841=CARTESIAN_POINT('Ctrl Pts',(20.1640140908158,67.8578280017397,25.));
#29842=CARTESIAN_POINT('Ctrl Pts',(20.0946498528238,67.8566884643292,25.));
#29843=CARTESIAN_POINT('Ctrl Pts',(20.0253448166408,67.8512836465463,25.));
#29844=CARTESIAN_POINT('Ctrl Pts',(19.9564239887308,67.8417867762202,25.));
#29845=CARTESIAN_POINT('Ctrl Pts',(19.8921287237172,67.8329272802895,25.));
#29846=CARTESIAN_POINT('Ctrl Pts',(19.8281673125328,67.8205056461074,25.));
#29847=CARTESIAN_POINT('Ctrl Pts',(19.7648241284675,67.8046280687348,25.));
#29848=CARTESIAN_POINT('Ctrl Pts',(19.7509594847671,67.8011527626487,25.));
#29849=CARTESIAN_POINT('Ctrl Pts',(19.7371245581731,67.7975117747354,25.));
#29850=CARTESIAN_POINT('Ctrl Pts',(19.7233225085399,67.7937060404833,25.));
#29851=CARTESIAN_POINT('Ctrl Pts',(19.7122620885151,67.790656274655,25.));
#29852=CARTESIAN_POINT('Ctrl Pts',(19.7012233271795,67.7875007728397,25.));
#29853=CARTESIAN_POINT('Ctrl Pts',(19.6902209057537,67.7842441420852,25.));
#29854=CARTESIAN_POINT('Ctrl Pts',(19.624658693414,67.7648382396226,25.));
#29855=CARTESIAN_POINT('Ctrl Pts',(19.560262855601,67.7418123378998,25.));
#29856=CARTESIAN_POINT('Ctrl Pts',(19.4973358510903,67.7153484561744,25.));
#29857=CARTESIAN_POINT('Ctrl Pts',(19.4347002019695,67.6890071036341,25.));
#29858=CARTESIAN_POINT('Ctrl Pts',(19.3735189237464,67.6592588311679,25.));
#29859=CARTESIAN_POINT('Ctrl Pts',(19.3141200864186,67.6262415908821,25.));
#29860=CARTESIAN_POINT('Ctrl Pts',(19.2559939626492,67.5939317969245,25.));
#29861=CARTESIAN_POINT('Ctrl Pts',(19.199574042523,67.5584909174538,25.));
#29862=CARTESIAN_POINT('Ctrl Pts',(19.1452076937093,67.5200188262395,25.));
#29863=CARTESIAN_POINT('Ctrl Pts',(19.1337111877064,67.5118833778005,25.));
#29864=CARTESIAN_POINT('Ctrl Pts',(19.1223066761945,67.5036122974171,25.));
#29865=CARTESIAN_POINT('Ctrl Pts',(19.1109977221854,67.4952064007952,25.));
#29866=CARTESIAN_POINT('Ctrl Pts',(19.100366622277,67.4873043501958,25.));
#29867=CARTESIAN_POINT('Ctrl Pts',(19.0898187360985,67.4792820489923,25.));
#29868=CARTESIAN_POINT('Ctrl Pts',(19.0793736026688,67.4711534357938,25.));
#29869=CARTESIAN_POINT('Ctrl Pts',(19.0278061913906,67.4310226377767,25.));
#29870=CARTESIAN_POINT('Ctrl Pts',(18.9786453544672,67.3882343524051,25.));
#29871=CARTESIAN_POINT('Ctrl Pts',(18.9321821714341,67.3429205912564,25.));
#29872=CARTESIAN_POINT('Ctrl Pts',(18.886602631737,67.2984686135769,25.));
#29873=CARTESIAN_POINT('Ctrl Pts',(18.8436185304839,67.2515856441284,25.));
#29874=CARTESIAN_POINT('Ctrl Pts',(18.8035471707609,67.2023705436618,25.));
#29875=CARTESIAN_POINT('Ctrl Pts',(18.7647769323282,67.154753462715,25.));
#29876=CARTESIAN_POINT('Ctrl Pts',(18.7287330112329,67.1049526682313,25.));
#29877=CARTESIAN_POINT('Ctrl Pts',(18.6957494603037,67.0530423374834,25.));
#29878=CARTESIAN_POINT('Ctrl Pts',(18.6902971461602,67.0444613502168,25.));
#29879=CARTESIAN_POINT('Ctrl Pts',(18.684928570876,67.0358226946663,25.));
#29880=CARTESIAN_POINT('Ctrl Pts',(18.6796453811788,67.0271266799546,25.));
#29881=CARTESIAN_POINT('Ctrl Pts',(18.6739897987629,67.0178177149714,25.));
#29882=CARTESIAN_POINT('Ctrl Pts',(18.6684320638271,67.0084430187688,25.));
#29883=CARTESIAN_POINT('Ctrl Pts',(18.6629725798064,66.9990042518226,25.));
#29884=CARTESIAN_POINT('Origin',(20.,66.,37.5459252805377));
#29885=CARTESIAN_POINT('Ctrl Pts',(17.9434278899737,66.0014963127332,35.7959252805377));
#29886=CARTESIAN_POINT('Ctrl Pts',(17.9426109499923,66.0996692927701,35.7905876687522));
#29887=CARTESIAN_POINT('Ctrl Pts',(17.9936360748142,66.8783591116969,35.7482056843029));
#29888=CARTESIAN_POINT('Ctrl Pts',(18.9885906510386,68.2081813101826,35.6687793271897));
#29889=CARTESIAN_POINT('Ctrl Pts',(21.3064560191417,68.0471889261963,35.5576462091981));
#29890=CARTESIAN_POINT('Ctrl Pts',(22.4285781845706,66.0128601788243,35.4465130912066));
#29891=CARTESIAN_POINT('Ctrl Pts',(21.3279816597525,63.9665950349013,35.335379973215));
#29892=CARTESIAN_POINT('Ctrl Pts',(19.0119582073911,63.7814655261371,35.2242468552234));
#29893=CARTESIAN_POINT('Ctrl Pts',(17.9980259373779,65.1068137265861,35.144428624331));
#29894=CARTESIAN_POINT('Ctrl Pts',(17.9427193490685,65.892962776772,35.1016547661024));
#29895=CARTESIAN_POINT('Ctrl Pts',(17.9436249754829,65.9983937900349,35.0959252805377));
#29896=CARTESIAN_POINT('Ctrl Pts',(17.9473272485919,65.9976786215907,35.8540747194623));
#29897=CARTESIAN_POINT('Ctrl Pts',(17.9508754702579,66.467827503345,35.8286277343138));
#29898=CARTESIAN_POINT('Ctrl Pts',(18.3433678783681,67.6294026063953,35.7661363765015));
#29899=CARTESIAN_POINT('Ctrl Pts',(20.2718170903172,68.4128312567252,35.6666006460253));
#29900=CARTESIAN_POINT('Ctrl Pts',(22.1745315590613,67.0812974610511,35.5554675280338));
#29901=CARTESIAN_POINT('Ctrl Pts',(22.0878552063855,64.7590834656903,35.4443344100422));
#29902=CARTESIAN_POINT('Ctrl Pts',(20.0898773670193,63.5731233891133,35.3332012920506));
#29903=CARTESIAN_POINT('Ctrl Pts',(18.2789899846852,64.474160336193,35.2364480618574));
#29904=CARTESIAN_POINT('Ctrl Pts',(17.95008404285,65.581879078884,35.1767392043279));
#29905=CARTESIAN_POINT('Ctrl Pts',(17.9479090025127,66.0011644690241,35.1540747194623));
#29906=CARTESIAN_POINT('Ctrl Pts',(21.2690708798523,67.0793586530486,36.));
#29907=CARTESIAN_POINT('Ctrl Pts',(21.627967898288,66.6573805147569,35.9629556273362));
#29908=CARTESIAN_POINT('Ctrl Pts',(21.8852403009264,65.4342572368484,35.8888668820084));
#29909=CARTESIAN_POINT('Ctrl Pts',(20.5452623374803,64.1066463862456,35.7777337640169));
#29910=CARTESIAN_POINT('Ctrl Pts',(18.7059924808176,64.516301386891,35.6666006460253));
#29911=CARTESIAN_POINT('Ctrl Pts',(18.0511940983536,66.2817529495446,35.5554675280338));
#29912=CARTESIAN_POINT('Ctrl Pts',(19.1799450174622,67.7904027559382,35.4443344100422));
#29913=CARTESIAN_POINT('Ctrl Pts',(21.0592800719747,67.6598694493458,35.3332012920506));
#29914=CARTESIAN_POINT('Ctrl Pts',(21.9691014748727,66.0104270874417,35.2220681740591));
#29915=CARTESIAN_POINT('Ctrl Pts',(21.0767331525235,64.3513066446749,35.1109350560675));
#29916=CARTESIAN_POINT('Ctrl Pts',(19.1988915310931,64.2012028551135,34.999801938076));
#29917=CARTESIAN_POINT('Ctrl Pts',(18.0542582879001,65.6973951096712,34.8886688200844));
#29918=CARTESIAN_POINT('Ctrl Pts',(18.6904432516101,67.4705602726572,34.7775357020928));
#29919=CARTESIAN_POINT('Ctrl Pts',(20.5251866927185,67.8978022666667,34.6664025841013));
#29920=CARTESIAN_POINT('Ctrl Pts',(21.8792583017954,66.5881052056475,34.5552694661097));
#29921=CARTESIAN_POINT('Ctrl Pts',(21.5133588964881,64.7401489682993,34.4441363481182));
#29922=CARTESIAN_POINT('Ctrl Pts',(19.7623737885107,64.0452590579031,34.3330032301266));
#29923=CARTESIAN_POINT('Ctrl Pts',(18.2288735799674,65.1394244562081,34.2218701121351));
#29924=CARTESIAN_POINT('Ctrl Pts',(18.3163779629365,67.0212227346053,34.1107369941435));
#29925=CARTESIAN_POINT('Ctrl Pts',(19.9447995104512,67.9683576357047,33.9996038761519));
#29926=CARTESIAN_POINT('Ctrl Pts',(21.6237427139031,67.1139742228354,33.8884707581604));
#29927=CARTESIAN_POINT('Ctrl Pts',(21.8165726780916,65.2400377215117,33.7773376401688));
#29928=CARTESIAN_POINT('Ctrl Pts',(20.3468038264876,64.0616486263943,33.6662045221773));
#29929=CARTESIAN_POINT('Ctrl Pts',(18.559626463418,64.6573149925867,33.5550714041857));
#29930=CARTESIAN_POINT('Ctrl Pts',(18.0907356532766,66.4818595294338,33.4439382861942));
#29931=CARTESIAN_POINT('Ctrl Pts',(19.3692787213201,67.865387256979,33.3328051682026));
#29932=CARTESIAN_POINT('Ctrl Pts',(21.2250827284832,67.541639147092,33.221672050211));
#29933=CARTESIAN_POINT('Ctrl Pts',(21.9596428037902,65.8069222109183,33.1105389322195));
#29934=CARTESIAN_POINT('Ctrl Pts',(20.9006606542602,64.248917667052,32.9994058142279));
#29935=CARTESIAN_POINT('Ctrl Pts',(19.0173584243029,64.2935725960923,32.8882726962364));
#29936=CARTESIAN_POINT('Ctrl Pts',(18.0334084408143,65.9000170495854,32.7771395782448));
#29937=CARTESIAN_POINT('Ctrl Pts',(18.8493604565844,67.5979698345543,32.6660064602532));
#29938=CARTESIAN_POINT('Ctrl Pts',(20.7184230712183,67.8333977314765,32.5548733422617));
#29939=CARTESIAN_POINT('Ctrl Pts',(21.9299566142173,66.3908278627113,32.4437402242701));
#29940=CARTESIAN_POINT('Ctrl Pts',(21.3751179015322,64.5905569511623,32.3326071062786));
#29941=CARTESIAN_POINT('Ctrl Pts',(19.5617171612518,64.0802637930451,32.221473988287));
#29942=CARTESIAN_POINT('Ctrl Pts',(18.1494501256381,65.3269887716151,32.1103408702955));
#29943=CARTESIAN_POINT('Ctrl Pts',(18.4308791719737,67.1896801158661,31.9992077523038));
#29944=CARTESIAN_POINT('Ctrl Pts',(20.1484293601129,67.9635293927237,31.8880746343123));
#29945=CARTESIAN_POINT('Ctrl Pts',(21.7301311557542,66.9402792855966,31.7769415163207));
#29946=CARTESIAN_POINT('Ctrl Pts',(21.7283488203504,65.0564485672595,31.6658083983292));
#29947=CARTESIAN_POINT('Ctrl Pts',(20.1447136174153,64.0361932579889,31.5546752803376));
#29948=CARTESIAN_POINT('Ctrl Pts',(18.4286308159493,64.8132911736871,31.4435421623461));
#29949=CARTESIAN_POINT('Ctrl Pts',(18.1507269402148,66.6765117156309,31.3324090443545));
#29950=CARTESIAN_POINT('Ctrl Pts',(19.5653505554741,67.9205621081879,31.221275926363));
#29951=CARTESIAN_POINT('Ctrl Pts',(21.3777824499989,67.4068384667431,31.1101428083714));
#29952=CARTESIAN_POINT('Ctrl Pts',(21.929213617296,65.6055208879127,30.9990096903798));
#29953=CARTESIAN_POINT('Ctrl Pts',(20.7149525489356,64.1652461190112,30.8878765723883));
#29954=CARTESIAN_POINT('Ctrl Pts',(18.8463387675313,64.4042103171995,30.7767434543967));
#29955=CARTESIAN_POINT('Ctrl Pts',(18.033601153746,66.103704042757,30.6656103364052));
#29956=CARTESIAN_POINT('Ctrl Pts',(19.0205891607567,67.7082837466316,30.5544772184136));
#29957=CARTESIAN_POINT('Ctrl Pts',(20.9039725170779,67.7493749281961,30.4433441004221));
#29958=CARTESIAN_POINT('Ctrl Pts',(21.9600046457578,66.1893693207493,30.3322109824305));
#29959=CARTESIAN_POINT('Ctrl Pts',(21.2221633776091,64.4560454574488,30.2210778644389));
#29960=CARTESIAN_POINT('Ctrl Pts',(19.3657500823907,64.1358095609499,30.1099447464474));
#29961=CARTESIAN_POINT('Ctrl Pts',(18.0898272756019,65.5217541280903,29.9988116284558));
#29962=CARTESIAN_POINT('Ctrl Pts',(18.5621697298479,67.3454081407765,29.8876785104642));
#29963=CARTESIAN_POINT('Ctrl Pts',(20.3504710397852,67.9376916682758,29.7765453924727));
#29964=CARTESIAN_POINT('Ctrl Pts',(21.8180074597053,66.7565235141681,29.6654122744811));
#29965=CARTESIAN_POINT('Ctrl Pts',(21.6216318964268,64.8829552634185,29.5542791564896));
#29966=CARTESIAN_POINT('Ctrl Pts',(19.941074994729,64.0317503220406,29.443146038498));
#29967=CARTESIAN_POINT('Ctrl Pts',(18.3144485771209,64.9819649554836,29.3320129205065));
#29968=CARTESIAN_POINT('Ctrl Pts',(18.2305051643892,66.863925331137,29.2208798025149));
#29969=CARTESIAN_POINT('Ctrl Pts',(19.7660730718466,67.9551872399639,29.1097466845233));
#29970=CARTESIAN_POINT('Ctrl Pts',(21.5157401112242,67.2569848313562,28.9986135665318));
#29971=CARTESIAN_POINT('Ctrl Pts',(21.87814214186,65.4083404306503,28.8874804485402));
#29972=CARTESIAN_POINT('Ctrl Pts',(20.5215945613111,64.101206155307,28.7763473305487));
#29973=CARTESIAN_POINT('Ctrl Pts',(18.6876631084887,64.5319227424242,28.6652142125571));
#29974=CARTESIAN_POINT('Ctrl Pts',(18.0548340318536,66.3062814186326,28.5540810945655));
#29975=CARTESIAN_POINT('Ctrl Pts',(19.2022974102536,67.800319285389,28.442947976574));
#29976=CARTESIAN_POINT('Ctrl Pts',(21.0798495960555,67.6466340822816,28.3318148585824));
#29977=CARTESIAN_POINT('Ctrl Pts',(21.9690809290854,65.9858845561824,28.2206817405909));
#29978=CARTESIAN_POINT('Ctrl Pts',(21.0561318935384,64.3380540398472,28.1095486225993));
#29979=CARTESIAN_POINT('Ctrl Pts',(19.1765693800943,64.2113018797919,27.9984155046077));
#29980=CARTESIAN_POINT('Ctrl Pts',(18.0506429798704,65.721636641838,27.8872823866162));
#29981=CARTESIAN_POINT('Ctrl Pts',(18.7088448504754,67.4867405055191,27.7761492686246));
#29982=CARTESIAN_POINT('Ctrl Pts',(20.5487627331737,67.8911209410725,27.665016150633));
#29983=CARTESIAN_POINT('Ctrl Pts',(21.8864313636263,66.5646730574428,27.5538830326415));
#29984=CARTESIAN_POINT('Ctrl Pts',(21.4975637603834,64.7214141665632,27.4427499146499));
#29985=CARTESIAN_POINT('Ctrl Pts',(19.738066861079,64.0483673546206,27.3316167966584));
#29986=CARTESIAN_POINT('Ctrl Pts',(18.2183014781556,65.1615315561838,27.2204836786668));
#29987=CARTESIAN_POINT('Ctrl Pts',(18.3292167132778,67.0420950774451,27.1093505606753));
#29988=CARTESIAN_POINT('Ctrl Pts',(19.9692985660544,67.9688921711125,26.9982174426838));
#29989=CARTESIAN_POINT('Ctrl Pts',(21.6374795950145,67.093681647467,26.8870843246921));
#29990=CARTESIAN_POINT('Ctrl Pts',(21.8069748172614,65.2174906480645,26.7759512067006));
#29991=CARTESIAN_POINT('Ctrl Pts',(20.3226556263046,64.0574829771209,26.664818088709));
#29992=CARTESIAN_POINT('Ctrl Pts',(18.5430291841408,64.6753434014641,26.5536849707175));
#29993=CARTESIAN_POINT('Ctrl Pts',(18.0968800225525,66.5055815646723,26.4425518527259));
#29994=CARTESIAN_POINT('Ctrl Pts',(19.3925406836826,67.8730918158693,26.3314187347344));
#29995=CARTESIAN_POINT('Ctrl Pts',(21.2441729909822,67.5262742434723,26.2202856167428));
#29996=CARTESIAN_POINT('Ctrl Pts',(21.957087271561,65.7825513461355,26.1091524987512));
#29997=CARTESIAN_POINT('Ctrl Pts',(20.8788021098056,64.2378441486145,25.9980193807597));
#29998=CARTESIAN_POINT('Ctrl Pts',(18.9961949733702,64.3059350666609,25.8868862627681));
#29999=CARTESIAN_POINT('Ctrl Pts',(18.0323250495028,65.9244934665604,25.7757531447766));
#30000=CARTESIAN_POINT('Ctrl Pts',(18.8693180936086,67.6121732190418,25.664620026785));
#30001=CARTESIAN_POINT('Ctrl Pts',(20.7412167255774,67.8242990731299,25.5534869087934));
#30002=CARTESIAN_POINT('Ctrl Pts',(21.9346029937715,66.3668134624633,25.4423537908019));
#30003=CARTESIAN_POINT('Ctrl Pts',(21.3576070175663,64.573488384656,25.3312206728103));
#30004=CARTESIAN_POINT('Ctrl Pts',(19.5375919330654,64.0859968791816,25.2200875548188));
#30005=CARTESIAN_POINT('Ctrl Pts',(18.141756289785,65.3498097603869,25.1089544368272));
#30006=CARTESIAN_POINT('Ctrl Pts',(18.4447228010167,67.2096329020469,24.9978213188356));
#30007=CARTESIAN_POINT('Ctrl Pts',(20.1751283187016,67.960491249224,24.8866882008441));
#30008=CARTESIAN_POINT('Ctrl Pts',(21.2151340020224,67.2672324081111,24.8125994555164));
#30009=CARTESIAN_POINT('Ctrl Pts',(21.4735782273626,66.7772536316049,24.7755550828525));
#30010=CARTESIAN_POINT('Ctrl Pts',(21.3677806246587,67.1633123698099,36.0748149723825));
#30011=CARTESIAN_POINT('Ctrl Pts',(21.7545930524415,66.7085123024943,36.0377705997186));
#30012=CARTESIAN_POINT('Ctrl Pts',(22.0318763887585,65.3902531353729,35.9636818543909));
#30013=CARTESIAN_POINT('Ctrl Pts',(20.5876734486638,63.9593792359159,35.8525487363994));
#30014=CARTESIAN_POINT('Ctrl Pts',(18.6053431364634,64.4008976582304,35.7414156184077));
#30015=CARTESIAN_POINT('Ctrl Pts',(17.8996138073842,66.3036680073947,35.6302825004163));
#30016=CARTESIAN_POINT('Ctrl Pts',(19.1161602286543,67.9296622740197,35.5191493824247));
#30017=CARTESIAN_POINT('Ctrl Pts',(21.1416720543637,67.7889759416293,35.4080162644332));
#30018=CARTESIAN_POINT('Ctrl Pts',(22.1222603781053,66.0112381179025,35.2968831464416));
#30019=CARTESIAN_POINT('Ctrl Pts',(21.1604826549332,64.2230694414171,35.18575002845));
#30020=CARTESIAN_POINT('Ctrl Pts',(19.1365804231924,64.0612904121213,35.0746169104584));
#30021=CARTESIAN_POINT('Ctrl Pts',(17.9029163330024,65.6738581646702,34.9634837924669));
#30022=CARTESIAN_POINT('Ctrl Pts',(18.5885844709106,67.5849420865818,34.8523506744753));
#30023=CARTESIAN_POINT('Ctrl Pts',(20.5660362979194,68.0454154381686,34.7412175564838));
#30024=CARTESIAN_POINT('Ctrl Pts',(22.0254291030805,66.6338486827774,34.6300844384922));
#30025=CARTESIAN_POINT('Ctrl Pts',(21.6310696349854,64.6421563535386,34.5189513205007));
#30026=CARTESIAN_POINT('Ctrl Pts',(19.743890957435,63.8932171328852,34.4078182025091));
#30027=CARTESIAN_POINT('Ctrl Pts',(18.0911133967366,65.0724879330689,34.2966850845175));
#30028=CARTESIAN_POINT('Ctrl Pts',(18.1854239679567,67.1006545749571,34.185551966526));
#30029=CARTESIAN_POINT('Ctrl Pts',(19.9405059549666,68.1214586822994,34.0744188485344));
#30030=CARTESIAN_POINT('Ctrl Pts',(21.7500392285148,67.2006203771226,33.9632857305429));
#30031=CARTESIAN_POINT('Ctrl Pts',(21.9578677218307,65.1809270100747,33.8521526125513));
#30032=CARTESIAN_POINT('Ctrl Pts',(20.373778613912,63.910881500246,33.7410194945598));
#30033=CARTESIAN_POINT('Ctrl Pts',(18.4475926074063,64.5528794590469,33.6298863765682));
#30034=CARTESIAN_POINT('Ctrl Pts',(17.9422309484369,66.5193390996755,33.5187532585767));
#30035=CARTESIAN_POINT('Ctrl Pts',(19.3202205186216,68.0104791529674,33.4076201405851));
#30036=CARTESIAN_POINT('Ctrl Pts',(21.3203710259418,67.6615495549417,33.2964870225935));
#30037=CARTESIAN_POINT('Ctrl Pts',(22.1120660010638,65.7919044056951,33.185353904602));
#30038=CARTESIAN_POINT('Ctrl Pts',(20.970715041884,64.1127165352126,33.0742207866104));
#30039=CARTESIAN_POINT('Ctrl Pts',(18.9409274694105,64.1608447743097,32.9630876686188));
#30040=CARTESIAN_POINT('Ctrl Pts',(17.8804447616159,65.8922402644766,32.8519545506273));
#30041=CARTESIAN_POINT('Ctrl Pts',(18.7598624328743,67.7222617059394,32.7408214326357));
#30042=CARTESIAN_POINT('Ctrl Pts',(20.7743028169038,67.9760014465848,32.6296883146442));
#30043=CARTESIAN_POINT('Ctrl Pts',(22.0800707866417,66.4212268886475,32.5185551966526));
#30044=CARTESIAN_POINT('Ctrl Pts',(21.4820761016564,64.4809289028958,32.4074220786611));
#30045=CARTESIAN_POINT('Ctrl Pts',(19.5276270344884,63.9309445752673,32.2962889606694));
#30046=CARTESIAN_POINT('Ctrl Pts',(18.0055122977753,65.2746412095833,32.185155842678));
#30047=CARTESIAN_POINT('Ctrl Pts',(18.3088312084093,67.2822147587319,32.0740227246863));
#30048=CARTESIAN_POINT('Ctrl Pts',(20.159974360862,68.1162548932082,31.9628896066948));
#30049=CARTESIAN_POINT('Ctrl Pts',(21.8647026817244,67.0134152544393,31.8517564887032));
#30050=CARTESIAN_POINT('Ctrl Pts',(21.8627817142903,64.983058087172,31.7406233707117));
#30051=CARTESIAN_POINT('Ctrl Pts',(20.1559696035638,63.8834461849685,31.6294902527201));
#30052=CARTESIAN_POINT('Ctrl Pts',(18.306407972752,64.7209876410282,31.5183571347286));
#30053=CARTESIAN_POINT('Ctrl Pts',(18.0068884244102,66.7291315494549,31.407224016737));
#30054=CARTESIAN_POINT('Ctrl Pts',(19.5315430381553,68.0699455654823,31.2960908987455));
#30055=CARTESIAN_POINT('Ctrl Pts',(21.484947901667,67.5162639277168,31.1849577807539));
#30056=CARTESIAN_POINT('Ctrl Pts',(22.0792699985932,65.5748378637382,31.0738246627623));
#30057=CARTESIAN_POINT('Ctrl Pts',(20.7705623535372,64.0225369210851,30.9626915447707));
#30058=CARTESIAN_POINT('Ctrl Pts',(18.7566057134853,64.2800880204431,30.8515584267792));
#30059=CARTESIAN_POINT('Ctrl Pts',(17.8806524639738,66.1117702585676,30.7404253087876));
#30060=CARTESIAN_POINT('Ctrl Pts',(18.9444094961397,67.8411559568164,30.6292921907961));
#30061=CARTESIAN_POINT('Ctrl Pts',(20.9742845050759,67.8854432561946,30.5181590728045));
#30062=CARTESIAN_POINT('Ctrl Pts',(22.1124559875022,66.2040986771801,30.407025954813));
#30063=CARTESIAN_POINT('Ctrl Pts',(21.3172246047091,64.3359549555647,30.2958928368214));
#30064=CARTESIAN_POINT('Ctrl Pts',(19.316417418231,63.9908107547912,30.1847597188299));
#30065=CARTESIAN_POINT('Ctrl Pts',(17.9412519161361,65.4845556321509,30.0736266008383));
#30066=CARTESIAN_POINT('Ctrl Pts',(18.4503336919285,67.4500554826586,29.9624934828468));
#30067=CARTESIAN_POINT('Ctrl Pts',(20.3777310671394,68.0884074818096,29.8513603648552));
#30068=CARTESIAN_POINT('Ctrl Pts',(21.9594141023544,66.8153667546909,29.7402272468636));
#30069=CARTESIAN_POINT('Ctrl Pts',(21.7477642293072,64.7960702811563,29.6290941288721));
#30070=CARTESIAN_POINT('Ctrl Pts',(19.9364917422682,63.8786576725195,29.5179610108805));
#30071=CARTESIAN_POINT('Ctrl Pts',(18.1833445123661,64.9027810572131,29.4068278928889));
#30072=CARTESIAN_POINT('Ctrl Pts',(18.0928718876097,66.9311224044622,29.2956947748974));
#30073=CARTESIAN_POINT('Ctrl Pts',(19.747877975144,68.1072638785266,29.1845616569058));
#30074=CARTESIAN_POINT('Ctrl Pts',(21.6336360632527,67.3547545098655,29.0734285389143));
#30075=CARTESIAN_POINT('Ctrl Pts',(22.0242261269836,65.3623204911576,28.9622954209227));
#30076=CARTESIAN_POINT('Ctrl Pts',(20.5621647665351,63.9535158577631,28.8511623029311));
#30077=CARTESIAN_POINT('Ctrl Pts',(18.5855880851643,64.4177340601748,28.7400291849396));
#30078=CARTESIAN_POINT('Ctrl Pts',(17.9035368589611,66.3301043280951,28.628896066948));
#30079=CARTESIAN_POINT('Ctrl Pts',(19.1402512154229,67.9403501221627,28.5177629489565));
#30080=CARTESIAN_POINT('Ctrl Pts',(21.1638414989099,67.7747111129913,28.4066298309649));
#30081=CARTESIAN_POINT('Ctrl Pts',(22.1222382342439,65.9847866412596,28.2954967129734));
#30082=CARTESIAN_POINT('Ctrl Pts',(21.1382790071064,64.208786034243,28.1843635949818));
#30083=CARTESIAN_POINT('Ctrl Pts',(19.1125220304568,64.0721749501739,28.0732304769902));
#30084=CARTESIAN_POINT('Ctrl Pts',(17.8990198222922,65.6999852301763,27.9620973589987));
#30085=CARTESIAN_POINT('Ctrl Pts',(18.6084173666064,67.6023808359554,27.8509642410071));
#30086=CARTESIAN_POINT('Ctrl Pts',(20.5914461090282,68.0382144316372,27.7398311230155));
#30087=CARTESIAN_POINT('Ctrl Pts',(22.0331600936403,66.6085939560183,27.6286980050241));
#30088=CARTESIAN_POINT('Ctrl Pts',(21.6140459356233,64.6219643380822,27.5175648870324));
#30089=CARTESIAN_POINT('Ctrl Pts',(19.7176934101476,63.8965671963791,27.4064317690409));
#30090=CARTESIAN_POINT('Ctrl Pts',(18.079718985085,65.0963145478738,27.2952986510493));
#30091=CARTESIAN_POINT('Ctrl Pts',(18.199261330582,67.1231503918422,27.1841655330577));
#30092=CARTESIAN_POINT('Ctrl Pts',(19.9669105743685,68.1220347944658,27.0730324150662));
#30093=CARTESIAN_POINT('Ctrl Pts',(21.7648445795207,67.1787494226676,26.9618992970746));
#30094=CARTESIAN_POINT('Ctrl Pts',(21.9475233287081,65.1566262001724,26.8507661790831));
#30095=CARTESIAN_POINT('Ctrl Pts',(20.3477521398551,63.9063918421381,26.7396330610915));
#30096=CARTESIAN_POINT('Ctrl Pts',(18.4297043732834,64.5723101376224,26.6284999431));
#30097=CARTESIAN_POINT('Ctrl Pts',(17.9488532335904,66.5449062612042,26.5173668251084));
#30098=CARTESIAN_POINT('Ctrl Pts',(19.3452918222943,68.0187829810191,26.4062337071169));
#30099=CARTESIAN_POINT('Ctrl Pts',(21.3409461502948,67.6449895520258,26.2951005891253));
#30100=CARTESIAN_POINT('Ctrl Pts',(22.109311696695,65.7656379479381,26.1839674711337));
#30101=CARTESIAN_POINT('Ctrl Pts',(20.9471563155252,64.1007817061923,26.0728343531422));
#30102=CARTESIAN_POINT('Ctrl Pts',(18.9181179017211,64.1741688115918,25.9617012351506));
#30103=CARTESIAN_POINT('Ctrl Pts',(17.879277102923,65.9186204843926,25.850568117159));
#30104=CARTESIAN_POINT('Ctrl Pts',(18.781372397108,67.7375698454729,25.7394349991675));
#30105=CARTESIAN_POINT('Ctrl Pts',(20.7988693870556,67.9661950844702,25.6283018811759));
#30106=CARTESIAN_POINT('Ctrl Pts',(22.0850785667664,66.3953446216335,25.5171687631844));
#30107=CARTESIAN_POINT('Ctrl Pts',(21.4632032016557,64.4625327242989,25.4060356451928));
#30108=CARTESIAN_POINT('Ctrl Pts',(19.5016253192157,63.9371235872212,25.2949025272012));
#30109=CARTESIAN_POINT('Ctrl Pts',(17.9972200268106,65.299237240249,25.1837694092097));
#30110=CARTESIAN_POINT('Ctrl Pts',(18.3237516103194,67.3037194948181,25.0726362912181));
#30111=CARTESIAN_POINT('Ctrl Pts',(20.1887499941509,68.1129804395273,24.9615031732266));
#30112=CARTESIAN_POINT('Ctrl Pts',(21.3096484764694,67.3657991545403,24.8874144278989));
#30113=CARTESIAN_POINT('Ctrl Pts',(21.5881947811615,66.837709283723,24.850370055235));
#30114=CARTESIAN_POINT('Ctrl Pts',(21.4664903694652,67.2472660865711,36.149629944765));
#30115=CARTESIAN_POINT('Ctrl Pts',(21.8812182065951,66.7596440902318,36.1125855721011));
#30116=CARTESIAN_POINT('Ctrl Pts',(22.1785124765907,65.3462490338972,36.0384968267734));
#30117=CARTESIAN_POINT('Ctrl Pts',(20.6300845598474,63.8121120855864,35.9273637087819));
#30118=CARTESIAN_POINT('Ctrl Pts',(18.5046937921093,64.2854939295697,35.8162305907903));
#30119=CARTESIAN_POINT('Ctrl Pts',(17.7480335164148,66.325583065245,35.7050974727988));
#30120=CARTESIAN_POINT('Ctrl Pts',(19.0523754398465,68.0689217921011,35.5939643548072));
#30121=CARTESIAN_POINT('Ctrl Pts',(21.2240640367527,67.9180824339128,35.4828312368156));
#30122=CARTESIAN_POINT('Ctrl Pts',(22.275419281338,66.0120491483635,35.3716981188241));
#30123=CARTESIAN_POINT('Ctrl Pts',(21.2442321573429,64.0948322381591,35.2605650008325));
#30124=CARTESIAN_POINT('Ctrl Pts',(19.0742693152918,63.9213779691293,35.149431882841));
#30125=CARTESIAN_POINT('Ctrl Pts',(17.7515743781046,65.650321219669,35.0382987648494));
#30126=CARTESIAN_POINT('Ctrl Pts',(18.486725690211,67.6993239005066,34.9271656468578));
#30127=CARTESIAN_POINT('Ctrl Pts',(20.6068859031203,68.1930286096704,34.8160325288663));
#30128=CARTESIAN_POINT('Ctrl Pts',(22.1715999043656,66.6795921599075,34.7048994108747));
#30129=CARTESIAN_POINT('Ctrl Pts',(21.7487803734828,64.5441637387779,34.5937662928832));
#30130=CARTESIAN_POINT('Ctrl Pts',(19.7254081263593,63.7411752078672,34.4826331748916));
#30131=CARTESIAN_POINT('Ctrl Pts',(17.9533532135058,65.0055514099299,34.3715000569001));
#30132=CARTESIAN_POINT('Ctrl Pts',(18.0544699729771,67.1800864153088,34.2603669389085));
#30133=CARTESIAN_POINT('Ctrl Pts',(19.936212399482,68.274559728894,34.1492338209169));
#30134=CARTESIAN_POINT('Ctrl Pts',(21.8763357431267,67.2872665314098,34.0381007029254));
#30135=CARTESIAN_POINT('Ctrl Pts',(22.0991627655698,65.1218162986378,33.9269675849338));
#30136=CARTESIAN_POINT('Ctrl Pts',(20.4007534013364,63.7601143740976,33.8158344669422));
#30137=CARTESIAN_POINT('Ctrl Pts',(18.3355587513947,64.4484439255071,33.7047013489507));
#30138=CARTESIAN_POINT('Ctrl Pts',(17.7937262435972,66.556818669917,33.5935682309591));
#30139=CARTESIAN_POINT('Ctrl Pts',(19.2711623159232,68.1555710489559,33.4824351129676));
#30140=CARTESIAN_POINT('Ctrl Pts',(21.4156593234003,67.7814599627911,33.371301994976));
#30141=CARTESIAN_POINT('Ctrl Pts',(22.2644891983374,65.776886600472,33.2601688769844));
#30142=CARTESIAN_POINT('Ctrl Pts',(21.0407694295078,63.9765154033731,33.1490357589929));
#30143=CARTESIAN_POINT('Ctrl Pts',(18.8644965145181,64.0281169525272,33.0379026410013));
#30144=CARTESIAN_POINT('Ctrl Pts',(17.7274810824176,65.8844634793678,32.9267695230098));
#30145=CARTESIAN_POINT('Ctrl Pts',(18.6703644091643,67.8465535773246,32.8156364050182));
#30146=CARTESIAN_POINT('Ctrl Pts',(20.8301825625893,68.1186051616932,32.7045032870267));
#30147=CARTESIAN_POINT('Ctrl Pts',(22.2301849590661,66.4516259145837,32.5933701690351));
#30148=CARTESIAN_POINT('Ctrl Pts',(21.5890343017806,64.3713008546293,32.4822370510436));
#30149=CARTESIAN_POINT('Ctrl Pts',(19.493536907725,63.7816253574895,32.371103933052));
#30150=CARTESIAN_POINT('Ctrl Pts',(17.8615744699125,65.2222936475516,32.2599708150604));
#30151=CARTESIAN_POINT('Ctrl Pts',(18.1867832448448,67.3747494015975,32.1488376970689));
#30152=CARTESIAN_POINT('Ctrl Pts',(20.1715193616111,68.2689803936927,32.0377045790773));
#30153=CARTESIAN_POINT('Ctrl Pts',(21.9992742076947,67.086551223282,31.9265714610857));
#30154=CARTESIAN_POINT('Ctrl Pts',(21.9972146082301,64.9096676070843,31.8154383430942));
#30155=CARTESIAN_POINT('Ctrl Pts',(20.1672255897123,63.7306991119479,31.7043052251026));
#30156=CARTESIAN_POINT('Ctrl Pts',(18.1841851295548,64.6286841083692,31.5931721071111));
#30157=CARTESIAN_POINT('Ctrl Pts',(17.8630499086056,66.7817513832787,31.4820389891195));
#30158=CARTESIAN_POINT('Ctrl Pts',(19.4977355208365,68.2193290227768,31.3709058711279));
#30159=CARTESIAN_POINT('Ctrl Pts',(21.5921133533351,67.6256893886905,31.2597727531364));
#30160=CARTESIAN_POINT('Ctrl Pts',(22.2293263798905,65.5441548395638,31.1486396351448));
#30161=CARTESIAN_POINT('Ctrl Pts',(20.8261721581388,63.879827723159,31.0375065171533));
#30162=CARTESIAN_POINT('Ctrl Pts',(18.6668726594392,64.1559657236867,30.9263733991617));
#30163=CARTESIAN_POINT('Ctrl Pts',(17.7277037742016,66.1198364743782,30.8152402811701));
#30164=CARTESIAN_POINT('Ctrl Pts',(18.8682298315227,67.9740281670011,30.7041071631786));
#30165=CARTESIAN_POINT('Ctrl Pts',(21.0445964930739,68.021511584193,30.592974045187));
#30166=CARTESIAN_POINT('Ctrl Pts',(22.2649073292466,66.2188280336109,30.4818409271955));
#30167=CARTESIAN_POINT('Ctrl Pts',(21.412285831809,64.2158644536806,30.3707078092039));
#30168=CARTESIAN_POINT('Ctrl Pts',(19.2670847540712,63.8458119486327,30.2595746912124));
#30169=CARTESIAN_POINT('Ctrl Pts',(17.7926765566704,65.4473571362115,30.1484415732208));
#30170=CARTESIAN_POINT('Ctrl Pts',(18.338497654009,67.5547028245408,30.0373084552292));
#30171=CARTESIAN_POINT('Ctrl Pts',(20.4049910944936,68.2391232953435,29.9261753372377));
#30172=CARTESIAN_POINT('Ctrl Pts',(22.1008207450036,66.8742099952136,29.8150422192461));
#30173=CARTESIAN_POINT('Ctrl Pts',(21.8738965621875,64.7091852988942,29.7039091012546));
#30174=CARTESIAN_POINT('Ctrl Pts',(19.9319084898074,63.7255650229983,29.592775983263));
#30175=CARTESIAN_POINT('Ctrl Pts',(18.0522404476114,64.8235971589427,29.4816428652714));
#30176=CARTESIAN_POINT('Ctrl Pts',(17.9552386108303,66.9983194777874,29.3705097472799));
#30177=CARTESIAN_POINT('Ctrl Pts',(19.7296828784414,68.2593405170892,29.2593766292883));
#30178=CARTESIAN_POINT('Ctrl Pts',(21.7515320152811,67.4525241883749,29.1482435112968));
#30179=CARTESIAN_POINT('Ctrl Pts',(22.1703101121073,65.3163005516648,29.0371103933052));
#30180=CARTESIAN_POINT('Ctrl Pts',(20.6027349717591,63.8058255602192,28.9259772753137));
#30181=CARTESIAN_POINT('Ctrl Pts',(18.48351306184,64.3035453779253,28.8148441573221));
#30182=CARTESIAN_POINT('Ctrl Pts',(17.7522396860685,66.3539272375576,28.7037110393305));
#30183=CARTESIAN_POINT('Ctrl Pts',(19.0782050205922,68.0803809589363,28.592577921339));
#30184=CARTESIAN_POINT('Ctrl Pts',(21.2478334017644,67.902788143701,28.4814448033474));
#30185=CARTESIAN_POINT('Ctrl Pts',(22.2753955394023,65.9836887263368,28.3703116853558));
#30186=CARTESIAN_POINT('Ctrl Pts',(21.2204261206745,64.0795180286389,28.2591785673643));
#30187=CARTESIAN_POINT('Ctrl Pts',(19.0484746808193,63.9330480205558,28.1480454493727));
#30188=CARTESIAN_POINT('Ctrl Pts',(17.7473966647141,65.6783338185146,28.0369123313811));
#30189=CARTESIAN_POINT('Ctrl Pts',(18.5079898827373,67.7180211663916,27.9257792133896));
#30190=CARTESIAN_POINT('Ctrl Pts',(20.6341294848828,68.1853079222018,27.814646095398));
#30191=CARTESIAN_POINT('Ctrl Pts',(22.1798888236542,66.6525148545939,27.7035129774065));
#30192=CARTESIAN_POINT('Ctrl Pts',(21.7305281108632,64.5225145096011,27.5923798594149));
#30193=CARTESIAN_POINT('Ctrl Pts',(19.6973199592161,63.7447670381374,27.4812467414234));
#30194=CARTESIAN_POINT('Ctrl Pts',(17.9411364920144,65.0310975395638,27.3701136234318));
#30195=CARTESIAN_POINT('Ctrl Pts',(18.0693059478863,67.2042057062393,27.2589805054402));
#30196=CARTESIAN_POINT('Ctrl Pts',(19.9645225826826,68.2751774178192,27.1478473874487));
#30197=CARTESIAN_POINT('Ctrl Pts',(21.8922095640269,67.2638171978682,27.0367142694571));
#30198=CARTESIAN_POINT('Ctrl Pts',(22.0880718401547,65.0957617522804,26.9255811514656));
#30199=CARTESIAN_POINT('Ctrl Pts',(20.3728486534058,63.7553007071551,26.814448033474));
#30200=CARTESIAN_POINT('Ctrl Pts',(18.3163795624261,64.4692768737807,26.7033149154825));
#30201=CARTESIAN_POINT('Ctrl Pts',(17.8008264446283,66.5842309577361,26.5921817974909));
#30202=CARTESIAN_POINT('Ctrl Pts',(19.2980429609061,68.164474146169,26.4810486794993));
#30203=CARTESIAN_POINT('Ctrl Pts',(21.4377193096073,67.7637048605792,26.3699155615078));
#30204=CARTESIAN_POINT('Ctrl Pts',(22.2615361218289,65.7487245497409,26.2587824435162));
#30205=CARTESIAN_POINT('Ctrl Pts',(21.0155105212449,63.9637192637702,26.1476493255247));
#30206=CARTESIAN_POINT('Ctrl Pts',(18.8400408300719,64.0424025565226,26.0365162075331));
#30207=CARTESIAN_POINT('Ctrl Pts',(17.7262291563432,65.9127475022248,25.9253830895415));
#30208=CARTESIAN_POINT('Ctrl Pts',(18.6934267006075,67.8629664719039,25.81424997155));
#30209=CARTESIAN_POINT('Ctrl Pts',(20.8565220485339,68.1080910958107,25.7031168535584));
#30210=CARTESIAN_POINT('Ctrl Pts',(22.2355541397614,66.4238757808037,25.5919837355669));
#30211=CARTESIAN_POINT('Ctrl Pts',(21.5687993857451,64.3515770639418,25.4808506175753));
#30212=CARTESIAN_POINT('Ctrl Pts',(19.465658705366,63.7882502952606,25.3697174995837));
#30213=CARTESIAN_POINT('Ctrl Pts',(17.8526837638362,65.2486647201112,25.2585843815922));
#30214=CARTESIAN_POINT('Ctrl Pts',(18.2027804196222,67.3978060875893,25.1474512636006));
#30215=CARTESIAN_POINT('Ctrl Pts',(20.2023716696001,68.2654696298307,25.0363181456091));
#30216=CARTESIAN_POINT('Ctrl Pts',(21.4041629509165,67.4643659009696,24.9622294002814));
#30217=CARTESIAN_POINT('Ctrl Pts',(21.7028113349605,66.8981649358412,24.9251850276175));
#30218=CARTESIAN_POINT('Ctrl Pts',(21.5652001142716,67.3312198033323,36.2244449171475));
#30219=CARTESIAN_POINT('Ctrl Pts',(22.0078433607486,66.8107758779692,36.1874005444836));
#30220=CARTESIAN_POINT('Ctrl Pts',(22.3251485644228,65.3022449324216,36.1133117991559));
#30221=CARTESIAN_POINT('Ctrl Pts',(20.672495671031,63.6648449352568,36.0021786811644));
#30222=CARTESIAN_POINT('Ctrl Pts',(18.4040444477551,64.1700902009091,35.8910455631728));
#30223=CARTESIAN_POINT('Ctrl Pts',(17.5964532254454,66.3474981230952,35.7799124451812));
#30224=CARTESIAN_POINT('Ctrl Pts',(18.9885906510386,68.2081813101826,35.6687793271897));
#30225=CARTESIAN_POINT('Ctrl Pts',(21.3064560191417,68.0471889261963,35.5576462091981));
#30226=CARTESIAN_POINT('Ctrl Pts',(22.4285781845706,66.0128601788243,35.4465130912066));
#30227=CARTESIAN_POINT('Ctrl Pts',(21.3279816597525,63.9665950349013,35.335379973215));
#30228=CARTESIAN_POINT('Ctrl Pts',(19.0119582073911,63.7814655261371,35.2242468552234));
#30229=CARTESIAN_POINT('Ctrl Pts',(17.6002324232069,65.626784274668,35.1131137372319));
#30230=CARTESIAN_POINT('Ctrl Pts',(18.3848669095114,67.8137057144312,35.0019806192403));
#30231=CARTESIAN_POINT('Ctrl Pts',(20.6477355083213,68.3406417811724,34.8908475012488));
#30232=CARTESIAN_POINT('Ctrl Pts',(22.3177707056507,66.7253356370374,34.7797143832572));
#30233=CARTESIAN_POINT('Ctrl Pts',(21.8664911119801,64.4461711240172,34.6685812652656));
#30234=CARTESIAN_POINT('Ctrl Pts',(19.7069252952836,63.5891332828492,34.5574481472741));
#30235=CARTESIAN_POINT('Ctrl Pts',(17.8155930302749,64.9386148867908,34.4463150292825));
#30236=CARTESIAN_POINT('Ctrl Pts',(17.9235159779974,67.2595182556605,34.335181911291));
#30237=CARTESIAN_POINT('Ctrl Pts',(19.9319188439973,68.4276607754887,34.2240487932994));
#30238=CARTESIAN_POINT('Ctrl Pts',(22.0026322577385,67.3739126856969,34.1129156753079));
#30239=CARTESIAN_POINT('Ctrl Pts',(22.2404578093089,65.0627055872007,34.0017825573163));
#30240=CARTESIAN_POINT('Ctrl Pts',(20.4277281887608,63.6093472479493,33.8906494393247));
#30241=CARTESIAN_POINT('Ctrl Pts',(18.223524895383,64.3440083919673,33.7795163213331));
#30242=CARTESIAN_POINT('Ctrl Pts',(17.6452215387575,66.5942982401586,33.6683832033416));
#30243=CARTESIAN_POINT('Ctrl Pts',(19.2221041132247,68.3006629449443,33.55725008535));
#30244=CARTESIAN_POINT('Ctrl Pts',(21.5109476208589,67.9013703706408,33.4461169673585));
#30245=CARTESIAN_POINT('Ctrl Pts',(22.416912395611,65.7618687952487,33.3349838493669));
#30246=CARTESIAN_POINT('Ctrl Pts',(21.1108238171316,63.8403142715337,33.2238507313754));
#30247=CARTESIAN_POINT('Ctrl Pts',(18.7880655596257,63.8953891307446,33.1127176133838));
#30248=CARTESIAN_POINT('Ctrl Pts',(17.5745174032192,65.8766866942591,33.0015844953923));
#30249=CARTESIAN_POINT('Ctrl Pts',(18.5808663854542,67.9708454487097,32.8904513774007));
#30250=CARTESIAN_POINT('Ctrl Pts',(20.8860623082748,68.2612088768015,32.7793182594092));
#30251=CARTESIAN_POINT('Ctrl Pts',(22.3802991314904,66.4820249405198,32.6681851414175));
#30252=CARTESIAN_POINT('Ctrl Pts',(21.6959925019048,64.261672806363,32.5570520234261));
#30253=CARTESIAN_POINT('Ctrl Pts',(19.4594467809617,63.6323061397115,32.4459189054344));
#30254=CARTESIAN_POINT('Ctrl Pts',(17.7176366420497,65.1699460855199,32.3347857874429));
#30255=CARTESIAN_POINT('Ctrl Pts',(18.0647352812803,67.4672840444633,32.2236526694513));
#30256=CARTESIAN_POINT('Ctrl Pts',(20.1830643623602,68.4217058941771,32.1125195514598));
#30257=CARTESIAN_POINT('Ctrl Pts',(22.133845733665,67.1596871921246,32.0013864334682));
#30258=CARTESIAN_POINT('Ctrl Pts',(22.1316475021699,64.8362771269967,31.8902533154767));
#30259=CARTESIAN_POINT('Ctrl Pts',(20.1784815758609,63.5779520389273,31.7791201974851));
#30260=CARTESIAN_POINT('Ctrl Pts',(18.0619622863575,64.5363805757104,31.6679870794936));
#30261=CARTESIAN_POINT('Ctrl Pts',(17.719211392801,66.8343712171026,31.556853961502));
#30262=CARTESIAN_POINT('Ctrl Pts',(19.4639280035177,68.3687124800713,31.4457208435104));
#30263=CARTESIAN_POINT('Ctrl Pts',(21.6992788050032,67.7351148496642,31.3345877255189));
#30264=CARTESIAN_POINT('Ctrl Pts',(22.3793827611878,65.5134718153893,31.2234546075273));
#30265=CARTESIAN_POINT('Ctrl Pts',(20.8817819627404,63.737118525233,31.1123214895358));
#30266=CARTESIAN_POINT('Ctrl Pts',(18.5771396053932,64.0318434269302,31.0011883715442));
#30267=CARTESIAN_POINT('Ctrl Pts',(17.5747550844295,66.1279026901889,30.8900552535526));
#30268=CARTESIAN_POINT('Ctrl Pts',(18.7920501669056,68.1069003771858,30.7789221355611));
#30269=CARTESIAN_POINT('Ctrl Pts',(21.1149084810719,68.1575799121915,30.6677890175695));
#30270=CARTESIAN_POINT('Ctrl Pts',(22.4173586709909,66.2335573900417,30.556655899578));
#30271=CARTESIAN_POINT('Ctrl Pts',(21.507347058909,64.0957739517965,30.4455227815864));
#30272=CARTESIAN_POINT('Ctrl Pts',(19.2177520899114,63.700813142474,30.3343896635948));
#30273=CARTESIAN_POINT('Ctrl Pts',(17.6441011972046,65.4101586402722,30.2232565456033));
#30274=CARTESIAN_POINT('Ctrl Pts',(18.2266616160895,67.6593501664229,30.1121234276117));
#30275=CARTESIAN_POINT('Ctrl Pts',(20.4322511218479,68.3898391088773,30.0009903096202));
#30276=CARTESIAN_POINT('Ctrl Pts',(22.2422273876527,66.9330532357364,29.8898571916286));
#30277=CARTESIAN_POINT('Ctrl Pts',(22.0000288950678,64.622300316632,29.778724073637));
#30278=CARTESIAN_POINT('Ctrl Pts',(19.9273252373466,63.5724723734772,29.6675909556455));
#30279=CARTESIAN_POINT('Ctrl Pts',(17.9211363828566,64.7444132606722,29.5564578376539));
#30280=CARTESIAN_POINT('Ctrl Pts',(17.8176053340508,67.0655165511127,29.4453247196624));
#30281=CARTESIAN_POINT('Ctrl Pts',(19.7114877817388,68.4114171556518,29.3341916016708));
#30282=CARTESIAN_POINT('Ctrl Pts',(21.8694279673096,67.5502938668842,29.2230584836792));
#30283=CARTESIAN_POINT('Ctrl Pts',(22.316394097231,65.2702806121721,29.1119253656877));
#30284=CARTESIAN_POINT('Ctrl Pts',(20.6433051769832,63.6581352626753,29.0007922476961));
#30285=CARTESIAN_POINT('Ctrl Pts',(18.3814380385156,64.1893566956759,28.8896591297046));
#30286=CARTESIAN_POINT('Ctrl Pts',(17.600942513176,66.37775014702,28.778526011713));
#30287=CARTESIAN_POINT('Ctrl Pts',(19.0161588257614,68.2204117957101,28.6673928937215));
#30288=CARTESIAN_POINT('Ctrl Pts',(21.3318253046188,68.0308651744107,28.5562597757299));
#30289=CARTESIAN_POINT('Ctrl Pts',(22.4285528445608,65.982590811414,28.4451266577383));
#30290=CARTESIAN_POINT('Ctrl Pts',(21.3025732342425,63.9502500230349,28.3339935397468));
#30291=CARTESIAN_POINT('Ctrl Pts',(18.9844273311818,63.7939210909379,28.2228604217552));
#30292=CARTESIAN_POINT('Ctrl Pts',(17.595773507136,65.6566824068527,28.1117273037637));
#30293=CARTESIAN_POINT('Ctrl Pts',(18.4075623988682,67.833661496828,28.0005941857721));
#30294=CARTESIAN_POINT('Ctrl Pts',(20.6768128607374,68.3324014127664,27.8894610677805));
#30295=CARTESIAN_POINT('Ctrl Pts',(22.3266175536682,66.6964357531696,27.778327949789));
#30296=CARTESIAN_POINT('Ctrl Pts',(21.8470102861031,64.4230646811199,27.6671948317974));
#30297=CARTESIAN_POINT('Ctrl Pts',(19.6769465082846,63.592966879896,27.5560617138059));
#30298=CARTESIAN_POINT('Ctrl Pts',(17.8025539989437,64.9658805312536,27.4449285958143));
#30299=CARTESIAN_POINT('Ctrl Pts',(17.9393505651906,67.2852610206366,27.3337954778227));
#30300=CARTESIAN_POINT('Ctrl Pts',(19.9621345909966,68.4283200411723,27.2226623598312));
#30301=CARTESIAN_POINT('Ctrl Pts',(22.0195745485331,67.3488849730689,27.1115292418396));
#30302=CARTESIAN_POINT('Ctrl Pts',(22.2286203516014,65.0348973043881,27.0003961238481));
#30303=CARTESIAN_POINT('Ctrl Pts',(20.3979451669564,63.6042095721724,26.8892630058565));
#30304=CARTESIAN_POINT('Ctrl Pts',(18.2030547515686,64.366243609939,26.7781298878649));
#30305=CARTESIAN_POINT('Ctrl Pts',(17.6527996556662,66.6235556542679,26.6669967698734));
#30306=CARTESIAN_POINT('Ctrl Pts',(19.2507940995179,68.310165311319,26.5558636518818));
#30307=CARTESIAN_POINT('Ctrl Pts',(21.5344924689199,67.8824201691326,26.4447305338903));
#30308=CARTESIAN_POINT('Ctrl Pts',(22.4137605469628,65.7318111515436,26.3335974158987));
#30309=CARTESIAN_POINT('Ctrl Pts',(21.0838647269646,63.8266568213479,26.2224642979072));
#30310=CARTESIAN_POINT('Ctrl Pts',(18.7619637584228,63.9106363014535,26.1113311799156));
#30311=CARTESIAN_POINT('Ctrl Pts',(17.5731812097634,65.906874520057,26.000198061924));
#30312=CARTESIAN_POINT('Ctrl Pts',(18.605481004107,67.988363098335,25.8890649439325));
#30313=CARTESIAN_POINT('Ctrl Pts',(20.9141747100121,68.249987107151,25.7779318259409));
#30314=CARTESIAN_POINT('Ctrl Pts',(22.3860297127563,66.4524069399739,25.6667987079494));
#30315=CARTESIAN_POINT('Ctrl Pts',(21.6743955698345,64.2406214035846,25.5556655899578));
#30316=CARTESIAN_POINT('Ctrl Pts',(19.4296920915163,63.6393770033003,25.4445324719662));
#30317=CARTESIAN_POINT('Ctrl Pts',(17.7081475008618,65.1980921999731,25.3333993539747));
#30318=CARTESIAN_POINT('Ctrl Pts',(18.081809228925,67.4918926803607,25.2222662359831));
#30319=CARTESIAN_POINT('Ctrl Pts',(20.2159933450493,68.4179588201339,25.1111331179916));
#30320=CARTESIAN_POINT('Ctrl Pts',(21.4986774253635,67.5629326473988,25.0370443726639));
#30321=CARTESIAN_POINT('Ctrl Pts',(21.8174278887594,66.9586205879593,25.));
#30322=CARTESIAN_POINT('Ctrl Pts',(21.2690708798523,67.0793586530486,36.));
#30323=CARTESIAN_POINT('Ctrl Pts',(21.3144000771637,67.0370713228889,36.));
#30324=CARTESIAN_POINT('Ctrl Pts',(21.3569992688451,66.9922148769181,36.));
#30325=CARTESIAN_POINT('Ctrl Pts',(21.3968699348127,66.9451343396547,36.));
#30326=CARTESIAN_POINT('Ctrl Pts',(21.4393722087531,66.8949463168699,36.));
#30327=CARTESIAN_POINT('Ctrl Pts',(21.4787746097791,66.8422306840625,36.));
#30328=CARTESIAN_POINT('Ctrl Pts',(21.5150500980415,66.7873506773072,36.));
#30329=CARTESIAN_POINT('Ctrl Pts',(21.5467911502712,66.7393306713963,36.));
#30330=CARTESIAN_POINT('Ctrl Pts',(21.5761379164984,66.6896523410759,36.));
#30331=CARTESIAN_POINT('Ctrl Pts',(21.6030493891106,66.6385314719273,36.));
#30332=CARTESIAN_POINT('Ctrl Pts',(21.6165496501045,66.612886458528,36.));
#30333=CARTESIAN_POINT('Ctrl Pts',(21.6294366912151,66.5868780640734,36.));
#30334=CARTESIAN_POINT('Ctrl Pts',(21.6417029941218,66.5605316893449,36.));
#30335=CARTESIAN_POINT('Ctrl Pts',(21.647311956908,66.5484843889866,36.));
#30336=CARTESIAN_POINT('Ctrl Pts',(21.6527917063131,66.5363647353609,36.));
#30337=CARTESIAN_POINT('Ctrl Pts',(21.6581330108966,66.5241951160997,36.));
#30338=CARTESIAN_POINT('Ctrl Pts',(21.6850519415314,66.462863070413,36.));
#30339=CARTESIAN_POINT('Ctrl Pts',(21.7085097094311,66.4001555622147,36.));
#30340=CARTESIAN_POINT('Ctrl Pts',(21.7284828098912,66.3364303588019,36.));
#30341=CARTESIAN_POINT('Ctrl Pts',(21.7488102273524,66.2715746887893,36.));
#30342=CARTESIAN_POINT('Ctrl Pts',(21.7655288042216,66.20566405463,36.));
#30343=CARTESIAN_POINT('Ctrl Pts',(21.7785744463911,66.1390390910945,36.));
#30344=CARTESIAN_POINT('Ctrl Pts',(21.7894856788381,66.0833147001856,36.));
#30345=CARTESIAN_POINT('Ctrl Pts',(21.7978269670469,66.0270896613916,36.));
#30346=CARTESIAN_POINT('Ctrl Pts',(21.8035359856737,65.970550992101,36.));
#30347=CARTESIAN_POINT('Ctrl Pts',(21.8061656064956,65.9445088171278,36.));
#30348=CARTESIAN_POINT('Ctrl Pts',(21.8082364301197,65.9183999892448,36.));
#30349=CARTESIAN_POINT('Ctrl Pts',(21.8097405642396,65.8922423831419,36.));
#30350=CARTESIAN_POINT('Ctrl Pts',(21.8103979291679,65.8808104950978,36.));
#30351=CARTESIAN_POINT('Ctrl Pts',(21.8109469376435,65.8693694952185,36.));
#30352=CARTESIAN_POINT('Ctrl Pts',(21.8113865961963,65.8579350105965,36.));
#30353=CARTESIAN_POINT('Ctrl Pts',(21.8140829654057,65.7878087909138,36.));
#30354=CARTESIAN_POINT('Ctrl Pts',(21.8126785983873,65.7177962634573,36.));
#30355=CARTESIAN_POINT('Ctrl Pts',(21.8071188655741,65.6482582300993,36.));
#30356=CARTESIAN_POINT('Ctrl Pts',(21.8021493024575,65.5861017097425,36.));
#30357=CARTESIAN_POINT('Ctrl Pts',(21.7938593908609,65.5243233307745,36.));
#30358=CARTESIAN_POINT('Ctrl Pts',(21.7821770073433,65.4631686326352,36.));
#30359=CARTESIAN_POINT('Ctrl Pts',(21.7694465551382,65.3965275263397,36.));
#30360=CARTESIAN_POINT('Ctrl Pts',(21.7526887129988,65.3306261926924,36.));
#30361=CARTESIAN_POINT('Ctrl Pts',(21.7321487118934,65.2656782084348,36.));
#30362=CARTESIAN_POINT('Ctrl Pts',(21.7242193534609,65.2406053837546,36.));
#30363=CARTESIAN_POINT('Ctrl Pts',(21.7157257837476,65.2156746844024,36.));
#30364=CARTESIAN_POINT('Ctrl Pts',(21.7066801015395,65.1908987184666,36.));
#30365=CARTESIAN_POINT('Ctrl Pts',(21.7027127271974,65.1800321492803,36.));
#30366=CARTESIAN_POINT('Ctrl Pts',(21.698639247911,65.1691959127051,36.));
#30367=CARTESIAN_POINT('Ctrl Pts',(21.6944657697982,65.1584036090012,36.));
#30368=CARTESIAN_POINT('Ctrl Pts',(21.6692429532713,65.0931792831816,36.));
#30369=CARTESIAN_POINT('Ctrl Pts',(21.6403293178684,65.0294403704392,36.));
#30370=CARTESIAN_POINT('Ctrl Pts',(21.6080375203115,64.9674056751725,36.));
#30371=CARTESIAN_POINT('Ctrl Pts',(21.5749977153262,64.903934007783,36.));
#30372=CARTESIAN_POINT('Ctrl Pts',(21.5384211298212,64.8422456059961,36.));
#30373=CARTESIAN_POINT('Ctrl Pts',(21.4985865170694,64.7825785480101,36.));
#30374=CARTESIAN_POINT('Ctrl Pts',(21.4680938596675,64.7369045215376,36.));
#30375=CARTESIAN_POINT('Ctrl Pts',(21.4356909069961,64.6924148931467,36.));
#30376=CARTESIAN_POINT('Ctrl Pts',(21.401483143624,64.6492225546256,36.));
#30377=CARTESIAN_POINT('Ctrl Pts',(21.3801865973203,64.6223325288946,36.));
#30378=CARTESIAN_POINT('Ctrl Pts',(21.3581902064885,64.5959454384605,36.));
#30379=CARTESIAN_POINT('Ctrl Pts',(21.3355165165973,64.570090213464,36.));
#30380=CARTESIAN_POINT('Ctrl Pts',(21.3228384297211,64.5556331581599,36.));
#30381=CARTESIAN_POINT('Ctrl Pts',(21.3099441169479,64.5413378602927,36.));
#30382=CARTESIAN_POINT('Ctrl Pts',(21.2968612031401,64.527234782426,36.));
#30383=CARTESIAN_POINT('Ctrl Pts',(21.2459899661476,64.4723967679729,36.));
#30384=CARTESIAN_POINT('Ctrl Pts',(21.192222187541,64.42040369654,36.));
#30385=CARTESIAN_POINT('Ctrl Pts',(21.1358428134485,64.3715194870934,36.));
#30386=CARTESIAN_POINT('Ctrl Pts',(21.0936832442526,64.334964678816,36.));
#30387=CARTESIAN_POINT('Ctrl Pts',(21.0500621658713,64.3001484832718,36.));
#30388=CARTESIAN_POINT('Ctrl Pts',(21.0050823390709,64.2671910015265,36.));
#30389=CARTESIAN_POINT('Ctrl Pts',(20.9910186946901,64.2568863308347,36.));
#30390=CARTESIAN_POINT('Ctrl Pts',(20.9768221267921,64.2467634444957,36.));
#30391=CARTESIAN_POINT('Ctrl Pts',(20.9624955349648,64.2368262403725,36.));
#30392=CARTESIAN_POINT('Ctrl Pts',(20.9487061818225,64.2272616755022,36.));
#30393=CARTESIAN_POINT('Ctrl Pts',(20.9348034145042,64.2178740747608,36.));
#30394=CARTESIAN_POINT('Ctrl Pts',(20.9207951922747,64.2086696546068,36.));
#30395=CARTESIAN_POINT('Ctrl Pts',(20.8578415028037,64.1673045050084,36.));
#30396=CARTESIAN_POINT('Ctrl Pts',(20.7927303594474,64.129615031017,36.));
#30397=CARTESIAN_POINT('Ctrl Pts',(20.7257230462104,64.0958803998092,36.));
#30398=CARTESIAN_POINT('Ctrl Pts',(20.674495644503,64.0700901178109,36.));
#30399=CARTESIAN_POINT('Ctrl Pts',(20.6221590194026,64.046611719858,36.));
#30400=CARTESIAN_POINT('Ctrl Pts',(20.5688160527906,64.0255852000049,36.));
#30401=CARTESIAN_POINT('Ctrl Pts',(20.5563688085073,64.0206787944249,36.));
#30402=CARTESIAN_POINT('Ctrl Pts',(20.5438667254187,64.0159059590366,36.));
#30403=CARTESIAN_POINT('Ctrl Pts',(20.5313117419429,64.0112661051077,36.));
#30404=CARTESIAN_POINT('Ctrl Pts',(18.332682423241,65.9986976781594,34.8714803633902));
#30405=CARTESIAN_POINT('Ctrl Pts',(18.3319481375098,65.9132137662013,34.8772098489549));
#30406=CARTESIAN_POINT('Ctrl Pts',(18.3379547564459,65.8278333817693,34.8829393345197));
#30407=CARTESIAN_POINT('Ctrl Pts',(18.3510613223839,65.7435572610759,34.8886688200844));
#30408=CARTESIAN_POINT('Ctrl Pts',(18.4358027022978,65.198664358152,34.9257131927483));
#30409=CARTESIAN_POINT('Ctrl Pts',(18.8173471166954,64.6999336066327,34.9627575654121));
#30410=CARTESIAN_POINT('Ctrl Pts',(19.321092927466,64.4755855291333,34.999801938076));
#30411=CARTESIAN_POINT('Ctrl Pts',(19.8248387382366,64.251237451634,35.0368463107398));
#30412=CARTESIAN_POINT('Ctrl Pts',(20.4507859453801,64.3012720481544,35.0738906834037));
#30413=CARTESIAN_POINT('Ctrl Pts',(20.9124876026766,64.6028094202091,35.1109350560675));
#30414=CARTESIAN_POINT('Ctrl Pts',(21.3741892599732,64.9043467922638,35.1479794287314));
#30415=CARTESIAN_POINT('Ctrl Pts',(21.671645367423,65.4573869398528,35.1850238013952));
#30416=CARTESIAN_POINT('Ctrl Pts',(21.6687365206648,66.0088140739646,35.2220681740591));
#30417=CARTESIAN_POINT('Ctrl Pts',(21.6658276739067,66.5602412080764,35.2591125467229));
#30418=CARTESIAN_POINT('Ctrl Pts',(21.3625538729407,67.1100553287111,35.2961569193868));
#30419=CARTESIAN_POINT('Ctrl Pts',(20.8976944633723,67.4067179401272,35.3332012920506));
#30420=CARTESIAN_POINT('Ctrl Pts',(20.4328350538039,67.7033805515432,35.3702456647145));
#30421=CARTESIAN_POINT('Ctrl Pts',(19.806390035633,67.7468916537407,35.4072900373783));
#30422=CARTESIAN_POINT('Ctrl Pts',(19.3050423733628,67.5172055704405,35.4443344100422));
#30423=CARTESIAN_POINT('Ctrl Pts',(18.8036947110926,67.2875194871403,35.4813787827061));
#30424=CARTESIAN_POINT('Ctrl Pts',(18.4274444047231,66.7846362183425,35.5184231553699));
#30425=CARTESIAN_POINT('Ctrl Pts',(18.3484523152824,66.2389526568346,35.5554675280338));
#30426=CARTESIAN_POINT('Ctrl Pts',(18.337070583666,66.1603267603867,35.5608051398193));
#30427=CARTESIAN_POINT('Ctrl Pts',(18.3318602470798,66.0808122845869,35.5661427516047));
#30428=CARTESIAN_POINT('Ctrl Pts',(18.3325226254757,66.0012132166996,35.5714803633902));
#30429=CARTESIAN_POINT('Ctrl Pts',(19.4698297828115,64.0148256743282,36.));
#30430=CARTESIAN_POINT('Ctrl Pts',(18.809740437582,64.1911123142462,35.9629556273362));
#30431=CARTESIAN_POINT('Ctrl Pts',(17.6907270524739,65.2513727719513,35.8888668820085));
#30432=CARTESIAN_POINT('Ctrl Pts',(18.1186749695233,67.5381215598298,35.7777337640169));
#30433=CARTESIAN_POINT('Ctrl Pts',(20.2718170903172,68.4128312567252,35.6666006460253));
#30434=CARTESIAN_POINT('Ctrl Pts',(22.1745315590613,67.0812974610511,35.5554675280338));
#30435=CARTESIAN_POINT('Ctrl Pts',(22.0878552063855,64.7590834656903,35.4443344100422));
#30436=CARTESIAN_POINT('Ctrl Pts',(20.0898773670193,63.5731233891133,35.3332012920506));
#30437=CARTESIAN_POINT('Ctrl Pts',(18.0098479899297,64.6080763840108,35.2220681740591));
#30438=CARTESIAN_POINT('Ctrl Pts',(17.7511798490307,66.91710303298,35.1109350560675));
#30439=CARTESIAN_POINT('Ctrl Pts',(19.5507726973617,68.3866954932114,34.999801938076));
#30440=CARTESIAN_POINT('Ctrl Pts',(21.761489833587,67.6719231014153,34.8886688200844));
#30441=CARTESIAN_POINT('Ctrl Pts',(22.3600352949887,65.4269244270303,34.7775357020928));
#30442=CARTESIAN_POINT('Ctrl Pts',(20.7985769670495,63.7064353263736,34.6664025841013));
#30443=CARTESIAN_POINT('Ctrl Pts',(18.5062328763905,64.0851027489721,34.5552694661098));
#30444=CARTESIAN_POINT('Ctrl Pts',(17.5810415914568,66.2163615818994,34.4441363481181));
#30445=CARTESIAN_POINT('Ctrl Pts',(18.869777083907,68.1495967375546,34.3330032301266));
#30446=CARTESIAN_POINT('Ctrl Pts',(21.1929366566675,68.1154368741692,34.221870112135));
#30447=CARTESIAN_POINT('Ctrl Pts',(22.4242738572048,66.1451456586872,34.1107369941435));
#30448=CARTESIAN_POINT('Ctrl Pts',(21.4368201000595,64.0420115549533,33.9996038761519));
#30449=CARTESIAN_POINT('Ctrl Pts',(19.1343320873597,63.7309054758618,33.8884707581604));
#30450=CARTESIAN_POINT('Ctrl Pts',(17.6241373942269,65.4965640490266,33.7773376401688));
#30451=CARTESIAN_POINT('Ctrl Pts',(18.2884256842001,67.7229870029778,33.6662045221773));
#30452=CARTESIAN_POINT('Ctrl Pts',(20.5192141482499,68.3724644440178,33.5550714041857));
#30453=CARTESIAN_POINT('Ctrl Pts',(22.2747973910883,66.850569042428,33.4439382861942));
#30454=CARTESIAN_POINT('Ctrl Pts',(21.9483965247762,64.5501993772306,33.3328051682026));
#30455=CARTESIAN_POINT('Ctrl Pts',(19.8387464716884,63.5767443045379,33.221672050211));
#30456=CARTESIAN_POINT('Ctrl Pts',(17.8766819941674,64.8211482232738,33.1105389322195));
#30457=CARTESIAN_POINT('Ctrl Pts',(17.8579617287779,67.144483686959,32.9994058142279));
#30458=CARTESIAN_POINT('Ctrl Pts',(19.7997191989097,68.420342634033,32.8882726962363));
#30459=CARTESIAN_POINT('Ctrl Pts',(21.924781541228,67.4810087386156,32.7771395782448));
#30460=CARTESIAN_POINT('Ctrl Pts',(22.2882080583246,65.1861973537148,32.6660064602532));
#30461=CARTESIAN_POINT('Ctrl Pts',(20.5573764974643,63.6362101816373,32.5548733422617));
#30462=CARTESIAN_POINT('Ctrl Pts',(18.3164120279928,64.2496564891946,32.4437402242701));
#30463=CARTESIAN_POINT('Ctrl Pts',(17.6163335358825,66.4650860706858,32.3326071062786));
#30464=CARTESIAN_POINT('Ctrl Pts',(19.0978804119286,68.2548505746783,32.221473988287));
#30465=CARTESIAN_POINT('Ctrl Pts',(21.4050826420595,67.9808870826703,32.1103408702955));
#30466=CARTESIAN_POINT('Ctrl Pts',(22.4262979346632,65.8939377656472,31.9992077523039));
#30467=CARTESIAN_POINT('Ctrl Pts',(21.2268698593072,63.9040607800724,31.8880746343123));
#30468=CARTESIAN_POINT('Ctrl Pts',(18.9045621995861,63.8324698639393,31.7769415163208));
#30469=CARTESIAN_POINT('Ctrl Pts',(17.5848423308155,65.7446878414837,31.6658083983292));
#30470=CARTESIAN_POINT('Ctrl Pts',(18.4755698205621,67.8905775554909,31.5546752803376));
#30471=CARTESIAN_POINT('Ctrl Pts',(20.7615158115174,68.3061362783054,31.4435421623461));
#30472=CARTESIAN_POINT('Ctrl Pts',(22.3504925588018,66.6110283105753,31.3324090443545));
#30473=CARTESIAN_POINT('Ctrl Pts',(21.7882060017851,64.3566831831669,31.2212759263629));
#30474=CARTESIAN_POINT('Ctrl Pts',(19.5892829288324,63.6063662868436,31.1101428083714));
#30475=CARTESIAN_POINT('Ctrl Pts',(17.7662642850786,65.0467971773061,30.9990096903798));
#30476=CARTESIAN_POINT('Ctrl Pts',(17.9876484866019,67.3596368087955,30.8878765723883));
#30477=CARTESIAN_POINT('Ctrl Pts',(20.0508159985709,68.4280833180919,30.7767434543967));
#30478=CARTESIAN_POINT('Ctrl Pts',(22.0674747085496,67.2742524062426,30.6656103364052));
#30479=CARTESIAN_POINT('Ctrl Pts',(22.1918991902521,64.954175538114,30.5544772184136));
#30480=CARTESIAN_POINT('Ctrl Pts',(20.3102112607245,63.5912783807532,30.4433441004221));
#30481=CARTESIAN_POINT('Ctrl Pts',(18.1446057755856,64.4329380556861,30.3322109824305));
#30482=CARTESIAN_POINT('Ctrl Pts',(17.6771301122358,66.7088345010122,30.2210778644389));
#30483=CARTESIAN_POINT('Ctrl Pts',(19.3356363974357,68.3359777115578,30.1099447464474));
#30484=CARTESIAN_POINT('Ctrl Pts',(21.602194400799,67.8251421772989,29.9988116284558));
#30485=CARTESIAN_POINT('Ctrl Pts',(22.402361026794,65.6438646854799,29.8876785104642));
#30486=CARTESIAN_POINT('Ctrl Pts',(21.0037922850585,63.7885362508592,29.7765453924727));
#30487=CARTESIAN_POINT('Ctrl Pts',(18.6865133351581,63.957226481817,29.6654122744811));
#30488=CARTESIAN_POINT('Ctrl Pts',(17.5713890792524,65.9955434393982,29.5542791564896));
#30489=CARTESIAN_POINT('Ctrl Pts',(18.6790251272092,68.0379392166506,29.443146038498));
#30490=CARTESIAN_POINT('Ctrl Pts',(20.9956693718085,68.2151328103185,29.3320129205064));
#30491=CARTESIAN_POINT('Ctrl Pts',(22.4010378181641,66.3649496692051,29.2208798025149));
#30492=CARTESIAN_POINT('Ctrl Pts',(21.6088819494082,64.1807502265562,29.1097466845233));
#30493=CARTESIAN_POINT('Ctrl Pts',(19.3442139955776,63.6615997815364,28.9986135665318));
#30494=CARTESIAN_POINT('Ctrl Pts',(17.6797472044798,65.2826452549903,28.8874804485402));
#30495=CARTESIAN_POINT('Ctrl Pts',(18.1388670961024,67.5602420258845,28.7763473305487));
#30496=CARTESIAN_POINT('Ctrl Pts',(20.301369074849,68.4098438841618,28.6652142125571));
#30497=CARTESIAN_POINT('Ctrl Pts',(22.1880462145232,67.053861769123,28.5540810945655));
#30498=CARTESIAN_POINT('Ctrl Pts',(22.0721373380047,64.7333438833879,28.442947976574));
#30499=CARTESIAN_POINT('Ctrl Pts',(20.059726811216,63.5721195306752,28.3318148585824));
#30500=CARTESIAN_POINT('Ctrl Pts',(17.9926519559727,64.6329869439321,28.2206817405909));
#30501=CARTESIAN_POINT('Ctrl Pts',(17.7627810390829,66.9449985112133,28.1095486225993));
#30502=CARTESIAN_POINT('Ctrl Pts',(19.5805009712835,68.3921102462499,27.9984155046077));
#30503=CARTESIAN_POINT('Ctrl Pts',(21.7821629259284,67.6498685313834,27.8872823866162));
#30504=CARTESIAN_POINT('Ctrl Pts',(22.3527192254304,65.3976021983889,27.7761492686246));
#30505=CARTESIAN_POINT('Ctrl Pts',(20.7699742878597,63.6966740436017,27.6650161506331));
#30506=CARTESIAN_POINT('Ctrl Pts',(18.482518575813,64.103840462084,27.5538830326415));
#30507=CARTESIAN_POINT('Ctrl Pts',(17.5839215913354,66.2464467218836,27.4427499146499));
#30508=CARTESIAN_POINT('Ctrl Pts',(18.8966146610587,68.1634952415589,27.3316167966584));
#30509=CARTESIAN_POINT('Ctrl Pts',(21.2191694244532,68.1004277622309,27.2204836786668));
#30510=CARTESIAN_POINT('Ctrl Pts',(22.4258923392674,66.1149661220525,27.1093505606753));
#30511=CARTESIAN_POINT('Ctrl Pts',(21.4123431135179,64.0242829635948,26.9982174426837));
#30512=CARTESIAN_POINT('Ctrl Pts',(19.1061618600091,63.7418537970392,26.8870843246921));
#30513=CARTESIAN_POINT('Ctrl Pts',(17.6180564951812,65.5261689217424,26.7759512067006));
#30514=CARTESIAN_POINT('Ctrl Pts',(18.3099994949436,67.7441528860369,26.664818088709));
#30515=CARTESIAN_POINT('Ctrl Pts',(20.5486976409782,68.3658195058375,26.5536849707175));
#30516=CARTESIAN_POINT('Ctrl Pts',(22.2852057779767,66.8221949443221,26.4425518527259));
#30517=CARTESIAN_POINT('Ctrl Pts',(21.9302043029995,64.5260653118046,26.3314187347344));
#30518=CARTESIAN_POINT('Ctrl Pts',(19.8086025603331,63.5789385134492,26.2202856167428));
#30519=CARTESIAN_POINT('Ctrl Pts',(17.8621779143328,64.8476628902778,26.1091524987512));
#30520=CARTESIAN_POINT('Ctrl Pts',(17.8723669486581,67.1710507268108,25.9980193807597));
#30521=CARTESIAN_POINT('Ctrl Pts',(19.8298599336245,68.4226484781515,25.8868862627681));
#30522=CARTESIAN_POINT('Ctrl Pts',(21.9430509921809,67.4569397340099,25.7757531447766));
#30523=CARTESIAN_POINT('Ctrl Pts',(22.2779267956692,65.1577888874642,25.664620026785));
#30524=CARTESIAN_POINT('Ctrl Pts',(20.5278716209092,63.6294498681163,25.5534869087934));
#30525=CARTESIAN_POINT('Ctrl Pts',(18.2948524671343,64.2707574153019,25.4423537908019));
#30526=CARTESIAN_POINT('Ctrl Pts',(17.6221226867318,66.4946844357757,25.3312206728103));
#30527=CARTESIAN_POINT('Ctrl Pts',(19.1263753077513,68.2659593106943,25.2200875548188));
#30528=CARTESIAN_POINT('Ctrl Pts',(21.4288959883911,67.963134090779,25.1089544368272));
#30529=CARTESIAN_POINT('Ctrl Pts',(22.4262527337127,65.8639872238968,24.9978213188357));
#30530=CARTESIAN_POINT('Ctrl Pts',(21.1976535364003,63.8884104850849,24.8866882008441));
#30531=CARTESIAN_POINT('Ctrl Pts',(19.6563391459161,63.8620828587222,24.8125994555164));
#30532=CARTESIAN_POINT('Ctrl Pts',(19.0504464477386,64.1778184465077,24.7755550828525));
#30533=CARTESIAN_POINT('Ctrl Pts',(19.5032651029124,64.1400211999972,36.0748149723825));
#30534=CARTESIAN_POINT('Ctrl Pts',(18.8848044607624,64.3051902779623,36.0377705997186));
#30535=CARTESIAN_POINT('Ctrl Pts',(17.8363619404734,65.2985851392148,35.963681854391));
#30536=CARTESIAN_POINT('Ctrl Pts',(18.2373212128777,67.4411195309724,35.8525487363994));
#30537=CARTESIAN_POINT('Ctrl Pts',(20.2546748761206,68.2606654375174,35.7414156184078));
#30538=CARTESIAN_POINT('Ctrl Pts',(22.0373941711252,67.0131051606116,35.6302825004163));
#30539=CARTESIAN_POINT('Ctrl Pts',(21.9561840847596,64.8373421837361,35.5191493824247));
#30540=CARTESIAN_POINT('Ctrl Pts',(20.0842092279223,63.7261749821672,35.4080162644331));
#30541=CARTESIAN_POINT('Ctrl Pts',(18.1353574345361,64.6958584022151,35.2968831464416));
#30542=CARTESIAN_POINT('Ctrl Pts',(17.8930022659816,66.8592656960662,35.18575002845));
#30543=CARTESIAN_POINT('Ctrl Pts',(19.5791033318916,68.2361779326022,35.0746169104584));
#30544=CARTESIAN_POINT('Ctrl Pts',(21.6504010275187,67.5664828441779,34.9634837924669));
#30545=CARTESIAN_POINT('Ctrl Pts',(22.2111990665867,65.4630655843475,34.8523506744753));
#30546=CARTESIAN_POINT('Ctrl Pts',(20.7482145067436,63.8510795680691,34.7412175564838));
#30547=CARTESIAN_POINT('Ctrl Pts',(18.6004376814038,64.2058662329868,34.6300844384922));
#30548=CARTESIAN_POINT('Ctrl Pts',(17.7335938210583,66.2027166834992,34.5189513205006));
#30549=CARTESIAN_POINT('Ctrl Pts',(18.9410548806594,68.0140318705027,34.4078182025091));
#30550=CARTESIAN_POINT('Ctrl Pts',(21.1177038018548,67.9820263076229,34.2966850845175));
#30551=CARTESIAN_POINT('Ctrl Pts',(22.2713864074764,66.135992010666,34.185551966526));
#30552=CARTESIAN_POINT('Ctrl Pts',(21.3462066736251,64.16549259612,34.0744188485344));
#30553=CARTESIAN_POINT('Ctrl Pts',(19.1889256552778,63.8740065013327,33.9632857305429));
#30554=CARTESIAN_POINT('Ctrl Pts',(17.7739717760243,65.5283133658033,33.8521526125513));
#30555=CARTESIAN_POINT('Ctrl Pts',(18.3963665553957,67.6143263877517,33.7410194945598));
#30556=CARTESIAN_POINT('Ctrl Pts',(20.4864697754337,68.2228443681591,33.6298863765682));
#30557=CARTESIAN_POINT('Ctrl Pts',(22.1313367128573,66.7969276886147,33.5187532585767));
#30558=CARTESIAN_POINT('Ctrl Pts',(21.8255204005102,64.6416314236435,33.4076201405851));
#30559=CARTESIAN_POINT('Ctrl Pts',(19.8489159666199,63.7295675436361,33.2964870225935));
#30560=CARTESIAN_POINT('Ctrl Pts',(18.0105895862942,64.8954928115371,33.185353904602));
#30561=CARTESIAN_POINT('Ctrl Pts',(17.9930499192208,67.0723065310512,33.0742207866104));
#30562=CARTESIAN_POINT('Ctrl Pts',(19.8123499587627,68.2677031078975,32.9630876686188));
#30563=CARTESIAN_POINT('Ctrl Pts',(21.8033947019285,67.3876085444093,32.8519545506273));
#30564=CARTESIAN_POINT('Ctrl Pts',(22.1439016329405,65.2375200253688,32.7408214326357));
#30565=CARTESIAN_POINT('Ctrl Pts',(20.522225406352,63.7852831900144,32.6296883146442));
#30566=CARTESIAN_POINT('Ctrl Pts',(18.4225879332721,64.360042349571,32.5185551966526));
#30567=CARTESIAN_POINT('Ctrl Pts',(17.7666600699987,66.4357552989003,32.407422078661));
#30568=CARTESIAN_POINT('Ctrl Pts',(19.154772814064,68.1126478475166,32.2962889606695));
#30569=CARTESIAN_POINT('Ctrl Pts',(21.3164707465165,67.8559619330757,32.1851558426779));
#30570=CARTESIAN_POINT('Ctrl Pts',(22.2732828359731,65.9006266075346,32.0740227246864));
#30571=CARTESIAN_POINT('Ctrl Pts',(21.1494969984068,64.0362417220762,31.9628896066948));
#30572=CARTESIAN_POINT('Ctrl Pts',(18.9736462641375,63.9691657053464,31.8517564887033));
#30573=CARTESIAN_POINT('Ctrl Pts',(17.737154865819,65.7607891679424,31.7406233707117));
#30574=CARTESIAN_POINT('Ctrl Pts',(18.5717083990195,67.7713477992842,31.6294902527202));
#30575=CARTESIAN_POINT('Ctrl Pts',(20.713490622447,68.1606992051511,31.5183571347285));
#30576=CARTESIAN_POINT('Ctrl Pts',(22.2022581454937,66.5724936541716,31.407224016737));
#30577=CARTESIAN_POINT('Ctrl Pts',(21.6754323337487,64.4603193777638,31.2960908987454));
#30578=CARTESIAN_POINT('Ctrl Pts',(19.6151849057827,63.7573214080651,31.1849577807539));
#30579=CARTESIAN_POINT('Ctrl Pts',(17.907135398219,65.1069111566746,31.0738246627623));
#30580=CARTESIAN_POINT('Ctrl Pts',(18.1145579485532,67.2738909663297,30.9626915447708));
#30581=CARTESIAN_POINT('Ctrl Pts',(20.0476112746476,68.2749556237401,30.8515584267792));
#30582=CARTESIAN_POINT('Ctrl Pts',(21.9370888882229,67.1938913529227,30.7404253087876));
#30583=CARTESIAN_POINT('Ctrl Pts',(22.053666508221,65.0201307248047,30.6292921907961));
#30584=CARTESIAN_POINT('Ctrl Pts',(20.2906477083691,63.7431850246242,30.5181590728045));
#30585=CARTESIAN_POINT('Ctrl Pts',(18.2616166860355,64.5317652172796,30.407025954813));
#30586=CARTESIAN_POINT('Ctrl Pts',(17.8236224947427,66.6641316722385,30.2958928368214));
#30587=CARTESIAN_POINT('Ctrl Pts',(19.3775346576452,68.1886586807968,30.1847597188299));
#30588=CARTESIAN_POINT('Ctrl Pts',(21.501151601868,67.7100391199237,30.0736266008383));
#30589=CARTESIAN_POINT('Ctrl Pts',(22.2508555153098,65.6663244500125,29.9624934828467));
#30590=CARTESIAN_POINT('Ctrl Pts',(20.9404878683304,63.9280027767916,29.8513603648552));
#30591=CARTESIAN_POINT('Ctrl Pts',(18.7693487070131,64.0860545152668,29.7402272468636));
#30592=CARTESIAN_POINT('Ctrl Pts',(17.7245500470004,65.9958244935304,29.6290941288721));
#30593=CARTESIAN_POINT('Ctrl Pts',(18.7623327448103,67.909416059661,29.5179610108805));
#30594=CARTESIAN_POINT('Ctrl Pts',(20.9328772286783,68.0754348941062,29.4068278928889));
#30595=CARTESIAN_POINT('Ctrl Pts',(22.24961575517,66.3419340251441,29.2956947748974));
#30596=CARTESIAN_POINT('Ctrl Pts',(21.5074173985168,64.2954816779778,29.1845616569058));
#30597=CARTESIAN_POINT('Ctrl Pts',(19.3855713073705,63.8090715883138,29.0734285389143));
#30598=CARTESIAN_POINT('Ctrl Pts',(17.8260745393962,65.3278854151269,28.9622954209227));
#30599=CARTESIAN_POINT('Ctrl Pts',(18.2562399178391,67.4618449641881,28.8511623029311));
#30600=CARTESIAN_POINT('Ctrl Pts',(20.2823631572033,68.2578664643672,28.7400291849396));
#30601=CARTESIAN_POINT('Ctrl Pts',(22.0500565213901,66.9873997075995,28.628896066948));
#30602=CARTESIAN_POINT('Ctrl Pts',(21.9414574677611,64.8132258747628,28.5177629489565));
#30603=CARTESIAN_POINT('Ctrl Pts',(20.0559601246183,63.7252344323179,28.4066298309649));
#30604=CARTESIAN_POINT('Ctrl Pts',(18.1192458728508,64.7191979713152,28.2954967129734));
#30605=CARTESIAN_POINT('Ctrl Pts',(17.9038718240213,66.8854019388429,28.1843635949818));
#30606=CARTESIAN_POINT('Ctrl Pts',(19.6069567846287,68.2412512028579,28.0732304769903));
#30607=CARTESIAN_POINT('Ctrl Pts',(21.6697703660137,67.5458191512356,27.9620973589987));
#30608=CARTESIAN_POINT('Ctrl Pts',(22.2043443868229,65.4355925695414,27.8509642410071));
#30609=CARTESIAN_POINT('Ctrl Pts',(20.7214156628193,63.8419338830873,27.7398311230155));
#30610=CARTESIAN_POINT('Ctrl Pts',(18.5782189292465,64.2234222474375,27.628698005024));
#30611=CARTESIAN_POINT('Ctrl Pts',(17.7362921930093,66.2309044964494,27.5175648870324));
#30612=CARTESIAN_POINT('Ctrl Pts',(18.9661999391564,68.0270538618038,27.4064317690409));
#30613=CARTESIAN_POINT('Ctrl Pts',(21.1422821934428,67.9679637491608,27.2952986510493));
#30614=CARTESIAN_POINT('Ctrl Pts',(22.2729028195545,66.107715754214,27.1841655330578));
#30615=CARTESIAN_POINT('Ctrl Pts',(21.3232733344888,64.1488820629017,27.0730324150662));
#30616=CARTESIAN_POINT('Ctrl Pts',(19.1625319905069,63.8842643638399,26.9618992970746));
#30617=CARTESIAN_POINT('Ctrl Pts',(17.7682743704294,65.556051199663,26.8507661790831));
#30618=CARTESIAN_POINT('Ctrl Pts',(18.4165798082567,67.6341574389921,26.7396330610915));
#30619=CARTESIAN_POINT('Ctrl Pts',(20.5140938841659,68.2166184947016,26.6284999431));
#30620=CARTESIAN_POINT('Ctrl Pts',(22.1410886921693,66.7703430102498,26.5173668251084));
#30621=CARTESIAN_POINT('Ctrl Pts',(21.8084754758444,64.6190193792151,26.4062337071169));
#30622=CARTESIAN_POINT('Ctrl Pts',(19.8206730887299,63.7316233742022,26.2951005891253));
#30623=CARTESIAN_POINT('Ctrl Pts',(17.9970002099573,64.9203353242972,26.1839674711337));
#30624=CARTESIAN_POINT('Ctrl Pts',(18.0065466702315,67.097198113752,26.0728343531422));
#30625=CARTESIAN_POINT('Ctrl Pts',(19.8405898603477,68.2698635333681,25.9617012351506));
#30626=CARTESIAN_POINT('Ctrl Pts',(21.8205119852927,67.3650574577238,25.8505681171591));
#30627=CARTESIAN_POINT('Ctrl Pts',(22.1342687607394,65.2109031462952,25.7394349991675));
#30628=CARTESIAN_POINT('Ctrl Pts',(20.4945812623694,63.7789492173915,25.6283018811759));
#30629=CARTESIAN_POINT('Ctrl Pts',(18.4023880316233,64.3798125403864,25.5171687631844));
#30630=CARTESIAN_POINT('Ctrl Pts',(17.7720841265718,66.4634870355391,25.4060356451928));
#30631=CARTESIAN_POINT('Ctrl Pts',(19.1814706720067,68.1230560082598,25.2949025272013));
#30632=CARTESIAN_POINT('Ctrl Pts',(21.3387822980822,67.8393285381504,25.1837694092097));
#30633=CARTESIAN_POINT('Ctrl Pts',(22.2732404856321,65.8725649043462,25.0726362912182));
#30634=CARTESIAN_POINT('Ctrl Pts',(21.122123210363,64.0215784169376,24.9615031732266));
#30635=CARTESIAN_POINT('Ctrl Pts',(19.6780122054164,63.996911149053,24.8874144278989));
#30636=CARTESIAN_POINT('Ctrl Pts',(19.1103302849356,64.2927347913866,24.850370055235));
#30637=CARTESIAN_POINT('Ctrl Pts',(19.5367004230133,64.2652167256662,36.149629944765));
#30638=CARTESIAN_POINT('Ctrl Pts',(18.9598684839429,64.4192682416784,36.1125855721011));
#30639=CARTESIAN_POINT('Ctrl Pts',(17.9819968284729,65.3457975064782,36.0384968267734));
#30640=CARTESIAN_POINT('Ctrl Pts',(18.3559674562322,67.3441175021151,35.9273637087819));
#30641=CARTESIAN_POINT('Ctrl Pts',(20.2375326619242,68.1084996183096,35.8162305907903));
#30642=CARTESIAN_POINT('Ctrl Pts',(21.9002567831891,66.9449128601723,35.7050974727988));
#30643=CARTESIAN_POINT('Ctrl Pts',(21.8245129631337,64.9156009017816,35.5939643548072));
#30644=CARTESIAN_POINT('Ctrl Pts',(20.0785410888253,63.8792265752211,35.4828312368157));
#30645=CARTESIAN_POINT('Ctrl Pts',(18.2608668791425,64.7836404204194,35.371698118824));
#30646=CARTESIAN_POINT('Ctrl Pts',(18.0348246829324,66.8014283591525,35.2605650008325));
#30647=CARTESIAN_POINT('Ctrl Pts',(19.6074339664214,68.0856603719928,35.1494318828409));
#30648=CARTESIAN_POINT('Ctrl Pts',(21.5393122214503,67.4610425869407,35.0382987648494));
#30649=CARTESIAN_POINT('Ctrl Pts',(22.0623628381848,65.4992067416645,34.9271656468578));
#30650=CARTESIAN_POINT('Ctrl Pts',(20.6978520464377,63.9957238097648,34.8160325288663));
#30651=CARTESIAN_POINT('Ctrl Pts',(18.6946424864171,64.3266297170013,34.7048994108747));
#30652=CARTESIAN_POINT('Ctrl Pts',(17.8861460506599,66.189071785099,34.5937662928832));
#30653=CARTESIAN_POINT('Ctrl Pts',(19.0123326774118,67.8784670034509,34.4826331748916));
#30654=CARTESIAN_POINT('Ctrl Pts',(21.042470947042,67.8486157410765,34.3715000569));
#30655=CARTESIAN_POINT('Ctrl Pts',(22.118498957748,66.1268383626448,34.2603669389085));
#30656=CARTESIAN_POINT('Ctrl Pts',(21.2555932471907,64.2889736372867,34.1492338209169));
#30657=CARTESIAN_POINT('Ctrl Pts',(19.2435192231959,64.0171075268036,34.0381007029254));
#30658=CARTESIAN_POINT('Ctrl Pts',(17.9238061578216,65.5600626825801,33.9269675849338));
#30659=CARTESIAN_POINT('Ctrl Pts',(18.5043074265913,67.5056657725256,33.8158344669422));
#30660=CARTESIAN_POINT('Ctrl Pts',(20.4537254026176,68.0732242923004,33.7047013489507));
#30661=CARTESIAN_POINT('Ctrl Pts',(21.9878760346263,66.7432863348013,33.5935682309592));
#30662=CARTESIAN_POINT('Ctrl Pts',(21.7026442762442,64.7330634700566,33.4824351129676));
#30663=CARTESIAN_POINT('Ctrl Pts',(19.8590854615513,63.8823907827342,33.371301994976));
#30664=CARTESIAN_POINT('Ctrl Pts',(18.1444971784209,64.9698373998005,33.2601688769845));
#30665=CARTESIAN_POINT('Ctrl Pts',(18.1281381096636,67.0001293751432,33.1490357589929));
#30666=CARTESIAN_POINT('Ctrl Pts',(19.8249807186157,68.1150635817621,33.0379026410013));
#30667=CARTESIAN_POINT('Ctrl Pts',(21.6820078626288,67.2942083502029,32.9267695230098));
#30668=CARTESIAN_POINT('Ctrl Pts',(21.9995952075565,65.2888426970229,32.8156364050182));
#30669=CARTESIAN_POINT('Ctrl Pts',(20.4870743152396,63.9343561983915,32.7045032870266));
#30670=CARTESIAN_POINT('Ctrl Pts',(18.5287638385514,64.4704282099475,32.5933701690351));
#30671=CARTESIAN_POINT('Ctrl Pts',(17.9169866041149,66.4064245271147,32.4822370510436));
#30672=CARTESIAN_POINT('Ctrl Pts',(19.2116652161993,67.9704451203549,32.3711039330519));
#30673=CARTESIAN_POINT('Ctrl Pts',(21.2278588509736,67.7310367834812,32.2599708150604));
#30674=CARTESIAN_POINT('Ctrl Pts',(22.120267737283,65.9073154494221,32.1488376970688));
#30675=CARTESIAN_POINT('Ctrl Pts',(21.0721241375063,64.16842266408,32.0377045790773));
#30676=CARTESIAN_POINT('Ctrl Pts',(19.0427303286889,64.1058615467534,31.9265714610857));
#30677=CARTESIAN_POINT('Ctrl Pts',(17.8894674008225,65.7768904944012,31.8154383430942));
#30678=CARTESIAN_POINT('Ctrl Pts',(18.667846977477,67.6521180430775,31.7043052251026));
#30679=CARTESIAN_POINT('Ctrl Pts',(20.6654654333766,68.0152621319967,31.5931721071111));
#30680=CARTESIAN_POINT('Ctrl Pts',(22.0540237321857,66.5339589977681,31.4820389891195));
#30681=CARTESIAN_POINT('Ctrl Pts',(21.5626586657121,64.5639555723606,31.3709058711279));
#30682=CARTESIAN_POINT('Ctrl Pts',(19.6410868827332,63.9082765292868,31.2597727531364));
#30683=CARTESIAN_POINT('Ctrl Pts',(18.0480065113594,65.167025136043,31.1486396351448));
#30684=CARTESIAN_POINT('Ctrl Pts',(18.2414674105046,67.1881451238641,31.0375065171532));
#30685=CARTESIAN_POINT('Ctrl Pts',(20.0444065507242,68.1218279293882,30.9263733991617));
#30686=CARTESIAN_POINT('Ctrl Pts',(21.8067030678963,67.1135302996029,30.8152402811701));
#30687=CARTESIAN_POINT('Ctrl Pts',(21.9154338261898,65.0860859114954,30.7041071631786));
#30688=CARTESIAN_POINT('Ctrl Pts',(20.2710841560138,63.8950916684954,30.592974045187));
#30689=CARTESIAN_POINT('Ctrl Pts',(18.3786275964855,64.630592378873,30.4818409271955));
#30690=CARTESIAN_POINT('Ctrl Pts',(17.9701148772496,66.6194288434647,30.3707078092039));
#30691=CARTESIAN_POINT('Ctrl Pts',(19.4194329178548,68.041339650036,30.2595746912123));
#30692=CARTESIAN_POINT('Ctrl Pts',(21.4001088029369,67.5949360625485,30.1484415732208));
#30693=CARTESIAN_POINT('Ctrl Pts',(22.0993500038257,65.688784214545,30.0373084552292));
#30694=CARTESIAN_POINT('Ctrl Pts',(20.8771834516022,64.0674693027239,29.9261753372377));
#30695=CARTESIAN_POINT('Ctrl Pts',(18.8521840788682,64.2148825487168,29.8150422192461));
#30696=CARTESIAN_POINT('Ctrl Pts',(17.8777110147484,65.9961055476625,29.7039091012546));
#30697=CARTESIAN_POINT('Ctrl Pts',(18.8456403624114,67.7808929026714,29.592775983263));
#30698=CARTESIAN_POINT('Ctrl Pts',(20.870085085548,67.935736977894,29.4816428652714));
#30699=CARTESIAN_POINT('Ctrl Pts',(22.0981936921759,66.318918381083,29.3705097472799));
#30700=CARTESIAN_POINT('Ctrl Pts',(21.4059528476254,64.4102131293996,29.2593766292883));
#30701=CARTESIAN_POINT('Ctrl Pts',(19.4269286191633,63.9565433950913,29.1482435112968));
#30702=CARTESIAN_POINT('Ctrl Pts',(17.9724018743126,65.3731255752635,29.0371103933052));
#30703=CARTESIAN_POINT('Ctrl Pts',(18.3736127395757,67.3634479024916,28.9259772753137));
#30704=CARTESIAN_POINT('Ctrl Pts',(20.2633572395576,68.1058890445728,28.8148441573221));
#30705=CARTESIAN_POINT('Ctrl Pts',(21.912066828257,66.9209376460759,28.7037110393305));
#30706=CARTESIAN_POINT('Ctrl Pts',(21.8107775975175,64.8931078661378,28.592577921339));
#30707=CARTESIAN_POINT('Ctrl Pts',(20.0521934380205,63.8783493339604,28.4814448033474));
#30708=CARTESIAN_POINT('Ctrl Pts',(18.2458397897289,64.8054089986984,28.3703116853558));
#30709=CARTESIAN_POINT('Ctrl Pts',(18.0449626089597,66.8258053664725,28.2591785673643));
#30710=CARTESIAN_POINT('Ctrl Pts',(19.633412597974,68.0903921594658,28.1480454493727));
#30711=CARTESIAN_POINT('Ctrl Pts',(21.5573778060989,67.441769771088,28.0369123313812));
#30712=CARTESIAN_POINT('Ctrl Pts',(22.0559695482155,65.4735829406938,27.9257792133896));
#30713=CARTESIAN_POINT('Ctrl Pts',(20.6728570377789,63.987193722573,27.814646095398));
#30714=CARTESIAN_POINT('Ctrl Pts',(18.6739192826801,64.3430040327909,27.7035129774065));
#30715=CARTESIAN_POINT('Ctrl Pts',(17.8886627946832,66.2153622710153,27.5923798594149));
#30716=CARTESIAN_POINT('Ctrl Pts',(19.035785217254,67.8906124820486,27.4812467414234));
#30717=CARTESIAN_POINT('Ctrl Pts',(21.0653949624323,67.8354997360908,27.3701136234318));
#30718=CARTESIAN_POINT('Ctrl Pts',(22.1199132998416,66.1004653863756,27.2589805054402));
#30719=CARTESIAN_POINT('Ctrl Pts',(21.2342035554597,64.2734811622086,27.1478473874487));
#30720=CARTESIAN_POINT('Ctrl Pts',(19.2189021210048,64.0266749306405,27.0367142694571));
#30721=CARTESIAN_POINT('Ctrl Pts',(17.9184922456775,65.5859334775838,26.9255811514656));
#30722=CARTESIAN_POINT('Ctrl Pts',(18.5231601215699,67.524161991947,26.814448033474));
#30723=CARTESIAN_POINT('Ctrl Pts',(20.4794901273535,68.0674174835658,26.7033149154825));
#30724=CARTESIAN_POINT('Ctrl Pts',(21.9969716063619,66.7184910761775,26.5921817974909));
#30725=CARTESIAN_POINT('Ctrl Pts',(21.6867466486893,64.7119734466258,26.4810486794993));
#30726=CARTESIAN_POINT('Ctrl Pts',(19.8327436171269,63.8843082349551,26.3699155615078));
#30727=CARTESIAN_POINT('Ctrl Pts',(18.1318225055817,64.9930077583167,26.2587824435162));
#30728=CARTESIAN_POINT('Ctrl Pts',(18.140726391805,67.0233455006932,26.1476493255247));
#30729=CARTESIAN_POINT('Ctrl Pts',(19.8513197870709,68.1170785885846,26.0365162075331));
#30730=CARTESIAN_POINT('Ctrl Pts',(21.6979729784046,67.2731751814378,25.9253830895416));
#30731=CARTESIAN_POINT('Ctrl Pts',(21.9906107258095,65.2640174051259,25.81424997155));
#30732=CARTESIAN_POINT('Ctrl Pts',(20.4612909038297,63.9284485666668,25.7031168535584));
#30733=CARTESIAN_POINT('Ctrl Pts',(18.5099235961124,64.4888676654707,25.5919837355669));
#30734=CARTESIAN_POINT('Ctrl Pts',(17.9220455664116,66.4322896353026,25.4808506175753));
#30735=CARTESIAN_POINT('Ctrl Pts',(19.2365660362622,67.9801527058252,25.3697174995838));
#30736=CARTESIAN_POINT('Ctrl Pts',(21.2486686077732,67.7155229855219,25.2585843815922));
#30737=CARTESIAN_POINT('Ctrl Pts',(22.1202282375515,65.8811425847956,25.1474512636007));
#30738=CARTESIAN_POINT('Ctrl Pts',(21.0465928843257,64.1547463487904,25.0363181456091));
#30739=CARTESIAN_POINT('Ctrl Pts',(19.6996852649168,64.1317394393838,24.9622294002814));
#30740=CARTESIAN_POINT('Ctrl Pts',(19.1702141221326,64.4076511362656,24.9251850276175));
#30741=CARTESIAN_POINT('Ctrl Pts',(19.5701357431142,64.3904122513351,36.2244449171475));
#30742=CARTESIAN_POINT('Ctrl Pts',(19.0349325071233,64.5333462053944,36.1874005444836));
#30743=CARTESIAN_POINT('Ctrl Pts',(18.1276317164724,65.3930098737417,36.1133117991559));
#30744=CARTESIAN_POINT('Ctrl Pts',(18.4746136995867,67.2471154732578,36.0021786811644));
#30745=CARTESIAN_POINT('Ctrl Pts',(20.2203904477277,67.9563337991017,35.8910455631728));
#30746=CARTESIAN_POINT('Ctrl Pts',(21.763119395253,66.8767205597329,35.7799124451812));
#30747=CARTESIAN_POINT('Ctrl Pts',(21.6928418415078,64.9938596198273,35.6687793271897));
#30748=CARTESIAN_POINT('Ctrl Pts',(20.0728729497283,64.0322781682749,35.5576462091981));
#30749=CARTESIAN_POINT('Ctrl Pts',(18.3863763237488,64.8714224386236,35.4465130912065));
#30750=CARTESIAN_POINT('Ctrl Pts',(18.1766470998833,66.7435910222386,35.335379973215));
#30751=CARTESIAN_POINT('Ctrl Pts',(19.6357646009513,67.9351428113835,35.2242468552234));
#30752=CARTESIAN_POINT('Ctrl Pts',(21.4282234153819,67.3556023297033,35.1131137372319));
#30753=CARTESIAN_POINT('Ctrl Pts',(21.9135266097828,65.5353478989816,35.0019806192403));
#30754=CARTESIAN_POINT('Ctrl Pts',(20.6474895861319,64.1403680514604,34.8908475012488));
#30755=CARTESIAN_POINT('Ctrl Pts',(18.7888472914304,64.447393201016,34.7797143832572));
#30756=CARTESIAN_POINT('Ctrl Pts',(18.0386982802614,66.1754268866989,34.6685812652656));
#30757=CARTESIAN_POINT('Ctrl Pts',(19.0836104741642,67.742902136399,34.5574481472741));
#30758=CARTESIAN_POINT('Ctrl Pts',(20.9672380922293,67.7152051745302,34.4463150292825));
#30759=CARTESIAN_POINT('Ctrl Pts',(21.9656115080195,66.1176847146236,34.335181911291));
#30760=CARTESIAN_POINT('Ctrl Pts',(21.1649798207563,64.4124546784534,34.2240487932994));
#30761=CARTESIAN_POINT('Ctrl Pts',(19.2981127911139,64.1602085522744,34.1129156753079));
#30762=CARTESIAN_POINT('Ctrl Pts',(18.073640539619,65.5918119993568,34.0017825573163));
#30763=CARTESIAN_POINT('Ctrl Pts',(18.6122482977868,67.3970051572994,33.8906494393248));
#30764=CARTESIAN_POINT('Ctrl Pts',(20.4209810298014,67.9236042164417,33.7795163213331));
#30765=CARTESIAN_POINT('Ctrl Pts',(21.8444153563953,66.689644980988,33.6683832033417));
#30766=CARTESIAN_POINT('Ctrl Pts',(21.5797681519781,64.8244955164696,33.55725008535));
#30767=CARTESIAN_POINT('Ctrl Pts',(19.8692549564828,64.0352140218324,33.4461169673585));
#30768=CARTESIAN_POINT('Ctrl Pts',(18.2784047705477,65.0441819880638,33.3349838493669));
#30769=CARTESIAN_POINT('Ctrl Pts',(18.2632263001066,66.9279522192353,33.2238507313754));
#30770=CARTESIAN_POINT('Ctrl Pts',(19.8376114784687,67.9624240556267,33.1127176133838));
#30771=CARTESIAN_POINT('Ctrl Pts',(21.5606210233293,67.2008081559964,33.0015844953923));
#30772=CARTESIAN_POINT('Ctrl Pts',(21.8552887821724,65.3401653686769,32.8904513774007));
#30773=CARTESIAN_POINT('Ctrl Pts',(20.4519232241273,64.0834292067686,32.7793182594091));
#30774=CARTESIAN_POINT('Ctrl Pts',(18.6349397438307,64.5808140703239,32.6681851414176));
#30775=CARTESIAN_POINT('Ctrl Pts',(18.0673131382311,66.3770937553291,32.557052023426));
#30776=CARTESIAN_POINT('Ctrl Pts',(19.2685576183346,67.8282423931933,32.4459189054345));
#30777=CARTESIAN_POINT('Ctrl Pts',(21.1392469554306,67.6061116338867,32.3347857874429));
#30778=CARTESIAN_POINT('Ctrl Pts',(21.9672526385929,65.9140042913095,32.2236526694513));
#30779=CARTESIAN_POINT('Ctrl Pts',(20.9947512766059,64.3006036060839,32.1125195514598));
#30780=CARTESIAN_POINT('Ctrl Pts',(19.1118143932403,64.2425573881604,32.0013864334682));
#30781=CARTESIAN_POINT('Ctrl Pts',(18.0417799358261,65.79299182086,31.8902533154767));
#30782=CARTESIAN_POINT('Ctrl Pts',(18.7639855559345,67.5328882868707,31.7791201974851));
#30783=CARTESIAN_POINT('Ctrl Pts',(20.6174402443061,67.8698250588426,31.6679870794936));
#30784=CARTESIAN_POINT('Ctrl Pts',(21.9057893188776,66.4954243413644,31.556853961502));
#30785=CARTESIAN_POINT('Ctrl Pts',(21.4498849976757,64.6675917669575,31.4457208435104));
#30786=CARTESIAN_POINT('Ctrl Pts',(19.6669888596835,64.0592316505081,31.3345877255189));
#30787=CARTESIAN_POINT('Ctrl Pts',(18.1888776244998,65.2271391154115,31.2234546075273));
#30788=CARTESIAN_POINT('Ctrl Pts',(18.3683768724559,67.1023992813984,31.1123214895357));
#30789=CARTESIAN_POINT('Ctrl Pts',(20.0412018268009,67.9687002350364,31.0011883715442));
#30790=CARTESIAN_POINT('Ctrl Pts',(21.6763172475696,67.0331692462831,30.8900552535526));
#30791=CARTESIAN_POINT('Ctrl Pts',(21.7772011441587,65.1520410981861,30.7789221355611));
#30792=CARTESIAN_POINT('Ctrl Pts',(20.2515206036584,64.0469983123664,30.6677890175695));
#30793=CARTESIAN_POINT('Ctrl Pts',(18.4956385069354,64.7294195404663,30.556655899578));
#30794=CARTESIAN_POINT('Ctrl Pts',(18.1166072597565,66.574726014691,30.4455227815864));
#30795=CARTESIAN_POINT('Ctrl Pts',(19.4613311780644,67.8940206192749,30.3343896635949));
#30796=CARTESIAN_POINT('Ctrl Pts',(21.2990660040059,67.4798330051734,30.2232565456033));
#30797=CARTESIAN_POINT('Ctrl Pts',(21.9478444923416,65.7112439790775,30.1121234276117));
#30798=CARTESIAN_POINT('Ctrl Pts',(20.8138790348741,64.2069358286563,30.0009903096202));
#30799=CARTESIAN_POINT('Ctrl Pts',(18.9350194507232,64.3437105821668,29.8898571916286));
#30800=CARTESIAN_POINT('Ctrl Pts',(18.0308719824964,65.9963866017945,29.7787240736371));
#30801=CARTESIAN_POINT('Ctrl Pts',(18.9289479800125,67.6523697456819,29.6675909556455));
#30802=CARTESIAN_POINT('Ctrl Pts',(20.8072929424178,67.7960390616817,29.5564578376539));
#30803=CARTESIAN_POINT('Ctrl Pts',(21.9467716291819,66.2959027370219,29.4453247196624));
#30804=CARTESIAN_POINT('Ctrl Pts',(21.3044882967339,64.5249445808212,29.3341916016708));
#30805=CARTESIAN_POINT('Ctrl Pts',(19.4682859309562,64.1040152018687,29.2230584836793));
#30806=CARTESIAN_POINT('Ctrl Pts',(18.118729209229,65.4183657354002,29.1119253656877));
#30807=CARTESIAN_POINT('Ctrl Pts',(18.4909855613124,67.2650508407951,29.0007922476961));
#30808=CARTESIAN_POINT('Ctrl Pts',(20.2443513219119,67.9539116247784,28.8896591297046));
#30809=CARTESIAN_POINT('Ctrl Pts',(21.7740771351238,66.8544755845523,28.778526011713));
#30810=CARTESIAN_POINT('Ctrl Pts',(21.6800977272738,64.9729898575127,28.6673928937215));
#30811=CARTESIAN_POINT('Ctrl Pts',(20.0484267514227,64.0314642356028,28.5562597757298));
#30812=CARTESIAN_POINT('Ctrl Pts',(18.3724337066069,64.8916200260816,28.4451266577384));
#30813=CARTESIAN_POINT('Ctrl Pts',(18.1860533938981,66.7662087941021,28.3339935397467));
#30814=CARTESIAN_POINT('Ctrl Pts',(19.6598684113193,67.9395331160738,28.2228604217553));
#30815=CARTESIAN_POINT('Ctrl Pts',(21.4449852461841,67.3377203909403,28.1117273037636));
#30816=CARTESIAN_POINT('Ctrl Pts',(21.907594709608,65.5115733118462,28.0005941857721));
#30817=CARTESIAN_POINT('Ctrl Pts',(20.6242984127384,64.1324535620588,27.8894610677805));
#30818=CARTESIAN_POINT('Ctrl Pts',(18.7696196361136,64.4625858181443,27.778327949789));
#30819=CARTESIAN_POINT('Ctrl Pts',(18.0410333963571,66.1998200455812,27.6671948317974));
#30820=CARTESIAN_POINT('Ctrl Pts',(19.1053704953516,67.7541711022934,27.5560617138059));
#30821=CARTESIAN_POINT('Ctrl Pts',(20.9885077314219,67.7030357230207,27.4449285958143));
#30822=CARTESIAN_POINT('Ctrl Pts',(21.9669237801287,66.0932150185373,27.3337954778227));
#30823=CARTESIAN_POINT('Ctrl Pts',(21.1451337764306,64.3980802615155,27.2226623598312));
#30824=CARTESIAN_POINT('Ctrl Pts',(19.2752722515027,64.1690854974412,27.1115292418396));
#30825=CARTESIAN_POINT('Ctrl Pts',(18.0687101209256,65.6158157555045,27.0003961238481));
#30826=CARTESIAN_POINT('Ctrl Pts',(18.6297404348831,67.414166544902,26.8892630058565));
#30827=CARTESIAN_POINT('Ctrl Pts',(20.4448863705412,67.9182164724299,26.778129887865));
#30828=CARTESIAN_POINT('Ctrl Pts',(21.8528545205544,66.6666391421051,26.6669967698734));
#30829=CARTESIAN_POINT('Ctrl Pts',(21.5650178215341,64.8049275140365,26.5558636518819));
#30830=CARTESIAN_POINT('Ctrl Pts',(19.8448141455237,64.0369930957082,26.4447305338902));
#30831=CARTESIAN_POINT('Ctrl Pts',(18.2666448012062,65.0656801923361,26.3335974158987));
#30832=CARTESIAN_POINT('Ctrl Pts',(18.2749061133784,66.9494928876345,26.2224642979072));
#30833=CARTESIAN_POINT('Ctrl Pts',(19.8620497137941,67.9642936438011,26.1113311799156));
#30834=CARTESIAN_POINT('Ctrl Pts',(21.5754339715164,67.1812929051517,26.000198061924));
#30835=CARTESIAN_POINT('Ctrl Pts',(21.8469526908796,65.3171316639569,25.8890649439325));
#30836=CARTESIAN_POINT('Ctrl Pts',(20.42800054529,64.0779479159419,25.7779318259409));
#30837=CARTESIAN_POINT('Ctrl Pts',(18.6174591606014,64.5979227905551,25.6667987079493));
#30838=CARTESIAN_POINT('Ctrl Pts',(18.0720070062515,66.4010922350662,25.5556655899578));
#30839=CARTESIAN_POINT('Ctrl Pts',(19.2916614005177,67.8372494033905,25.4445324719663));
#30840=CARTESIAN_POINT('Ctrl Pts',(21.1585549174642,67.5917174328935,25.3333993539747));
#30841=CARTESIAN_POINT('Ctrl Pts',(21.9672159894709,65.8897202652449,25.2222662359831));
#30842=CARTESIAN_POINT('Ctrl Pts',(20.9710625582884,64.2879142806432,25.1111331179916));
#30843=CARTESIAN_POINT('Ctrl Pts',(19.7213583244172,64.2665677297147,25.0370443726639));
#30844=CARTESIAN_POINT('Ctrl Pts',(19.2300979593296,64.5225674811446,25.));
#30845=CARTESIAN_POINT('Ctrl Pts',(18.3361559304958,66.0009441564151,35.3785196366098));
#30846=CARTESIAN_POINT('Ctrl Pts',(18.3350370261301,66.2166368244897,35.3641397488115));
#30847=CARTESIAN_POINT('Ctrl Pts',(18.3739569457115,66.4319423497591,35.3497598610133));
#30848=CARTESIAN_POINT('Ctrl Pts',(18.4547882207056,66.630154889827,35.335379973215));
#30849=CARTESIAN_POINT('Ctrl Pts',(18.6630196002393,67.1407749519536,35.2983356005512));
#30850=CARTESIAN_POINT('Ctrl Pts',(19.1493921005953,67.5379588816685,35.2612912278873));
#30851=CARTESIAN_POINT('Ctrl Pts',(19.6913214865117,67.639960766246,35.2242468552234));
#30852=CARTESIAN_POINT('Ctrl Pts',(20.2332508724282,67.7419626508234,35.1872024825596));
#30853=CARTESIAN_POINT('Ctrl Pts',(20.830737143905,67.5487824902634,35.1501581098958));
#30854=CARTESIAN_POINT('Ctrl Pts',(21.2103641453769,67.1488166715297,35.1131137372319));
#30855=CARTESIAN_POINT('Ctrl Pts',(21.5899911468489,66.7488508527961,35.076069364568));
#30856=CARTESIAN_POINT('Ctrl Pts',(21.7517588783158,66.1420993758888,35.0390249919042));
#30857=CARTESIAN_POINT('Ctrl Pts',(21.6216365734408,65.6062269961817,35.0019806192403));
#30858=CARTESIAN_POINT('Ctrl Pts',(21.4915142685658,65.0703546164746,34.9649362465764));
#30859=CARTESIAN_POINT('Ctrl Pts',(21.0695019273488,64.6053613339675,34.9278918739126));
#30860=CARTESIAN_POINT('Ctrl Pts',(20.5487220409568,64.4240355509732,34.8908475012488));
#30861=CARTESIAN_POINT('Ctrl Pts',(20.0279421545647,64.2427097679789,34.8538031285849));
#30862=CARTESIAN_POINT('Ctrl Pts',(19.4083947229975,64.3450514844974,34.8167587559211));
#30863=CARTESIAN_POINT('Ctrl Pts',(18.9735961720191,64.6842279570372,34.7797143832572));
#30864=CARTESIAN_POINT('Ctrl Pts',(18.5776806249338,64.9930726815236,34.7459828010414));
#30865=CARTESIAN_POINT('Ctrl Pts',(18.3349481418111,65.4982870590469,34.7122512188256));
#30866=CARTESIAN_POINT('Ctrl Pts',(18.3317911471719,66.0008588710395,34.6785196366098));
#30867=CARTESIAN_POINT('Ctrl Pts',(19.4698297828115,64.0148256743282,36.));
#30868=CARTESIAN_POINT('Ctrl Pts',(19.4011650087939,64.0402496944362,36.));
#30869=CARTESIAN_POINT('Ctrl Pts',(19.3342035794783,64.0695633948039,36.));
#30870=CARTESIAN_POINT('Ctrl Pts',(19.2691344316336,64.1024727495347,36.));
#30871=CARTESIAN_POINT('Ctrl Pts',(19.202254333301,64.1362980100978,36.));
#30872=CARTESIAN_POINT('Ctrl Pts',(19.1373725394216,64.1739225412136,36.));
#30873=CARTESIAN_POINT('Ctrl Pts',(19.0747254199949,64.2150717234713,36.));
#30874=CARTESIAN_POINT('Ctrl Pts',(19.0217926982225,64.2498400932789,36.));
#30875=CARTESIAN_POINT('Ctrl Pts',(18.9704556772988,64.2871258137782,36.));
#30876=CARTESIAN_POINT('Ctrl Pts',(18.9208796779014,64.3267812441764,36.));
#30877=CARTESIAN_POINT('Ctrl Pts',(18.8988500225955,64.3444025825921,36.));
#30878=CARTESIAN_POINT('Ctrl Pts',(18.8771683964782,64.3624920156554,36.));
#30879=CARTESIAN_POINT('Ctrl Pts',(18.8558508586253,64.381037312981,36.));
#30880=CARTESIAN_POINT('Ctrl Pts',(18.8441382800365,64.3912267285635,36.));
#30881=CARTESIAN_POINT('Ctrl Pts',(18.8325356292319,64.401553765981,36.));
#30882=CARTESIAN_POINT('Ctrl Pts',(18.8210457040405,64.4120164383406,36.));
#30883=CARTESIAN_POINT('Ctrl Pts',(18.8104521548357,64.421662874902,36.));
#30884=CARTESIAN_POINT('Ctrl Pts',(18.799952995123,64.4314261244654,36.));
#30885=CARTESIAN_POINT('Ctrl Pts',(18.7895663054278,64.4412891742485,36.));
#30886=CARTESIAN_POINT('Ctrl Pts',(18.7364815316182,64.4916977049905,36.));
#30887=CARTESIAN_POINT('Ctrl Pts',(18.6862367517015,64.5447946360434,36.));
#30888=CARTESIAN_POINT('Ctrl Pts',(18.63905063298,64.6003205030525,36.));
#30889=CARTESIAN_POINT('Ctrl Pts',(18.5922306751828,64.6554154932839,36.));
#30890=CARTESIAN_POINT('Ctrl Pts',(18.5484215844064,64.7129027523719,36.));
#30891=CARTESIAN_POINT('Ctrl Pts',(18.5078817685123,64.7725530493182,36.));
#30892=CARTESIAN_POINT('Ctrl Pts',(18.4741933336872,64.8221222221587,36.));
#30893=CARTESIAN_POINT('Ctrl Pts',(18.4427631560478,64.8731857427967,36.));
#30894=CARTESIAN_POINT('Ctrl Pts',(18.4137671253403,64.9256185424461,36.));
#30895=CARTESIAN_POINT('Ctrl Pts',(18.4016609562457,64.9475098262932,36.));
#30896=CARTESIAN_POINT('Ctrl Pts',(18.389979418784,64.9696398359853,36.));
#30897=CARTESIAN_POINT('Ctrl Pts',(18.3787367554887,64.991999552123,36.));
#30898=CARTESIAN_POINT('Ctrl Pts',(18.3735359303309,65.0023430953879,36.));
#30899=CARTESIAN_POINT('Ctrl Pts',(18.3684290349839,65.0127357949179,36.));
#30900=CARTESIAN_POINT('Ctrl Pts',(18.3634175445956,65.0231767558657,36.));
#30901=CARTESIAN_POINT('Ctrl Pts',(18.358185554435,65.0340771070014,36.));
#30902=CARTESIAN_POINT('Ctrl Pts',(18.3530611587919,65.0450226072079,36.));
#30903=CARTESIAN_POINT('Ctrl Pts',(18.3480474161898,65.0560079490254,36.));
#30904=CARTESIAN_POINT('Ctrl Pts',(18.31950701775,65.1185412813777,36.));
#30905=CARTESIAN_POINT('Ctrl Pts',(18.2945275906019,65.1824076820533,36.));
#30906=CARTESIAN_POINT('Ctrl Pts',(18.2733325947284,65.2474026988709,36.));
#30907=CARTESIAN_POINT('Ctrl Pts',(18.2541301194199,65.3062875985454,36.));
#30908=CARTESIAN_POINT('Ctrl Pts',(18.2380343018762,65.36609948651,36.));
#30909=CARTESIAN_POINT('Ctrl Pts',(18.2252480174595,65.4266911450279,36.));
#30910=CARTESIAN_POINT('Ctrl Pts',(18.2101155115003,65.4984010807457,36.));
#30911=CARTESIAN_POINT('Ctrl Pts',(18.1996179357092,65.5712047291577,36.));
#30912=CARTESIAN_POINT('Ctrl Pts',(18.1936801509955,65.6446789881755,36.));
#30913=CARTESIAN_POINT('Ctrl Pts',(18.1923733282017,65.6608496378493,36.));
#30914=CARTESIAN_POINT('Ctrl Pts',(18.1912875955242,65.6770526886534,36.));
#30915=CARTESIAN_POINT('Ctrl Pts',(18.1904225212166,65.6932834657235,36.));
#30916=CARTESIAN_POINT('Ctrl Pts',(18.1895271920146,65.7100818939691,36.));
#30917=CARTESIAN_POINT('Ctrl Pts',(18.1888682156112,65.7269162162858,36.));
#30918=CARTESIAN_POINT('Ctrl Pts',(18.1884456743354,65.7437469754922,36.));
#30919=CARTESIAN_POINT('Ctrl Pts',(18.1867244318773,65.8123078925095,36.));
#30920=CARTESIAN_POINT('Ctrl Pts',(18.1889147956501,65.8808963864675,36.));
#30921=CARTESIAN_POINT('Ctrl Pts',(18.1948961812499,65.9491741310747,36.));
#30922=CARTESIAN_POINT('Ctrl Pts',(18.2008763308016,66.0174377661452,36.));
#30923=CARTESIAN_POINT('Ctrl Pts',(18.2106463891817,66.0853918518815,36.));
#30924=CARTESIAN_POINT('Ctrl Pts',(18.224135451783,66.1526832386545,36.));
#30925=CARTESIAN_POINT('Ctrl Pts',(18.2338954440545,66.2013718269017,36.));
#30926=CARTESIAN_POINT('Ctrl Pts',(18.2456034689683,66.2497132117657,36.));
#30927=CARTESIAN_POINT('Ctrl Pts',(18.2592468713223,66.297563972578,36.));
#30928=CARTESIAN_POINT('Ctrl Pts',(18.2694832221723,66.3334653675088,36.));
#30929=CARTESIAN_POINT('Ctrl Pts',(18.2808092805504,66.369090426564,36.));
#30930=CARTESIAN_POINT('Ctrl Pts',(18.2932236165998,66.4043744002987,36.));
#30931=CARTESIAN_POINT('Ctrl Pts',(18.2973531525319,66.4161113499661,36.));
#30932=CARTESIAN_POINT('Ctrl Pts',(18.301599913114,66.4278013646143,36.));
#30933=CARTESIAN_POINT('Ctrl Pts',(18.305963253358,66.4394418832697,36.));
#30934=CARTESIAN_POINT('Ctrl Pts',(18.32908720388,66.5011319561002,36.));
#30935=CARTESIAN_POINT('Ctrl Pts',(18.3554837407933,66.5614384947313,36.));
#30936=CARTESIAN_POINT('Ctrl Pts',(18.3851028692742,66.6200274070333,36.));
#30937=CARTESIAN_POINT('Ctrl Pts',(18.4059351993179,66.6612353567799,36.));
#30938=CARTESIAN_POINT('Ctrl Pts',(18.4283625607903,66.7015930886865,36.));
#30939=CARTESIAN_POINT('Ctrl Pts',(18.4523779599159,66.7409730135987,36.));
#30940=CARTESIAN_POINT('Ctrl Pts',(18.4600909786022,66.7536206525209,36.));
#30941=CARTESIAN_POINT('Ctrl Pts',(18.4679689605213,66.7661690371134,36.));
#30942=CARTESIAN_POINT('Ctrl Pts',(18.476008349553,66.7786083058229,36.));
#30943=CARTESIAN_POINT('Ctrl Pts',(18.5102528592992,66.8315945037637,36.));
#30944=CARTESIAN_POINT('Ctrl Pts',(18.5473531312327,66.882496911613,36.));
#30945=CARTESIAN_POINT('Ctrl Pts',(18.5872749277835,66.9310003064575,36.));
#30946=CARTESIAN_POINT('Ctrl Pts',(18.6240617394812,66.9756948194054,36.));
#30947=CARTESIAN_POINT('Ctrl Pts',(18.6632449234927,67.0183523994197,36.));
#30948=CARTESIAN_POINT('Ctrl Pts',(18.7048191306495,67.0586935104123,36.));
#30949=CARTESIAN_POINT('Ctrl Pts',(18.7126374799383,67.066279966487,36.));
#30950=CARTESIAN_POINT('Ctrl Pts',(18.7205404424604,67.0737843957438,36.));
#30951=CARTESIAN_POINT('Ctrl Pts',(18.7285264260868,67.0812061322332,36.));
#30952=CARTESIAN_POINT('Origin',(20.,66.,30.));
#30953=CARTESIAN_POINT('Origin',(-20.,66.,25.));
#30954=CARTESIAN_POINT('Ctrl Pts',(-20.7699020406705,64.5225674811446,25.));
#30955=CARTESIAN_POINT('Ctrl Pts',(-20.7181607868987,64.4874948453559,25.));
#30956=CARTESIAN_POINT('Ctrl Pts',(-20.6644430498644,64.4556772957763,25.));
#30957=CARTESIAN_POINT('Ctrl Pts',(-20.609080128741,64.4270507909171,25.));
#30958=CARTESIAN_POINT('Ctrl Pts',(-20.5739699369606,64.408896364539,25.));
#30959=CARTESIAN_POINT('Ctrl Pts',(-20.5381971797729,64.3920259834258,25.));
#30960=CARTESIAN_POINT('Ctrl Pts',(-20.501838755596,64.3764305264031,25.));
#30961=CARTESIAN_POINT('Ctrl Pts',(-20.4770533105217,64.3657991431075,25.));
#30962=CARTESIAN_POINT('Ctrl Pts',(-20.4519955812217,64.3557603488702,25.));
#30963=CARTESIAN_POINT('Ctrl Pts',(-20.4266886866948,64.3463128385714,25.));
#30964=CARTESIAN_POINT('Ctrl Pts',(-20.4131995684787,64.3412771127089,25.));
#30965=CARTESIAN_POINT('Ctrl Pts',(-20.3996397067877,64.3364095523361,25.));
#30966=CARTESIAN_POINT('Ctrl Pts',(-20.3860263063337,64.3317144816325,25.));
#30967=CARTESIAN_POINT('Ctrl Pts',(-20.3236619057568,64.3102058753821,25.));
#30968=CARTESIAN_POINT('Ctrl Pts',(-20.2601062052714,64.2922869409266,25.));
#30969=CARTESIAN_POINT('Ctrl Pts',(-20.1957090968652,64.277911135731,25.));
#30970=CARTESIAN_POINT('Ctrl Pts',(-20.1492566725938,64.2675412446177,25.));
#30971=CARTESIAN_POINT('Ctrl Pts',(-20.1023655335798,64.2590157983247,25.));
#30972=CARTESIAN_POINT('Ctrl Pts',(-20.055157896439,64.2523313578685,25.));
#30973=CARTESIAN_POINT('Ctrl Pts',(-20.0422585355377,64.2505048523476,25.));
#30974=CARTESIAN_POINT('Ctrl Pts',(-20.029335510413,64.2488158742319,25.));
#30975=CARTESIAN_POINT('Ctrl Pts',(-20.0163912478524,64.2472645140858,25.));
#30976=CARTESIAN_POINT('Ctrl Pts',(-20.0030607156547,64.2456668598138,25.));
#30977=CARTESIAN_POINT('Ctrl Pts',(-19.98971558118,64.2442161491718,25.));
#30978=CARTESIAN_POINT('Ctrl Pts',(-19.9763641001265,64.2429124587624,25.));
#30979=CARTESIAN_POINT('Ctrl Pts',(-19.9088329220123,64.2363184525327,25.));
#30980=CARTESIAN_POINT('Ctrl Pts',(-19.8410980617049,64.2334768385416,25.));
#30981=CARTESIAN_POINT('Ctrl Pts',(-19.7735141943155,64.234339667057,25.));
#30982=CARTESIAN_POINT('Ctrl Pts',(-19.7049517537314,64.2352149888032,25.));
#30983=CARTESIAN_POINT('Ctrl Pts',(-19.6365437003715,64.2399024721089,25.));
#30984=CARTESIAN_POINT('Ctrl Pts',(-19.5686388483405,64.2484003486578,25.));
#30985=CARTESIAN_POINT('Ctrl Pts',(-19.5265709671915,64.2536648864631,25.));
#30986=CARTESIAN_POINT('Ctrl Pts',(-19.4846958449925,64.26039280583,25.));
#30987=CARTESIAN_POINT('Ctrl Pts',(-19.4430950409565,64.2685936305935,25.));
#30988=CARTESIAN_POINT('Ctrl Pts',(-19.4090314604675,64.275308631923,25.));
#30989=CARTESIAN_POINT('Ctrl Pts',(-19.3751517611351,64.2830113026909,25.));
#30990=CARTESIAN_POINT('Ctrl Pts',(-19.3415010618013,64.2917108536401,25.));
#30991=CARTESIAN_POINT('Ctrl Pts',(-19.3277178667536,64.2952741557389,25.));
#30992=CARTESIAN_POINT('Ctrl Pts',(-19.3139706268034,64.2990055872543,25.));
#30993=CARTESIAN_POINT('Ctrl Pts',(-19.3002856997927,64.3028989400252,25.));
#30994=CARTESIAN_POINT('Ctrl Pts',(-19.232490402017,64.3221866578365,25.));
#30995=CARTESIAN_POINT('Ctrl Pts',(-19.1661047027307,64.3454735719371,25.));
#30996=CARTESIAN_POINT('Ctrl Pts',(-19.1014913319554,64.3727409719143,25.));
#30997=CARTESIAN_POINT('Ctrl Pts',(-19.0943245786266,64.3757654036567,25.));
#30998=CARTESIAN_POINT('Ctrl Pts',(-19.0871796217495,64.378838858274,25.));
#30999=CARTESIAN_POINT('Ctrl Pts',(-19.080056952154,64.3819613496012,25.));
#31000=CARTESIAN_POINT('Ctrl Pts',(-19.0183043681621,64.4090329279418,25.));
#31001=CARTESIAN_POINT('Ctrl Pts',(-18.9582262212172,64.4397861035812,25.));
#31002=CARTESIAN_POINT('Ctrl Pts',(-18.8999644475876,64.4739106753168,25.));
#31003=CARTESIAN_POINT('Ctrl Pts',(-18.8372885650046,64.5106206399824,25.));
#31004=CARTESIAN_POINT('Ctrl Pts',(-18.7767137054592,64.5512322190085,25.));
#31005=CARTESIAN_POINT('Ctrl Pts',(-18.7184364558154,64.5954203083505,25.));
#31006=CARTESIAN_POINT('Ctrl Pts',(-18.7079112053861,64.6034009647672,25.));
#31007=CARTESIAN_POINT('Ctrl Pts',(-18.6974609734778,64.6114984307375,25.));
#31008=CARTESIAN_POINT('Ctrl Pts',(-18.6870870232366,64.6197109799285,25.));
#31009=CARTESIAN_POINT('Ctrl Pts',(-18.6779109752736,64.6269752084551,25.));
#31010=CARTESIAN_POINT('Ctrl Pts',(-18.6688016088713,64.6343239571117,25.));
#31011=CARTESIAN_POINT('Ctrl Pts',(-18.6597615752311,64.6417539289658,25.));
#31012=CARTESIAN_POINT('Ctrl Pts',(-18.6048583606212,64.6868786879536,25.));
#31013=CARTESIAN_POINT('Ctrl Pts',(-18.5524872699802,64.7350141921525,25.));
#31014=CARTESIAN_POINT('Ctrl Pts',(-18.5027983210669,64.7858104381237,25.));
#31015=CARTESIAN_POINT('Ctrl Pts',(-18.4520616126594,64.8376777924631,25.));
#31016=CARTESIAN_POINT('Ctrl Pts',(-18.4041205870664,64.8923198235062,25.));
#31017=CARTESIAN_POINT('Ctrl Pts',(-18.3591551614209,64.9494152063453,25.));
#31018=CARTESIAN_POINT('Ctrl Pts',(-18.3139169717322,65.0068569345651,25.));
#31019=CARTESIAN_POINT('Ctrl Pts',(-18.2716898043235,65.0667825982523,25.));
#31020=CARTESIAN_POINT('Ctrl Pts',(-18.2326888228849,65.1289065313088,25.));
#31021=CARTESIAN_POINT('Ctrl Pts',(-18.2230617875061,65.1442412557014,25.));
#31022=CARTESIAN_POINT('Ctrl Pts',(-18.2136315088657,65.15971008858,25.));
#31023=CARTESIAN_POINT('Ctrl Pts',(-18.2044016076695,65.1753090388636,25.));
#31024=CARTESIAN_POINT('Ctrl Pts',(-18.1971519546457,65.1875612802137,25.));
#31025=CARTESIAN_POINT('Ctrl Pts',(-18.190025183174,65.1998953465914,25.));
#31026=CARTESIAN_POINT('Ctrl Pts',(-18.1830335133096,65.2122902250167,25.));
#31027=CARTESIAN_POINT('Ctrl Pts',(-18.1460182981017,65.2779110425448,25.));
#31028=CARTESIAN_POINT('Ctrl Pts',(-18.1127171633531,65.3453488100055,25.));
#31029=CARTESIAN_POINT('Ctrl Pts',(-18.0833108421231,65.4142572038605,25.));
#31030=CARTESIAN_POINT('Ctrl Pts',(-18.0538724456395,65.4832407602693,25.));
#31031=CARTESIAN_POINT('Ctrl Pts',(-18.0283365989439,65.5536989822687,25.));
#31032=CARTESIAN_POINT('Ctrl Pts',(-18.0069203644551,65.625322123177,25.));
#31033=CARTESIAN_POINT('Ctrl Pts',(-17.9859913623068,65.6953157941337,25.));
#31034=CARTESIAN_POINT('Ctrl Pts',(-17.9689961000931,65.7664228590063,25.));
#31035=CARTESIAN_POINT('Ctrl Pts',(-17.9561807640613,65.8383774456246,25.));
#31036=CARTESIAN_POINT('Ctrl Pts',(-17.9534319160524,65.853811471051,25.));
#31037=CARTESIAN_POINT('Ctrl Pts',(-17.9508755620075,65.869284549427,25.));
#31038=CARTESIAN_POINT('Ctrl Pts',(-17.9485144392445,65.8847941411762,25.));
#31039=CARTESIAN_POINT('Ctrl Pts',(-17.946501247731,65.8980182644525,25.));
#31040=CARTESIAN_POINT('Ctrl Pts',(-17.9446299912251,65.9112689334149,25.));
#31041=CARTESIAN_POINT('Ctrl Pts',(-17.9428998421776,65.9245444497166,25.));
#31042=CARTESIAN_POINT('Ctrl Pts',(-18.1825721112406,66.9586205879593,25.));
#31043=CARTESIAN_POINT('Ctrl Pts',(-18.2234186096542,67.0211003824849,25.));
#31044=CARTESIAN_POINT('Ctrl Pts',(-18.267861786798,67.0810294578375,25.));
#31045=CARTESIAN_POINT('Ctrl Pts',(-18.3155727964654,67.1382580395458,25.));
#31046=CARTESIAN_POINT('Ctrl Pts',(-18.362032339418,67.193985507242,25.));
#31047=CARTESIAN_POINT('Ctrl Pts',(-18.4115915278402,67.2471524989451,25.));
#31048=CARTESIAN_POINT('Ctrl Pts',(-18.463972782879,67.297583049384,25.));
#31049=CARTESIAN_POINT('Ctrl Pts',(-18.4756644509254,67.3088393137612,25.));
#31050=CARTESIAN_POINT('Ctrl Pts',(-18.4874983796361,67.3199605477055,25.));
#31051=CARTESIAN_POINT('Ctrl Pts',(-18.499466497088,67.330939853898,25.));
#31052=CARTESIAN_POINT('Ctrl Pts',(-18.5543876416691,67.3813233887536,25.));
#31053=CARTESIAN_POINT('Ctrl Pts',(-18.6120225103212,67.4286224459823,25.));
#31054=CARTESIAN_POINT('Ctrl Pts',(-18.6720549591814,67.4726645370967,25.));
#31055=CARTESIAN_POINT('Ctrl Pts',(-18.7141994128617,67.503583313595,25.));
#31056=CARTESIAN_POINT('Ctrl Pts',(-18.7575261800742,67.532896022068,25.));
#31057=CARTESIAN_POINT('Ctrl Pts',(-18.8019312037584,67.5605285808541,25.));
#31058=CARTESIAN_POINT('Ctrl Pts',(-18.8188066330934,67.5710298992737,25.));
#31059=CARTESIAN_POINT('Ctrl Pts',(-18.8358378192095,67.5812884311884,25.));
#31060=CARTESIAN_POINT('Ctrl Pts',(-18.8530191260934,67.5912996232851,25.));
#31061=CARTESIAN_POINT('Ctrl Pts',(-18.8694037899796,67.6008466279871,25.));
#31062=CARTESIAN_POINT('Ctrl Pts',(-18.8859302919879,67.6101714338832,25.));
#31063=CARTESIAN_POINT('Ctrl Pts',(-18.9025641525663,67.6192541843043,25.));
#31064=CARTESIAN_POINT('Ctrl Pts',(-18.9662810595884,67.6540461534543,25.));
#31065=CARTESIAN_POINT('Ctrl Pts',(-19.0316369227313,67.6853309714246,25.));
#31066=CARTESIAN_POINT('Ctrl Pts',(-19.0983400435049,67.7129470016749,25.));
#31067=CARTESIAN_POINT('Ctrl Pts',(-19.1636108196435,67.739970021099,25.));
#31068=CARTESIAN_POINT('Ctrl Pts',(-19.2301725386384,67.7634802778805,25.));
#31069=CARTESIAN_POINT('Ctrl Pts',(-19.2977604960306,67.7832780673405,25.));
#31070=CARTESIAN_POINT('Ctrl Pts',(-19.363866135499,67.8026416578796,25.));
#31071=CARTESIAN_POINT('Ctrl Pts',(-19.4309542545466,67.8184539478542,25.));
#31072=CARTESIAN_POINT('Ctrl Pts',(-19.4987732524779,67.8304795008119,25.));
#31073=CARTESIAN_POINT('Ctrl Pts',(-19.5208334683506,67.8343911819386,25.));
#31074=CARTESIAN_POINT('Ctrl Pts',(-19.5429709379166,67.8379018005825,25.));
#31075=CARTESIAN_POINT('Ctrl Pts',(-19.5651767076627,67.8410020802634,25.));
#31076=CARTESIAN_POINT('Ctrl Pts',(-19.577661186311,67.8427451126339,25.));
#31077=CARTESIAN_POINT('Ctrl Pts',(-19.5901685388999,67.8443584849207,25.));
#31078=CARTESIAN_POINT('Ctrl Pts',(-19.6026794702511,67.8458386692007,25.));
#31079=CARTESIAN_POINT('Ctrl Pts',(-19.6705100870722,67.8538637961796,25.));
#31080=CARTESIAN_POINT('Ctrl Pts',(-19.7385642439572,67.8579957018903,25.));
#31081=CARTESIAN_POINT('Ctrl Pts',(-19.8065962194624,67.8580563450086,25.));
#31082=CARTESIAN_POINT('Ctrl Pts',(-19.8163931634452,67.8580650779202,25.));
#31083=CARTESIAN_POINT('Ctrl Pts',(-19.8261896412384,67.8579892951331,25.));
#31084=CARTESIAN_POINT('Ctrl Pts',(-19.8359849096261,67.8578283749833,25.));
#31085=CARTESIAN_POINT('Ctrl Pts',(-19.905349147844,67.8566888346295,25.));
#31086=CARTESIAN_POINT('Ctrl Pts',(-19.9746541960652,67.8512840088951,25.));
#31087=CARTESIAN_POINT('Ctrl Pts',(-20.0435750455083,67.8417871266218,25.));
#31088=CARTESIAN_POINT('Ctrl Pts',(-20.1078703307363,67.8329276195282,25.));
#31089=CARTESIAN_POINT('Ctrl Pts',(-20.1718317704019,67.8205059706896,25.));
#31090=CARTESIAN_POINT('Ctrl Pts',(-20.2351749893643,67.8046283759774,25.));
#31091=CARTESIAN_POINT('Ctrl Pts',(-20.2490396161921,67.8011530722398,25.));
#31092=CARTESIAN_POINT('Ctrl Pts',(-20.2628745263258,67.7975120871324,25.));
#31093=CARTESIAN_POINT('Ctrl Pts',(-20.2766765599084,67.793706356147,25.));
#31094=CARTESIAN_POINT('Ctrl Pts',(-20.2877369911298,67.7906565863026,25.));
#31095=CARTESIAN_POINT('Ctrl Pts',(-20.2987757638788,67.787501080294,25.));
#31096=CARTESIAN_POINT('Ctrl Pts',(-20.3097781968535,67.7842444451942,25.));
#31097=CARTESIAN_POINT('Ctrl Pts',(-20.3753404535977,67.7648385240647,25.));
#31098=CARTESIAN_POINT('Ctrl Pts',(-20.4397363417765,67.7418126009015,25.));
#31099=CARTESIAN_POINT('Ctrl Pts',(-20.502663400315,67.7153486959875,25.));
#31100=CARTESIAN_POINT('Ctrl Pts',(-20.5652990969205,67.6890073230124,25.));
#31101=CARTESIAN_POINT('Ctrl Pts',(-20.6264804265539,67.6592590290608,25.));
#31102=CARTESIAN_POINT('Ctrl Pts',(-20.6858793170701,67.6262417671952,25.));
#31103=CARTESIAN_POINT('Ctrl Pts',(-20.7440054791047,67.5939319597818,25.));
#31104=CARTESIAN_POINT('Ctrl Pts',(-20.8004254400109,67.5584910682472,25.));
#31105=CARTESIAN_POINT('Ctrl Pts',(-20.8547918303173,67.52001896722,25.));
#31106=CARTESIAN_POINT('Ctrl Pts',(-20.8662882857036,67.5118835587336,25.));
#31107=CARTESIAN_POINT('Ctrl Pts',(-20.8776927475808,67.503612519805,25.));
#31108=CARTESIAN_POINT('Ctrl Pts',(-20.8890016529758,67.4952066661362,25.));
#31109=CARTESIAN_POINT('Ctrl Pts',(-20.8996328294733,67.4873045650181,25.));
#31110=CARTESIAN_POINT('Ctrl Pts',(-20.9101807913445,67.4792822117678,25.));
#31111=CARTESIAN_POINT('Ctrl Pts',(-20.9206259991789,67.4711535452534,25.));
#31112=CARTESIAN_POINT('Ctrl Pts',(-20.9721934579281,67.431022732941,25.));
#31113=CARTESIAN_POINT('Ctrl Pts',(-21.0213543413904,67.3882344350529,25.));
#31114=CARTESIAN_POINT('Ctrl Pts',(-21.0678175681512,67.34292066402,25.));
#31115=CARTESIAN_POINT('Ctrl Pts',(-21.1133971413376,67.2984686858183,25.));
#31116=CARTESIAN_POINT('Ctrl Pts',(-21.1563812744484,67.2515857193821,25.));
#31117=CARTESIAN_POINT('Ctrl Pts',(-21.196452662785,67.2023706262552,25.));
#31118=CARTESIAN_POINT('Ctrl Pts',(-21.2352229187693,67.1547535648547,25.));
#31119=CARTESIAN_POINT('Ctrl Pts',(-21.2712668558046,67.1049527951087,25.));
#31120=CARTESIAN_POINT('Ctrl Pts',(-21.3042504198252,67.0530424950224,25.));
#31121=CARTESIAN_POINT('Ctrl Pts',(-21.3097028004787,67.0444614115553,25.));
#31122=CARTESIAN_POINT('Ctrl Pts',(-21.3150714402185,67.0358226586051,25.));
#31123=CARTESIAN_POINT('Ctrl Pts',(-21.3203546922529,67.0271265453092,25.));
#31124=CARTESIAN_POINT('Ctrl Pts',(-21.3260102782519,67.0178175787331,25.));
#31125=CARTESIAN_POINT('Ctrl Pts',(-21.3315680165281,67.0084428810478,25.));
#31126=CARTESIAN_POINT('Ctrl Pts',(-21.3370275036536,66.9990041127266,25.));
#31127=CARTESIAN_POINT('Origin',(-20.,66.,37.5459252805377));
#31128=CARTESIAN_POINT('Ctrl Pts',(-22.0565719673595,66.0014962574405,35.7959252805377));
#31129=CARTESIAN_POINT('Ctrl Pts',(-22.0573889181502,66.099669215357,35.7905876687522));
#31130=CARTESIAN_POINT('Ctrl Pts',(-22.0063638713597,66.8783588803798,35.7482056843029));
#31131=CARTESIAN_POINT('Ctrl Pts',(-21.0114091850863,68.208181319433,35.6687793271896));
#31132=CARTESIAN_POINT('Ctrl Pts',(-18.6935441236518,68.0471886637504,35.5576462091982));
#31133=CARTESIAN_POINT('Ctrl Pts',(-17.5714219821268,66.0128602375846,35.4465130912065));
#31134=CARTESIAN_POINT('Ctrl Pts',(-18.6720184527178,63.9665951580731,35.335379973215));
#31135=CARTESIAN_POINT('Ctrl Pts',(-20.988041711498,63.7814657159201,35.2242468552234));
#31136=CARTESIAN_POINT('Ctrl Pts',(-22.0019739085829,65.1068137933338,35.144428624331));
#31137=CARTESIAN_POINT('Ctrl Pts',(-22.057280493024,65.8929627817184,35.1016547661024));
#31138=CARTESIAN_POINT('Ctrl Pts',(-22.0563748666992,65.9983937868295,35.0959252805377));
#31139=CARTESIAN_POINT('Ctrl Pts',(-22.0526727182563,65.9976789726186,35.8540747194623));
#31140=CARTESIAN_POINT('Ctrl Pts',(-22.0491245254771,66.4678277317379,35.8286277343138));
#31141=CARTESIAN_POINT('Ctrl Pts',(-21.6566322253174,67.6294023146612,35.7661363765015));
#31142=CARTESIAN_POINT('Ctrl Pts',(-19.7281828950178,68.4128315562992,35.6666006460254));
#31143=CARTESIAN_POINT('Ctrl Pts',(-17.8254683675795,67.0812973613349,35.5554675280337));
#31144=CARTESIAN_POINT('Ctrl Pts',(-17.9121447447308,64.7590835038729,35.4443344100422));
#31145=CARTESIAN_POINT('Ctrl Pts',(-19.9101226209547,63.5731232768953,35.3332012920507));
#31146=CARTESIAN_POINT('Ctrl Pts',(-21.7210100698093,64.4741603064334,35.2364480618573));
#31147=CARTESIAN_POINT('Ctrl Pts',(-22.0499160183042,65.5818790726719,35.1767392043279));
#31148=CARTESIAN_POINT('Ctrl Pts',(-22.0520910576133,66.0011644713934,35.1540747194623));
#31149=CARTESIAN_POINT('Ctrl Pts',(-18.7309291201477,67.0793586530486,36.));
#31150=CARTESIAN_POINT('Ctrl Pts',(-18.372032101712,66.6573805147568,35.9629556273362));
#31151=CARTESIAN_POINT('Ctrl Pts',(-18.1147584132015,65.4342585881912,35.8888668820084));
#31152=CARTESIAN_POINT('Ctrl Pts',(-19.454738309765,64.1066458935492,35.7777337640169));
#31153=CARTESIAN_POINT('Ctrl Pts',(-21.294007127745,64.5163018976528,35.6666006460253));
#31154=CARTESIAN_POINT('Ctrl Pts',(-21.9488058936235,66.2817526841271,35.5554675280338));
#31155=CARTESIAN_POINT('Ctrl Pts',(-20.8200548496672,67.7904027634385,35.4443344100422));
#31156=CARTESIAN_POINT('Ctrl Pts',(-18.9407200438028,67.6598692365535,35.3332012920506));
#31157=CARTESIAN_POINT('Ctrl Pts',(-18.0308986602863,66.0104271350851,35.2220681740591));
#31158=CARTESIAN_POINT('Ctrl Pts',(-18.9232669386679,64.351306744543,35.1109350560675));
#31159=CARTESIAN_POINT('Ctrl Pts',(-20.8011084031418,64.2012030089904,34.999801938076));
#31160=CARTESIAN_POINT('Ctrl Pts',(-21.9457415640057,65.697395124653,34.8886688200844));
#31161=CARTESIAN_POINT('Ctrl Pts',(-21.3095566464544,67.4705601638215,34.7775357020928));
#31162=CARTESIAN_POINT('Ctrl Pts',(-19.4748133482442,67.8978021178438,34.6664025841013));
#31163=CARTESIAN_POINT('Ctrl Pts',(-18.1207418428944,66.5881051616333,34.5552694661097));
#31164=CARTESIAN_POINT('Ctrl Pts',(-18.4866412203222,64.7401490647328,34.4441363481182));
#31165=CARTESIAN_POINT('Ctrl Pts',(-20.2376261931116,64.0452592090235,34.3330032301266));
#31166=CARTESIAN_POINT('Ctrl Pts',(-21.7711262834811,65.1394245223657,34.2218701121351));
#31167=CARTESIAN_POINT('Ctrl Pts',(-21.6836219072211,67.0212226559639,34.1107369941435));
#31168=CARTESIAN_POINT('Ctrl Pts',(-20.0552004852982,67.9683574838607,33.9996038761519));
#31169=CARTESIAN_POINT('Ctrl Pts',(-18.3762574113062,67.1139741369633,33.8884707581604));
#31170=CARTESIAN_POINT('Ctrl Pts',(-18.1834274619919,65.240037780099,33.7773376401688));
#31171=CARTESIAN_POINT('Ctrl Pts',(-19.6531962002549,64.0616487758754,33.6662045221773));
#31172=CARTESIAN_POINT('Ctrl Pts',(-21.4403734255104,64.6573150961213,33.5550714041857));
#31173=CARTESIAN_POINT('Ctrl Pts',(-21.9092641994935,66.4818594922784,33.4439382861941));
#31174=CARTESIAN_POINT('Ctrl Pts',(-20.6307212300429,67.8653871131315,33.3328051682026));
#31175=CARTESIAN_POINT('Ctrl Pts',(-18.7749173659869,67.5416390282116,33.221672050211));
#31176=CARTESIAN_POINT('Ctrl Pts',(-18.0403573473244,65.8069222258068,33.1105389322195));
#31177=CARTESIAN_POINT('Ctrl Pts',(-19.0993394151928,64.248917802084,32.9994058142279));
#31178=CARTESIAN_POINT('Ctrl Pts',(-20.9826414999224,64.2935727276805,32.8882726962364));
#31179=CARTESIAN_POINT('Ctrl Pts',(-21.9665914075352,65.9000170572955,32.7771395782447));
#31180=CARTESIAN_POINT('Ctrl Pts',(-21.1506394546859,67.5979697113295,32.6660064602533));
#31181=CARTESIAN_POINT('Ctrl Pts',(-19.2815769841816,67.833397590097,32.5548733422616));
#31182=CARTESIAN_POINT('Ctrl Pts',(-18.0700435346081,66.3908278325732,32.4437402242701));
#31183=CARTESIAN_POINT('Ctrl Pts',(-18.6248822045078,64.590557059849,32.3326071062785));
#31184=CARTESIAN_POINT('Ctrl Pts',(-20.4382828049508,64.0802639410825,32.221473988287));
#31185=CARTESIAN_POINT('Ctrl Pts',(-21.8505497316599,65.3269888235133,32.1103408702954));
#31186=CARTESIAN_POINT('Ctrl Pts',(-21.5691207070261,67.189680024126,31.9992077523039));
#31187=CARTESIAN_POINT('Ctrl Pts',(-19.8515706513329,67.9635292413093,31.8880746343123));
#31188=CARTESIAN_POINT('Ctrl Pts',(-18.269868977662,66.9402792130885,31.7769415163208));
#31189=CARTESIAN_POINT('Ctrl Pts',(-18.2716513129284,65.0564486400198,31.6658083983292));
#31190=CARTESIAN_POINT('Ctrl Pts',(-19.8552863937441,64.0361934094247,31.5546752803376));
#31191=CARTESIAN_POINT('Ctrl Pts',(-21.5713690628773,64.8132912651982,31.4435421623461));
#31192=CARTESIAN_POINT('Ctrl Pts',(-21.8492729171815,66.6765116634631,31.3324090443545));
#31193=CARTESIAN_POINT('Ctrl Pts',(-20.4346494110085,67.9205619600867,31.2212759263629));
#31194=CARTESIAN_POINT('Ctrl Pts',(-18.6222176562464,67.406838358257,31.1101428083714));
#31195=CARTESIAN_POINT('Ctrl Pts',(-18.0707865314722,65.6055209183322,30.9990096903798));
#31196=CARTESIAN_POINT('Ctrl Pts',(-19.2850475061968,64.165246260495,30.8878765723883));
#31197=CARTESIAN_POINT('Ctrl Pts',(-21.1536611435061,64.4042104402565,30.7767434543968));
#31198=CARTESIAN_POINT('Ctrl Pts',(-21.9663986946184,66.1037040347599,30.6656103364051));
#31199=CARTESIAN_POINT('Ctrl Pts',(-20.9794107637176,67.7082836149003,30.5544772184136));
#31200=CARTESIAN_POINT('Ctrl Pts',(-19.0960275526304,67.7493747932959,30.4433441004221));
#31201=CARTESIAN_POINT('Ctrl Pts',(-18.0399955053847,66.1893693061462,30.3322109824305));
#31202=CARTESIAN_POINT('Ctrl Pts',(-18.7778367166361,64.4560455765083,30.2210778644389));
#31203=CARTESIAN_POINT('Ctrl Pts',(-20.6342498687002,64.1358097047038,30.1099447464473));
#31204=CARTESIAN_POINT('Ctrl Pts',(-21.9101725770983,65.5217541649695,29.9988116284558));
#31205=CARTESIAN_POINT('Ctrl Pts',(-21.4378301592761,67.3454080370277,29.8876785104642));
#31206=CARTESIAN_POINT('Ctrl Pts',(-19.6495289872407,67.9376915188538,29.7765453924727));
#31207=CARTESIAN_POINT('Ctrl Pts',(-18.1819926804873,66.75652345583,29.6654122744811));
#31208=CARTESIAN_POINT('Ctrl Pts',(-18.3783682286227,64.8829553495575,29.5542791564896));
#31209=CARTESIAN_POINT('Ctrl Pts',(-20.0589250007271,64.0317504738189,29.443146038498));
#31210=CARTESIAN_POINT('Ctrl Pts',(-21.6855512929007,64.9819650339878,29.3320129205065));
#31211=CARTESIAN_POINT('Ctrl Pts',(-21.7694946991591,66.8639252645168,29.2208798025149));
#31212=CARTESIAN_POINT('Ctrl Pts',(-20.2339269101145,67.9551870891929,29.1097466845233));
#31213=CARTESIAN_POINT('Ctrl Pts',(-18.4842600056596,67.2569847344258,28.9986135665318));
#31214=CARTESIAN_POINT('Ctrl Pts',(-18.1218580029699,65.408340476275,28.8874804485402));
#31215=CARTESIAN_POINT('Ctrl Pts',(-19.4784054789109,64.1012063017294,28.7763473305487));
#31216=CARTESIAN_POINT('Ctrl Pts',(-21.3123367903127,64.5319228556325,28.6652142125571));
#31217=CARTESIAN_POINT('Ctrl Pts',(-21.9451658181481,66.3062813950144,28.5540810945656));
#31218=CARTESIAN_POINT('Ctrl Pts',(-20.7977025282328,67.8003191465602,28.442947976574));
#31219=CARTESIAN_POINT('Ctrl Pts',(-18.9201504872152,67.6466339553042,28.3318148585824));
#31220=CARTESIAN_POINT('Ctrl Pts',(-18.0309192227571,65.9858845572708,28.2206817405909));
#31221=CARTESIAN_POINT('Ctrl Pts',(-18.9438681879035,64.3380541680053,28.1095486225993));
#31222=CARTESIAN_POINT('Ctrl Pts',(-20.8234305564082,64.2113020177245,27.9984155046077));
#31223=CARTESIAN_POINT('Ctrl Pts',(-21.9493568698083,65.7216366633037,27.8872823866162));
#31224=CARTESIAN_POINT('Ctrl Pts',(-21.291155049959,67.4867403908715,27.7761492686246));
#31225=CARTESIAN_POINT('Ctrl Pts',(-19.4512373091435,67.891120795242,27.6650161506331));
#31226=CARTESIAN_POINT('Ctrl Pts',(-18.1135687818421,66.5646730138986,27.5538830326415));
#31227=CARTESIAN_POINT('Ctrl Pts',(-18.5024363551,64.7214142651596,27.4427499146499));
#31228=CARTESIAN_POINT('Ctrl Pts',(-20.2619331187203,64.0483675051169,27.3316167966584));
#31229=CARTESIAN_POINT('Ctrl Pts',(-21.7816983844559,65.1615316208422,27.2204836786668));
#31230=CARTESIAN_POINT('Ctrl Pts',(-21.6707831578744,67.0420949970833,27.1093505606753));
#31231=CARTESIAN_POINT('Ctrl Pts',(-20.0307014315933,67.9688920192891,26.9982174426837));
#31232=CARTESIAN_POINT('Ctrl Pts',(-18.3625205312278,67.093681563121,26.8870843246922));
#31233=CARTESIAN_POINT('Ctrl Pts',(-18.193025322136,65.217490708422,26.7759512067006));
#31234=CARTESIAN_POINT('Ctrl Pts',(-19.6773443984712,64.0574831268864,26.664818088709));
#31235=CARTESIAN_POINT('Ctrl Pts',(-21.4569707037066,64.6753435036645,26.5536849707175));
#31236=CARTESIAN_POINT('Ctrl Pts',(-21.9031198303154,66.5055815255925,26.4425518527259));
#31237=CARTESIAN_POINT('Ctrl Pts',(-20.6074592701813,67.8730916715933,26.3314187347344));
#31238=CARTESIAN_POINT('Ctrl Pts',(-18.7558271036352,67.5262741254895,26.2202856167428));
#31239=CARTESIAN_POINT('Ctrl Pts',(-18.0429128818286,65.7825513633931,26.1091524987513));
#31240=CARTESIAN_POINT('Ctrl Pts',(-19.1211979533711,64.2378442836875,25.9980193807597));
#31241=CARTESIAN_POINT('Ctrl Pts',(-21.0038049577023,64.3059351985902,25.8868862627681));
#31242=CARTESIAN_POINT('Ctrl Pts',(-21.9676747832011,65.9244934704524,25.7757531447766));
#31243=CARTESIAN_POINT('Ctrl Pts',(-21.1306818475489,67.6121730972753,25.664620026785));
#31244=CARTESIAN_POINT('Ctrl Pts',(-19.2587832804016,67.8242989299444,25.5534869087934));
#31245=CARTESIAN_POINT('Ctrl Pts',(-18.0653972468034,66.3668134340257,25.4423537908019));
#31246=CARTESIAN_POINT('Ctrl Pts',(-18.642392926108,64.5734885052306,25.3312206728103));
#31247=CARTESIAN_POINT('Ctrl Pts',(-20.4624083103757,64.0859969852348,25.2200875548188));
#31248=CARTESIAN_POINT('Ctrl Pts',(-21.8582430905867,65.3498099340575,25.1089544368272));
#31249=CARTESIAN_POINT('Ctrl Pts',(-21.5552778968737,67.2096324841655,24.9978213188357));
#31250=CARTESIAN_POINT('Ctrl Pts',(-19.82486994896,67.9604919410323,24.8866882008441));
#31251=CARTESIAN_POINT('Ctrl Pts',(-18.7848659979775,67.2672324081111,24.8125994555164));
#31252=CARTESIAN_POINT('Ctrl Pts',(-18.5264217726374,66.7772536316049,24.7755550828525));
#31253=CARTESIAN_POINT('Ctrl Pts',(-18.6322193753412,67.1633123698098,36.0748149723825));
#31254=CARTESIAN_POINT('Ctrl Pts',(-18.2454069475584,66.7085123024942,36.0377705997186));
#31255=CARTESIAN_POINT('Ctrl Pts',(-17.9681222253528,65.3902545918245,35.9636818543909));
#31256=CARTESIAN_POINT('Ctrl Pts',(-19.4123272489249,63.9593787048971,35.8525487363994));
#31257=CARTESIAN_POINT('Ctrl Pts',(-21.3946564416527,64.4008982087198,35.7414156184078));
#31258=CARTESIAN_POINT('Ctrl Pts',(-22.1003861839689,66.3036677213329,35.6302825004163));
#31259=CARTESIAN_POINT('Ctrl Pts',(-20.8838396281403,67.9296622821033,35.5191493824247));
#31260=CARTESIAN_POINT('Ctrl Pts',(-18.8583280704192,67.7889757122858,35.4080162644331));
#31261=CARTESIAN_POINT('Ctrl Pts',(-17.8777397675665,66.0112381692516,35.2968831464416));
#31262=CARTESIAN_POINT('Ctrl Pts',(-18.8395174433512,64.223069549053,35.18575002845));
#31263=CARTESIAN_POINT('Ctrl Pts',(-20.8634195059272,64.0612905779669,35.0746169104585));
#31264=CARTESIAN_POINT('Ctrl Pts',(-22.0970835073845,65.6738581808173,34.9634837924669));
#31265=CARTESIAN_POINT('Ctrl Pts',(-21.4114154192253,67.5849419692808,34.8523506744753));
#31266=CARTESIAN_POINT('Ctrl Pts',(-19.4339637462294,68.0454152777701,34.7412175564838));
#31267=CARTESIAN_POINT('Ctrl Pts',(-17.9745710528634,66.6338486353397,34.6300844384922));
#31268=CARTESIAN_POINT('Ctrl Pts',(-18.3689304909105,64.6421564574729,34.5189513205007));
#31269=CARTESIAN_POINT('Ctrl Pts',(-20.2561090227579,63.8932172957598,34.4078182025091));
#31270=CARTESIAN_POINT('Ctrl Pts',(-21.9088864560908,65.0724880043724,34.2966850845175));
#31271=CARTESIAN_POINT('Ctrl Pts',(-21.8145758921015,67.1006544901989,34.185551966526));
#31272=CARTESIAN_POINT('Ctrl Pts',(-20.0594940404522,68.1214585186447,34.0744188485344));
#31273=CARTESIAN_POINT('Ctrl Pts',(-18.2499609064333,67.2006202845713,33.9632857305429));
#31274=CARTESIAN_POINT('Ctrl Pts',(-18.0421324291486,65.180927073219,33.8521526125513));
#31275=CARTESIAN_POINT('Ctrl Pts',(-19.6262214149106,63.9108816613538,33.7410194945598));
#31276=CARTESIAN_POINT('Ctrl Pts',(-21.5524072728828,64.5528795706346,33.6298863765682));
#31277=CARTESIAN_POINT('Ctrl Pts',(-22.0577688928814,66.51933905963,33.5187532585766));
#31278=CARTESIAN_POINT('Ctrl Pts',(-20.6797794289583,68.0104789979313,33.4076201405851));
#31279=CARTESIAN_POINT('Ctrl Pts',(-18.6796290758763,67.6615494268146,33.2964870225935));
#31280=CARTESIAN_POINT('Ctrl Pts',(-17.8879341618047,65.7919044217416,33.185353904602));
#31281=CARTESIAN_POINT('Ctrl Pts',(-19.0292850329711,64.1127166807475,33.0742207866104));
#31282=CARTESIAN_POINT('Ctrl Pts',(-21.059072448921,64.1608449161331,32.9630876686188));
#31283=CARTESIAN_POINT('Ctrl Pts',(-22.119555074938,65.8922402727864,32.8519545506273));
#31284=CARTESIAN_POINT('Ctrl Pts',(-21.2401374714945,67.7222615731301,32.7408214326357));
#31285=CARTESIAN_POINT('Ctrl Pts',(-19.2256972428052,67.9760012942087,32.6296883146441));
#31286=CARTESIAN_POINT('Ctrl Pts',(-17.9199293737595,66.4212268561652,32.5185551966526));
#31287=CARTESIAN_POINT('Ctrl Pts',(-18.5179240126315,64.4809290200364,32.407422078661));
#31288=CARTESIAN_POINT('Ctrl Pts',(-20.4723729290854,63.9309447348192,32.2962889606695));
#31289=CARTESIAN_POINT('Ctrl Pts',(-21.9944875484231,65.2746412655183,32.1851558426779));
#31290=CARTESIAN_POINT('Ctrl Pts',(-21.691168661179,67.282214659856,32.0740227246864));
#31291=CARTESIAN_POINT('Ctrl Pts',(-19.840025651474,68.1162547300167,31.9628896066948));
#31292=CARTESIAN_POINT('Ctrl Pts',(-18.135297462069,67.0134151762913,31.8517564887032));
#31293=CARTESIAN_POINT('Ctrl Pts',(-18.1372184293551,64.9830581655917,31.7406233707117));
#31294=CARTESIAN_POINT('Ctrl Pts',(-19.8440304084636,63.8834463481829,31.6294902527201));
#31295=CARTESIAN_POINT('Ctrl Pts',(-21.6935918966495,64.7209877396572,31.5183571347286));
#31296=CARTESIAN_POINT('Ctrl Pts',(-21.9931114218943,66.7291314932291,31.407224016737));
#31297=CARTESIAN_POINT('Ctrl Pts',(-20.4684569257203,68.0699454058618,31.2960908987455));
#31298=CARTESIAN_POINT('Ctrl Pts',(-18.5150522128422,67.5162638107925,31.1849577807539));
#31299=CARTESIAN_POINT('Ctrl Pts',(-17.9207301617462,65.5748378965238,31.0738246627623));
#31300=CARTESIAN_POINT('Ctrl Pts',(-19.2294377058835,64.0225370735738,30.9626915447708));
#31301=CARTESIAN_POINT('Ctrl Pts',(-21.2433941906325,64.2800881530714,30.8515584267792));
#31302=CARTESIAN_POINT('Ctrl Pts',(-22.1193473725962,66.1117702499486,30.7404253087876));
#31303=CARTESIAN_POINT('Ctrl Pts',(-21.0555904224601,67.8411558148388,30.6292921907961));
#31304=CARTESIAN_POINT('Ctrl Pts',(-19.0257155700544,67.8854431108016,30.5181590728045));
#31305=CARTESIAN_POINT('Ctrl Pts',(-17.8875441753963,66.2040986614413,30.407025954813));
#31306=CARTESIAN_POINT('Ctrl Pts',(-18.6827754968666,64.3359550838847,30.2958928368214));
#31307=CARTESIAN_POINT('Ctrl Pts',(-20.6835825290558,63.9908109097266,30.1847597188299));
#31308=CARTESIAN_POINT('Ctrl Pts',(-22.0587479251069,65.4845556718986,30.0736266008383));
#31309=CARTESIAN_POINT('Ctrl Pts',(-21.5496661885715,67.4500553708401,29.9624934828468));
#31310=CARTESIAN_POINT('Ctrl Pts',(-19.6222689619886,68.0884073207655,29.8513603648552));
#31311=CARTESIAN_POINT('Ctrl Pts',(-18.0405860487425,66.8153666918152,29.7402272468636));
#31312=CARTESIAN_POINT('Ctrl Pts',(-18.2522359054689,64.7960703739953,29.6290941288721));
#31313=CARTESIAN_POINT('Ctrl Pts',(-20.0635082528345,63.8786578361033,29.5179610108805));
#31314=CARTESIAN_POINT('Ctrl Pts',(-21.8166553475456,64.9027811418235,29.406827892889));
#31315=CARTESIAN_POINT('Ctrl Pts',(-21.9071279653252,66.9311223326602,29.2956947748974));
#31316=CARTESIAN_POINT('Ctrl Pts',(-20.2521220054139,68.1072637160285,29.1845616569058));
#31317=CARTESIAN_POINT('Ctrl Pts',(-18.3663640627225,67.3547544053958,29.0734285389143));
#31318=CARTESIAN_POINT('Ctrl Pts',(-17.9757740291112,65.362320540331,28.9622954209227));
#31319=CARTESIAN_POINT('Ctrl Pts',(-19.4378352768154,63.9535160155744,28.8511623029312));
#31320=CARTESIAN_POINT('Ctrl Pts',(-21.4144118057657,64.4177341821886,28.7400291849396));
#31321=CARTESIAN_POINT('Ctrl Pts',(-22.0964629793736,66.3301043026398,28.628896066948));
#31322=CARTESIAN_POINT('Ctrl Pts',(-20.8597487182789,67.9403499725357,28.5177629489565));
#31323=CARTESIAN_POINT('Ctrl Pts',(-18.8361585908377,67.7747109761374,28.4066298309649));
#31324=CARTESIAN_POINT('Ctrl Pts',(-17.8777619294091,65.9847866424326,28.2954967129734));
#31325=CARTESIAN_POINT('Ctrl Pts',(-18.8617210806702,64.2087861723696,28.1843635949818));
#31326=CARTESIAN_POINT('Ctrl Pts',(-20.8874779011068,64.072175098835,28.0732304769902));
#31327=CARTESIAN_POINT('Ctrl Pts',(-22.1009800156942,65.6999852533116,27.9620973589987));
#31328=CARTESIAN_POINT('Ctrl Pts',(-21.3915825260838,67.6023807123903,27.8509642410071));
#31329=CARTESIAN_POINT('Ctrl Pts',(-19.4085539365804,68.0382142744638,27.7398311230156));
#31330=CARTESIAN_POINT('Ctrl Pts',(-17.9668400631429,66.6085939090873,27.628698005024));
#31331=CARTESIAN_POINT('Ctrl Pts',(-18.3859541888425,64.6219644443474,27.5175648870324));
#31332=CARTESIAN_POINT('Ctrl Pts',(-20.2823065680806,63.8965673585811,27.4064317690409));
#31333=CARTESIAN_POINT('Ctrl Pts',(-21.9202808668403,65.0963146175614,27.2952986510493));
#31334=CARTESIAN_POINT('Ctrl Pts',(-21.8007385305482,67.1231503052298,27.1841655330578));
#31335=CARTESIAN_POINT('Ctrl Pts',(-20.0330894230963,68.1220346308335,27.0730324150662));
#31336=CARTESIAN_POINT('Ctrl Pts',(-18.2351555565408,67.178749331761,26.9618992970747));
#31337=CARTESIAN_POINT('Ctrl Pts',(-18.0524768215319,65.1566262652246,26.8507661790831));
#31338=CARTESIAN_POINT('Ctrl Pts',(-19.6522478868477,63.9063920035524,26.7396330610915));
#31339=CARTESIAN_POINT('Ctrl Pts',(-21.5702955058407,64.5723102477722,26.6284999431));
#31340=CARTESIAN_POINT('Ctrl Pts',(-22.0511466078334,66.5449062190847,26.5173668251084));
#31341=CARTESIAN_POINT('Ctrl Pts',(-20.654708127981,68.0187828255213,26.4062337071169));
#31342=CARTESIAN_POINT('Ctrl Pts',(-18.6590539516821,67.644989424866,26.2951005891253));
#31343=CARTESIAN_POINT('Ctrl Pts',(-17.8906884686255,65.7656379665382,26.1839674711338));
#31344=CARTESIAN_POINT('Ctrl Pts',(-19.0528437525653,64.1007818517715,26.0728343531422));
#31345=CARTESIAN_POINT('Ctrl Pts',(-21.0818820239902,64.1741689537826,25.9617012351506));
#31346=CARTESIAN_POINT('Ctrl Pts',(-22.1207227167685,65.9186204885875,25.8505681171591));
#31347=CARTESIAN_POINT('Ctrl Pts',(-21.2186275394726,67.7375697142351,25.7394349991675));
#31348=CARTESIAN_POINT('Ctrl Pts',(-19.2011306193885,67.9661949301477,25.6283018811759));
#31349=CARTESIAN_POINT('Ctrl Pts',(-17.9149216925206,66.395344590984,25.5171687631844));
#31350=CARTESIAN_POINT('Ctrl Pts',(-18.5367967376375,64.4625328542518,25.4060356451928));
#31351=CARTESIAN_POINT('Ctrl Pts',(-20.4983749431605,63.9371237015234,25.2949025272012));
#31352=CARTESIAN_POINT('Ctrl Pts',(-22.0027793053657,65.2992374274278,25.1837694092097));
#31353=CARTESIAN_POINT('Ctrl Pts',(-21.6762491418536,67.3037190444335,25.0726362912181));
#31354=CARTESIAN_POINT('Ctrl Pts',(-19.8112481387675,68.1129811851452,24.9615031732266));
#31355=CARTESIAN_POINT('Ctrl Pts',(-18.6903515235305,67.3657991545403,24.8874144278989));
#31356=CARTESIAN_POINT('Ctrl Pts',(-18.4118052188384,66.837709283723,24.850370055235));
#31357=CARTESIAN_POINT('Ctrl Pts',(-18.5335096305348,67.247266086571,36.149629944765));
#31358=CARTESIAN_POINT('Ctrl Pts',(-18.1187817934049,66.7596440902317,36.1125855721011));
#31359=CARTESIAN_POINT('Ctrl Pts',(-17.8214860375041,65.3462505954579,36.0384968267734));
#31360=CARTESIAN_POINT('Ctrl Pts',(-19.3699161880848,63.8121115162452,35.9273637087819));
#31361=CARTESIAN_POINT('Ctrl Pts',(-21.4953057555605,64.2854945197867,35.8162305907903));
#31362=CARTESIAN_POINT('Ctrl Pts',(-22.2519664743143,66.3255827585387,35.7050974727988));
#31363=CARTESIAN_POINT('Ctrl Pts',(-20.9476244066133,68.0689218007681,35.5939643548072));
#31364=CARTESIAN_POINT('Ctrl Pts',(-18.7759360970355,67.9180821880181,35.4828312368156));
#31365=CARTESIAN_POINT('Ctrl Pts',(-17.7245808748466,66.0120492034181,35.3716981188241));
#31366=CARTESIAN_POINT('Ctrl Pts',(-18.7557679480345,64.0948323535631,35.2605650008325));
#31367=CARTESIAN_POINT('Ctrl Pts',(-20.9257306087126,63.9213781469436,35.149431882841));
#31368=CARTESIAN_POINT('Ctrl Pts',(-22.2484254507633,65.6503212369814,35.0382987648494));
#31369=CARTESIAN_POINT('Ctrl Pts',(-21.5132741919963,67.6993237747403,34.9271656468578));
#31370=CARTESIAN_POINT('Ctrl Pts',(-19.3931141442146,68.1930284376963,34.8160325288663));
#31371=CARTESIAN_POINT('Ctrl Pts',(-17.8284002628325,66.6795921090463,34.7048994108747));
#31372=CARTESIAN_POINT('Ctrl Pts',(-18.2512197614988,64.5441638502129,34.5937662928831));
#31373=CARTESIAN_POINT('Ctrl Pts',(-20.2745918524042,63.7411753824961,34.4826331748916));
#31374=CARTESIAN_POINT('Ctrl Pts',(-22.0466466287005,65.0055514863792,34.3715000569));
#31375=CARTESIAN_POINT('Ctrl Pts',(-21.9455298769819,67.1800863244337,34.2603669389085));
#31376=CARTESIAN_POINT('Ctrl Pts',(-20.0637875956061,68.2745595534289,34.1492338209169));
#31377=CARTESIAN_POINT('Ctrl Pts',(-18.1236644015604,67.2872664321791,34.0381007029254));
#31378=CARTESIAN_POINT('Ctrl Pts',(-17.9008373963053,65.1218163663389,33.9269675849338));
#31379=CARTESIAN_POINT('Ctrl Pts',(-19.5992466295663,63.7601145468323,33.8158344669422));
#31380=CARTESIAN_POINT('Ctrl Pts',(-21.6644411202551,64.4484440451478,33.7047013489507));
#31381=CARTESIAN_POINT('Ctrl Pts',(-22.2062735862694,66.5568186269816,33.5935682309591));
#31382=CARTESIAN_POINT('Ctrl Pts',(-20.7288376278737,68.1555708827312,33.4824351129676));
#31383=CARTESIAN_POINT('Ctrl Pts',(-18.5843407857658,67.7814598254175,33.371301994976));
#31384=CARTESIAN_POINT('Ctrl Pts',(-17.735510976285,65.7768866176765,33.2601688769845));
#31385=CARTESIAN_POINT('Ctrl Pts',(-18.9592306507495,63.9765155594109,33.1490357589929));
#31386=CARTESIAN_POINT('Ctrl Pts',(-21.1355033979196,64.0281171045857,33.0379026410013));
#31387=CARTESIAN_POINT('Ctrl Pts',(-22.2725187423409,65.8844634882773,32.9267695230097));
#31388=CARTESIAN_POINT('Ctrl Pts',(-21.329635488303,67.8465534349308,32.8156364050182));
#31389=CARTESIAN_POINT('Ctrl Pts',(-19.1698175014287,68.1186049983203,32.7045032870266));
#31390=CARTESIAN_POINT('Ctrl Pts',(-17.769815212911,66.4516258797572,32.5933701690351));
#31391=CARTESIAN_POINT('Ctrl Pts',(-18.4109658207552,64.3713009802238,32.4822370510435));
#31392=CARTESIAN_POINT('Ctrl Pts',(-20.50646305322,63.7816255285558,32.371103933052));
#31393=CARTESIAN_POINT('Ctrl Pts',(-22.1384253651864,65.2222937075232,32.2599708150604));
#31394=CARTESIAN_POINT('Ctrl Pts',(-21.8132166153319,67.3747492955862,32.1488376970689));
#31395=CARTESIAN_POINT('Ctrl Pts',(-19.8284806516152,68.2689802187239,32.0377045790773));
#31396=CARTESIAN_POINT('Ctrl Pts',(-18.000725946476,67.0865511394943,31.9265714610858));
#31397=CARTESIAN_POINT('Ctrl Pts',(-18.0027855457819,64.9096676911634,31.8154383430942));
#31398=CARTESIAN_POINT('Ctrl Pts',(-19.832774423183,63.7306992869412,31.7043052251026));
#31399=CARTESIAN_POINT('Ctrl Pts',(-21.8158147304217,64.6286842141161,31.593172107111));
#31400=CARTESIAN_POINT('Ctrl Pts',(-22.136949926607,66.7817513229953,31.4820389891195));
#31401=CARTESIAN_POINT('Ctrl Pts',(-20.5022644404321,68.2193288516369,31.3709058711279));
#31402=CARTESIAN_POINT('Ctrl Pts',(-18.407886769438,67.625689263328,31.2597727531364));
#31403=CARTESIAN_POINT('Ctrl Pts',(-17.7706737920203,65.5441548747155,31.1486396351448));
#31404=CARTESIAN_POINT('Ctrl Pts',(-19.1738279055702,63.8798278866525,31.0375065171532));
#31405=CARTESIAN_POINT('Ctrl Pts',(-21.333127237759,64.1559658658865,30.9263733991617));
#31406=CARTESIAN_POINT('Ctrl Pts',(-22.2722960505739,66.1198364651373,30.8152402811701));
#31407=CARTESIAN_POINT('Ctrl Pts',(-21.1317700812027,67.9740280147772,30.7041071631786));
#31408=CARTESIAN_POINT('Ctrl Pts',(-18.9554035874784,68.0215114283074,30.592974045187));
#31409=CARTESIAN_POINT('Ctrl Pts',(-17.735092845408,66.2188280167362,30.4818409271955));
#31410=CARTESIAN_POINT('Ctrl Pts',(-18.5877142770972,64.2158645912613,30.3707078092039));
#31411=CARTESIAN_POINT('Ctrl Pts',(-20.7329151894114,63.8458121147493,30.2595746912123));
#31412=CARTESIAN_POINT('Ctrl Pts',(-22.2073232731155,65.4473571788279,30.1484415732208));
#31413=CARTESIAN_POINT('Ctrl Pts',(-21.6615022178669,67.5547027046525,30.0373084552292));
#31414=CARTESIAN_POINT('Ctrl Pts',(-19.5950089367365,68.2391231226771,29.9261753372376));
#31415=CARTESIAN_POINT('Ctrl Pts',(-17.8991794169977,66.8742099278003,29.8150422192461));
#31416=CARTESIAN_POINT('Ctrl Pts',(-18.126103582315,64.7091853984332,29.7039091012545));
#31417=CARTESIAN_POINT('Ctrl Pts',(-20.0680915049419,63.7255651983877,29.592775983263));
#31418=CARTESIAN_POINT('Ctrl Pts',(-21.9477594021904,64.8235972496592,29.4816428652714));
#31419=CARTESIAN_POINT('Ctrl Pts',(-22.0447612314913,66.9983194008037,29.3705097472799));
#31420=CARTESIAN_POINT('Ctrl Pts',(-20.2703171007134,68.2593403428639,29.2593766292883));
#31421=CARTESIAN_POINT('Ctrl Pts',(-18.2484681197853,67.4525240763659,29.1482435112968));
#31422=CARTESIAN_POINT('Ctrl Pts',(-17.8296900552526,65.316300604387,29.0371103933052));
#31423=CARTESIAN_POINT('Ctrl Pts',(-19.3972650747199,63.8058257294195,28.9259772753136));
#31424=CARTESIAN_POINT('Ctrl Pts',(-21.5164868212187,64.3035455087446,28.8148441573221));
#31425=CARTESIAN_POINT('Ctrl Pts',(-22.2477601405991,66.3539272102652,28.7037110393305));
#31426=CARTESIAN_POINT('Ctrl Pts',(-20.9217949083251,68.0803807985112,28.592577921339));
#31427=CARTESIAN_POINT('Ctrl Pts',(-18.7521666944602,67.9027879969706,28.4814448033474));
#31428=CARTESIAN_POINT('Ctrl Pts',(-17.7246046360611,65.9836887275945,28.3703116853559));
#31429=CARTESIAN_POINT('Ctrl Pts',(-18.7795739734368,64.0795181767337,28.2591785673643));
#31430=CARTESIAN_POINT('Ctrl Pts',(-20.9515252458054,63.9330481799455,28.1480454493727));
#31431=CARTESIAN_POINT('Ctrl Pts',(-22.2526031615802,65.6783338433195,28.0369123313812));
#31432=CARTESIAN_POINT('Ctrl Pts',(-21.4920100022086,67.7180210339092,27.9257792133896));
#31433=CARTESIAN_POINT('Ctrl Pts',(-19.3658705640173,68.1853077536856,27.8146460953981));
#31434=CARTESIAN_POINT('Ctrl Pts',(-17.8201113444436,66.652514804276,27.7035129774064));
#31435=CARTESIAN_POINT('Ctrl Pts',(-18.269472022585,64.5225146235353,27.592379859415));
#31436=CARTESIAN_POINT('Ctrl Pts',(-20.3026800174408,63.7447672120453,27.4812467414234));
#31437=CARTESIAN_POINT('Ctrl Pts',(-22.0588633492247,65.0310976142806,27.3701136234318));
#31438=CARTESIAN_POINT('Ctrl Pts',(-21.930693903222,67.2042056133763,27.2589805054403));
#31439=CARTESIAN_POINT('Ctrl Pts',(-20.0354774145993,68.2751772423777,27.1478473874487));
#31440=CARTESIAN_POINT('Ctrl Pts',(-18.1077905818539,67.2638171004012,27.0367142694571));
#31441=CARTESIAN_POINT('Ctrl Pts',(-17.9119283209277,65.0957618220271,26.9255811514656));
#31442=CARTESIAN_POINT('Ctrl Pts',(-19.6271513752242,63.7553008802185,26.814448033474));
#31443=CARTESIAN_POINT('Ctrl Pts',(-21.6836203079748,64.4692769918797,26.7033149154825));
#31444=CARTESIAN_POINT('Ctrl Pts',(-22.1991733853515,66.5842309125769,26.5921817974909));
#31445=CARTESIAN_POINT('Ctrl Pts',(-20.7019569857807,68.1644739794492,26.4810486794993));
#31446=CARTESIAN_POINT('Ctrl Pts',(-18.5622807997289,67.7637047242426,26.3699155615078));
#31447=CARTESIAN_POINT('Ctrl Pts',(-17.7384640554224,65.7487245696832,26.2587824435162));
#31448=CARTESIAN_POINT('Ctrl Pts',(-18.9844895517596,63.9637194198555,26.1476493255246));
#31449=CARTESIAN_POINT('Ctrl Pts',(-21.1599590902781,64.0424027089751,26.0365162075331));
#31450=CARTESIAN_POINT('Ctrl Pts',(-22.2737706503358,65.9127475067224,25.9253830895415));
#31451=CARTESIAN_POINT('Ctrl Pts',(-21.3065732313963,67.862966331195,25.81424997155));
#31452=CARTESIAN_POINT('Ctrl Pts',(-19.1434779583753,68.1080909303509,25.7031168535584));
#31453=CARTESIAN_POINT('Ctrl Pts',(-17.7644461382379,66.4238757479422,25.5919837355669));
#31454=CARTESIAN_POINT('Ctrl Pts',(-18.431200549167,64.3515772032731,25.4808506175753));
#31455=CARTESIAN_POINT('Ctrl Pts',(-20.5343415759454,63.7882504178119,25.3697174995837));
#31456=CARTESIAN_POINT('Ctrl Pts',(-22.1473155201447,65.2486649207981,25.2585843815922));
#31457=CARTESIAN_POINT('Ctrl Pts',(-21.7972203868335,67.3978056047015,25.1474512636006));
#31458=CARTESIAN_POINT('Ctrl Pts',(-19.7976263285751,68.2654704292581,25.0363181456091));
#31459=CARTESIAN_POINT('Ctrl Pts',(-18.5958370490835,67.4643659009695,24.9622294002814));
#31460=CARTESIAN_POINT('Ctrl Pts',(-18.2971886650395,66.8981649358411,24.9251850276175));
#31461=CARTESIAN_POINT('Ctrl Pts',(-18.4347998857283,67.3312198033323,36.2244449171475));
#31462=CARTESIAN_POINT('Ctrl Pts',(-17.9921566392513,66.8107758779691,36.1874005444836));
#31463=CARTESIAN_POINT('Ctrl Pts',(-17.6748498496554,65.3022465990912,36.1133117991559));
#31464=CARTESIAN_POINT('Ctrl Pts',(-19.3275051272447,63.6648443275931,36.0021786811644));
#31465=CARTESIAN_POINT('Ctrl Pts',(-21.5959550694682,64.1700908308537,35.8910455631727));
#31466=CARTESIAN_POINT('Ctrl Pts',(-22.4035467646596,66.3474977957444,35.7799124451813));
#31467=CARTESIAN_POINT('Ctrl Pts',(-21.0114091850863,68.208181319433,35.6687793271896));
#31468=CARTESIAN_POINT('Ctrl Pts',(-18.6935441236518,68.0471886637504,35.5576462091982));
#31469=CARTESIAN_POINT('Ctrl Pts',(-17.5714219821268,66.0128602375846,35.4465130912065));
#31470=CARTESIAN_POINT('Ctrl Pts',(-18.6720184527178,63.9665951580731,35.335379973215));
#31471=CARTESIAN_POINT('Ctrl Pts',(-20.988041711498,63.7814657159201,35.2242468552234));
#31472=CARTESIAN_POINT('Ctrl Pts',(-22.3997673941421,65.6267842931457,35.1131137372319));
#31473=CARTESIAN_POINT('Ctrl Pts',(-21.6151329647672,67.8137055801995,35.0019806192403));
#31474=CARTESIAN_POINT('Ctrl Pts',(-19.3522645421998,68.3406415976227,34.8908475012488));
#31475=CARTESIAN_POINT('Ctrl Pts',(-17.6822294728015,66.7253355827527,34.7797143832572));
#31476=CARTESIAN_POINT('Ctrl Pts',(-18.1335090320871,64.4461712429531,34.6685812652656));
#31477=CARTESIAN_POINT('Ctrl Pts',(-20.2930746820505,63.5891334692323,34.5574481472741));
#31478=CARTESIAN_POINT('Ctrl Pts',(-22.1844068013102,64.9386149683859,34.4463150292826));
#31479=CARTESIAN_POINT('Ctrl Pts',(-22.0764838618623,67.2595181586686,34.3351819112909));
#31480=CARTESIAN_POINT('Ctrl Pts',(-20.0680811507602,68.427660588213,34.2240487932995));
#31481=CARTESIAN_POINT('Ctrl Pts',(-17.9973678966875,67.3739125797871,34.1129156753078));
#31482=CARTESIAN_POINT('Ctrl Pts',(-17.7595423634621,65.0627056594589,34.0017825573163));
#31483=CARTESIAN_POINT('Ctrl Pts',(-19.572271844222,63.6093474323109,33.8906494393247));
#31484=CARTESIAN_POINT('Ctrl Pts',(-21.7764749676275,64.344008519661,33.7795163213332));
#31485=CARTESIAN_POINT('Ctrl Pts',(-22.3547782796574,66.5942981943332,33.6683832033416));
#31486=CARTESIAN_POINT('Ctrl Pts',(-20.7778958267891,68.3006627675311,33.5572500853501));
#31487=CARTESIAN_POINT('Ctrl Pts',(-18.4890524956552,67.9013702240204,33.4461169673585));
#31488=CARTESIAN_POINT('Ctrl Pts',(-17.5830877907652,65.7618688136113,33.334983849367));
#31489=CARTESIAN_POINT('Ctrl Pts',(-18.8891762685279,63.8403144380744,33.2238507313753));
#31490=CARTESIAN_POINT('Ctrl Pts',(-21.2119343469181,63.8953892930382,33.1127176133839));
#31491=CARTESIAN_POINT('Ctrl Pts',(-22.4254824097437,65.8766867037682,33.0015844953922));
#31492=CARTESIAN_POINT('Ctrl Pts',(-21.4191335051115,67.9708452967313,32.8904513774008));
#31493=CARTESIAN_POINT('Ctrl Pts',(-19.1139377600523,68.2612087024321,32.7793182594091));
#31494=CARTESIAN_POINT('Ctrl Pts',(-17.6197010520624,66.4820249033491,32.6681851414176));
#31495=CARTESIAN_POINT('Ctrl Pts',(-18.304007628879,64.2616729404111,32.557052023426));
#31496=CARTESIAN_POINT('Ctrl Pts',(-20.5405531773546,63.6323063222924,32.4459189054345));
#31497=CARTESIAN_POINT('Ctrl Pts',(-22.2823631819496,65.1699461495282,32.3347857874429));
#31498=CARTESIAN_POINT('Ctrl Pts',(-21.9352645694849,67.4672839313162,32.2236526694514));
#31499=CARTESIAN_POINT('Ctrl Pts',(-19.8169356517564,68.4217057074312,32.1125195514598));
#31500=CARTESIAN_POINT('Ctrl Pts',(-17.866154430883,67.1596871026972,32.0013864334682));
#31501=CARTESIAN_POINT('Ctrl Pts',(-17.8683526622086,64.8362772167352,31.8902533154766));
#31502=CARTESIAN_POINT('Ctrl Pts',(-19.8215184379026,63.5779522256995,31.7791201974851));
#31503=CARTESIAN_POINT('Ctrl Pts',(-21.9380375641939,64.5363806885751,31.6679870794935));
#31504=CARTESIAN_POINT('Ctrl Pts',(-22.2807884313198,66.8343711527615,31.556853961502));
#31505=CARTESIAN_POINT('Ctrl Pts',(-20.5360719551439,68.3687122974119,31.4457208435104));
#31506=CARTESIAN_POINT('Ctrl Pts',(-18.3007213260338,67.7351147158636,31.3345877255189));
#31507=CARTESIAN_POINT('Ctrl Pts',(-17.6206174222944,65.513471852907,31.2234546075273));
#31508=CARTESIAN_POINT('Ctrl Pts',(-19.1182181052569,63.7371186997313,31.1123214895358));
#31509=CARTESIAN_POINT('Ctrl Pts',(-21.4228602848854,64.0318435787015,31.0011883715442));
#31510=CARTESIAN_POINT('Ctrl Pts',(-22.4252447285517,66.127902680326,30.8900552535526));
#31511=CARTESIAN_POINT('Ctrl Pts',(-21.2079497399452,68.1069002147157,30.778922135561));
#31512=CARTESIAN_POINT('Ctrl Pts',(-18.8850916049024,68.1575797458132,30.6677890175695));
#31513=CARTESIAN_POINT('Ctrl Pts',(-17.5826415154197,66.2335573720312,30.5566558995779));
#31514=CARTESIAN_POINT('Ctrl Pts',(-18.4926530573277,64.0957740986377,30.4455227815864));
#31515=CARTESIAN_POINT('Ctrl Pts',(-20.7822478497669,63.7008133197721,30.3343896635948));
#31516=CARTESIAN_POINT('Ctrl Pts',(-22.3558986211242,65.410158685757,30.2232565456033));
#31517=CARTESIAN_POINT('Ctrl Pts',(-21.7733382471624,67.659350038465,30.1121234276117));
#31518=CARTESIAN_POINT('Ctrl Pts',(-19.5677489114844,68.3898389245888,30.0009903096202));
#31519=CARTESIAN_POINT('Ctrl Pts',(-17.7577727852529,66.9330531637854,29.8898571916286));
#31520=CARTESIAN_POINT('Ctrl Pts',(-17.9999712591612,64.6223004228711,29.7787240736371));
#31521=CARTESIAN_POINT('Ctrl Pts',(-20.0726747570493,63.5724725606719,29.6675909556455));
#31522=CARTESIAN_POINT('Ctrl Pts',(-22.0788634568353,64.7444133574949,29.5564578376539));
#31523=CARTESIAN_POINT('Ctrl Pts',(-22.1823944976574,67.0655164689471,29.4453247196624));
#31524=CARTESIAN_POINT('Ctrl Pts',(-20.288512196013,68.4114169696994,29.3341916016708));
#31525=CARTESIAN_POINT('Ctrl Pts',(-18.1305721768482,67.5502937473358,29.2230584836793));
#31526=CARTESIAN_POINT('Ctrl Pts',(-17.683606081394,65.270280668443,29.1119253656876));
#31527=CARTESIAN_POINT('Ctrl Pts',(-19.3566948726244,63.6581354432645,29.0007922476961));
#31528=CARTESIAN_POINT('Ctrl Pts',(-21.6185618366717,64.1893568353006,28.8896591297046));
#31529=CARTESIAN_POINT('Ctrl Pts',(-22.3990573018246,66.3777501178906,28.778526011713));
#31530=CARTESIAN_POINT('Ctrl Pts',(-20.9838410983712,68.2204116244866,28.6673928937214));
#31531=CARTESIAN_POINT('Ctrl Pts',(-18.6681747980826,68.0308650178038,28.5562597757299));
#31532=CARTESIAN_POINT('Ctrl Pts',(-17.5714473427131,65.9825908127564,28.4451266577384));
#31533=CARTESIAN_POINT('Ctrl Pts',(-18.6974268662034,63.9502501810978,28.3339935397467));
#31534=CARTESIAN_POINT('Ctrl Pts',(-21.015572590504,63.7939212610561,28.2228604217552));
#31535=CARTESIAN_POINT('Ctrl Pts',(-22.4042263074661,65.6566824333273,28.1117273037636));
#31536=CARTESIAN_POINT('Ctrl Pts',(-21.5924374783333,67.8336613554281,28.0005941857721));
#31537=CARTESIAN_POINT('Ctrl Pts',(-19.3231871914542,68.3324012329073,27.8894610677805));
#31538=CARTESIAN_POINT('Ctrl Pts',(-17.6733826257443,66.6964356994646,27.778327949789));
#31539=CARTESIAN_POINT('Ctrl Pts',(-18.1529898563275,64.4230648027232,27.6671948317974));
#31540=CARTESIAN_POINT('Ctrl Pts',(-20.3230534668011,63.5929670655095,27.5560617138059));
#31541=CARTESIAN_POINT('Ctrl Pts',(-22.1974458316091,64.9658806109998,27.4449285958143));
#31542=CARTESIAN_POINT('Ctrl Pts',(-22.0606492758959,67.2852609215228,27.3337954778227));
#31543=CARTESIAN_POINT('Ctrl Pts',(-20.0378654061023,68.4283198539221,27.2226623598312));
#31544=CARTESIAN_POINT('Ctrl Pts',(-17.980425607167,67.3488848690413,27.1115292418396));
#31545=CARTESIAN_POINT('Ctrl Pts',(-17.7713798203235,65.0348973788296,27.0003961238481));
#31546=CARTESIAN_POINT('Ctrl Pts',(-19.6020548636007,63.6042097568846,26.8892630058565));
#31547=CARTESIAN_POINT('Ctrl Pts',(-21.7969451101088,64.3662437359872,26.778129887865));
#31548=CARTESIAN_POINT('Ctrl Pts',(-22.3472001628695,66.6235556060692,26.6669967698734));
#31549=CARTESIAN_POINT('Ctrl Pts',(-20.7492058435804,68.3101651333771,26.5558636518819));
#31550=CARTESIAN_POINT('Ctrl Pts',(-18.4655076477758,67.8824200236192,26.4447305338902));
#31551=CARTESIAN_POINT('Ctrl Pts',(-17.5862396422193,65.7318111728283,26.3335974158987));
#31552=CARTESIAN_POINT('Ctrl Pts',(-18.9161353509539,63.8266569879394,26.2224642979071));
#31553=CARTESIAN_POINT('Ctrl Pts',(-21.2380361565659,63.9106364641676,26.1113311799156));
#31554=CARTESIAN_POINT('Ctrl Pts',(-22.4268185839031,65.9068745248573,26.000198061924));
#31555=CARTESIAN_POINT('Ctrl Pts',(-21.3945189233201,67.988362948155,25.8890649439324));
#31556=CARTESIAN_POINT('Ctrl Pts',(-19.0858252973621,68.2499869305541,25.777931825941));
#31557=CARTESIAN_POINT('Ctrl Pts',(-17.6139705839552,66.4524069049006,25.6667987079493));
#31558=CARTESIAN_POINT('Ctrl Pts',(-18.3256043606965,64.2406215522943,25.5556655899578));
#31559=CARTESIAN_POINT('Ctrl Pts',(-20.5703082087302,63.6393771341005,25.4445324719662));
#31560=CARTESIAN_POINT('Ctrl Pts',(-22.2918517349237,65.1980924141684,25.3333993539747));
#31561=CARTESIAN_POINT('Ctrl Pts',(-21.9181916318134,67.4918921649695,25.2222662359831));
#31562=CARTESIAN_POINT('Ctrl Pts',(-19.7840045183826,68.4179596733709,25.1111331179915));
#31563=CARTESIAN_POINT('Ctrl Pts',(-18.5013225746364,67.5629326473987,25.0370443726639));
#31564=CARTESIAN_POINT('Ctrl Pts',(-18.1825721112405,66.9586205879592,25.));
#31565=CARTESIAN_POINT('Ctrl Pts',(-18.7309291201477,67.0793586530486,36.));
#31566=CARTESIAN_POINT('Ctrl Pts',(-18.6855998783608,67.037071281398,36.));
#31567=CARTESIAN_POINT('Ctrl Pts',(-18.6430006396261,66.9922147972381,36.));
#31568=CARTESIAN_POINT('Ctrl Pts',(-18.6031299258315,66.9451342242319,36.));
#31569=CARTESIAN_POINT('Ctrl Pts',(-18.5606276474992,66.8949462183622,36.));
#31570=CARTESIAN_POINT('Ctrl Pts',(-18.5212252344066,66.8422306107827,36.));
#31571=CARTESIAN_POINT('Ctrl Pts',(-18.4849497284356,66.7873506353329,36.));
#31572=CARTESIAN_POINT('Ctrl Pts',(-18.4532086607109,66.7393306568143,36.));
#31573=CARTESIAN_POINT('Ctrl Pts',(-18.4238618746648,66.6896523585445,36.));
#31574=CARTESIAN_POINT('Ctrl Pts',(-18.3969503791963,66.6385315246993,36.));
#31575=CARTESIAN_POINT('Ctrl Pts',(-18.3834500893461,66.6128864959755,36.));
#31576=CARTESIAN_POINT('Ctrl Pts',(-18.3705630201934,66.5868780860802,36.));
#31577=CARTESIAN_POINT('Ctrl Pts',(-18.3582966902476,66.5605316957194,36.));
#31578=CARTESIAN_POINT('Ctrl Pts',(-18.3526877469073,66.5484844565366,36.));
#31579=CARTESIAN_POINT('Ctrl Pts',(-18.3472080157328,66.5363648649589,36.));
#31580=CARTESIAN_POINT('Ctrl Pts',(-18.3418667280703,66.5241953083072,36.));
#31581=CARTESIAN_POINT('Ctrl Pts',(-18.3149477441457,66.462863262446,36.));
#31582=CARTESIAN_POINT('Ctrl Pts',(-18.2914899255357,66.4001557545952,36.));
#31583=CARTESIAN_POINT('Ctrl Pts',(-18.2715167789656,66.336430550718,36.));
#31584=CARTESIAN_POINT('Ctrl Pts',(-18.2511893221814,66.2715749044961,36.));
#31585=CARTESIAN_POINT('Ctrl Pts',(-18.2344707080506,66.2056642940756,36.));
#31586=CARTESIAN_POINT('Ctrl Pts',(-18.2214250327644,66.1390393524431,36.));
#31587=CARTESIAN_POINT('Ctrl Pts',(-18.2105137796048,66.0833150155311,36.));
#31588=CARTESIAN_POINT('Ctrl Pts',(-18.2021724702928,66.0270900300921,36.));
#31589=CARTESIAN_POINT('Ctrl Pts',(-18.1964634312906,65.9705514121168,36.));
#31590=CARTESIAN_POINT('Ctrl Pts',(-18.1938337965334,65.9445092157172,36.));
#31591=CARTESIAN_POINT('Ctrl Pts',(-18.1917629610617,65.9184003657446,36.));
#31592=CARTESIAN_POINT('Ctrl Pts',(-18.1902588173323,65.8922427368446,36.));
#31593=CARTESIAN_POINT('Ctrl Pts',(-18.1896014517996,65.8808109013618,36.));
#31594=CARTESIAN_POINT('Ctrl Pts',(-18.1890524419704,65.8693699541686,36.));
#31595=CARTESIAN_POINT('Ctrl Pts',(-18.1886127813066,65.857935522043,36.));
#31596=CARTESIAN_POINT('Ctrl Pts',(-18.1859163883022,65.7878093421686,36.));
#31597=CARTESIAN_POINT('Ctrl Pts',(-18.1873207361518,65.7177968496091,36.));
#31598=CARTESIAN_POINT('Ctrl Pts',(-18.1928804564878,65.6482588440327,36.));
#31599=CARTESIAN_POINT('Ctrl Pts',(-18.1978500052571,65.5861023884661,36.));
#31600=CARTESIAN_POINT('Ctrl Pts',(-18.2061399035841,65.5243240681204,36.));
#31601=CARTESIAN_POINT('Ctrl Pts',(-18.2178222762375,65.4631694203924,36.));
#31602=CARTESIAN_POINT('Ctrl Pts',(-18.2305527201426,65.3965283505056,36.));
#31603=CARTESIAN_POINT('Ctrl Pts',(-18.2473105590726,65.3306270439365,36.));
#31604=CARTESIAN_POINT('Ctrl Pts',(-18.2678505607771,65.2656790787157,36.));
#31605=CARTESIAN_POINT('Ctrl Pts',(-18.2757799272864,65.2406062365768,36.));
#31606=CARTESIAN_POINT('Ctrl Pts',(-18.2842735067606,65.2156755188473,36.));
#31607=CARTESIAN_POINT('Ctrl Pts',(-18.2933192003048,65.1908995337231,36.));
#31608=CARTESIAN_POINT('Ctrl Pts',(-18.2972865790838,65.1800329575862,36.));
#31609=CARTESIAN_POINT('Ctrl Pts',(-18.3013600630916,65.1691967138699,36.));
#31610=CARTESIAN_POINT('Ctrl Pts',(-18.3055335461828,65.1584044028859,36.));
#31611=CARTESIAN_POINT('Ctrl Pts',(-18.3307563695742,65.0931800931219,36.));
#31612=CARTESIAN_POINT('Ctrl Pts',(-18.3596700145117,65.0294411884365,36.));
#31613=CARTESIAN_POINT('Ctrl Pts',(-18.3919618229701,64.9674064946292,36.));
#31614=CARTESIAN_POINT('Ctrl Pts',(-18.4250016473144,64.903934812971,36.));
#31615=CARTESIAN_POINT('Ctrl Pts',(-18.461578255366,64.8422463908931,36.));
#31616=CARTESIAN_POINT('Ctrl Pts',(-18.5014128922655,64.7825793081379,36.));
#31617=CARTESIAN_POINT('Ctrl Pts',(-18.5319056213951,64.7369051829538,36.));
#31618=CARTESIAN_POINT('Ctrl Pts',(-18.5643086534008,64.6924154573582,36.));
#31619=CARTESIAN_POINT('Ctrl Pts',(-18.5985165024735,64.6492230243908,36.));
#31620=CARTESIAN_POINT('Ctrl Pts',(-18.6198130829703,64.6223329640543,36.));
#31621=CARTESIAN_POINT('Ctrl Pts',(-18.6418095092061,64.5959458391794,36.));
#31622=CARTESIAN_POINT('Ctrl Pts',(-18.6644832354918,64.570090580138,36.));
#31623=CARTESIAN_POINT('Ctrl Pts',(-18.6771613061568,64.5556335474889,36.));
#31624=CARTESIAN_POINT('Ctrl Pts',(-18.6900556017823,64.5413382714678,36.));
#31625=CARTESIAN_POINT('Ctrl Pts',(-18.7031384975848,64.5272352145414,36.));
#31626=CARTESIAN_POINT('Ctrl Pts',(-18.7540097800711,64.4723971569995,36.));
#31627=CARTESIAN_POINT('Ctrl Pts',(-18.8077776043746,64.4204040417605,36.));
#31628=CARTESIAN_POINT('Ctrl Pts',(-18.8641570225205,64.3715197896026,36.));
#31629=CARTESIAN_POINT('Ctrl Pts',(-18.9063166280107,64.3349649464802,36.));
#31630=CARTESIAN_POINT('Ctrl Pts',(-18.9499377420014,64.3001487169774,36.));
#31631=CARTESIAN_POINT('Ctrl Pts',(-18.9949176029387,64.2671912029343,36.));
#31632=CARTESIAN_POINT('Ctrl Pts',(-19.0089812491819,64.2568865286001,36.));
#31633=CARTESIAN_POINT('Ctrl Pts',(-19.0231778186317,64.2467636385533,36.));
#31634=CARTESIAN_POINT('Ctrl Pts',(-19.0375044116818,64.2368264306734,36.));
#31635=CARTESIAN_POINT('Ctrl Pts',(-19.0512937814086,64.2272618515002,36.));
#31636=CARTESIAN_POINT('Ctrl Pts',(-19.0651965653016,64.2178742367791,36.));
#31637=CARTESIAN_POINT('Ctrl Pts',(-19.0792048040081,64.2086698030378,36.));
#31638=CARTESIAN_POINT('Ctrl Pts',(-19.142158533753,64.1673046145694,36.));
#31639=CARTESIAN_POINT('Ctrl Pts',(-19.2072697134705,64.1296151054152,36.));
#31640=CARTESIAN_POINT('Ctrl Pts',(-19.274277057303,64.0958804445685,36.));
#31641=CARTESIAN_POINT('Ctrl Pts',(-19.3255044901851,64.070090135992,36.));
#31642=CARTESIAN_POINT('Ctrl Pts',(-19.3778411434284,64.0466117153907,36.));
#31643=CARTESIAN_POINT('Ctrl Pts',(-19.4311841342659,64.0255851777059,36.));
#31644=CARTESIAN_POINT('Ctrl Pts',(-19.4436313822641,64.0206787687289,36.));
#31645=CARTESIAN_POINT('Ctrl Pts',(-19.4561334688371,64.0159059301644,36.));
#31646=CARTESIAN_POINT('Ctrl Pts',(-19.4686884555734,64.0112660732732,36.));
#31647=CARTESIAN_POINT('Ctrl Pts',(-21.6673174487995,65.9986976755605,34.8714803633902));
#31648=CARTESIAN_POINT('Ctrl Pts',(-21.6680517344582,65.9132137702119,34.8772098489549));
#31649=CARTESIAN_POINT('Ctrl Pts',(-21.6620451159422,65.8278333924919,34.8829393345197));
#31650=CARTESIAN_POINT('Ctrl Pts',(-21.6489385509365,65.7435572785707,34.8886688200844));
#31651=CARTESIAN_POINT('Ctrl Pts',(-21.5641971770511,65.1986644194321,34.9257131927483));
#31652=CARTESIAN_POINT('Ctrl Pts',(-21.1826527900964,64.6999337142113,34.9627575654121));
#31653=CARTESIAN_POINT('Ctrl Pts',(-20.6789070192068,64.4755856508596,34.999801938076));
#31654=CARTESIAN_POINT('Ctrl Pts',(-20.1751612483172,64.2512375875079,35.0368463107398));
#31655=CARTESIAN_POINT('Ctrl Pts',(-19.5492140934925,64.3012721660255,35.0738906834037));
#31656=CARTESIAN_POINT('Ctrl Pts',(-19.0875124696833,64.6028095203746,35.1109350560675));
#31657=CARTESIAN_POINT('Ctrl Pts',(-18.625810845874,64.9043468747237,35.1479794287314));
#31658=CARTESIAN_POINT('Ctrl Pts',(-18.3283547530802,65.4573870049044,35.1850238013952));
#31659=CARTESIAN_POINT('Ctrl Pts',(-18.331263603936,66.0088140869061,35.2220681740591));
#31660=CARTESIAN_POINT('Ctrl Pts',(-18.3341724547918,66.5602411689079,35.2591125467229));
#31661=CARTESIAN_POINT('Ctrl Pts',(-18.6374462492973,67.1100552027307,35.2961569193868));
#31662=CARTESIAN_POINT('Ctrl Pts',(-19.1023056141942,67.4067178074562,35.3332012920506));
#31663=CARTESIAN_POINT('Ctrl Pts',(-19.567164979091,67.7033804121818,35.3702456647145));
#31664=CARTESIAN_POINT('Ctrl Pts',(-20.1936099143791,67.7468915878102,35.4072900373783));
#31665=CARTESIAN_POINT('Ctrl Pts',(-20.6949575560159,67.5172054957391,35.4443344100422));
#31666=CARTESIAN_POINT('Ctrl Pts',(-21.1963051976527,67.287519403668,35.4813787827061));
#31667=CARTESIAN_POINT('Ctrl Pts',(-21.5725555456381,66.7846360438976,35.5184231553699));
#31668=CARTESIAN_POINT('Ctrl Pts',(-21.6515475919844,66.2389525662666,35.5554675280338));
#31669=CARTESIAN_POINT('Ctrl Pts',(-21.6629293173915,66.1603266819043,35.5608051398192));
#31670=CARTESIAN_POINT('Ctrl Pts',(-21.6681396460096,66.0808122218201,35.5661427516047));
#31671=CARTESIAN_POINT('Ctrl Pts',(-21.6674772588494,66.0012131718681,35.5714803633902));
#31672=CARTESIAN_POINT('Ctrl Pts',(-20.5301702171886,64.0148256743283,36.));
#31673=CARTESIAN_POINT('Ctrl Pts',(-21.1902595624181,64.1911123142463,35.9629556273362));
#31674=CARTESIAN_POINT('Ctrl Pts',(-22.3092728128736,65.2513736304872,35.8888668820085));
#31675=CARTESIAN_POINT('Ctrl Pts',(-21.8813251479519,67.5381211991997,35.7777337640168));
#31676=CARTESIAN_POINT('Ctrl Pts',(-19.7281828950178,68.4128315562992,35.6666006460254));
#31677=CARTESIAN_POINT('Ctrl Pts',(-17.8254683675795,67.0812973613349,35.5554675280337));
#31678=CARTESIAN_POINT('Ctrl Pts',(-17.9121447447308,64.7590835038729,35.4443344100422));
#31679=CARTESIAN_POINT('Ctrl Pts',(-19.9101226209547,63.5731232768953,35.3332012920507));
#31680=CARTESIAN_POINT('Ctrl Pts',(-21.9901520744513,64.6080763665066,35.2220681740591));
#31681=CARTESIAN_POINT('Ctrl Pts',(-22.2488202123297,66.9171030470485,35.1109350560676));
#31682=CARTESIAN_POINT('Ctrl Pts',(-20.4492273182073,68.3866955695652,34.999801938076));
#31683=CARTESIAN_POINT('Ctrl Pts',(-18.2385101136685,67.6719231463612,34.8886688200844));
#31684=CARTESIAN_POINT('Ctrl Pts',(-17.6399646371577,65.4269244123525,34.7775357020929));
#31685=CARTESIAN_POINT('Ctrl Pts',(-19.2014230092252,63.706435258535,34.6664025841013));
#31686=CARTESIAN_POINT('Ctrl Pts',(-21.4937671673603,64.0851026938035,34.5552694661097));
#31687=CARTESIAN_POINT('Ctrl Pts',(-22.4189584788097,66.2163615878931,34.4441363481182));
#31688=CARTESIAN_POINT('Ctrl Pts',(-21.1302229490745,68.1495968002898,34.3330032301266));
#31689=CARTESIAN_POINT('Ctrl Pts',(-18.8070633085623,68.1154369356633,34.2218701121351));
#31690=CARTESIAN_POINT('Ctrl Pts',(-17.5757260722497,66.1451456629571,34.1107369941435));
#31691=CARTESIAN_POINT('Ctrl Pts',(-18.5631798581025,64.0420114979335,33.999603876152));
#31692=CARTESIAN_POINT('Ctrl Pts',(-20.8656679378464,63.730905409822,33.8884707581604));
#31693=CARTESIAN_POINT('Ctrl Pts',(-22.3758626749296,65.4965640343655,33.7773376401688));
#31694=CARTESIAN_POINT('Ctrl Pts',(-21.7115743656249,67.7229870531365,33.6662045221772));
#31695=CARTESIAN_POINT('Ctrl Pts',(-19.4807858366348,68.3724645130774,33.5550714041857));
#31696=CARTESIAN_POINT('Ctrl Pts',(-17.7252025426939,66.8505690671885,33.4439382861941));
#31697=CARTESIAN_POINT('Ctrl Pts',(-18.0516034185067,64.550199335027,33.3328051682026));
#31698=CARTESIAN_POINT('Ctrl Pts',(-20.1612535330058,63.5767442339982,33.221672050211));
#31699=CARTESIAN_POINT('Ctrl Pts',(-22.1233180676414,64.821148188958,33.1105389322195));
#31700=CARTESIAN_POINT('Ctrl Pts',(-22.1420383335758,67.1444837202745,32.9994058142279));
#31701=CARTESIAN_POINT('Ctrl Pts',(-20.2002808069203,68.4203427044879,32.8882726962364));
#31702=CARTESIAN_POINT('Ctrl Pts',(-18.0752184027424,67.4810087817272,32.7771395782448));
#31703=CARTESIAN_POINT('Ctrl Pts',(-17.7117918750668,65.1861973300252,32.6660064602532));
#31704=CARTESIAN_POINT('Ctrl Pts',(-19.4426234863108,63.6362101128286,32.5548733422617));
#31705=CARTESIAN_POINT('Ctrl Pts',(-21.6835880210157,64.2496564382428,32.4437402242701));
#31706=CARTESIAN_POINT('Ctrl Pts',(-22.3836665335049,66.4650860842244,32.3326071062786));
#31707=CARTESIAN_POINT('Ctrl Pts',(-20.9021196143316,68.2548506403159,32.221473988287));
#31708=CARTESIAN_POINT('Ctrl Pts',(-18.5949173170392,67.9808871403329,32.1103408702954));
#31709=CARTESIAN_POINT('Ctrl Pts',(-17.5737019947084,65.8939377625597,31.9992077523039));
#31710=CARTESIAN_POINT('Ctrl Pts',(-18.7731301049792,63.9040607190605,31.8880746343123));
#31711=CARTESIAN_POINT('Ctrl Pts',(-21.0954378323017,63.8324698008436,31.7769415163208));
#31712=CARTESIAN_POINT('Ctrl Pts',(-22.4151577394886,65.7446878340517,31.6658083983292));
#31713=CARTESIAN_POINT('Ctrl Pts',(-21.5244302238133,67.8905776105247,31.5546752803377));
#31714=CARTESIAN_POINT('Ctrl Pts',(-19.2384841663151,68.3061363454358,31.4435421623461));
#31715=CARTESIAN_POINT('Ctrl Pts',(-17.6495073727765,66.611028328362,31.3324090443545));
#31716=CARTESIAN_POINT('Ctrl Pts',(-18.2117939461611,64.3566831353306,31.221275926363));
#31717=CARTESIAN_POINT('Ctrl Pts',(-20.4107170831235,63.6063662171661,31.1101428083713));
#31718=CARTESIAN_POINT('Ctrl Pts',(-22.2337357799444,65.0467971495588,30.9990096903799));
#31719=CARTESIAN_POINT('Ctrl Pts',(-22.0123515719766,67.3596368483739,30.8878765723882));
#31720=CARTESIAN_POINT('Ctrl Pts',(-19.9491839999498,68.4280833887723,30.7767434543968));
#31721=CARTESIAN_POINT('Ctrl Pts',(-17.9325252312672,67.2742524433354,30.6656103364051));
#31722=CARTESIAN_POINT('Ctrl Pts',(-17.8081007459427,64.9541755076705,30.5544772184136));
#31723=CARTESIAN_POINT('Ctrl Pts',(-19.6897887302455,63.5912783106364,30.4433441004221));
#31724=CARTESIAN_POINT('Ctrl Pts',(-21.8553942784241,64.4329380100698,30.3322109824304));
#31725=CARTESIAN_POINT('Ctrl Pts',(-22.3228699553819,66.7088345216461,30.221077864439));
#31726=CARTESIAN_POINT('Ctrl Pts',(-20.6643636219036,68.335977779557,30.1099447464473));
#31727=CARTESIAN_POINT('Ctrl Pts',(-18.3978055525618,67.8251422304279,29.9988116284558));
#31728=CARTESIAN_POINT('Ctrl Pts',(-17.5976389032744,65.643864675113,29.8876785104642));
#31729=CARTESIAN_POINT('Ctrl Pts',(-18.9962076857216,63.7885361864844,29.7765453924727));
#31730=CARTESIAN_POINT('Ctrl Pts',(-21.3134867030769,63.9572264223528,29.6654122744811));
#31731=CARTESIAN_POINT('Ctrl Pts',(-22.4286109914434,65.9955434392686,29.5542791564896));
#31732=CARTESIAN_POINT('Ctrl Pts',(-21.3209749112437,68.037939275974,29.4431460384979));
#31733=CARTESIAN_POINT('Ctrl Pts',(-19.0043305992079,68.2151328748,29.3320129205065));
#31734=CARTESIAN_POINT('Ctrl Pts',(-17.5989621119428,66.3649496798285,29.2208798025149));
#31735=CARTESIAN_POINT('Ctrl Pts',(-18.391118003758,64.1807501735986,29.1097466845233));
#31736=CARTESIAN_POINT('Ctrl Pts',(-20.6557860235121,63.6615997134667,28.9986135665318));
#31737=CARTESIAN_POINT('Ctrl Pts',(-22.3202528630616,65.2826452341084,28.8874804485401));
#31738=CARTESIAN_POINT('Ctrl Pts',(-21.8611329580743,67.5602420713026,28.7763473305487));
#31739=CARTESIAN_POINT('Ctrl Pts',(-19.6986309163782,68.4098439543111,28.665214212557));
#31740=CARTESIAN_POINT('Ctrl Pts',(-17.8119537217837,67.0538617998004,28.5540810945656));
#31741=CARTESIAN_POINT('Ctrl Pts',(-17.9278626016764,64.733343846516,28.442947976574));
#31742=CARTESIAN_POINT('Ctrl Pts',(-19.9402731870454,63.5721194600009,28.3318148585824));
#31743=CARTESIAN_POINT('Ctrl Pts',(-22.0073481024602,64.6329869041389,28.2206817405909));
#31744=CARTESIAN_POINT('Ctrl Pts',(-22.2372190260415,66.944998538722,28.1095486225993));
#31745=CARTESIAN_POINT('Ctrl Pts',(-20.4194990409278,68.3921103158831,27.9984155046077));
#31746=CARTESIAN_POINT('Ctrl Pts',(-18.2178370221936,67.6498685794103,27.8872823866162));
#31747=CARTESIAN_POINT('Ctrl Pts',(-17.647280706083,65.3976021808533,27.7761492686246));
#31748=CARTESIAN_POINT('Ctrl Pts',(-19.2300256897269,63.6966739765529,27.6650161506331));
#31749=CARTESIAN_POINT('Ctrl Pts',(-21.51748146836,64.1038404068878,27.5538830326415));
#31750=CARTESIAN_POINT('Ctrl Pts',(-22.4160784789961,66.2464467290574,27.44274991465));
#31751=CARTESIAN_POINT('Ctrl Pts',(-21.1033853710592,68.1634953045376,27.3316167966584));
#31752=CARTESIAN_POINT('Ctrl Pts',(-18.7808305400592,68.1004278233727,27.2204836786668));
#31753=CARTESIAN_POINT('Ctrl Pts',(-17.5741075901122,66.1149661254002,27.1093505606753));
#31754=CARTESIAN_POINT('Ctrl Pts',(-18.5876568453766,64.0242829060802,26.9982174426837));
#31755=CARTESIAN_POINT('Ctrl Pts',(-20.8938381659967,63.7418537313102,26.8870843246922));
#31756=CARTESIAN_POINT('Ctrl Pts',(-22.3819435741815,65.5261689079406,26.7759512067006));
#31757=CARTESIAN_POINT('Ctrl Pts',(-21.6900005542035,67.7441529368256,26.664818088709));
#31758=CARTESIAN_POINT('Ctrl Pts',(-19.4513023431397,68.3658195746722,26.5536849707175));
#31759=CARTESIAN_POINT('Ctrl Pts',(-17.714794155333,66.8221949683201,26.4425518527259));
#31760=CARTESIAN_POINT('Ctrl Pts',(-18.0697956411282,64.5260652687741,26.3314187347344));
#31761=CARTESIAN_POINT('Ctrl Pts',(-20.1913974446539,63.5789384432151,26.2202856167427));
#31762=CARTESIAN_POINT('Ctrl Pts',(-22.1378221489769,64.8476628562653,26.1091524987513));
#31763=CARTESIAN_POINT('Ctrl Pts',(-22.127633111299,67.1710507618066,25.9980193807596));
#31764=CARTESIAN_POINT('Ctrl Pts',(-20.1701400749251,68.4226485469194,25.8868862627681));
#31765=CARTESIAN_POINT('Ctrl Pts',(-18.0569489447748,67.4569397798106,25.7757531447766));
#31766=CARTESIAN_POINT('Ctrl Pts',(-17.7220731495743,65.1577888564038,25.664620026785));
#31767=CARTESIAN_POINT('Ctrl Pts',(-19.4721283434274,63.6294498117299,25.5534869087935));
#31768=CARTESIAN_POINT('Ctrl Pts',(-21.7051476175159,64.2707573406571,25.4423537908019));
#31769=CARTESIAN_POINT('Ctrl Pts',(-22.3778773235377,66.4946844969483,25.3312206728103));
#31770=CARTESIAN_POINT('Ctrl Pts',(-20.8736248136923,68.2659592866881,25.2200875548188));
#31771=CARTESIAN_POINT('Ctrl Pts',(-18.5711038201239,67.9631343216322,25.1089544368272));
#31772=CARTESIAN_POINT('Ctrl Pts',(-17.5737474231758,65.8639868785843,24.9978213188357));
#31773=CARTESIAN_POINT('Ctrl Pts',(-18.8023459831469,63.888411209226,24.8866882008441));
#31774=CARTESIAN_POINT('Ctrl Pts',(-20.343660854084,63.8620828587222,24.8125994555164));
#31775=CARTESIAN_POINT('Ctrl Pts',(-20.9495535522615,64.1778184465077,24.7755550828525));
#31776=CARTESIAN_POINT('Ctrl Pts',(-20.4967348970876,64.1400211999972,36.0748149723825));
#31777=CARTESIAN_POINT('Ctrl Pts',(-21.1151955392376,64.3051902779623,36.0377705997186));
#31778=CARTESIAN_POINT('Ctrl Pts',(-22.163637933366,65.2985859436069,35.9636818543909));
#31779=CARTESIAN_POINT('Ctrl Pts',(-21.7626788971888,67.4411191930855,35.8525487363994));
#31780=CARTESIAN_POINT('Ctrl Pts',(-19.7453251101392,68.2606657181987,35.7414156184078));
#31781=CARTESIAN_POINT('Ctrl Pts',(-17.962605760142,67.0131050671841,35.6302825004162));
#31782=CARTESIAN_POINT('Ctrl Pts',(-18.0438158694395,64.8373422195106,35.5191493824247));
#31783=CARTESIAN_POINT('Ctrl Pts',(-19.9157907608102,63.7261748770262,35.4080162644331));
#31784=CARTESIAN_POINT('Ctrl Pts',(-21.8646426257847,64.6958583858148,35.2968831464416));
#31785=CARTESIAN_POINT('Ctrl Pts',(-22.1069977915091,66.8592657092475,35.18575002845));
#31786=CARTESIAN_POINT('Ctrl Pts',(-20.4208966826956,68.2361780041406,35.0746169104584));
#31787=CARTESIAN_POINT('Ctrl Pts',(-18.3495989230632,67.5664828862893,34.9634837924669));
#31788=CARTESIAN_POINT('Ctrl Pts',(-17.7888008698389,65.4630655705954,34.8523506744753));
#31789=CARTESIAN_POINT('Ctrl Pts',(-19.2517854710274,63.8510795045088,34.7412175564838));
#31790=CARTESIAN_POINT('Ctrl Pts',(-21.3995623595878,64.2058661812974,34.6300844384922));
#31791=CARTESIAN_POINT('Ctrl Pts',(-22.2664062447768,66.2027166891148,34.5189513205007));
#31792=CARTESIAN_POINT('Ctrl Pts',(-21.0589451502421,68.0140319292816,34.4078182025091));
#31793=CARTESIAN_POINT('Ctrl Pts',(-18.8822961655679,67.9820263652388,34.2966850845176));
#31794=CARTESIAN_POINT('Ctrl Pts',(-17.7286135264271,66.1359920146667,34.185551966526));
#31795=CARTESIAN_POINT('Ctrl Pts',(-18.6537932871754,64.1654925426962,34.0744188485344));
#31796=CARTESIAN_POINT('Ctrl Pts',(-20.8110743683388,63.8740064394576,33.9632857305429));
#31797=CARTESIAN_POINT('Ctrl Pts',(-22.2260282887709,65.5283133520668,33.8521526125513));
#31798=CARTESIAN_POINT('Ctrl Pts',(-21.6036334912871,67.6143264347472,33.7410194945597));
#31799=CARTESIAN_POINT('Ctrl Pts',(-19.5135302104043,68.2228444328634,33.6298863765682));
#31800=CARTESIAN_POINT('Ctrl Pts',(-17.868663225101,66.7969277118137,33.5187532585766));
#31801=CARTESIAN_POINT('Ctrl Pts',(-18.1744795463496,64.6416313841015,33.4076201405851));
#31802=CARTESIAN_POINT('Ctrl Pts',(-20.1510840377783,63.7295674775451,33.2964870225935));
#31803=CARTESIAN_POINT('Ctrl Pts',(-21.9894104716166,64.8954927793853,33.1853539046019));
#31804=CARTESIAN_POINT('Ctrl Pts',(-22.0069501392006,67.0723065622656,33.0742207866104));
#31805=CARTESIAN_POINT('Ctrl Pts',(-20.1876500466996,68.2677031739092,32.9630876686188));
#31806=CARTESIAN_POINT('Ctrl Pts',(-18.1966052455756,67.387608584802,32.8519545506273));
#31807=CARTESIAN_POINT('Ctrl Pts',(-17.8560983046515,65.2375200031732,32.7408214326357));
#31808=CARTESIAN_POINT('Ctrl Pts',(-19.4777745784464,63.7852831255451,32.6296883146441));
#31809=CARTESIAN_POINT('Ctrl Pts',(-21.5774121126457,64.3600423018326,32.5185551966526));
#31810=CARTESIAN_POINT('Ctrl Pts',(-22.2333399950128,66.435755311585,32.407422078661));
#31811=CARTESIAN_POINT('Ctrl Pts',(-20.8452272105401,68.1126479090148,32.2962889606695));
#31812=CARTESIAN_POINT('Ctrl Pts',(-18.6835292151616,67.8559619871019,32.1851558426779));
#31813=CARTESIAN_POINT('Ctrl Pts',(-17.7267170978527,65.9006266046419,32.0740227246864));
#31814=CARTESIAN_POINT('Ctrl Pts',(-18.850502968132,64.036241664912,31.9628896066948));
#31815=CARTESIAN_POINT('Ctrl Pts',(-21.0263537657393,63.9691656462299,31.8517564887033));
#31816=CARTESIAN_POINT('Ctrl Pts',(-22.2628452000513,65.7607891609791,31.7406233707116));
#31817=CARTESIAN_POINT('Ctrl Pts',(-21.4282916425573,67.7713478508474,31.6294902527201));
#31818=CARTESIAN_POINT('Ctrl Pts',(-19.2865093567836,68.1606992680479,31.5183571347286));
#31819=CARTESIAN_POINT('Ctrl Pts',(-17.7977417903996,66.5724936708367,31.407224016737));
#31820=CARTESIAN_POINT('Ctrl Pts',(-18.3245676174803,64.4603193329442,31.2960908987455));
#31821=CARTESIAN_POINT('Ctrl Pts',(-20.3848151054191,63.7573213427819,31.1849577807539));
#31822=CARTESIAN_POINT('Ctrl Pts',(-22.0928646627033,65.1069111306771,31.0738246627624));
#31823=CARTESIAN_POINT('Ctrl Pts',(-21.885442106331,67.2738910034122,30.9626915447707));
#31824=CARTESIAN_POINT('Ctrl Pts',(-19.9523887239665,68.274955689963,30.8515584267792));
#31825=CARTESIAN_POINT('Ctrl Pts',(-18.0629110553893,67.1938913876763,30.7404253087876));
#31826=CARTESIAN_POINT('Ctrl Pts',(-17.9463334319978,65.0201306962811,30.6292921907961));
#31827=CARTESIAN_POINT('Ctrl Pts',(-19.7093522831703,63.7431849589295,30.5181590728045));
#31828=CARTESIAN_POINT('Ctrl Pts',(-21.738383364568,64.53176517454,30.407025954813));
#31829=CARTESIAN_POINT('Ctrl Pts',(-22.1763775686106,66.6641316915711,30.2958928368214));
#31830=CARTESIAN_POINT('Ctrl Pts',(-20.6224653604744,68.1886587445077,30.1847597188299));
#31831=CARTESIAN_POINT('Ctrl Pts',(-18.4988483544341,67.7100391697021,30.0736266008383));
#31832=CARTESIAN_POINT('Ctrl Pts',(-17.7491444191688,65.6663244402993,29.9624934828468));
#31833=CARTESIAN_POINT('Ctrl Pts',(-19.0595121042925,63.9280027164766,29.8513603648552));
#31834=CARTESIAN_POINT('Ctrl Pts',(-21.2306513288106,64.0860544595529,29.7402272468636));
#31835=CARTESIAN_POINT('Ctrl Pts',(-22.2754500192369,65.9958244934088,29.6290941288721));
#31836=CARTESIAN_POINT('Ctrl Pts',(-21.2376672912176,67.9094161152432,29.5179610108805));
#31837=CARTESIAN_POINT('Ctrl Pts',(-19.067122744166,68.0754349545212,29.406827892889));
#31838=CARTESIAN_POINT('Ctrl Pts',(-17.7503841793447,66.3419340350975,29.2956947748974));
#31839=CARTESIAN_POINT('Ctrl Pts',(-18.492582557603,64.2954816283601,29.1845616569058));
#31840=CARTESIAN_POINT('Ctrl Pts',(-20.6144287105154,63.8090715245369,29.0734285389143));
#31841=CARTESIAN_POINT('Ctrl Pts',(-22.1739255238857,65.3278853955619,28.9622954209227));
#31842=CARTESIAN_POINT('Ctrl Pts',(-21.7437601329209,67.4618450067418,28.8511623029312));
#31843=CARTESIAN_POINT('Ctrl Pts',(-19.7176368345772,68.2578665300926,28.7400291849396));
#31844=CARTESIAN_POINT('Ctrl Pts',(-17.9499434189336,66.9873997363422,28.628896066948));
#31845=CARTESIAN_POINT('Ctrl Pts',(-18.0585424757241,64.8132258402162,28.5177629489565));
#31846=CARTESIAN_POINT('Ctrl Pts',(-19.9440398737528,63.7252343661005,28.4066298309649));
#31847=CARTESIAN_POINT('Ctrl Pts',(-21.8807541818971,64.7191979340316,28.2954967129734));
#31848=CARTESIAN_POINT('Ctrl Pts',(-22.096128236996,66.8854019646168,28.1843635949818));
#31849=CARTESIAN_POINT('Ctrl Pts',(-20.3930432268125,68.2412512680995,28.0732304769902));
#31850=CARTESIAN_POINT('Ctrl Pts',(-18.3302295853801,67.5458191962338,27.9620973589987));
#31851=CARTESIAN_POINT('Ctrl Pts',(-17.7956555490096,65.4355925531116,27.8509642410071));
#31852=CARTESIAN_POINT('Ctrl Pts',(-19.2785843161808,63.841933820267,27.7398311230155));
#31853=CARTESIAN_POINT('Ctrl Pts',(-21.4217811121406,64.2234221957222,27.628698005024));
#31854=CARTESIAN_POINT('Ctrl Pts',(-22.2637078728867,66.2309045031708,27.5175648870325));
#31855=CARTESIAN_POINT('Ctrl Pts',(-21.0338000909361,68.0270539208107,27.4064317690409));
#31856=CARTESIAN_POINT('Ctrl Pts',(-18.8577177733077,67.9679638064466,27.2952986510493));
#31857=CARTESIAN_POINT('Ctrl Pts',(-17.7270971142788,66.1077157573507,27.1841655330578));
#31858=CARTESIAN_POINT('Ctrl Pts',(-18.6767266269981,64.1488820090142,27.0730324150662));
#31859=CARTESIAN_POINT('Ctrl Pts',(-20.8374680338588,63.8842643022561,26.9618992970747));
#31860=CARTESIAN_POINT('Ctrl Pts',(-22.231725694559,65.5560511867317,26.8507661790831));
#31861=CARTESIAN_POINT('Ctrl Pts',(-21.5834202377908,67.6341574865776,26.7396330610915));
#31862=CARTESIAN_POINT('Ctrl Pts',(-19.4859061009536,68.2166185591953,26.6284999430999));
#31863=CARTESIAN_POINT('Ctrl Pts',(-17.8589112453462,66.7703430327343,26.5173668251085));
#31864=CARTESIAN_POINT('Ctrl Pts',(-18.191524471807,64.6190193388985,26.4062337071168));
#31865=CARTESIAN_POINT('Ctrl Pts',(-20.1793269159424,63.7316233083974,26.2951005891253));
#31866=CARTESIAN_POINT('Ctrl Pts',(-22.0029998493598,64.9203352924298,26.1839674711337));
#31867=CARTESIAN_POINT('Ctrl Pts',(-21.9934533859443,67.0971981465407,26.0728343531422));
#31868=CARTESIAN_POINT('Ctrl Pts',(-20.1594101476628,68.2698635977991,25.9617012351506));
#31869=CARTESIAN_POINT('Ctrl Pts',(-18.1794879556388,67.3650575006361,25.8505681171591));
#31870=CARTESIAN_POINT('Ctrl Pts',(-17.8657311879574,65.2109031171935,25.7394349991675));
#31871=CARTESIAN_POINT('Ctrl Pts',(-19.5054187042162,63.7789491645613,25.6283018811759));
#31872=CARTESIAN_POINT('Ctrl Pts',(-21.5976120476884,64.3798124704489,25.5171687631844));
#31873=CARTESIAN_POINT('Ctrl Pts',(-22.2279158830502,66.4634870928539,25.4060356451928));
#31874=CARTESIAN_POINT('Ctrl Pts',(-20.818529441778,68.1230559857674,25.2949025272013));
#31875=CARTESIAN_POINT('Ctrl Pts',(-18.6612175225089,67.8393287544449,25.1837694092097));
#31876=CARTESIAN_POINT('Ctrl Pts',(-17.7267596613622,65.8725645808109,25.0726362912181));
#31877=CARTESIAN_POINT('Ctrl Pts',(-18.8778763394841,64.0215790954106,24.9615031732266));
#31878=CARTESIAN_POINT('Ctrl Pts',(-20.3219877945836,63.996911149053,24.8874144278989));
#31879=CARTESIAN_POINT('Ctrl Pts',(-20.8896697150645,64.2927347913867,24.850370055235));
#31880=CARTESIAN_POINT('Ctrl Pts',(-20.4632995769867,64.2652167256662,36.149629944765));
#31881=CARTESIAN_POINT('Ctrl Pts',(-21.0401315160572,64.4192682416784,36.1125855721011));
#31882=CARTESIAN_POINT('Ctrl Pts',(-22.0180030538584,65.3457982567266,36.0384968267734));
#31883=CARTESIAN_POINT('Ctrl Pts',(-21.6440326464257,67.3441171869714,35.9273637087819));
#31884=CARTESIAN_POINT('Ctrl Pts',(-19.7624673252605,68.1084998800982,35.8162305907903));
#31885=CARTESIAN_POINT('Ctrl Pts',(-18.0997431527045,66.9449127730333,35.7050974727987));
#31886=CARTESIAN_POINT('Ctrl Pts',(-18.1754869941483,64.9156009351482,35.5939643548072));
#31887=CARTESIAN_POINT('Ctrl Pts',(-19.9214589006656,63.8792264771571,35.4828312368156));
#31888=CARTESIAN_POINT('Ctrl Pts',(-21.7391331771181,64.7836404051231,35.371698118824));
#31889=CARTESIAN_POINT('Ctrl Pts',(-21.9651753706885,66.8014283714463,35.2605650008325));
#31890=CARTESIAN_POINT('Ctrl Pts',(-20.3925660471839,68.0856604387161,35.1494318828409));
#31891=CARTESIAN_POINT('Ctrl Pts',(-18.4606877324579,67.4610426262175,35.0382987648494));
#31892=CARTESIAN_POINT('Ctrl Pts',(-17.93763710252,65.4992067288381,34.9271656468578));
#31893=CARTESIAN_POINT('Ctrl Pts',(-19.3021479328295,63.9957237504828,34.8160325288663));
#31894=CARTESIAN_POINT('Ctrl Pts',(-21.3053575518154,64.3266296687912,34.7048994108747));
#31895=CARTESIAN_POINT('Ctrl Pts',(-22.113854010744,66.1890717903366,34.5937662928832));
#31896=CARTESIAN_POINT('Ctrl Pts',(-20.9876673514096,67.8784670582733,34.4826331748916));
#31897=CARTESIAN_POINT('Ctrl Pts',(-18.9575290225734,67.8486157948143,34.3715000569));
#31898=CARTESIAN_POINT('Ctrl Pts',(-17.8815009806044,66.1268383663763,34.2603669389085));
#31899=CARTESIAN_POINT('Ctrl Pts',(-18.7444067162484,64.2889735874589,34.1492338209169));
#31900=CARTESIAN_POINT('Ctrl Pts',(-20.756480798831,64.0171074690934,34.0381007029254));
#31901=CARTESIAN_POINT('Ctrl Pts',(-22.0761939026122,65.5600626697681,33.9269675849338));
#31902=CARTESIAN_POINT('Ctrl Pts',(-21.4956926169493,67.5056658163578,33.8158344669422));
#31903=CARTESIAN_POINT('Ctrl Pts',(-19.5462745841737,68.0732243526495,33.7047013489507));
#31904=CARTESIAN_POINT('Ctrl Pts',(-18.012123907508,66.7432863564387,33.5935682309591));
#31905=CARTESIAN_POINT('Ctrl Pts',(-18.2973556741925,64.7330634331763,33.4824351129676));
#31906=CARTESIAN_POINT('Ctrl Pts',(-20.1409145425508,63.8823907210918,33.371301994976));
#31907=CARTESIAN_POINT('Ctrl Pts',(-21.8555028755919,64.9698373698129,33.2601688769845));
#31908=CARTESIAN_POINT('Ctrl Pts',(-21.8718619448253,67.0001294042565,33.1490357589929));
#31909=CARTESIAN_POINT('Ctrl Pts',(-20.175019286479,68.1150636433306,33.0379026410013));
#31910=CARTESIAN_POINT('Ctrl Pts',(-18.3179920884086,67.2942083878766,32.9267695230098));
#31911=CARTESIAN_POINT('Ctrl Pts',(-18.0004047342363,65.2888426763213,32.8156364050182));
#31912=CARTESIAN_POINT('Ctrl Pts',(-19.5129256705819,63.9343561382617,32.7045032870267));
#31913=CARTESIAN_POINT('Ctrl Pts',(-21.4712362042757,64.4704281654224,32.5933701690351));
#31914=CARTESIAN_POINT('Ctrl Pts',(-22.0830134565206,66.4064245389456,32.4822370510435));
#31915=CARTESIAN_POINT('Ctrl Pts',(-20.7883348067487,67.9704451777137,32.371103933052));
#31916=CARTESIAN_POINT('Ctrl Pts',(-18.772141113284,67.7310368338708,32.2599708150604));
#31917=CARTESIAN_POINT('Ctrl Pts',(-17.879732200997,65.907315446724,32.1488376970689));
#31918=CARTESIAN_POINT('Ctrl Pts',(-18.9278758312847,64.1684226107636,32.0377045790773));
#31919=CARTESIAN_POINT('Ctrl Pts',(-20.9572696991769,64.105861491616,31.9265714610858));
#31920=CARTESIAN_POINT('Ctrl Pts',(-22.1105326606141,65.7768904879066,31.8154383430941));
#31921=CARTESIAN_POINT('Ctrl Pts',(-21.3321530613013,67.6521180911699,31.7043052251027));
#31922=CARTESIAN_POINT('Ctrl Pts',(-19.334534547252,68.0152621906601,31.593172107111));
#31923=CARTESIAN_POINT('Ctrl Pts',(-17.9459762080226,66.5339590133113,31.4820389891195));
#31924=CARTESIAN_POINT('Ctrl Pts',(-18.4373412887996,64.5639555305579,31.3709058711279));
#31925=CARTESIAN_POINT('Ctrl Pts',(-20.3589131277147,63.9082764683976,31.2597727531364));
#31926=CARTESIAN_POINT('Ctrl Pts',(-21.9519935454622,65.1670251117956,31.1486396351448));
#31927=CARTESIAN_POINT('Ctrl Pts',(-21.7585326406854,67.1881451584504,31.0375065171532));
#31928=CARTESIAN_POINT('Ctrl Pts',(-19.9555934479831,68.1218279911537,30.9263733991617));
#31929=CARTESIAN_POINT('Ctrl Pts',(-18.1932968795114,67.1135303320171,30.8152402811701));
#31930=CARTESIAN_POINT('Ctrl Pts',(-18.0845661180528,65.0860858848918,30.7041071631786));
#31931=CARTESIAN_POINT('Ctrl Pts',(-19.7289158360952,63.8950916072225,30.592974045187));
#31932=CARTESIAN_POINT('Ctrl Pts',(-21.621372450712,64.6305923390101,30.4818409271955));
#31933=CARTESIAN_POINT('Ctrl Pts',(-22.0298851818394,66.6194288614961,30.3707078092039));
#31934=CARTESIAN_POINT('Ctrl Pts',(-20.5805670990452,68.0413397094584,30.2595746912124));
#31935=CARTESIAN_POINT('Ctrl Pts',(-18.5998911563065,67.5949361089764,30.1484415732208));
#31936=CARTESIAN_POINT('Ctrl Pts',(-17.9006499350632,65.6887842054856,30.0373084552293));
#31937=CARTESIAN_POINT('Ctrl Pts',(-19.1228165228634,64.0674692464688,29.9261753372376));
#31938=CARTESIAN_POINT('Ctrl Pts',(-21.1478159545443,64.2148824967529,29.8150422192461));
#31939=CARTESIAN_POINT('Ctrl Pts',(-22.1222890470305,65.996105547549,29.7039091012546));
#31940=CARTESIAN_POINT('Ctrl Pts',(-21.1543596711915,67.7808929545126,29.592775983263));
#31941=CARTESIAN_POINT('Ctrl Pts',(-19.1299148891241,67.9357370342423,29.4816428652714));
#31942=CARTESIAN_POINT('Ctrl Pts',(-17.9018062467466,66.3189183903665,29.3705097472799));
#31943=CARTESIAN_POINT('Ctrl Pts',(-18.594047111448,64.4102130831215,29.2593766292883));
#31944=CARTESIAN_POINT('Ctrl Pts',(-20.5730713975186,63.9565433356072,29.1482435112968));
#31945=CARTESIAN_POINT('Ctrl Pts',(-22.0275981847098,65.3731255570155,29.0371103933052));
#31946=CARTESIAN_POINT('Ctrl Pts',(-21.6263873077676,67.363447942181,28.9259772753137));
#31947=CARTESIAN_POINT('Ctrl Pts',(-19.7366427527761,68.1058891058742,28.8148441573221));
#31948=CARTESIAN_POINT('Ctrl Pts',(-18.0879331160836,66.920937672884,28.7037110393305));
#31949=CARTESIAN_POINT('Ctrl Pts',(-18.1892223497717,64.8931078339165,28.592577921339));
#31950=CARTESIAN_POINT('Ctrl Pts',(-19.9478065604602,63.8783492722001,28.4814448033474));
#31951=CARTESIAN_POINT('Ctrl Pts',(-21.754160261334,64.8054089639244,28.3703116853558));
#31952=CARTESIAN_POINT('Ctrl Pts',(-21.9550374479505,66.8258053905114,28.2591785673643));
#31953=CARTESIAN_POINT('Ctrl Pts',(-20.3665874126971,68.0903922203161,28.1480454493727));
#31954=CARTESIAN_POINT('Ctrl Pts',(-18.4426221485666,67.4417698130572,28.0369123313812));
#31955=CARTESIAN_POINT('Ctrl Pts',(-17.9440303919362,65.47358292537,27.9257792133896));
#31956=CARTESIAN_POINT('Ctrl Pts',(-19.3271429426348,63.9871936639811,27.8146460953981));
#31957=CARTESIAN_POINT('Ctrl Pts',(-21.3260807559213,64.3430039845566,27.7035129774064));
#31958=CARTESIAN_POINT('Ctrl Pts',(-22.1113372667774,66.2153622772843,27.592379859415));
#31959=CARTESIAN_POINT('Ctrl Pts',(-20.9642148108129,67.8906125370837,27.4812467414234));
#31960=CARTESIAN_POINT('Ctrl Pts',(-18.9346050065562,67.8354997895207,27.3701136234318));
#31961=CARTESIAN_POINT('Ctrl Pts',(-17.8800866384454,66.1004653893011,27.2589805054403));
#31962=CARTESIAN_POINT('Ctrl Pts',(-18.7657964086194,64.2734811119483,27.1478473874487));
#31963=CARTESIAN_POINT('Ctrl Pts',(-20.7810979017209,64.0266748732019,27.0367142694572));
#31964=CARTESIAN_POINT('Ctrl Pts',(-22.0815078149365,65.5859334655229,26.9255811514656));
#31965=CARTESIAN_POINT('Ctrl Pts',(-21.4768399213782,67.5241620363296,26.814448033474));
#31966=CARTESIAN_POINT('Ctrl Pts',(-19.5205098587676,68.0674175437184,26.7033149154824));
#31967=CARTESIAN_POINT('Ctrl Pts',(-18.0030283353595,66.7184910971486,26.5921817974909));
#31968=CARTESIAN_POINT('Ctrl Pts',(-18.3132533024857,64.7119734090229,26.4810486794993));
#31969=CARTESIAN_POINT('Ctrl Pts',(-20.1672563872311,63.8843081735796,26.3699155615078));
#31970=CARTESIAN_POINT('Ctrl Pts',(-21.8681775497427,64.9930077285944,26.2587824435162));
#31971=CARTESIAN_POINT('Ctrl Pts',(-21.8592736605897,67.0233455312749,26.1476493255247));
#31972=CARTESIAN_POINT('Ctrl Pts',(-20.1486802204003,68.1170786486788,26.0365162075331));
#31973=CARTESIAN_POINT('Ctrl Pts',(-18.3020269665029,67.2731752214615,25.9253830895416));
#31974=CARTESIAN_POINT('Ctrl Pts',(-18.0093892263405,65.2640173779833,25.8142499715499));
#31975=CARTESIAN_POINT('Ctrl Pts',(-19.5387090650051,63.9284485173924,25.7031168535584));
#31976=CARTESIAN_POINT('Ctrl Pts',(-21.4900764778608,64.4888676002409,25.5919837355669));
#31977=CARTESIAN_POINT('Ctrl Pts',(-22.0779544425627,66.4322896887595,25.4808506175753));
#31978=CARTESIAN_POINT('Ctrl Pts',(-20.7634340698636,67.9801526848469,25.3697174995838));
#31979=CARTESIAN_POINT('Ctrl Pts',(-18.7513312248939,67.7155231872575,25.2585843815922));
#31980=CARTESIAN_POINT('Ctrl Pts',(-17.8797718995485,65.8811422830375,25.1474512636006));
#31981=CARTESIAN_POINT('Ctrl Pts',(-18.9534066958213,64.1547469815952,25.0363181456091));
#31982=CARTESIAN_POINT('Ctrl Pts',(-20.3003147350832,64.1317394393838,24.9622294002814));
#31983=CARTESIAN_POINT('Ctrl Pts',(-20.8297858778675,64.4076511362656,24.9251850276175));
#31984=CARTESIAN_POINT('Ctrl Pts',(-20.4298642568858,64.3904122513351,36.2244449171475));
#31985=CARTESIAN_POINT('Ctrl Pts',(-20.9650674928767,64.5333462053945,36.1874005444836));
#31986=CARTESIAN_POINT('Ctrl Pts',(-21.8723681743508,65.3930105698463,36.1133117991559));
#31987=CARTESIAN_POINT('Ctrl Pts',(-21.5253863956627,67.2471151808573,36.0021786811643));
#31988=CARTESIAN_POINT('Ctrl Pts',(-19.7796095403819,67.9563340419976,35.8910455631728));
#31989=CARTESIAN_POINT('Ctrl Pts',(-18.236880545267,66.8767204788825,35.7799124451813));
#31990=CARTESIAN_POINT('Ctrl Pts',(-18.307158118857,64.9938596507859,35.6687793271897));
#31991=CARTESIAN_POINT('Ctrl Pts',(-19.927127040521,64.032278077288,35.5576462091981));
#31992=CARTESIAN_POINT('Ctrl Pts',(-21.6136237284516,64.8714224244312,35.4465130912065));
#31993=CARTESIAN_POINT('Ctrl Pts',(-21.8233529498679,66.7435910336453,35.3353799732151));
#31994=CARTESIAN_POINT('Ctrl Pts',(-20.3642354116722,67.9351428732915,35.2242468552234));
#31995=CARTESIAN_POINT('Ctrl Pts',(-18.5717765418526,67.3556023661456,35.1131137372319));
#31996=CARTESIAN_POINT('Ctrl Pts',(-18.0864733352012,65.5353478870809,35.0019806192403));
#31997=CARTESIAN_POINT('Ctrl Pts',(-19.3525103946316,64.1403679964566,34.8908475012488));
#31998=CARTESIAN_POINT('Ctrl Pts',(-21.2111527440429,64.447393156285,34.7797143832572));
#31999=CARTESIAN_POINT('Ctrl Pts',(-21.9613017767111,66.1754268915585,34.6685812652656));
#32000=CARTESIAN_POINT('Ctrl Pts',(-20.9163895525773,67.742902187265,34.5574481472741));
#32001=CARTESIAN_POINT('Ctrl Pts',(-19.0327618795789,67.7152052243898,34.4463150292825));
#32002=CARTESIAN_POINT('Ctrl Pts',(-18.0343884347818,66.1176847180857,34.3351819112909));
#32003=CARTESIAN_POINT('Ctrl Pts',(-18.8350201453212,64.4124546322215,34.2240487932994));
#32004=CARTESIAN_POINT('Ctrl Pts',(-20.7018872293234,64.1602084987291,34.1129156753078));
#32005=CARTESIAN_POINT('Ctrl Pts',(-21.9263595164535,65.5918119874694,34.0017825573163));
#32006=CARTESIAN_POINT('Ctrl Pts',(-21.3877517426115,67.3970051979684,33.8906494393247));
#32007=CARTESIAN_POINT('Ctrl Pts',(-19.5790189579431,67.9236042724355,33.7795163213332));
#32008=CARTESIAN_POINT('Ctrl Pts',(-18.1555845899151,66.6896450010639,33.6683832033416));
#32009=CARTESIAN_POINT('Ctrl Pts',(-18.4202318020353,64.8244954822508,33.5572500853501));
#32010=CARTESIAN_POINT('Ctrl Pts',(-20.1307450473233,64.0352139646386,33.4461169673585));
#32011=CARTESIAN_POINT('Ctrl Pts',(-21.7215952795671,65.0441819602404,33.3349838493669));
#32012=CARTESIAN_POINT('Ctrl Pts',(-21.7367737504501,66.9279522462476,33.2238507313754));
#32013=CARTESIAN_POINT('Ctrl Pts',(-20.1623885262583,67.9624241127519,33.1127176133838));
#32014=CARTESIAN_POINT('Ctrl Pts',(-18.4393789312417,67.2008081909514,33.0015844953923));
#32015=CARTESIAN_POINT('Ctrl Pts',(-18.144711163821,65.3401653494693,32.8904513774007));
#32016=CARTESIAN_POINT('Ctrl Pts',(-19.5480767627175,64.0834291509782,32.7793182594092));
#32017=CARTESIAN_POINT('Ctrl Pts',(-21.3650602959056,64.580814029012,32.6681851414176));
#32018=CARTESIAN_POINT('Ctrl Pts',(-21.9326869180286,66.3770937663063,32.557052023426));
#32019=CARTESIAN_POINT('Ctrl Pts',(-20.7314424029572,67.8282424464125,32.4459189054344));
#32020=CARTESIAN_POINT('Ctrl Pts',(-18.8607530114064,67.6061116806398,32.334785787443));
#32021=CARTESIAN_POINT('Ctrl Pts',(-18.0327473041412,65.9140042888062,32.2236526694513));
#32022=CARTESIAN_POINT('Ctrl Pts',(-19.0052486944375,64.3006035566151,32.1125195514598));
#32023=CARTESIAN_POINT('Ctrl Pts',(-20.8881856326145,64.2425573370022,32.0013864334682));
#32024=CARTESIAN_POINT('Ctrl Pts',(-21.9582201211768,65.7929918148341,31.8902533154766));
#32025=CARTESIAN_POINT('Ctrl Pts',(-21.2360144800452,67.5328883314924,31.7791201974851));
#32026=CARTESIAN_POINT('Ctrl Pts',(-19.3825597377204,67.8698251132723,31.6679870794935));
#32027=CARTESIAN_POINT('Ctrl Pts',(-18.0942106256457,66.4954243557859,31.556853961502));
#32028=CARTESIAN_POINT('Ctrl Pts',(-18.5501149601189,64.6675917281717,31.4457208435104));
#32029=CARTESIAN_POINT('Ctrl Pts',(-20.3330111500104,64.0592315940133,31.3345877255189));
#32030=CARTESIAN_POINT('Ctrl Pts',(-21.8111224282211,65.2271390929139,31.2234546075273));
#32031=CARTESIAN_POINT('Ctrl Pts',(-21.6316231750398,67.1023993134887,31.1123214895358));
#32032=CARTESIAN_POINT('Ctrl Pts',(-19.9587981719997,67.9687002923444,31.0011883715442));
#32033=CARTESIAN_POINT('Ctrl Pts',(-18.3236827036336,67.0331692763581,30.8900552535526));
#32034=CARTESIAN_POINT('Ctrl Pts',(-18.2227988041078,65.1520410735024,30.7789221355611));
#32035=CARTESIAN_POINT('Ctrl Pts',(-19.7484793890201,64.0469982555154,30.6677890175695));
#32036=CARTESIAN_POINT('Ctrl Pts',(-21.5043615368559,64.7294195034804,30.5566558995779));
#32037=CARTESIAN_POINT('Ctrl Pts',(-21.8833927950681,66.5747260314211,30.4455227815864));
#32038=CARTESIAN_POINT('Ctrl Pts',(-20.538668837616,67.8940206744091,30.3343896635948));
#32039=CARTESIAN_POINT('Ctrl Pts',(-18.7009339581788,67.4798330482506,30.2232565456033));
#32040=CARTESIAN_POINT('Ctrl Pts',(-18.0521554509576,65.711243970672,30.1121234276117));
#32041=CARTESIAN_POINT('Ctrl Pts',(-19.1861209414343,64.2069357764609,30.0009903096202));
#32042=CARTESIAN_POINT('Ctrl Pts',(-21.0649805802779,64.343710533953,29.8898571916286));
#32043=CARTESIAN_POINT('Ctrl Pts',(-21.969128074824,65.9963866016894,29.7787240736371));
#32044=CARTESIAN_POINT('Ctrl Pts',(-21.0710520511653,67.6523697937816,29.6675909556455));
#32045=CARTESIAN_POINT('Ctrl Pts',(-19.1927070340822,67.7960391139636,29.5564578376539));
#32046=CARTESIAN_POINT('Ctrl Pts',(-18.0532283141485,66.2959027456354,29.4453247196623));
#32047=CARTESIAN_POINT('Ctrl Pts',(-18.695511665293,64.524944537883,29.3341916016708));
#32048=CARTESIAN_POINT('Ctrl Pts',(-20.5317140845218,64.1040151466775,29.2230584836793));
#32049=CARTESIAN_POINT('Ctrl Pts',(-21.8812708455339,65.418365718469,29.1119253656877));
#32050=CARTESIAN_POINT('Ctrl Pts',(-21.5090144826143,67.2650508776204,29.0007922476962));
#32051=CARTESIAN_POINT('Ctrl Pts',(-19.7556486709751,67.9539116816557,28.8896591297046));
#32052=CARTESIAN_POINT('Ctrl Pts',(-18.2259228132335,66.8544756094258,28.778526011713));
#32053=CARTESIAN_POINT('Ctrl Pts',(-18.3199022238194,64.9729898276167,28.6673928937215));
#32054=CARTESIAN_POINT('Ctrl Pts',(-19.9515732471676,64.0314641782998,28.5562597757299));
#32055=CARTESIAN_POINT('Ctrl Pts',(-21.6275663407708,64.891619993817,28.4451266577383));
#32056=CARTESIAN_POINT('Ctrl Pts',(-21.813946658905,66.7662088164062,28.3339935397468));
#32057=CARTESIAN_POINT('Ctrl Pts',(-20.3401315985817,67.9395331725326,28.2228604217552));
#32058=CARTESIAN_POINT('Ctrl Pts',(-18.555014711753,67.3377204298807,28.1117273037637));
#32059=CARTESIAN_POINT('Ctrl Pts',(-18.0924052348628,65.5115732976283,28.0005941857721));
#32060=CARTESIAN_POINT('Ctrl Pts',(-19.3757015690887,64.1324535076954,27.8894610677806));
#32061=CARTESIAN_POINT('Ctrl Pts',(-21.230380399702,64.4625857733909,27.7783279497889));
#32062=CARTESIAN_POINT('Ctrl Pts',(-21.958966660668,66.1998200513978,27.6671948317975));
#32063=CARTESIAN_POINT('Ctrl Pts',(-20.8946295306897,67.7541711533567,27.5560617138058));
#32064=CARTESIAN_POINT('Ctrl Pts',(-19.0114922398047,67.7030357725946,27.4449285958143));
#32065=CARTESIAN_POINT('Ctrl Pts',(-18.033076162612,66.0932150212516,27.3337954778227));
#32066=CARTESIAN_POINT('Ctrl Pts',(-18.8548661902409,64.3980802148824,27.2226623598312));
#32067=CARTESIAN_POINT('Ctrl Pts',(-20.7247277695829,64.1690854441478,27.1115292418396));
#32068=CARTESIAN_POINT('Ctrl Pts',(-21.931289935314,65.6158157443139,27.0003961238481));
#32069=CARTESIAN_POINT('Ctrl Pts',(-21.3702596049656,67.4141665860817,26.8892630058565));
#32070=CARTESIAN_POINT('Ctrl Pts',(-19.5551136165815,67.9182165282414,26.7781298878649));
#32071=CARTESIAN_POINT('Ctrl Pts',(-18.1471454253728,66.6666391615628,26.6669967698734));
#32072=CARTESIAN_POINT('Ctrl Pts',(-18.4349821331645,64.8049274791473,26.5558636518818));
#32073=CARTESIAN_POINT('Ctrl Pts',(-20.1551858585197,64.036993038762,26.4447305338903));
#32074=CARTESIAN_POINT('Ctrl Pts',(-21.7333552501256,65.0656801647588,26.3335974158987));
#32075=CARTESIAN_POINT('Ctrl Pts',(-21.725093935235,66.9494929160091,26.2224642979072));
#32076=CARTESIAN_POINT('Ctrl Pts',(-20.137950293138,67.9642936995585,26.1113311799155));
#32077=CARTESIAN_POINT('Ctrl Pts',(-18.424565977367,67.181292942287,26.0001980619241));
#32078=CARTESIAN_POINT('Ctrl Pts',(-18.1530472647236,65.317131638773,25.8890649439324));
#32079=CARTESIAN_POINT('Ctrl Pts',(-19.5719994257939,64.0779478702237,25.7779318259409));
#32080=CARTESIAN_POINT('Ctrl Pts',(-21.3825409080333,64.5979227300327,25.6667987079493));
#32081=CARTESIAN_POINT('Ctrl Pts',(-21.9279930020751,66.4010922846652,25.5556655899578));
#32082=CARTESIAN_POINT('Ctrl Pts',(-20.7083386979493,67.8372493839263,25.4445324719662));
#32083=CARTESIAN_POINT('Ctrl Pts',(-18.841444927279,67.5917176200702,25.3333993539747));
#32084=CARTESIAN_POINT('Ctrl Pts',(-18.0327841377349,65.8897199852641,25.2222662359831));
#32085=CARTESIAN_POINT('Ctrl Pts',(-19.0289370521585,64.2879148677798,25.1111331179916));
#32086=CARTESIAN_POINT('Ctrl Pts',(-20.2786416755829,64.2665677297147,25.0370443726639));
#32087=CARTESIAN_POINT('Ctrl Pts',(-20.7699020406705,64.5225674811446,25.));
#32088=CARTESIAN_POINT('Ctrl Pts',(-21.6638441182547,66.0009441583361,35.3785196366098));
#32089=CARTESIAN_POINT('Ctrl Pts',(-21.6649630220915,66.2166368308252,35.3641397488116));
#32090=CARTESIAN_POINT('Ctrl Pts',(-21.6260431008204,66.4319423603926,35.3497598610133));
#32091=CARTESIAN_POINT('Ctrl Pts',(-21.5452118232659,66.630154905384,35.335379973215));
#32092=CARTESIAN_POINT('Ctrl Pts',(-21.336980437136,67.1407749801941,35.2983356005512));
#32093=CARTESIAN_POINT('Ctrl Pts',(-20.8506079244041,67.5379589267428,35.2612912278873));
#32094=CARTESIAN_POINT('Ctrl Pts',(-20.3086785230682,67.6399608154928,35.2242468552234));
#32095=CARTESIAN_POINT('Ctrl Pts',(-19.7667491217323,67.7419627042429,35.1872024825596));
#32096=CARTESIAN_POINT('Ctrl Pts',(-19.1692628317925,67.5487825351942,35.1501581098958));
#32097=CARTESIAN_POINT('Ctrl Pts',(-18.7896358190473,67.1488167041591,35.1131137372319));
#32098=CARTESIAN_POINT('Ctrl Pts',(-18.4100088063022,66.748850873124,35.0760693645681));
#32099=CARTESIAN_POINT('Ctrl Pts',(-18.2482410707517,66.1420993801025,35.0390249919042));
#32100=CARTESIAN_POINT('Ctrl Pts',(-18.3783633795482,65.6062269851543,35.0019806192403));
#32101=CARTESIAN_POINT('Ctrl Pts',(-18.5084856883447,65.0703545902061,34.9649362465764));
#32102=CARTESIAN_POINT('Ctrl Pts',(-18.9304980414881,64.6053612933314,34.9278918739126));
#32103=CARTESIAN_POINT('Ctrl Pts',(-19.4512779429618,64.4240355048654,34.8908475012488));
#32104=CARTESIAN_POINT('Ctrl Pts',(-19.9720578444354,64.2427097163994,34.8538031285849));
#32105=CARTESIAN_POINT('Ctrl Pts',(-20.5916052942391,64.3450514363422,34.8167587559211));
#32106=CARTESIAN_POINT('Ctrl Pts',(-21.0264038579191,64.6842279188592,34.7797143832572));
#32107=CARTESIAN_POINT('Ctrl Pts',(-21.4223194165699,64.9930726524306,34.7459828010414));
#32108=CARTESIAN_POINT('Ctrl Pts',(-21.6650519066689,65.4982870444721,34.7122512188256));
#32109=CARTESIAN_POINT('Ctrl Pts',(-21.6682089013646,66.0008588710179,34.6785196366098));
#32110=CARTESIAN_POINT('Ctrl Pts',(-20.5301702171886,64.0148256743283,36.));
#32111=CARTESIAN_POINT('Ctrl Pts',(-20.5988349732706,64.0402496877953,36.));
#32112=CARTESIAN_POINT('Ctrl Pts',(-20.6657963847736,64.069563384374,36.));
#32113=CARTESIAN_POINT('Ctrl Pts',(-20.730865515262,64.1024727373112,36.));
#32114=CARTESIAN_POINT('Ctrl Pts',(-20.7977456115802,64.1362980040343,36.));
#32115=CARTESIAN_POINT('Ctrl Pts',(-20.8626274029816,64.1739225452161,36.));
#32116=CARTESIAN_POINT('Ctrl Pts',(-20.9252745196845,64.2150717403274,36.));
#32117=CARTESIAN_POINT('Ctrl Pts',(-20.9782072426395,64.2498401232839,36.));
#32118=CARTESIAN_POINT('Ctrl Pts',(-21.0295442643604,64.2871258592549,36.));
#32119=CARTESIAN_POINT('Ctrl Pts',(-21.0791202642708,64.3267813067489,36.));
#32120=CARTESIAN_POINT('Ctrl Pts',(-21.101149928935,64.3444026600646,36.));
#32121=CARTESIAN_POINT('Ctrl Pts',(-21.1228315640659,64.3624921087365,36.));
#32122=CARTESIAN_POINT('Ctrl Pts',(-21.1441491105767,64.3810374223025,36.));
#32123=CARTESIAN_POINT('Ctrl Pts',(-21.1558616839704,64.3912268381502,36.));
#32124=CARTESIAN_POINT('Ctrl Pts',(-21.1674643296591,64.4015538757899,36.));
#32125=CARTESIAN_POINT('Ctrl Pts',(-21.1789542498192,64.4120165483206,36.));
#32126=CARTESIAN_POINT('Ctrl Pts',(-21.1895478048553,64.421662994574,36.));
#32127=CARTESIAN_POINT('Ctrl Pts',(-21.2000469702932,64.4314262540256,36.));
#32128=CARTESIAN_POINT('Ctrl Pts',(-21.2104336655795,64.4412893138512,36.));
#32129=CARTESIAN_POINT('Ctrl Pts',(-21.2635184366823,64.4916978662139,36.));
#32130=CARTESIAN_POINT('Ctrl Pts',(-21.3137632137796,64.5447948198095,36.));
#32131=CARTESIAN_POINT('Ctrl Pts',(-21.3609493297492,64.6003207092003,36.));
#32132=CARTESIAN_POINT('Ctrl Pts',(-21.4077692882983,64.6554157257375,36.));
#32133=CARTESIAN_POINT('Ctrl Pts',(-21.4515783794455,64.7129030113309,36.));
#32134=CARTESIAN_POINT('Ctrl Pts',(-21.4921181954482,64.772553333862,36.));
#32135=CARTESIAN_POINT('Ctrl Pts',(-21.525806627261,64.8221225233982,36.));
#32136=CARTESIAN_POINT('Ctrl Pts',(-21.5572368021225,64.8731860598217,36.));
#32137=CARTESIAN_POINT('Ctrl Pts',(-21.5862328303999,64.9256188737153,36.));
#32138=CARTESIAN_POINT('Ctrl Pts',(-21.5983389970515,64.9475101609266,36.));
#32139=CARTESIAN_POINT('Ctrl Pts',(-21.6100205322312,64.9696401736576,36.));
#32140=CARTESIAN_POINT('Ctrl Pts',(-21.6212631934191,64.9919998924642,36.));
#32141=CARTESIAN_POINT('Ctrl Pts',(-21.6264640159837,65.0023434337455,36.));
#32142=CARTESIAN_POINT('Ctrl Pts',(-21.6315709088334,65.0127361311819,36.));
#32143=CARTESIAN_POINT('Ctrl Pts',(-21.6365823968231,65.0231770899229,36.));
#32144=CARTESIAN_POINT('Ctrl Pts',(-21.6418143886053,65.0340774473501,36.));
#32145=CARTESIAN_POINT('Ctrl Pts',(-21.6469387858192,65.0450229538182,36.));
#32146=CARTESIAN_POINT('Ctrl Pts',(-21.6519525299279,65.0560083018318,36.));
#32147=CARTESIAN_POINT('Ctrl Pts',(-21.6804929294147,65.1185416529592,36.));
#32148=CARTESIAN_POINT('Ctrl Pts',(-21.7054723575398,65.1824080698791,36.));
#32149=CARTESIAN_POINT('Ctrl Pts',(-21.7266673544266,65.2474030994014,36.));
#32150=CARTESIAN_POINT('Ctrl Pts',(-21.7458698278921,65.3062880021194,36.));
#32151=CARTESIAN_POINT('Ctrl Pts',(-21.7619656445149,65.3660998899564,36.));
#32152=CARTESIAN_POINT('Ctrl Pts',(-21.7747519290966,65.4266915444502,36.));
#32153=CARTESIAN_POINT('Ctrl Pts',(-21.7898844361711,65.498401479766,36.));
#32154=CARTESIAN_POINT('Ctrl Pts',(-21.800382014036,65.5712051224472,36.));
#32155=CARTESIAN_POINT('Ctrl Pts',(-21.8063198015774,65.6446793714796,36.));
#32156=CARTESIAN_POINT('Ctrl Pts',(-21.8076266251147,65.6608500204544,36.));
#32157=CARTESIAN_POINT('Ctrl Pts',(-21.8087123585312,65.6770530703594,36.));
#32158=CARTESIAN_POINT('Ctrl Pts',(-21.8095774335713,65.6932838463402,36.));
#32159=CARTESIAN_POINT('Ctrl Pts',(-21.8104727633698,65.7100822704259,36.));
#32160=CARTESIAN_POINT('Ctrl Pts',(-21.8111317404483,65.726916588365,36.));
#32161=CARTESIAN_POINT('Ctrl Pts',(-21.8115542824738,65.7437473430029,36.));
#32162=CARTESIAN_POINT('Ctrl Pts',(-21.8132755281181,65.8123082466785,36.));
#32163=CARTESIAN_POINT('Ctrl Pts',(-21.8110851681684,65.880896724124,36.));
#32164=CARTESIAN_POINT('Ctrl Pts',(-21.805103786848,65.9491744499936,36.));
#32165=CARTESIAN_POINT('Ctrl Pts',(-21.7991236414508,66.0174380677464,36.));
#32166=CARTESIAN_POINT('Ctrl Pts',(-21.7893535875248,66.0853921339257,36.));
#32167=CARTESIAN_POINT('Ctrl Pts',(-21.7758645295054,66.1526834998075,36.));
#32168=CARTESIAN_POINT('Ctrl Pts',(-21.7661045372626,66.2013720893343,36.));
#32169=CARTESIAN_POINT('Ctrl Pts',(-21.754396511133,66.2497134745457,36.));
#32170=CARTESIAN_POINT('Ctrl Pts',(-21.7407531062633,66.2975642349732,36.));
#32171=CARTESIAN_POINT('Ctrl Pts',(-21.7305167536077,66.3334656293283,36.));
#32172=CARTESIAN_POINT('Ctrl Pts',(-21.7191906927092,66.3690906873999,36.));
#32173=CARTESIAN_POINT('Ctrl Pts',(-21.7067763533949,66.4043746598269,36.));
#32174=CARTESIAN_POINT('Ctrl Pts',(-21.7026468248699,66.4161115849203,36.));
#32175=CARTESIAN_POINT('Ctrl Pts',(-21.6984000721287,66.4278015750603,36.));
#32176=CARTESIAN_POINT('Ctrl Pts',(-21.6940367401084,66.4394420694249,36.));
#32177=CARTESIAN_POINT('Ctrl Pts',(-21.6709127910537,66.5011321258786,36.));
#32178=CARTESIAN_POINT('Ctrl Pts',(-21.6445162548684,66.5614386479359,36.));
#32179=CARTESIAN_POINT('Ctrl Pts',(-21.6148971262233,66.6200275442078,36.));
#32180=CARTESIAN_POINT('Ctrl Pts',(-21.5940647936945,66.6612354873671,36.));
#32181=CARTESIAN_POINT('Ctrl Pts',(-21.5716374289325,66.701593212762,36.));
#32182=CARTESIAN_POINT('Ctrl Pts',(-21.5476220256553,66.7409731314567,36.));
#32183=CARTESIAN_POINT('Ctrl Pts',(-21.5399090083264,66.7536207639698,36.));
#32184=CARTESIAN_POINT('Ctrl Pts',(-21.5320310277768,66.7661691422738,36.));
#32185=CARTESIAN_POINT('Ctrl Pts',(-21.5239916401704,66.7786084047584,36.));
#32186=CARTESIAN_POINT('Ctrl Pts',(-21.4897471261491,66.8315945921934,36.));
#32187=CARTESIAN_POINT('Ctrl Pts',(-21.4526468486123,66.8824969904464,36.));
#32188=CARTESIAN_POINT('Ctrl Pts',(-21.4127250449828,66.9310003772166,36.));
#32189=CARTESIAN_POINT('Ctrl Pts',(-21.375938254522,66.9756948489973,36.));
#32190=CARTESIAN_POINT('Ctrl Pts',(-21.3367550941085,67.018352392206,36.));
#32191=CARTESIAN_POINT('Ctrl Pts',(-21.2951809127703,67.0586934718916,36.));
#32192=CARTESIAN_POINT('Ctrl Pts',(-21.287362563767,67.0662799265132,36.));
#32193=CARTESIAN_POINT('Ctrl Pts',(-21.2794596015101,67.0737843544158,36.));
#32194=CARTESIAN_POINT('Ctrl Pts',(-21.2714736181291,67.081206089647,36.));
#32195=CARTESIAN_POINT('Origin',(-20.,66.,30.));
#32196=CARTESIAN_POINT('Origin',(20.,-66.,25.));
#32197=CARTESIAN_POINT('Ctrl Pts',(19.2300979593296,-67.4774325188554,25.));
#32198=CARTESIAN_POINT('Ctrl Pts',(19.2818392509066,-67.5125051802703,25.));
#32199=CARTESIAN_POINT('Ctrl Pts',(19.3355570235436,-67.5443227583893,25.));
#32200=CARTESIAN_POINT('Ctrl Pts',(19.3909199784615,-67.5729492931195,25.));
#32201=CARTESIAN_POINT('Ctrl Pts',(19.4260302284271,-67.5911037574452,25.));
#32202=CARTESIAN_POINT('Ctrl Pts',(19.4618030444597,-67.6079741743555,25.));
#32203=CARTESIAN_POINT('Ctrl Pts',(19.4981615280073,-67.6235696646503,25.));
#32204=CARTESIAN_POINT('Ctrl Pts',(19.5229478187718,-67.6342014160147,25.));
#32205=CARTESIAN_POINT('Ctrl Pts',(19.5480064116943,-67.6442405386499,25.));
#32206=CARTESIAN_POINT('Ctrl Pts',(19.5733141854998,-67.6536883376551,25.));
#32207=CARTESIAN_POINT('Ctrl Pts',(19.5868028134417,-67.6587238594133,25.));
#32208=CARTESIAN_POINT('Ctrl Pts',(19.600362177991,-67.6635912278487,25.));
#32209=CARTESIAN_POINT('Ctrl Pts',(19.6139750771008,-67.6682861195686,25.));
#32210=CARTESIAN_POINT('Ctrl Pts',(19.6763395178067,-67.6897947118182,25.));
#32211=CARTESIAN_POINT('Ctrl Pts',(19.7398952542217,-67.7077136324119,25.));
#32212=CARTESIAN_POINT('Ctrl Pts',(19.8042923951479,-67.7220894217911,25.));
#32213=CARTESIAN_POINT('Ctrl Pts',(19.8507447452963,-67.7324592797118,25.));
#32214=CARTESIAN_POINT('Ctrl Pts',(19.8976358065701,-67.7409846995403,25.));
#32215=CARTESIAN_POINT('Ctrl Pts',(19.9448433633825,-67.7476691194456,25.));
#32216=CARTESIAN_POINT('Ctrl Pts',(19.9577433322521,-67.7494957085452,25.));
#32217=CARTESIAN_POINT('Ctrl Pts',(19.9706669674625,-67.7511847572499,25.));
#32218=CARTESIAN_POINT('Ctrl Pts',(19.9836118418914,-67.7527361749649,25.));
#32219=CARTESIAN_POINT('Ctrl Pts',(19.9969414186446,-67.754333698496,25.));
#32220=CARTESIAN_POINT('Ctrl Pts',(20.0102855922404,-67.755784299122,25.));
#32221=CARTESIAN_POINT('Ctrl Pts',(20.0236361127826,-67.7570879007368,25.));
#32222=CARTESIAN_POINT('Ctrl Pts',(20.0911672976909,-67.7636819328885,25.));
#32223=CARTESIAN_POINT('Ctrl Pts',(20.1589021638891,-67.7665235696462,25.));
#32224=CARTESIAN_POINT('Ctrl Pts',(20.2264860370306,-67.7656607588407,25.));
#32225=CARTESIAN_POINT('Ctrl Pts',(20.2950484463622,-67.7647854555343,25.));
#32226=CARTESIAN_POINT('Ctrl Pts',(20.3634564684948,-67.7600979895892,25.));
#32227=CARTESIAN_POINT('Ctrl Pts',(20.4313612906511,-67.7516001272965,25.));
#32228=CARTESIAN_POINT('Ctrl Pts',(20.4734291139411,-67.7463356032476,25.));
#32229=CARTESIAN_POINT('Ctrl Pts',(20.5153041791594,-67.739607699183,25.));
#32230=CARTESIAN_POINT('Ctrl Pts',(20.5569049276303,-67.731406890815,25.));
#32231=CARTESIAN_POINT('Ctrl Pts',(20.5909685558849,-67.7246918845254,25.));
#32232=CARTESIAN_POINT('Ctrl Pts',(20.6248483029251,-67.7169892041243,25.));
#32233=CARTESIAN_POINT('Ctrl Pts',(20.6584990498341,-67.7082896385505,25.));
#32234=CARTESIAN_POINT('Ctrl Pts',(20.6722821167333,-67.704726368629,25.));
#32235=CARTESIAN_POINT('Ctrl Pts',(20.6860292290737,-67.7009949721105,25.));
#32236=CARTESIAN_POINT('Ctrl Pts',(20.6997140296679,-67.6971016570004,25.));
#32237=CARTESIAN_POINT('Ctrl Pts',(20.7675093077033,-67.6778139532044,25.));
#32238=CARTESIAN_POINT('Ctrl Pts',(20.8338949911143,-67.6545270467904,25.));
#32239=CARTESIAN_POINT('Ctrl Pts',(20.898508351168,-67.6272596461893,25.));
#32240=CARTESIAN_POINT('Ctrl Pts',(20.9056750502645,-67.6242352367624,25.));
#32241=CARTESIAN_POINT('Ctrl Pts',(20.9128199532954,-67.6211618050839,25.));
#32242=CARTESIAN_POINT('Ctrl Pts',(20.9199425694434,-67.6180393373165,25.));
#32243=CARTESIAN_POINT('Ctrl Pts',(20.9816951205624,-67.5909677745065,25.));
#32244=CARTESIAN_POINT('Ctrl Pts',(21.0417732412363,-67.5602146096881,25.));
#32245=CARTESIAN_POINT('Ctrl Pts',(21.1000349944499,-67.5260900451755,25.));
#32246=CARTESIAN_POINT('Ctrl Pts',(21.162710887036,-67.4893800695575,25.));
#32247=CARTESIAN_POINT('Ctrl Pts',(21.2232857612189,-67.4487684714382,25.));
#32248=CARTESIAN_POINT('Ctrl Pts',(21.281563029017,-67.4045803567109,25.));
#32249=CARTESIAN_POINT('Ctrl Pts',(21.2920881592725,-67.3965997893161,25.));
#32250=CARTESIAN_POINT('Ctrl Pts',(21.3025382728815,-67.3885024149022,25.));
#32251=CARTESIAN_POINT('Ctrl Pts',(21.3129121067363,-67.3802899597523,25.));
#32252=CARTESIAN_POINT('Ctrl Pts',(21.3220882756753,-67.3730256371388,25.));
#32253=CARTESIAN_POINT('Ctrl Pts',(21.3311977619232,-67.3656767917098,25.));
#32254=CARTESIAN_POINT('Ctrl Pts',(21.340237913509,-67.3582467210556,25.));
#32255=CARTESIAN_POINT('Ctrl Pts',(21.3951411261676,-67.31312195237,25.));
#32256=CARTESIAN_POINT('Ctrl Pts',(21.4475122197521,-67.2649864357061,25.));
#32257=CARTESIAN_POINT('Ctrl Pts',(21.4972011756428,-67.2141901758274,25.));
#32258=CARTESIAN_POINT('Ctrl Pts',(21.5479379013916,-67.1623227968428,25.));
#32259=CARTESIAN_POINT('Ctrl Pts',(21.5958789474072,-67.1076807385324,25.));
#32260=CARTESIAN_POINT('Ctrl Pts',(21.6408443956269,-67.0505853273705,25.));
#32261=CARTESIAN_POINT('Ctrl Pts',(21.6860826148688,-66.9931435619682,25.));
#32262=CARTESIAN_POINT('Ctrl Pts',(21.7283098131003,-66.9332178592765,25.));
#32263=CARTESIAN_POINT('Ctrl Pts',(21.7673108256436,-66.8710938870854,25.));
#32264=CARTESIAN_POINT('Ctrl Pts',(21.7769378410941,-66.855759197006,25.));
#32265=CARTESIAN_POINT('Ctrl Pts',(21.7863681009519,-66.8402903992017,25.));
#32266=CARTESIAN_POINT('Ctrl Pts',(21.7955979845278,-66.8246914847445,25.));
#32267=CARTESIAN_POINT('Ctrl Pts',(21.8028476850435,-66.8124391678809,25.));
#32268=CARTESIAN_POINT('Ctrl Pts',(21.8099745027199,-66.8001050249419,25.));
#32269=CARTESIAN_POINT('Ctrl Pts',(21.8169662172758,-66.7877100692794,25.));
#32270=CARTESIAN_POINT('Ctrl Pts',(21.8539814596018,-66.722089214223,25.));
#32271=CARTESIAN_POINT('Ctrl Pts',(21.8872826215013,-66.6546514104225,25.));
#32272=CARTESIAN_POINT('Ctrl Pts',(21.9166889688907,-66.5857429831168,25.));
#32273=CARTESIAN_POINT('Ctrl Pts',(21.9461273939939,-66.5167593875222,25.));
#32274=CARTESIAN_POINT('Ctrl Pts',(21.9716632676734,-66.4463011289855,25.));
#32275=CARTESIAN_POINT('Ctrl Pts',(21.9930795264615,-66.3746779559458,25.));
#32276=CARTESIAN_POINT('Ctrl Pts',(22.0140085505991,-66.3046842594656,25.));
#32277=CARTESIAN_POINT('Ctrl Pts',(22.0310038329003,-66.2335771734604,25.));
#32278=CARTESIAN_POINT('Ctrl Pts',(22.0438191861901,-66.1616225716972,25.));
#32279=CARTESIAN_POINT('Ctrl Pts',(22.0465680471256,-66.1461884912282,25.));
#32280=CARTESIAN_POINT('Ctrl Pts',(22.0491244126747,-66.1307153578235,25.));
#32281=CARTESIAN_POINT('Ctrl Pts',(22.0514855454828,-66.1152057111006,25.));
#32282=CARTESIAN_POINT('Ctrl Pts',(22.0534987389493,-66.1019815843837,25.));
#32283=CARTESIAN_POINT('Ctrl Pts',(22.0553699972796,-66.0887309121952,25.));
#32284=CARTESIAN_POINT('Ctrl Pts',(22.0571001480269,-66.0754553928761,25.));
#32285=CARTESIAN_POINT('Ctrl Pts',(21.8174278887595,-65.0413794120408,25.));
#32286=CARTESIAN_POINT('Ctrl Pts',(21.776581404545,-64.9788996392346,25.));
#32287=CARTESIAN_POINT('Ctrl Pts',(21.7321382352854,-64.9189705873501,25.));
#32288=CARTESIAN_POINT('Ctrl Pts',(21.6844272287858,-64.8617420298968,25.));
#32289=CARTESIAN_POINT('Ctrl Pts',(21.6379676706942,-64.8060145639606,25.));
#32290=CARTESIAN_POINT('Ctrl Pts',(21.5884084602278,-64.7528475767717,25.));
#32291=CARTESIAN_POINT('Ctrl Pts',(21.5360271780281,-64.7024170328902,25.));
#32292=CARTESIAN_POINT('Ctrl Pts',(21.5243355070385,-64.6911607729796,25.));
#32293=CARTESIAN_POINT('Ctrl Pts',(21.5125015752233,-64.6800395435489,25.));
#32294=CARTESIAN_POINT('Ctrl Pts',(21.500533454458,-64.6690602418449,25.));
#32295=CARTESIAN_POINT('Ctrl Pts',(21.4456122822129,-64.6186767161566,25.));
#32296=CARTESIAN_POINT('Ctrl Pts',(21.3879773812488,-64.5713776698141,25.));
#32297=CARTESIAN_POINT('Ctrl Pts',(21.3279448973862,-64.5273355904878,25.));
#32298=CARTESIAN_POINT('Ctrl Pts',(21.285800416715,-64.4964168204909,25.));
#32299=CARTESIAN_POINT('Ctrl Pts',(21.2424736210485,-64.4671041191484,25.));
#32300=CARTESIAN_POINT('Ctrl Pts',(21.1980685681425,-64.439471567851,25.));
#32301=CARTESIAN_POINT('Ctrl Pts',(21.1811931522648,-64.4289702675622,25.));
#32302=CARTESIAN_POINT('Ctrl Pts',(21.1641619799486,-64.4187117531234,25.));
#32303=CARTESIAN_POINT('Ctrl Pts',(21.1469806872212,-64.4087005778126,25.));
#32304=CARTESIAN_POINT('Ctrl Pts',(21.1305959674615,-64.3991535486957,25.));
#32305=CARTESIAN_POINT('Ctrl Pts',(21.1140694086939,-64.3898287196359,25.));
#32306=CARTESIAN_POINT('Ctrl Pts',(21.0974354907253,-64.380745947404,25.));
#32307=CARTESIAN_POINT('Ctrl Pts',(21.0337185410866,-64.3459539914757,25.));
#32308=CARTESIAN_POINT('Ctrl Pts',(20.9683626351681,-64.3146691870302,25.));
#32309=CARTESIAN_POINT('Ctrl Pts',(20.9016594733476,-64.2870531698814,25.));
#32310=CARTESIAN_POINT('Ctrl Pts',(20.8363886507365,-64.2600301606663,25.));
#32311=CARTESIAN_POINT('Ctrl Pts',(20.7698268866709,-64.2365199143679,25.));
#32312=CARTESIAN_POINT('Ctrl Pts',(20.7022388874947,-64.216722135039,25.));
#32313=CARTESIAN_POINT('Ctrl Pts',(20.6361332105615,-64.1973585554056,25.));
#32314=CARTESIAN_POINT('Ctrl Pts',(20.5690450572908,-64.1815462756357,25.));
#32315=CARTESIAN_POINT('Ctrl Pts',(20.5012260301962,-64.1695207315524,25.));
#32316=CARTESIAN_POINT('Ctrl Pts',(20.4791658489428,-64.1656090611331,25.));
#32317=CARTESIAN_POINT('Ctrl Pts',(20.4570284148415,-64.1620984514521,25.));
#32318=CARTESIAN_POINT('Ctrl Pts',(20.4348226814172,-64.158998178911,25.));
#32319=CARTESIAN_POINT('Ctrl Pts',(20.4223381809779,-64.1572551446612,25.));
#32320=CARTESIAN_POINT('Ctrl Pts',(20.4098308067038,-64.155641770794,25.));
#32321=CARTESIAN_POINT('Ctrl Pts',(20.3973198538599,-64.1541615852412,25.));
#32322=CARTESIAN_POINT('Ctrl Pts',(20.3294892107318,-64.1461364620353,25.));
#32323=CARTESIAN_POINT('Ctrl Pts',(20.2614350334953,-64.1420045587359,25.));
#32324=CARTESIAN_POINT('Ctrl Pts',(20.1934030453685,-64.1419439160697,25.));
#32325=CARTESIAN_POINT('Ctrl Pts',(20.1836061137927,-64.1419351832358,25.));
#32326=CARTESIAN_POINT('Ctrl Pts',(20.1738096485656,-64.1420109658147,25.));
#32327=CARTESIAN_POINT('Ctrl Pts',(20.1640143929054,-64.1421718854656,25.));
#32328=CARTESIAN_POINT('Ctrl Pts',(20.094650154852,-64.1433114237648,25.));
#32329=CARTESIAN_POINT('Ctrl Pts',(20.0253451150382,-64.1487162439491,25.));
#32330=CARTESIAN_POINT('Ctrl Pts',(19.9564242806281,-64.1582131178836,25.));
#32331=CARTESIAN_POINT('Ctrl Pts',(19.8921290095081,-64.1670726171864,25.));
#32332=CARTESIAN_POINT('Ctrl Pts',(19.8281675897192,-64.1794942557964,25.));
#32333=CARTESIAN_POINT('Ctrl Pts',(19.7648243951104,-64.1953718384076,25.));
#32334=CARTESIAN_POINT('Ctrl Pts',(19.7509597565193,-64.1988471437813,25.));
#32335=CARTESIAN_POINT('Ctrl Pts',(19.7371248349099,-64.2024881308436,25.));
#32336=CARTESIAN_POINT('Ctrl Pts',(19.7233227901375,-64.2062938641054,25.));
#32337=CARTESIAN_POINT('Ctrl Pts',(19.7122623666812,-64.2093436311602,25.));
#32338=CARTESIAN_POINT('Ctrl Pts',(19.7012236018487,-64.2124991342566,25.));
#32339=CARTESIAN_POINT('Ctrl Pts',(19.6902211768855,-64.215755766339,25.));
#32340=CARTESIAN_POINT('Ctrl Pts',(19.6246589511318,-64.2351616744452,25.));
#32341=CARTESIAN_POINT('Ctrl Pts',(19.5602630981036,-64.2581875826496,25.));
#32342=CARTESIAN_POINT('Ctrl Pts',(19.4973360772709,-64.2846514713848,25.));
#32343=CARTESIAN_POINT('Ctrl Pts',(19.4347004138036,-64.3109928301035,25.));
#32344=CARTESIAN_POINT('Ctrl Pts',(19.3735191200478,-64.3407411090656,25.));
#32345=CARTESIAN_POINT('Ctrl Pts',(19.31412026665,-64.3737583558761,25.));
#32346=CARTESIAN_POINT('Ctrl Pts',(19.2559941313215,-64.4060681539024,25.));
#32347=CARTESIAN_POINT('Ctrl Pts',(19.1995741988762,-64.4415090370213,25.));
#32348=CARTESIAN_POINT('Ctrl Pts',(19.1452078375279,-64.4799811312036,25.));
#32349=CARTESIAN_POINT('Ctrl Pts',(19.1337113467811,-64.4881165675986,25.));
#32350=CARTESIAN_POINT('Ctrl Pts',(19.1223068502292,-64.4963876354851,25.));
#32351=CARTESIAN_POINT('Ctrl Pts',(19.1109979108722,-64.5047935191582,25.));
#32352=CARTESIAN_POINT('Ctrl Pts',(19.1003667878726,-64.5126955849869,25.));
#32353=CARTESIAN_POINT('Ctrl Pts',(19.0898188788728,-64.5207179018802,25.));
#32354=CARTESIAN_POINT('Ctrl Pts',(19.0793737230102,-64.5288465311509,25.));
#32355=CARTESIAN_POINT('Ctrl Pts',(19.0278062973887,-64.5689773334901,25.));
#32356=CARTESIAN_POINT('Ctrl Pts',(18.9786454464034,-64.6117656226463,25.));
#32357=CARTESIAN_POINT('Ctrl Pts',(18.9321822501578,-64.6570793867845,25.));
#32358=CARTESIAN_POINT('Ctrl Pts',(18.8866027003471,-64.7015313646193,25.));
#32359=CARTESIAN_POINT('Ctrl Pts',(18.8436185894728,-64.7484143331547,25.));
#32360=CARTESIAN_POINT('Ctrl Pts',(18.803547221108,-64.7976294314002,25.));
#32361=CARTESIAN_POINT('Ctrl Pts',(18.7647769773783,-64.8452465064347,25.));
#32362=CARTESIAN_POINT('Ctrl Pts',(18.7287330514718,-64.8950472934368,25.));
#32363=CARTESIAN_POINT('Ctrl Pts',(18.6957494965908,-64.9469576149125,25.));
#32364=CARTESIAN_POINT('Ctrl Pts',(18.6902971623536,-64.9555386312423,25.));
#32365=CARTESIAN_POINT('Ctrl Pts',(18.6849285675962,-64.9641773162184,25.));
#32366=CARTESIAN_POINT('Ctrl Pts',(18.6796453590658,-64.9728733607135,25.));
#32367=CARTESIAN_POINT('Ctrl Pts',(18.6739897755669,-64.9821823261781,25.));
#32368=CARTESIAN_POINT('Ctrl Pts',(18.6684320396214,-64.9915570228288,25.));
#32369=CARTESIAN_POINT('Ctrl Pts',(18.6629725546622,-65.0009957901906,25.));
#32370=CARTESIAN_POINT('Origin',(20.,-66.,37.5459252805377));
#32371=CARTESIAN_POINT('Ctrl Pts',(17.9434279331127,-65.9985037039655,35.7959252805377));
#32372=CARTESIAN_POINT('Ctrl Pts',(17.9426109898666,-65.9003307306121,35.7905876687522));
#32373=CARTESIAN_POINT('Ctrl Pts',(17.9936360911193,-65.1216409581897,35.7482056843029));
#32374=CARTESIAN_POINT('Ctrl Pts',(18.9885907005499,-63.7918186870749,35.6687793271897));
#32375=CARTESIAN_POINT('Ctrl Pts',(21.3064559759895,-63.9528111531126,35.5576462091981));
#32376=CARTESIAN_POINT('Ctrl Pts',(22.4285781341657,-65.9871398034319,35.4465130912066));
#32377=CARTESIAN_POINT('Ctrl Pts',(21.3279816257553,-68.0334049278494,35.335379973215));
#32378=CARTESIAN_POINT('Ctrl Pts',(19.0119582319098,-68.2185344164948,35.2242468552235));
#32379=CARTESIAN_POINT('Ctrl Pts',(17.9980259839472,-66.8931862532338,35.144428624331));
#32380=CARTESIAN_POINT('Ctrl Pts',(17.9427193968075,-66.1070372217313,35.1016547661024));
#32381=CARTESIAN_POINT('Ctrl Pts',(17.9436250231948,-66.0016062109329,35.0959252805377));
#32382=CARTESIAN_POINT('Ctrl Pts',(17.9473272127329,-66.0023217579764,35.8540747194623));
#32383=CARTESIAN_POINT('Ctrl Pts',(17.9508754656456,-65.5321727435478,35.8286277343139));
#32384=CARTESIAN_POINT('Ctrl Pts',(18.3433679905248,-64.3705970778618,35.7661363765015));
#32385=CARTESIAN_POINT('Ctrl Pts',(20.2718170744413,-63.5871690673869,35.6666006460253));
#32386=CARTESIAN_POINT('Ctrl Pts',(22.1745314797546,-64.9187024309931,35.5554675280338));
#32387=CARTESIAN_POINT('Ctrl Pts',(22.0878551535464,-67.240916575683,35.4443344100422));
#32388=CARTESIAN_POINT('Ctrl Pts',(20.0898773540102,-68.4268764895147,35.3332012920506));
#32389=CARTESIAN_POINT('Ctrl Pts',(18.2789900436016,-67.5258396316566,35.2364480618574));
#32390=CARTESIAN_POINT('Ctrl Pts',(17.950084108963,-66.4181209144086,35.1767392043279));
#32391=CARTESIAN_POINT('Ctrl Pts',(17.9479090675131,-65.9988355335402,35.1540747194623));
#32392=CARTESIAN_POINT('Ctrl Pts',(21.2690708798524,-64.9206413469514,36.));
#32393=CARTESIAN_POINT('Ctrl Pts',(21.627967898288,-65.3426194852432,35.9629556273362));
#32394=CARTESIAN_POINT('Ctrl Pts',(21.8852406895061,-66.5657423547737,35.8888668820085));
#32395=CARTESIAN_POINT('Ctrl Pts',(20.5452621419689,-67.8933537625408,35.7777337640169));
#32396=CARTESIAN_POINT('Ctrl Pts',(18.7059925990704,-67.4836984587995,35.6666006460253));
#32397=CARTESIAN_POINT('Ctrl Pts',(18.0511941008261,-65.7182471306277,35.5554675280338));
#32398=CARTESIAN_POINT('Ctrl Pts',(19.1799450576061,-64.2095972418381,35.4443344100422));
#32399=CARTESIAN_POINT('Ctrl Pts',(21.0592800369867,-64.3401306149583,35.3332012920507));
#32400=CARTESIAN_POINT('Ctrl Pts',(21.9691014340041,-65.9895728981713,35.2220681740591));
#32401=CARTESIAN_POINT('Ctrl Pts',(21.0767331249584,-67.6486933251233,35.1109350560675));
#32402=CARTESIAN_POINT('Ctrl Pts',(19.198891550973,-67.7987970983723,34.999801938076));
#32403=CARTESIAN_POINT('Ctrl Pts',(18.0542583326729,-66.302604885796,34.8886688200844));
#32404=CARTESIAN_POINT('Ctrl Pts',(18.6904432824267,-64.5294397602479,34.7775357020929));
#32405=CARTESIAN_POINT('Ctrl Pts',(20.525186680335,-64.1021977783242,34.6664025841013));
#32406=CARTESIAN_POINT('Ctrl Pts',(21.8792582580528,-65.4118948076596,34.5552694661098));
#32407=CARTESIAN_POINT('Ctrl Pts',(21.513358861174,-67.2598510025468,34.4441363481182));
#32408=CARTESIAN_POINT('Ctrl Pts',(19.7623737940666,-67.9547408964103,34.3330032301266));
#32409=CARTESIAN_POINT('Ctrl Pts',(18.2288736212496,-66.860575523791,34.2218701121351));
#32410=CARTESIAN_POINT('Ctrl Pts',(18.3163780021904,-64.9787772891694,34.1107369941435));
#32411=CARTESIAN_POINT('Ctrl Pts',(19.9447995117363,-64.0316424102007,33.999603876152));
#32412=CARTESIAN_POINT('Ctrl Pts',(21.6237426760499,-64.8860258031255,33.8884707581604));
#32413=CARTESIAN_POINT('Ctrl Pts',(21.8165726357416,-66.7599622607762,33.7773376401688));
#32414=CARTESIAN_POINT('Ctrl Pts',(20.3468038184027,-67.9383513284147,33.6662045221772));
#32415=CARTESIAN_POINT('Ctrl Pts',(18.5596264969971,-67.3426849761128,33.5550714041857));
#32416=CARTESIAN_POINT('Ctrl Pts',(18.0907356977871,-65.5181404817989,33.4439382861942));
#32417=CARTESIAN_POINT('Ctrl Pts',(19.3692787360241,-64.1346127865089,33.3328051682026));
#32418=CARTESIAN_POINT('Ctrl Pts',(21.2250826999231,-64.4583608888479,33.2216720502111));
#32419=CARTESIAN_POINT('Ctrl Pts',(21.9596427581053,-66.1930777845806,33.1105389322195));
#32420=CARTESIAN_POINT('Ctrl Pts',(20.9006606332631,-67.7510822921252,32.9994058142279));
#32421=CARTESIAN_POINT('Ctrl Pts',(19.017358447211,-67.7064273641261,32.8882726962364));
#32422=CARTESIAN_POINT('Ctrl Pts',(18.0334084866612,-66.0999829480836,32.7771395782448));
#32423=CARTESIAN_POINT('Ctrl Pts',(18.8493604834091,-64.4020302026989,32.6660064602532));
#32424=CARTESIAN_POINT('Ctrl Pts',(20.7184230544699,-64.1666023112654,32.5548733422617));
#32425=CARTESIAN_POINT('Ctrl Pts',(21.9299565692245,-65.6091721464001,32.4437402242701));
#32426=CARTESIAN_POINT('Ctrl Pts',(21.3751178694742,-67.4094430159797,32.3326071062786));
#32427=CARTESIAN_POINT('Ctrl Pts',(19.5617171714693,-67.9197361622001,32.221473988287));
#32428=CARTESIAN_POINT('Ctrl Pts',(18.1494501687797,-66.6730112126951,32.1103408702954));
#32429=CARTESIAN_POINT('Ctrl Pts',(18.4308792085545,-64.8103199118686,31.9992077523039));
#32430=CARTESIAN_POINT('Ctrl Pts',(20.1484293566527,-64.0364706530518,31.8880746343123));
#32431=CARTESIAN_POINT('Ctrl Pts',(21.7301311154199,-65.0597207363241,31.7769415163208));
#32432=CARTESIAN_POINT('Ctrl Pts',(21.7283487800576,-66.9435514107436,31.6658083983292));
#32433=CARTESIAN_POINT('Ctrl Pts',(20.1447136140416,-67.963806696229,31.5546752803377));
#32434=CARTESIAN_POINT('Ctrl Pts',(18.4286308525823,-67.1867087986473,31.4435421623461));
#32435=CARTESIAN_POINT('Ctrl Pts',(18.1507269833267,-65.3234883001403,31.3324090443545));
#32436=CARTESIAN_POINT('Ctrl Pts',(19.5653505656071,-64.079437936586,31.221275926363));
#32437=CARTESIAN_POINT('Ctrl Pts',(21.377782417879,-64.5931615660544,31.1101428083714));
#32438=CARTESIAN_POINT('Ctrl Pts',(21.9292135723205,-66.394479102891,30.9990096903798));
#32439=CARTESIAN_POINT('Ctrl Pts',(20.7149525322679,-67.8347538382155,30.8878765723883));
#32440=CARTESIAN_POINT('Ctrl Pts',(18.8463387944264,-67.5957896455979,30.7767434543967));
#32441=CARTESIAN_POINT('Ctrl Pts',(18.0336011995884,-65.8962959596606,30.6656103364052));
#32442=CARTESIAN_POINT('Ctrl Pts',(19.0205891835897,-64.2917162931933,30.5544772184136));
#32443=CARTESIAN_POINT('Ctrl Pts',(20.9039724960038,-64.2506251125867,30.443344100422));
#32444=CARTESIAN_POINT('Ctrl Pts',(21.9600046000645,-65.8106306836656,30.3322109824305));
#32445=CARTESIAN_POINT('Ctrl Pts',(21.2221633491169,-67.5439545065572,30.2210778644389));
#32446=CARTESIAN_POINT('Ctrl Pts',(19.3657500971768,-67.8641903955905,30.1099447464474));
#32447=CARTESIAN_POINT('Ctrl Pts',(18.0898273201334,-66.4782458607604,29.9988116284558));
#32448=CARTESIAN_POINT('Ctrl Pts',(18.562169763368,-64.6545918905887,29.8876785104643));
#32449=CARTESIAN_POINT('Ctrl Pts',(20.3504710316148,-64.0623083768974,29.7765453924727));
#32450=CARTESIAN_POINT('Ctrl Pts',(21.8180074173223,-65.2434765034687,29.6654122744811));
#32451=CARTESIAN_POINT('Ctrl Pts',(21.6216318586219,-67.1170447105401,29.5542791564896));
#32452=CARTESIAN_POINT('Ctrl Pts',(19.9410749961026,-67.9682496320738,29.443146038498));
#32453=CARTESIAN_POINT('Ctrl Pts',(18.3144486164159,-67.018035020783,29.3320129205064));
#32454=CARTESIAN_POINT('Ctrl Pts',(18.2305052056412,-65.1360746890036,29.2208798025149));
#32455=CARTESIAN_POINT('Ctrl Pts',(19.7660730773002,-64.044812805617,29.1097466845233));
#32456=CARTESIAN_POINT('Ctrl Pts',(21.515740075888,-64.7430151979478,28.9986135665318));
#32457=CARTESIAN_POINT('Ctrl Pts',(21.8781420980751,-66.5916595555565,28.8874804485402));
#32458=CARTESIAN_POINT('Ctrl Pts',(20.5215945491511,-67.8987938004266,28.7763473305487));
#32459=CARTESIAN_POINT('Ctrl Pts',(18.6876631390829,-67.4680772233507,28.6652142125571));
#32460=CARTESIAN_POINT('Ctrl Pts',(18.054834077201,-65.6937185885076,28.5540810945655));
#32461=CARTESIAN_POINT('Ctrl Pts',(19.2022974288504,-64.1996807565816,28.442947976574));
#32462=CARTESIAN_POINT('Ctrl Pts',(21.0798495708812,-64.3533659561062,28.3318148585824));
#32463=CARTESIAN_POINT('Ctrl Pts',(21.9690808831804,-66.0141154434886,28.2206817405909));
#32464=CARTESIAN_POINT('Ctrl Pts',(21.0561318689169,-67.6619459214081,28.1095486225993));
#32465=CARTESIAN_POINT('Ctrl Pts',(19.1765693992908,-67.7886980785084,27.9984155046078));
#32466=CARTESIAN_POINT('Ctrl Pts',(18.0506430253154,-66.2783633516724,27.8872823866161));
#32467=CARTESIAN_POINT('Ctrl Pts',(18.7088448805761,-64.5132595291411,27.7761492686247));
#32468=CARTESIAN_POINT('Ctrl Pts',(20.5487627203804,-64.1088791030149,27.665016150633));
#32469=CARTESIAN_POINT('Ctrl Pts',(21.8864313196484,-65.4353269557215,27.5538830326415));
#32470=CARTESIAN_POINT('Ctrl Pts',(21.4975637254705,-67.2785858036292,27.4427499146499));
#32471=CARTESIAN_POINT('Ctrl Pts',(19.738066867186,-67.9516325998814,27.3316167966584));
#32472=CARTESIAN_POINT('Ctrl Pts',(18.2183015196908,-66.8384684242688,27.2204836786668));
#32473=CARTESIAN_POINT('Ctrl Pts',(18.329216752231,-64.9579049468497,27.1093505606753));
#32474=CARTESIAN_POINT('Ctrl Pts',(19.9692985667656,-64.0311078747868,26.9982174426837));
#32475=CARTESIAN_POINT('Ctrl Pts',(21.637479556849,-64.9063183780325,26.8870843246922));
#32476=CARTESIAN_POINT('Ctrl Pts',(21.8069747751189,-66.7825093336883,26.7759512067006));
#32477=CARTESIAN_POINT('Ctrl Pts',(20.3226556188142,-67.942516977602,26.6648180887091));
#32478=CARTESIAN_POINT('Ctrl Pts',(18.5430292180468,-67.3246565676388,26.5536849707175));
#32479=CARTESIAN_POINT('Ctrl Pts',(18.0968800670332,-65.4944184471421,26.4425518527259));
#32480=CARTESIAN_POINT('Ctrl Pts',(19.3925406976308,-64.1269082277483,26.3314187347344));
#32481=CARTESIAN_POINT('Ctrl Pts',(21.2441729623769,-64.473725792196,26.2202856167428));
#32482=CARTESIAN_POINT('Ctrl Pts',(21.9570872251895,-66.2174486486474,26.1091524987512));
#32483=CARTESIAN_POINT('Ctrl Pts',(20.878802090704,-67.7621558105501,25.9980193807597));
#32484=CARTESIAN_POINT('Ctrl Pts',(18.9961949942118,-67.6940648934545,25.8868862627682));
#32485=CARTESIAN_POINT('Ctrl Pts',(18.0323251000736,-66.0755065322627,25.7757531447765));
#32486=CARTESIAN_POINT('Ctrl Pts',(18.8693181114084,-64.3878268177706,25.664620026785));
#32487=CARTESIAN_POINT('Ctrl Pts',(20.7412167237518,-64.1757009701585,25.5534869087934));
#32488=CARTESIAN_POINT('Ctrl Pts',(21.9346029210715,-65.6331865461314,25.4423537908019));
#32489=CARTESIAN_POINT('Ctrl Pts',(21.3576070345443,-67.4265115788993,25.3312206728103));
#32490=CARTESIAN_POINT('Ctrl Pts',(19.5375918595496,-67.9140030887383,25.2200875548188));
#32491=CARTESIAN_POINT('Ctrl Pts',(18.1417564769822,-66.6501901871505,25.1089544368272));
#32492=CARTESIAN_POINT('Ctrl Pts',(18.4447225902452,-64.7903672241964,24.9978213188356));
#32493=CARTESIAN_POINT('Ctrl Pts',(20.1751288422123,-64.0395085417223,24.8866882008441));
#32494=CARTESIAN_POINT('Ctrl Pts',(21.2151340020225,-64.7327675918889,24.8125994555164));
#32495=CARTESIAN_POINT('Ctrl Pts',(21.4735782273626,-65.2227463683951,24.7755550828525));
#32496=CARTESIAN_POINT('Ctrl Pts',(21.3677806246588,-64.8366876301902,36.0748149723825));
#32497=CARTESIAN_POINT('Ctrl Pts',(21.7545930524416,-65.2914876975058,36.0377705997186));
#32498=CARTESIAN_POINT('Ctrl Pts',(22.0318768075623,-66.6097464244853,35.9636818543909));
#32499=CARTESIAN_POINT('Ctrl Pts',(20.5876732379454,-68.0406209244431,35.8525487363994));
#32500=CARTESIAN_POINT('Ctrl Pts',(18.6053432639141,-67.5991021754578,35.7414156184078));
#32501=CARTESIAN_POINT('Ctrl Pts',(17.899613810049,-65.6963320790133,35.6302825004163));
#32502=CARTESIAN_POINT('Ctrl Pts',(19.1161602719207,-64.0703377235837,35.5191493824247));
#32503=CARTESIAN_POINT('Ctrl Pts',(21.1416720166543,-64.2110241276764,35.4080162644332));
#32504=CARTESIAN_POINT('Ctrl Pts',(22.122260334058,-65.9887618665916,35.2968831464416));
#32505=CARTESIAN_POINT('Ctrl Pts',(21.1604826252241,-67.776930526032,35.18575002845));
#32506=CARTESIAN_POINT('Ctrl Pts',(19.1365804446186,-67.9387095377464,35.0746169104585));
#32507=CARTESIAN_POINT('Ctrl Pts',(17.9029163812577,-66.3261418304446,34.9634837924669));
#32508=CARTESIAN_POINT('Ctrl Pts',(18.5885845041241,-64.4150579488825,34.8523506744754));
#32509=CARTESIAN_POINT('Ctrl Pts',(20.5660362845728,-63.9545846103219,34.7412175564838));
#32510=CARTESIAN_POINT('Ctrl Pts',(22.0254290559355,-65.3661513315646,34.6300844384922));
#32511=CARTESIAN_POINT('Ctrl Pts',(21.6310695969247,-67.3578436150398,34.5189513205007));
#32512=CARTESIAN_POINT('Ctrl Pts',(19.7438909634229,-68.1067828178749,34.4078182025091));
#32513=CARTESIAN_POINT('Ctrl Pts',(18.0911134412297,-66.9275120453744,34.2966850845175));
#32514=CARTESIAN_POINT('Ctrl Pts',(18.1854240102639,-64.899345450667,34.185551966526));
#32515=CARTESIAN_POINT('Ctrl Pts',(19.9405059563517,-63.8785413671765,34.0744188485344));
#32516=CARTESIAN_POINT('Ctrl Pts',(21.7500391877175,-64.7993796508576,33.9632857305429));
#32517=CARTESIAN_POINT('Ctrl Pts',(21.9578676761867,-66.8190729708356,33.8521526125513));
#32518=CARTESIAN_POINT('Ctrl Pts',(20.3737786051983,-68.089118451048,33.7410194945598));
#32519=CARTESIAN_POINT('Ctrl Pts',(18.4475926435972,-67.447120507218,33.6298863765682));
#32520=CARTESIAN_POINT('Ctrl Pts',(17.9422309964094,-65.480660912431,33.5187532585767));
#32521=CARTESIAN_POINT('Ctrl Pts',(19.3202205344693,-63.989520893903,33.407620140585));
#32522=CARTESIAN_POINT('Ctrl Pts',(21.3203709951603,-64.3384504837937,33.2964870225936));
#32523=CARTESIAN_POINT('Ctrl Pts',(22.1120659518255,-66.2080955894538,33.1853539046019));
#32524=CARTESIAN_POINT('Ctrl Pts',(20.9707150192538,-67.8872834207894,33.0742207866104));
#32525=CARTESIAN_POINT('Ctrl Pts',(18.9409274941004,-67.8391551828144,32.9630876686188));
#32526=CARTESIAN_POINT('Ctrl Pts',(17.8804448110288,-66.1077597330111,32.8519545506273));
#32527=CARTESIAN_POINT('Ctrl Pts',(18.7598624617856,-64.2777383342113,32.7408214326357));
#32528=CARTESIAN_POINT('Ctrl Pts',(20.7743027988527,-64.0239985994815,32.6296883146442));
#32529=CARTESIAN_POINT('Ctrl Pts',(22.0800707381493,-65.5787731211726,32.5185551966526));
#32530=CARTESIAN_POINT('Ctrl Pts',(21.4820760671049,-67.5190710616904,32.4074220786611));
#32531=CARTESIAN_POINT('Ctrl Pts',(19.5276270455007,-68.069055376497,32.2962889606695));
#32532=CARTESIAN_POINT('Ctrl Pts',(18.0055123442725,-66.7253587735064,32.1851558426779));
#32533=CARTESIAN_POINT('Ctrl Pts',(18.3088312478353,-64.7177852711602,32.0740227246864));
#32534=CARTESIAN_POINT('Ctrl Pts',(20.1599743571327,-63.8837451561277,31.9628896066947));
#32535=CARTESIAN_POINT('Ctrl Pts',(21.8647026382529,-64.9865847691865,31.8517564887033));
#32536=CARTESIAN_POINT('Ctrl Pts',(21.8627816708634,-67.0169418891202,31.7406233707116));
#32537=CARTESIAN_POINT('Ctrl Pts',(20.1559695999277,-68.1165537656887,31.6294902527202));
#32538=CARTESIAN_POINT('Ctrl Pts',(18.3064080122344,-67.2790123291542,31.5183571347285));
#32539=CARTESIAN_POINT('Ctrl Pts',(18.0068884708754,-65.2708684675433,31.407224016737));
#32540=CARTESIAN_POINT('Ctrl Pts',(19.5315430490765,-63.930054482774,31.2960908987454));
#32541=CARTESIAN_POINT('Ctrl Pts',(21.4849478670487,-64.4837361076318,31.1849577807539));
#32542=CARTESIAN_POINT('Ctrl Pts',(22.0792699501195,-66.4251621263501,31.0738246627623));
#32543=CARTESIAN_POINT('Ctrl Pts',(20.7705623355731,-67.9774630328147,30.9626915447708));
#32544=CARTESIAN_POINT('Ctrl Pts',(18.7566057424723,-67.7199119394606,30.8515584267792));
#32545=CARTESIAN_POINT('Ctrl Pts',(17.8806525133819,-65.8882297440381,30.7404253087877));
#32546=CARTESIAN_POINT('Ctrl Pts',(18.9444095207486,-64.1588440861061,30.6292921907961));
#32547=CARTESIAN_POINT('Ctrl Pts',(20.9742844823626,-64.1145567877606,30.5181590728046));
#32548=CARTESIAN_POINT('Ctrl Pts',(22.1124559382548,-65.7959013275781,30.4070259548129));
#32549=CARTESIAN_POINT('Ctrl Pts',(21.3172245740007,-67.6640450056417,30.2958928368214));
#32550=CARTESIAN_POINT('Ctrl Pts',(19.3164174341671,-68.0091891983687,30.1847597188298));
#32551=CARTESIAN_POINT('Ctrl Pts',(17.9412519641314,-66.5154443558325,30.0736266008383));
#32552=CARTESIAN_POINT('Ctrl Pts',(18.4503337280557,-64.5499445511462,29.9624934828467));
#32553=CARTESIAN_POINT('Ctrl Pts',(20.3777310583335,-63.9115925668773,29.8513603648552));
#32554=CARTESIAN_POINT('Ctrl Pts',(21.9594140566749,-65.1846332643177,29.7402272468636));
#32555=CARTESIAN_POINT('Ctrl Pts',(21.7477641885617,-67.2039296907767,29.6290941288721));
#32556=CARTESIAN_POINT('Ctrl Pts',(19.9364917437487,-68.1213422780259,29.5179610108805));
#32557=CARTESIAN_POINT('Ctrl Pts',(18.1833445547175,-67.0972189172074,29.4068278928889));
#32558=CARTESIAN_POINT('Ctrl Pts',(18.0928719320704,-65.0688776172449,29.2956947748974));
#32559=CARTESIAN_POINT('Ctrl Pts',(19.7478779810218,-63.8927361705997,29.1845616569058));
#32560=CARTESIAN_POINT('Ctrl Pts',(21.6336360251679,-64.6452455217178,29.0734285389143));
#32561=CARTESIAN_POINT('Ctrl Pts',(22.0242260797931,-66.6376794939764,28.9622954209227));
#32562=CARTESIAN_POINT('Ctrl Pts',(20.5621647534294,-68.0464840945274,28.8511623029311));
#32563=CARTESIAN_POINT('Ctrl Pts',(18.5855881181383,-67.5822659029381,28.7400291849396));
#32564=CARTESIAN_POINT('Ctrl Pts',(17.9035369078357,-65.6698956796004,28.628896066948));
#32565=CARTESIAN_POINT('Ctrl Pts',(19.1402512354662,-64.0596499230725,28.5177629489565));
#32566=CARTESIAN_POINT('Ctrl Pts',(21.1638414717776,-64.2252889283823,28.4066298309649));
#32567=CARTESIAN_POINT('Ctrl Pts',(22.1222381847684,-66.0152133583859,28.2954967129734));
#32568=CARTESIAN_POINT('Ctrl Pts',(21.1382789805698,-67.7912139239986,28.1843635949818));
#32569=CARTESIAN_POINT('Ctrl Pts',(19.1125220511464,-67.927825004883,28.0732304769903));
#32570=CARTESIAN_POINT('Ctrl Pts',(17.8990198712721,-66.3000147628294,27.9620973589986));
#32571=CARTESIAN_POINT('Ctrl Pts',(18.6084173990482,-64.3976192014007,27.8509642410071));
#32572=CARTESIAN_POINT('Ctrl Pts',(20.5914460952399,-63.9617856158794,27.7398311230156));
#32573=CARTESIAN_POINT('Ctrl Pts',(22.0331600462417,-65.3914060581699,27.628698005024));
#32574=CARTESIAN_POINT('Ctrl Pts',(21.6140458979948,-67.3780356297918,27.5175648870324));
#32575=CARTESIAN_POINT('Ctrl Pts',(19.7176934167296,-68.1034327545841,27.4064317690409));
#32576=CARTESIAN_POINT('Ctrl Pts',(18.0797190298508,-66.9036854310583,27.2952986510493));
#32577=CARTESIAN_POINT('Ctrl Pts',(18.1992613725651,-64.8768496343423,27.1841655330578));
#32578=CARTESIAN_POINT('Ctrl Pts',(19.966910575135,-63.8779652550036,27.0730324150662));
#32579=CARTESIAN_POINT('Ctrl Pts',(21.7648445383867,-64.8212506048152,26.9618992970747));
#32580=CARTESIAN_POINT('Ctrl Pts',(21.9475232832876,-66.8433737801612,26.8507661790831));
#32581=CARTESIAN_POINT('Ctrl Pts',(20.3477521317823,-68.0936081090632,26.7396330610915));
#32582=CARTESIAN_POINT('Ctrl Pts',(18.4297044098267,-67.4276898290772,26.6284999431));
#32583=CARTESIAN_POINT('Ctrl Pts',(17.9488532815309,-65.4550937515292,26.5173668251084));
#32584=CARTESIAN_POINT('Ctrl Pts',(19.3452918373275,-63.981217065991,26.4062337071169));
#32585=CARTESIAN_POINT('Ctrl Pts',(21.3409461194645,-64.355010486417,26.2951005891253));
#32586=CARTESIAN_POINT('Ctrl Pts',(22.1093116467166,-66.2343620464388,26.1839674711338));
#32587=CARTESIAN_POINT('Ctrl Pts',(20.947156294938,-67.8992182497961,26.0728343531421));
#32588=CARTESIAN_POINT('Ctrl Pts',(18.9181179241837,-67.8258311454213,25.9617012351507));
#32589=CARTESIAN_POINT('Ctrl Pts',(17.8792771574272,-66.0813795143389,25.850568117159));
#32590=CARTESIAN_POINT('Ctrl Pts',(18.7813724162924,-64.2624301942028,25.7394349991675));
#32591=CARTESIAN_POINT('Ctrl Pts',(20.798869385088,-64.0338049621852,25.6283018811759));
#32592=CARTESIAN_POINT('Ctrl Pts',(22.0850784884117,-65.6046553876296,25.5171687631844));
#32593=CARTESIAN_POINT('Ctrl Pts',(21.4632032199543,-67.5374672364217,25.4060356451928));
#32594=CARTESIAN_POINT('Ctrl Pts',(19.5016252399817,-68.0628763782035,25.2949025272013));
#32595=CARTESIAN_POINT('Ctrl Pts',(17.9972202285682,-66.7007627032078,25.1837694092097));
#32596=CARTESIAN_POINT('Ctrl Pts',(18.3237513831539,-64.6962806412445,25.0726362912182));
#32597=CARTESIAN_POINT('Ctrl Pts',(20.1887505583808,-63.8870193351586,24.9615031732266));
#32598=CARTESIAN_POINT('Ctrl Pts',(21.3096484764695,-64.6342008454597,24.8874144278989));
#32599=CARTESIAN_POINT('Ctrl Pts',(21.5881947811615,-65.162290716277,24.850370055235));
#32600=CARTESIAN_POINT('Ctrl Pts',(21.4664903694652,-64.752733913429,36.149629944765));
#32601=CARTESIAN_POINT('Ctrl Pts',(21.8812182065951,-65.2403559097683,36.1125855721011));
#32602=CARTESIAN_POINT('Ctrl Pts',(22.1785129256187,-66.6537504941968,36.0384968267734));
#32603=CARTESIAN_POINT('Ctrl Pts',(20.6300843339218,-68.1878880863455,35.9273637087819));
#32604=CARTESIAN_POINT('Ctrl Pts',(18.5046939287577,-67.7145058921161,35.8162305907903));
#32605=CARTESIAN_POINT('Ctrl Pts',(17.748033519272,-65.674417027399,35.7050974727988));
#32606=CARTESIAN_POINT('Ctrl Pts',(19.0523754862353,-63.9310782053294,35.5939643548071));
#32607=CARTESIAN_POINT('Ctrl Pts',(21.2240639963219,-64.0819176403945,35.4828312368157));
#32608=CARTESIAN_POINT('Ctrl Pts',(22.2754192341118,-65.9879508350117,35.371698118824));
#32609=CARTESIAN_POINT('Ctrl Pts',(21.2442321254897,-67.9051677269406,35.2605650008325));
#32610=CARTESIAN_POINT('Ctrl Pts',(19.0742693382642,-68.0786219771207,35.1494318828409));
#32611=CARTESIAN_POINT('Ctrl Pts',(17.7515744298424,-66.3496787750931,35.0382987648494));
#32612=CARTESIAN_POINT('Ctrl Pts',(18.4867257258214,-64.3006761375172,34.9271656468578));
#32613=CARTESIAN_POINT('Ctrl Pts',(20.6068858888105,-63.8069714423194,34.8160325288663));
#32614=CARTESIAN_POINT('Ctrl Pts',(22.1715998538182,-65.3204078554697,34.7048994108747));
#32615=CARTESIAN_POINT('Ctrl Pts',(21.7487803326752,-67.4558362275328,34.5937662928832));
#32616=CARTESIAN_POINT('Ctrl Pts',(19.7254081327793,-68.2588247393393,34.4826331748916));
#32617=CARTESIAN_POINT('Ctrl Pts',(17.9533532612099,-66.9944485669578,34.3715000569001));
#32618=CARTESIAN_POINT('Ctrl Pts',(18.0544700183374,-64.8199136121645,34.2603669389084));
#32619=CARTESIAN_POINT('Ctrl Pts',(19.936212400967,-63.7254403241524,34.1492338209169));
#32620=CARTESIAN_POINT('Ctrl Pts',(21.876335699385,-64.7127334985896,34.0381007029253));
#32621=CARTESIAN_POINT('Ctrl Pts',(22.0991627166318,-66.878183680895,33.9269675849338));
#32622=CARTESIAN_POINT('Ctrl Pts',(20.4007533919938,-68.2398855736812,33.8158344669422));
#32623=CARTESIAN_POINT('Ctrl Pts',(18.3355587901974,-67.5515560383232,33.7047013489507));
#32624=CARTESIAN_POINT('Ctrl Pts',(17.7937262950319,-65.443181343063,33.5935682309591));
#32625=CARTESIAN_POINT('Ctrl Pts',(19.2711623329145,-63.844429001297,33.4824351129676));
#32626=CARTESIAN_POINT('Ctrl Pts',(21.4156592903974,-64.2185400787396,33.371301994976));
#32627=CARTESIAN_POINT('Ctrl Pts',(22.2644891455457,-66.2231133943269,33.2601688769845));
#32628=CARTESIAN_POINT('Ctrl Pts',(21.0407694052443,-68.0234845494536,33.1490357589929));
#32629=CARTESIAN_POINT('Ctrl Pts',(18.8644965409898,-67.9718830015026,33.0379026410013));
#32630=CARTESIAN_POINT('Ctrl Pts',(17.7274811353965,-66.1155365179385,32.9267695230098));
#32631=CARTESIAN_POINT('Ctrl Pts',(18.670364440162,-64.1534464657238,32.8156364050182));
#32632=CARTESIAN_POINT('Ctrl Pts',(20.8301825432355,-63.8813948876976,32.7045032870266));
#32633=CARTESIAN_POINT('Ctrl Pts',(22.230184907074,-65.5483740959451,32.5933701690351));
#32634=CARTESIAN_POINT('Ctrl Pts',(21.5890342647356,-67.6286991074011,32.4822370510435));
#32635=CARTESIAN_POINT('Ctrl Pts',(19.493536919532,-68.2183745907937,32.371103933052));
#32636=CARTESIAN_POINT('Ctrl Pts',(17.8615745197653,-66.7777063343178,32.2599708150604));
#32637=CARTESIAN_POINT('Ctrl Pts',(18.1867832871161,-64.6252506304517,32.1488376970689));
#32638=CARTESIAN_POINT('Ctrl Pts',(20.1715193576126,-63.7310196592038,32.0377045790772));
#32639=CARTESIAN_POINT('Ctrl Pts',(21.9992741610859,-64.9134488020487,31.9265714610858));
#32640=CARTESIAN_POINT('Ctrl Pts',(21.9972145616692,-67.090332367497,31.8154383430941));
#32641=CARTESIAN_POINT('Ctrl Pts',(20.1672255858137,-68.2693008351482,31.7043052251026));
#32642=CARTESIAN_POINT('Ctrl Pts',(18.1841851718866,-67.3713158596613,31.593172107111));
#32643=CARTESIAN_POINT('Ctrl Pts',(17.863049958424,-65.218248634946,31.4820389891195));
#32644=CARTESIAN_POINT('Ctrl Pts',(19.4977355325458,-63.7806710289621,31.3709058711279));
#32645=CARTESIAN_POINT('Ctrl Pts',(21.5921133162185,-64.3743106492091,31.2597727531364));
#32646=CARTESIAN_POINT('Ctrl Pts',(22.2293263279185,-66.4558451498092,31.1486396351448));
#32647=CARTESIAN_POINT('Ctrl Pts',(20.8261721388783,-68.1201722274138,31.0375065171533));
#32648=CARTESIAN_POINT('Ctrl Pts',(18.6668726905181,-67.8440342333234,30.9263733991617));
#32649=CARTESIAN_POINT('Ctrl Pts',(17.7277038271754,-65.8801635284154,30.8152402811702));
#32650=CARTESIAN_POINT('Ctrl Pts',(18.8682298579076,-64.0259718790191,30.7041071631786));
#32651=CARTESIAN_POINT('Ctrl Pts',(21.0445964687214,-63.9784884629342,30.592974045187));
#32652=CARTESIAN_POINT('Ctrl Pts',(22.2649072764451,-65.7811719714907,30.4818409271955));
#32653=CARTESIAN_POINT('Ctrl Pts',(21.4122857988845,-67.7841355047261,30.3707078092039));
#32654=CARTESIAN_POINT('Ctrl Pts',(19.2670847711574,-68.154188001147,30.2595746912124));
#32655=CARTESIAN_POINT('Ctrl Pts',(17.7926766081294,-66.5526428509046,30.1484415732208));
#32656=CARTESIAN_POINT('Ctrl Pts',(18.3384976927434,-64.4452972117037,30.0373084552292));
#32657=CARTESIAN_POINT('Ctrl Pts',(20.4049910850522,-63.760876756857,29.9261753372377));
#32658=CARTESIAN_POINT('Ctrl Pts',(22.1008206960275,-65.1257900251668,29.8150422192461));
#32659=CARTESIAN_POINT('Ctrl Pts',(21.8738965185015,-67.2908146710133,29.7039091012545));
#32660=CARTESIAN_POINT('Ctrl Pts',(19.9319084913948,-68.2744349239781,29.592775983263));
#32661=CARTESIAN_POINT('Ctrl Pts',(18.0522404930191,-67.1764028136319,29.4816428652714));
#32662=CARTESIAN_POINT('Ctrl Pts',(17.9552386584996,-65.0016805454862,29.3705097472799));
#32663=CARTESIAN_POINT('Ctrl Pts',(19.7296828847433,-63.7406595355825,29.2593766292883));
#32664=CARTESIAN_POINT('Ctrl Pts',(21.7515319744479,-64.5474758454877,29.1482435112967));
#32665=CARTESIAN_POINT('Ctrl Pts',(22.1703100615111,-66.6836994323963,29.0371103933052));
#32666=CARTESIAN_POINT('Ctrl Pts',(20.6027349577076,-68.1941743886282,28.9259772753136));
#32667=CARTESIAN_POINT('Ctrl Pts',(18.4835130971936,-67.6964545825255,28.8148441573221));
#32668=CARTESIAN_POINT('Ctrl Pts',(17.7522397384703,-65.6460727706933,28.7037110393305));
#32669=CARTESIAN_POINT('Ctrl Pts',(19.0782050420819,-63.9196190895633,28.592577921339));
#32670=CARTESIAN_POINT('Ctrl Pts',(21.2478333726739,-64.0972119006585,28.4814448033474));
#32671=CARTESIAN_POINT('Ctrl Pts',(22.2753954863563,-66.0163112732831,28.3703116853558));
#32672=CARTESIAN_POINT('Ctrl Pts',(21.2204260922228,-67.9204819265891,28.2591785673643));
#32673=CARTESIAN_POINT('Ctrl Pts',(19.048474703002,-68.0669519312575,28.1480454493727));
#32674=CARTESIAN_POINT('Ctrl Pts',(17.7473967172287,-66.3216661739864,28.0369123313812));
#32675=CARTESIAN_POINT('Ctrl Pts',(18.5079899175204,-64.2819788736603,27.9257792133896));
#32676=CARTESIAN_POINT('Ctrl Pts',(20.6341294700995,-63.8146921287439,27.8146460953981));
#32677=CARTESIAN_POINT('Ctrl Pts',(22.179888772835,-65.3474851606182,27.7035129774065));
#32678=CARTESIAN_POINT('Ctrl Pts',(21.7305280705192,-67.4774854559544,27.5923798594149));
#32679=CARTESIAN_POINT('Ctrl Pts',(19.6973199662731,-68.2552329092867,27.4812467414234));
#32680=CARTESIAN_POINT('Ctrl Pts',(17.9411365400108,-66.968902437848,27.3701136234318));
#32681=CARTESIAN_POINT('Ctrl Pts',(18.0693059928992,-64.7957943218349,27.2589805054402));
#32682=CARTESIAN_POINT('Ctrl Pts',(19.9645225835043,-63.7248226352203,27.1478473874487));
#32683=CARTESIAN_POINT('Ctrl Pts',(21.8922095199243,-64.736182831598,27.0367142694572));
#32684=CARTESIAN_POINT('Ctrl Pts',(22.0880717914564,-66.904238226634,26.9255811514656));
#32685=CARTESIAN_POINT('Ctrl Pts',(20.3728486447502,-68.2446992405243,26.814448033474));
#32686=CARTESIAN_POINT('Ctrl Pts',(18.3163796016065,-67.5307230905157,26.7033149154825));
#32687=CARTESIAN_POINT('Ctrl Pts',(17.8008264960285,-65.4157690559163,26.5921817974909));
#32688=CARTESIAN_POINT('Ctrl Pts',(19.2980429770242,-63.8355259042336,26.4810486794994));
#32689=CARTESIAN_POINT('Ctrl Pts',(21.4377192765522,-64.2362951806379,26.3699155615078));
#32690=CARTESIAN_POINT('Ctrl Pts',(22.2615360682436,-66.2512754442303,26.2587824435162));
#32691=CARTESIAN_POINT('Ctrl Pts',(21.0155104991719,-68.0362806890421,26.1476493255246));
#32692=CARTESIAN_POINT('Ctrl Pts',(18.8400408541557,-67.9575973973882,26.0365162075331));
#32693=CARTESIAN_POINT('Ctrl Pts',(17.7262292147809,-66.0872524964152,25.9253830895415));
#32694=CARTESIAN_POINT('Ctrl Pts',(18.6934267211763,-64.1370335706351,25.81424997155));
#32695=CARTESIAN_POINT('Ctrl Pts',(20.8565220464243,-63.8919089542118,25.7031168535584));
#32696=CARTESIAN_POINT('Ctrl Pts',(22.235554055752,-65.576124229128,25.5919837355669));
#32697=CARTESIAN_POINT('Ctrl Pts',(21.5687994053643,-67.6484228939442,25.4808506175753));
#32698=CARTESIAN_POINT('Ctrl Pts',(19.4656586204139,-68.2117496676687,25.3697174995837));
#32699=CARTESIAN_POINT('Ctrl Pts',(17.8526839801542,-66.7513352192652,25.2585843815922));
#32700=CARTESIAN_POINT('Ctrl Pts',(18.2027801760626,-64.6021940582926,25.1474512636006));
#32701=CARTESIAN_POINT('Ctrl Pts',(20.2023722745493,-63.7345301285949,25.0363181456091));
#32702=CARTESIAN_POINT('Ctrl Pts',(21.4041629509165,-64.5356340990305,24.9622294002814));
#32703=CARTESIAN_POINT('Ctrl Pts',(21.7028113349605,-65.1018350641589,24.9251850276175));
#32704=CARTESIAN_POINT('Ctrl Pts',(21.5652001142717,-64.6687801966678,36.2244449171475));
#32705=CARTESIAN_POINT('Ctrl Pts',(22.0078433607487,-65.1892241220309,36.1874005444836));
#32706=CARTESIAN_POINT('Ctrl Pts',(22.325149043675,-66.6977545639082,36.1133117991559));
#32707=CARTESIAN_POINT('Ctrl Pts',(20.6724954298983,-68.3351552482478,36.0021786811644));
#32708=CARTESIAN_POINT('Ctrl Pts',(18.4040445936014,-67.8299096087744,35.8910455631728));
#32709=CARTESIAN_POINT('Ctrl Pts',(17.5964532284949,-65.6525019757846,35.7799124451812));
#32710=CARTESIAN_POINT('Ctrl Pts',(18.9885907005499,-63.7918186870749,35.6687793271897));
#32711=CARTESIAN_POINT('Ctrl Pts',(21.3064559759895,-63.9528111531126,35.5576462091981));
#32712=CARTESIAN_POINT('Ctrl Pts',(22.4285781341657,-65.9871398034319,35.4465130912066));
#32713=CARTESIAN_POINT('Ctrl Pts',(21.3279816257553,-68.0334049278494,35.335379973215));
#32714=CARTESIAN_POINT('Ctrl Pts',(19.0119582319098,-68.2185344164948,35.2242468552235));
#32715=CARTESIAN_POINT('Ctrl Pts',(17.6002324784272,-66.3732157197415,35.1131137372319));
#32716=CARTESIAN_POINT('Ctrl Pts',(18.3848669475188,-64.186294326152,35.0019806192404));
#32717=CARTESIAN_POINT('Ctrl Pts',(20.6477354930483,-63.6593582743169,34.8908475012487));
#32718=CARTESIAN_POINT('Ctrl Pts',(22.317770651701,-65.2746643793748,34.7797143832572));
#32719=CARTESIAN_POINT('Ctrl Pts',(21.8664910684258,-67.5538288400258,34.6685812652657));
#32720=CARTESIAN_POINT('Ctrl Pts',(19.7069253021358,-68.4108666608038,34.5574481472741));
#32721=CARTESIAN_POINT('Ctrl Pts',(17.81559308119,-67.0613850885411,34.4463150292825));
#32722=CARTESIAN_POINT('Ctrl Pts',(17.923516026411,-64.740481773662,34.335181911291));
#32723=CARTESIAN_POINT('Ctrl Pts',(19.9319188455824,-63.5723392811283,34.2240487932994));
#32724=CARTESIAN_POINT('Ctrl Pts',(22.0026322110525,-64.6260873463218,34.1129156753078));
#32725=CARTESIAN_POINT('Ctrl Pts',(22.2404577570769,-66.9372943909543,34.0017825573163));
#32726=CARTESIAN_POINT('Ctrl Pts',(20.4277281787894,-68.3906526963146,33.8906494393247));
#32727=CARTESIAN_POINT('Ctrl Pts',(18.2235249367975,-67.6559915694283,33.7795163213332));
#32728=CARTESIAN_POINT('Ctrl Pts',(17.6452215936543,-65.4057017736952,33.6683832033416));
#32729=CARTESIAN_POINT('Ctrl Pts',(19.2221041313598,-63.699337108691,33.55725008535));
#32730=CARTESIAN_POINT('Ctrl Pts',(21.5109475856345,-64.0986296736855,33.4461169673585));
#32731=CARTESIAN_POINT('Ctrl Pts',(22.4169123392658,-66.2381311992,33.3349838493669));
#32732=CARTESIAN_POINT('Ctrl Pts',(21.110823791235,-68.1596856781178,33.2238507313754));
#32733=CARTESIAN_POINT('Ctrl Pts',(18.7880655878792,-68.1046108201909,33.1127176133838));
#32734=CARTESIAN_POINT('Ctrl Pts',(17.5745174597642,-66.123313302866,33.0015844953923));
#32735=CARTESIAN_POINT('Ctrl Pts',(18.5808664185384,-64.0291545972363,32.8904513774007));
#32736=CARTESIAN_POINT('Ctrl Pts',(20.8860622876183,-63.7387911759138,32.7793182594092));
#32737=CARTESIAN_POINT('Ctrl Pts',(22.3802990759988,-65.5179750707177,32.6681851414176));
#32738=CARTESIAN_POINT('Ctrl Pts',(21.6959924623663,-67.7383271531118,32.5570520234261));
#32739=CARTESIAN_POINT('Ctrl Pts',(19.4594467935634,-68.3676938050906,32.4459189054344));
#32740=CARTESIAN_POINT('Ctrl Pts',(17.7176366952581,-66.8300538951291,32.3347857874429));
#32741=CARTESIAN_POINT('Ctrl Pts',(18.0647353263969,-64.5327159897432,32.2236526694514));
#32742=CARTESIAN_POINT('Ctrl Pts',(20.1830643580926,-63.5782941622798,32.1125195514598));
#32743=CARTESIAN_POINT('Ctrl Pts',(22.1338456839189,-64.8403128349112,32.0013864334682));
#32744=CARTESIAN_POINT('Ctrl Pts',(22.131647452475,-67.1637228458735,31.8902533154766));
#32745=CARTESIAN_POINT('Ctrl Pts',(20.1784815716998,-68.4220479046079,31.7791201974851));
#32746=CARTESIAN_POINT('Ctrl Pts',(18.0619623315387,-67.4636193901682,31.6679870794935));
#32747=CARTESIAN_POINT('Ctrl Pts',(17.7192114459727,-65.165628802349,31.556853961502));
#32748=CARTESIAN_POINT('Ctrl Pts',(19.4639280160152,-63.6312875751501,31.4457208435104));
#32749=CARTESIAN_POINT('Ctrl Pts',(21.6992787653883,-64.2648851907865,31.3345877255189));
#32750=CARTESIAN_POINT('Ctrl Pts',(22.3793827057175,-66.4865281732684,31.2234546075273));
#32751=CARTESIAN_POINT('Ctrl Pts',(20.8817819421834,-68.2628814220129,31.1123214895357));
#32752=CARTESIAN_POINT('Ctrl Pts',(18.577139638564,-67.9681565271862,31.0011883715442));
#32753=CARTESIAN_POINT('Ctrl Pts',(17.5747551409689,-65.8720973127928,30.8900552535526));
#32754=CARTESIAN_POINT('Ctrl Pts',(18.7920501950665,-63.8930996719321,30.7789221355611));
#32755=CARTESIAN_POINT('Ctrl Pts',(21.1149084550803,-63.8424201381079,30.6677890175695));
#32756=CARTESIAN_POINT('Ctrl Pts',(22.4173586146354,-65.7664426154033,30.556655899578));
#32757=CARTESIAN_POINT('Ctrl Pts',(21.5073470237683,-67.9042260038106,30.4455227815864));
#32758=CARTESIAN_POINT('Ctrl Pts',(19.2177521081477,-68.2991868039253,30.3343896635948));
#32759=CARTESIAN_POINT('Ctrl Pts',(17.6441012521274,-66.5898413459768,30.2232565456033));
#32760=CARTESIAN_POINT('Ctrl Pts',(18.2266616574312,-64.3406498722612,30.1121234276117));
#32761=CARTESIAN_POINT('Ctrl Pts',(20.432251111771,-63.6101609468367,30.0009903096202));
#32762=CARTESIAN_POINT('Ctrl Pts',(22.24222733538,-65.0669467860159,29.8898571916286));
#32763=CARTESIAN_POINT('Ctrl Pts',(22.0000288484413,-67.3776996512498,29.7787240736371));
#32764=CARTESIAN_POINT('Ctrl Pts',(19.9273252390408,-68.4275275699302,29.6675909556455));
#32765=CARTESIAN_POINT('Ctrl Pts',(17.9211364313208,-67.2555867100563,29.5564578376539));
#32766=CARTESIAN_POINT('Ctrl Pts',(17.8176053849288,-64.9344834737275,29.4453247196624));
#32767=CARTESIAN_POINT('Ctrl Pts',(19.7114877884649,-63.5885829005652,29.3341916016708));
#32768=CARTESIAN_POINT('Ctrl Pts',(21.869427923728,-64.4497061692577,29.2230584836792));
#32769=CARTESIAN_POINT('Ctrl Pts',(22.3163940432292,-66.7297193708161,29.1119253656877));
#32770=CARTESIAN_POINT('Ctrl Pts',(20.6433051619858,-68.3418646827291,29.0007922476961));
#32771=CARTESIAN_POINT('Ctrl Pts',(18.3814380762489,-67.8106432621128,28.8896591297046));
#32772=CARTESIAN_POINT('Ctrl Pts',(17.6009425691049,-65.6222498617862,28.778526011713));
#32773=CARTESIAN_POINT('Ctrl Pts',(19.0161588486977,-63.7795882560541,28.6673928937214));
#32774=CARTESIAN_POINT('Ctrl Pts',(21.3318252735703,-63.9691348729347,28.5562597757299));
#32775=CARTESIAN_POINT('Ctrl Pts',(22.4285527879442,-66.0174091881803,28.4451266577383));
#32776=CARTESIAN_POINT('Ctrl Pts',(21.3025732038757,-68.0497499291796,28.3339935397468));
#32777=CARTESIAN_POINT('Ctrl Pts',(18.9844273548577,-68.2060788576321,28.2228604217552));
#32778=CARTESIAN_POINT('Ctrl Pts',(17.5957735631854,-66.3433175851434,28.1117273037636));
#32779=CARTESIAN_POINT('Ctrl Pts',(18.4075624359926,-64.16633854592,28.0005941857721));
#32780=CARTESIAN_POINT('Ctrl Pts',(20.676812844959,-63.6675986416085,27.8894610677805));
#32781=CARTESIAN_POINT('Ctrl Pts',(22.3266174994283,-65.3035642630666,27.778327949789));
#32782=CARTESIAN_POINT('Ctrl Pts',(21.8470102430435,-67.576935282117,27.6671948317974));
#32783=CARTESIAN_POINT('Ctrl Pts',(19.6769465158166,-68.4070330639894,27.5560617138059));
#32784=CARTESIAN_POINT('Ctrl Pts',(17.8025540501709,-67.0341194446376,27.4449285958143));
#32785=CARTESIAN_POINT('Ctrl Pts',(17.9393506132333,-64.7147390093274,27.3337954778228));
#32786=CARTESIAN_POINT('Ctrl Pts',(19.9621345918737,-63.5716800154371,27.2226623598312));
#32787=CARTESIAN_POINT('Ctrl Pts',(22.0195745014619,-64.6511150583807,27.1115292418397));
#32788=CARTESIAN_POINT('Ctrl Pts',(22.2286202996251,-66.9651026731069,27.000396123848));
#32789=CARTESIAN_POINT('Ctrl Pts',(20.3979451577182,-68.3957903719854,26.8892630058565));
#32790=CARTESIAN_POINT('Ctrl Pts',(18.2030547933863,-67.6337563519543,26.7781298878649));
#32791=CARTESIAN_POINT('Ctrl Pts',(17.6527997105261,-65.3764443603032,26.6669967698734));
#32792=CARTESIAN_POINT('Ctrl Pts',(19.2507941167209,-63.6898347424764,26.5558636518818));
#32793=CARTESIAN_POINT('Ctrl Pts',(21.5344924336398,-64.1175798748589,26.4447305338903));
#32794=CARTESIAN_POINT('Ctrl Pts',(22.4137604897707,-66.2681888420218,26.3335974158987));
#32795=CARTESIAN_POINT('Ctrl Pts',(21.0838647034058,-68.1733431282881,26.2224642979072));
#32796=CARTESIAN_POINT('Ctrl Pts',(18.7619637841276,-68.0893636493551,26.1113311799156));
#32797=CARTESIAN_POINT('Ctrl Pts',(17.5731812721346,-66.0931254784914,26.000198061924));
#32798=CARTESIAN_POINT('Ctrl Pts',(18.6054810260603,-64.0116369470673,25.8890649439325));
#32799=CARTESIAN_POINT('Ctrl Pts',(20.9141747077605,-63.7500129462385,25.7779318259409));
#32800=CARTESIAN_POINT('Ctrl Pts',(22.3860296230922,-65.5475930706263,25.6667987079494));
#32801=CARTESIAN_POINT('Ctrl Pts',(21.6743955907743,-67.7593785514666,25.5556655899578));
#32802=CARTESIAN_POINT('Ctrl Pts',(19.429692000846,-68.3606229571339,25.4445324719662));
#32803=CARTESIAN_POINT('Ctrl Pts',(17.7081477317402,-66.8019077353226,25.3333993539747));
#32804=CARTESIAN_POINT('Ctrl Pts',(18.0818089689714,-64.5081074753406,25.2222662359831));
#32805=CARTESIAN_POINT('Ctrl Pts',(20.2159939907177,-63.5820409220313,25.1111331179916));
#32806=CARTESIAN_POINT('Ctrl Pts',(21.4986774253636,-64.4370673526013,25.0370443726639));
#32807=CARTESIAN_POINT('Ctrl Pts',(21.8174278887595,-65.0413794120408,25.));
#32808=CARTESIAN_POINT('Ctrl Pts',(21.2690708798524,-64.9206413469514,36.));
#32809=CARTESIAN_POINT('Ctrl Pts',(21.3144000906036,-64.9629286896491,36.));
#32810=CARTESIAN_POINT('Ctrl Pts',(21.3569992965038,-65.00778514716,36.));
#32811=CARTESIAN_POINT('Ctrl Pts',(21.3968699769242,-65.0548656952241,36.));
#32812=CARTESIAN_POINT('Ctrl Pts',(21.4393722521919,-65.1050537128971,36.));
#32813=CARTESIAN_POINT('Ctrl Pts',(21.4787746568644,-65.1577693380806,36.));
#32814=CARTESIAN_POINT('Ctrl Pts',(21.5150501504783,-65.2126493353753,36.));
#32815=CARTESIAN_POINT('Ctrl Pts',(21.5467912073906,-65.2606693330081,36.));
#32816=CARTESIAN_POINT('Ctrl Pts',(21.576137979607,-65.3103476536427,36.));
#32817=CARTESIAN_POINT('Ctrl Pts',(21.6030494591265,-65.3614685121224,36.));
#32818=CARTESIAN_POINT('Ctrl Pts',(21.6165497288404,-65.3871135301522,36.));
#32819=CARTESIAN_POINT('Ctrl Pts',(21.6294367784251,-65.4131219292723,36.));
#32820=CARTESIAN_POINT('Ctrl Pts',(21.6417030895028,-65.4394683087242,36.));
#32821=CARTESIAN_POINT('Ctrl Pts',(21.6473120464069,-65.4515155905833,36.));
#32822=CARTESIAN_POINT('Ctrl Pts',(21.6527917902974,-65.4636352254459,36.));
#32823=CARTESIAN_POINT('Ctrl Pts',(21.6581330897624,-65.4758048257742,36.));
#32824=CARTESIAN_POINT('Ctrl Pts',(21.6850520365028,-65.5371368715128,36.));
#32825=CARTESIAN_POINT('Ctrl Pts',(21.7085098197287,-65.5998443796051,36.));
#32826=CARTESIAN_POINT('Ctrl Pts',(21.7284829341248,-65.6635695831573,36.));
#32827=CARTESIAN_POINT('Ctrl Pts',(21.748810363471,-65.728425245979,36.));
#32828=CARTESIAN_POINT('Ctrl Pts',(21.7655289516023,-65.794335872963,36.));
#32829=CARTESIAN_POINT('Ctrl Pts',(21.7785746037815,-65.8609608298779,36.));
#32830=CARTESIAN_POINT('Ctrl Pts',(21.7894858424902,-65.9166852044715,36.));
#32831=CARTESIAN_POINT('Ctrl Pts',(21.7978271370784,-65.9729102271441,36.));
#32832=CARTESIAN_POINT('Ctrl Pts',(21.8035361618645,-66.0294488809297,36.));
#32833=CARTESIAN_POINT('Ctrl Pts',(21.8061657868978,-66.0554910623717,36.));
#32834=CARTESIAN_POINT('Ctrl Pts',(21.8082366141026,-66.0815998969239,36.));
#32835=CARTESIAN_POINT('Ctrl Pts',(21.8097407511271,-66.1077575099097,36.));
#32836=CARTESIAN_POINT('Ctrl Pts',(21.8103981162414,-66.1191893821185,36.));
#32837=CARTESIAN_POINT('Ctrl Pts',(21.8109471251284,-66.1306303661247,36.));
#32838=CARTESIAN_POINT('Ctrl Pts',(21.8113867843205,-66.142064834931,36.));
#32839=CARTESIAN_POINT('Ctrl Pts',(21.8140831607178,-66.2121910425829,36.));
#32840=CARTESIAN_POINT('Ctrl Pts',(21.8126787994894,-66.2822035594926,36.));
#32841=CARTESIAN_POINT('Ctrl Pts',(21.807119070444,-66.3517415844535,36.));
#32842=CARTESIAN_POINT('Ctrl Pts',(21.8021495116634,-66.4138980851956,36.));
#32843=CARTESIAN_POINT('Ctrl Pts',(21.7938596040808,-66.4756764464129,36.));
#32844=CARTESIAN_POINT('Ctrl Pts',(21.7821772238541,-66.5368311292835,36.));
#32845=CARTESIAN_POINT('Ctrl Pts',(21.7694467741587,-66.6034722245754,36.));
#32846=CARTESIAN_POINT('Ctrl Pts',(21.7526889329907,-66.6693735500384,36.));
#32847=CARTESIAN_POINT('Ctrl Pts',(21.7321489317058,-66.7343215285417,36.));
#32848=CARTESIAN_POINT('Ctrl Pts',(21.7242195708332,-66.759394358497,36.));
#32849=CARTESIAN_POINT('Ctrl Pts',(21.7157259981709,-66.7843250634018,36.));
#32850=CARTESIAN_POINT('Ctrl Pts',(21.7066803125378,-66.8091010351353,36.));
#32851=CARTESIAN_POINT('Ctrl Pts',(21.7027129368494,-66.8199676064378,36.));
#32852=CARTESIAN_POINT('Ctrl Pts',(21.6986394561303,-66.8308038451866,36.));
#32853=CARTESIAN_POINT('Ctrl Pts',(21.6944659765069,-66.8415961511061,36.));
#32854=CARTESIAN_POINT('Ctrl Pts',(21.6692431579055,-66.9068204720712,36.));
#32855=CARTESIAN_POINT('Ctrl Pts',(21.6403295196211,-66.9705593823762,36.));
#32856=CARTESIAN_POINT('Ctrl Pts',(21.6080377187698,-67.0325940771992,36.));
#32857=CARTESIAN_POINT('Ctrl Pts',(21.5749979079346,-67.096065748897,36.));
#32858=CARTESIAN_POINT('Ctrl Pts',(21.5384213156165,-67.157754156812,36.));
#32859=CARTESIAN_POINT('Ctrl Pts',(21.4985866955678,-67.2174212222795,36.));
#32860=CARTESIAN_POINT('Ctrl Pts',(21.4680940165069,-67.2630952785546,36.));
#32861=CARTESIAN_POINT('Ctrl Pts',(21.4356910398801,-67.3075849362939,36.));
#32862=CARTESIAN_POINT('Ctrl Pts',(21.4014832506304,-67.3507773033314,36.));
#32863=CARTESIAN_POINT('Ctrl Pts',(21.3801866940076,-67.3776673395035,36.));
#32864=CARTESIAN_POINT('Ctrl Pts',(21.3581902924914,-67.4040544403295,36.));
#32865=CARTESIAN_POINT('Ctrl Pts',(21.3355165916172,-67.429909675599,36.));
#32866=CARTESIAN_POINT('Ctrl Pts',(21.3228385096308,-67.4443667240687,36.));
#32867=CARTESIAN_POINT('Ctrl Pts',(21.3099442020298,-67.4586620153457,36.));
#32868=CARTESIAN_POINT('Ctrl Pts',(21.2968612936531,-67.4727650868957,36.));
#32869=CARTESIAN_POINT('Ctrl Pts',(21.2459900429151,-67.5276031143693,36.));
#32870=CARTESIAN_POINT('Ctrl Pts',(21.1922222505013,-67.5795961990397,36.));
#32871=CARTESIAN_POINT('Ctrl Pts',(21.1358428630979,-67.6284804213933,36.));
#32872=CARTESIAN_POINT('Ctrl Pts',(21.0936832829337,-67.665035240202,36.));
#32873=CARTESIAN_POINT('Ctrl Pts',(21.0500621937908,-67.6998514460096,36.));
#32874=CARTESIAN_POINT('Ctrl Pts',(21.0050823566734,-67.7328089375165,36.));
#32875=CARTESIAN_POINT('Ctrl Pts',(20.9910187117724,-67.7431136092779,36.));
#32876=CARTESIAN_POINT('Ctrl Pts',(20.9768221434489,-67.7532364967075,36.));
#32877=CARTESIAN_POINT('Ctrl Pts',(20.9624955512963,-67.7631737019372,36.));
#32878=CARTESIAN_POINT('Ctrl Pts',(20.948706193103,-67.7727382711587,36.));
#32879=CARTESIAN_POINT('Ctrl Pts',(20.9348034207359,-67.7821258761528,36.));
#32880=CARTESIAN_POINT('Ctrl Pts',(20.9207951934865,-67.7913303004398,36.));
#32881=CARTESIAN_POINT('Ctrl Pts',(20.8578414918468,-67.8326954617846,36.));
#32882=CARTESIAN_POINT('Ctrl Pts',(20.7927303375038,-67.8703849464026,36.));
#32883=CARTESIAN_POINT('Ctrl Pts',(20.725723015022,-67.9041195865683,36.));
#32884=CARTESIAN_POINT('Ctrl Pts',(20.6744956038834,-67.9299098766049,36.));
#32885=CARTESIAN_POINT('Ctrl Pts',(20.6221589702671,-67.9533882814079,36.));
#32886=CARTESIAN_POINT('Ctrl Pts',(20.5688159963225,-67.9744148066548,36.));
#32887=CARTESIAN_POINT('Ctrl Pts',(20.5563687509165,-67.9793212132615,36.));
#32888=CARTESIAN_POINT('Ctrl Pts',(20.5438666667748,-67.9840940496098,36.));
#32889=CARTESIAN_POINT('Ctrl Pts',(20.5313116823135,-67.9887339044341,36.));
#32890=CARTESIAN_POINT('Ctrl Pts',(18.332682461926,-66.0013023226252,34.8714803633902));
#32891=CARTESIAN_POINT('Ctrl Pts',(18.3319481762167,-66.0867862325851,34.8772098489549));
#32892=CARTESIAN_POINT('Ctrl Pts',(18.3379547950258,-66.1721666149879,34.8829393345197));
#32893=CARTESIAN_POINT('Ctrl Pts',(18.3510613606819,-66.256442733634,34.8886688200844));
#32894=CARTESIAN_POINT('Ctrl Pts',(18.435802738773,-66.8013356233214,34.9257131927482));
#32895=CARTESIAN_POINT('Ctrl Pts',(18.817347144873,-67.3000663608468,34.9627575654121));
#32896=CARTESIAN_POINT('Ctrl Pts',(19.3210929435872,-67.5244144340681,34.999801938076));
#32897=CARTESIAN_POINT('Ctrl Pts',(19.8248387423015,-67.7487625072893,35.0368463107398));
#32898=CARTESIAN_POINT('Ctrl Pts',(20.45078593363,-67.6987279162063,35.0738906834037));
#32899=CARTESIAN_POINT('Ctrl Pts',(20.9124875808018,-67.3971905495061,35.1109350560675));
#32900=CARTESIAN_POINT('Ctrl Pts',(21.3741892279737,-67.095653182806,35.1479794287314));
#32901=CARTESIAN_POINT('Ctrl Pts',(21.6716453309889,-66.5426130404886,35.1850238013952));
#32902=CARTESIAN_POINT('Ctrl Pts',(21.6687364829936,-65.9911859221278,35.2220681740591));
#32903=CARTESIAN_POINT('Ctrl Pts',(21.6658276349983,-65.439758803767,35.2591125467229));
#32904=CARTESIAN_POINT('Ctrl Pts',(21.3625538359925,-64.8899447093626,35.2961569193868));
#32905=CARTESIAN_POINT('Ctrl Pts',(20.8976944399262,-64.5932820999738,35.3332012920506));
#32906=CARTESIAN_POINT('Ctrl Pts',(20.4328350438599,-64.2966194905849,35.3702456647145));
#32907=CARTESIAN_POINT('Ctrl Pts',(19.806390050733,-64.2531083662115,35.4072900373783));
#32908=CARTESIAN_POINT('Ctrl Pts',(19.3050423947062,-64.4827944521564,35.4443344100422));
#32909=CARTESIAN_POINT('Ctrl Pts',(18.8036947386794,-64.7124805381013,35.481378782706));
#32910=CARTESIAN_POINT('Ctrl Pts',(18.4274444197528,-65.2153638343645,35.5184231553699));
#32911=CARTESIAN_POINT('Ctrl Pts',(18.3484523433302,-65.7610473705247,35.5554675280338));
#32912=CARTESIAN_POINT('Ctrl Pts',(18.3370706135895,-65.8396732633204,35.5608051398192));
#32913=CARTESIAN_POINT('Ctrl Pts',(18.3318602794101,-65.9191877343715,35.5661427516047));
#32914=CARTESIAN_POINT('Ctrl Pts',(18.3325226604529,-65.9987867968397,35.5714803633902));
#32915=CARTESIAN_POINT('Ctrl Pts',(19.4698297828114,-67.9851743256717,36.));
#32916=CARTESIAN_POINT('Ctrl Pts',(18.8097404375819,-67.8088876857537,35.9629556273362));
#32917=CARTESIAN_POINT('Ctrl Pts',(17.6907269068218,-66.7486281566044,35.8888668820084));
#32918=CARTESIAN_POINT('Ctrl Pts',(18.1186750965977,-64.4618780498746,35.7777337640169));
#32919=CARTESIAN_POINT('Ctrl Pts',(20.2718170744413,-63.5871690673869,35.6666006460253));
#32920=CARTESIAN_POINT('Ctrl Pts',(22.1745314797546,-64.9187024309931,35.5554675280338));
#32921=CARTESIAN_POINT('Ctrl Pts',(22.0878551535464,-67.240916575683,35.4443344100422));
#32922=CARTESIAN_POINT('Ctrl Pts',(20.0898773540102,-68.4268764895147,35.3332012920506));
#32923=CARTESIAN_POINT('Ctrl Pts',(18.0098480595359,-67.3919235970992,35.2220681740591));
#32924=CARTESIAN_POINT('Ctrl Pts',(17.751179915361,-65.0828969822093,35.1109350560676));
#32925=CARTESIAN_POINT('Ctrl Pts',(19.5507727141961,-63.6133045893429,34.9998019380759));
#32926=CARTESIAN_POINT('Ctrl Pts',(21.761489776565,-64.3280769471683,34.8886688200845));
#32927=CARTESIAN_POINT('Ctrl Pts',(22.3600352216356,-66.5730755571057,34.7775357020928));
#32928=CARTESIAN_POINT('Ctrl Pts',(20.7985769413999,-68.2935646002867,34.6664025841013));
#32929=CARTESIAN_POINT('Ctrl Pts',(18.5062329236883,-67.9148971913879,34.5552694661097));
#32930=CARTESIAN_POINT('Ctrl Pts',(17.5810416674194,-65.7836384245792,34.4441363481182));
#32931=CARTESIAN_POINT('Ctrl Pts',(18.8697771195624,-63.8504033302666,34.3330032301266));
#32932=CARTESIAN_POINT('Ctrl Pts',(21.1929366190789,-63.8845631923098,34.2218701121351));
#32933=CARTESIAN_POINT('Ctrl Pts',(22.4242737809404,-65.8548543459294,34.1107369941435));
#32934=CARTESIAN_POINT('Ctrl Pts',(21.4368200548297,-67.9579883834045,33.9996038761519));
#32935=CARTESIAN_POINT('Ctrl Pts',(19.134332114609,-68.2690944527448,33.8884707581604));
#32936=CARTESIAN_POINT('Ctrl Pts',(17.6241374689897,-66.5034359351233,33.7773376401688));
#32937=CARTESIAN_POINT('Ctrl Pts',(18.2884257380644,-64.2770130512471,33.6662045221773));
#32938=CARTESIAN_POINT('Ctrl Pts',(20.5192141319096,-63.6275356306401,33.5550714041857));
#32939=CARTESIAN_POINT('Ctrl Pts',(22.2747973195027,-65.14943098434,33.4439382861942));
#32940=CARTESIAN_POINT('Ctrl Pts',(21.9483964634611,-67.4498005771448,33.3328051682026));
#32941=CARTESIAN_POINT('Ctrl Pts',(19.838746476763,-68.4232556192041,33.221672050211));
#32942=CARTESIAN_POINT('Ctrl Pts',(17.8766820609866,-67.1788517396284,33.1105389322195));
#32943=CARTESIAN_POINT('Ctrl Pts',(17.8579617961865,-64.855516349057,32.9994058142279));
#32944=CARTESIAN_POINT('Ctrl Pts',(19.7997192052125,-63.5796574421335,32.8882726962363));
#32945=CARTESIAN_POINT('Ctrl Pts',(21.9247814806566,-64.5189913079908,32.7771395782448));
#32946=CARTESIAN_POINT('Ctrl Pts',(22.2882079863162,-66.8138026206755,32.6660064602532));
#32947=CARTESIAN_POINT('Ctrl Pts',(20.5573764799239,-68.3637897439758,32.5548733422617));
#32948=CARTESIAN_POINT('Ctrl Pts',(18.3164120809741,-67.7503434557233,32.4437402242701));
#32949=CARTESIAN_POINT('Ctrl Pts',(17.6163336108949,-65.53491394395,32.3326071062785));
#32950=CARTESIAN_POINT('Ctrl Pts',(19.0978804403178,-63.7451494962803,32.221473988287));
#32951=CARTESIAN_POINT('Ctrl Pts',(21.4050825978426,-64.0191129796669,32.1103408702954));
#32952=CARTESIAN_POINT('Ctrl Pts',(22.4262978583092,-66.1060622310153,31.9992077523039));
#32953=CARTESIAN_POINT('Ctrl Pts',(21.2268698206984,-68.0959391539699,31.8880746343123));
#32954=CARTESIAN_POINT('Ctrl Pts',(18.9045622340586,-68.16753006785,31.7769415163208));
#32955=CARTESIAN_POINT('Ctrl Pts',(17.5848424068188,-66.2553121504816,31.6658083983292));
#32956=CARTESIAN_POINT('Ctrl Pts',(18.4755698685349,-64.1094225040042,31.5546752803376));
#32957=CARTESIAN_POINT('Ctrl Pts',(20.7615157875532,-63.6938637942672,31.4435421623461));
#32958=CARTESIAN_POINT('Ctrl Pts',(22.3504924848334,-65.3889717086535,31.3324090443545));
#32959=CARTESIAN_POINT('Ctrl Pts',(21.7882059455114,-67.6433167651191,31.221275926363));
#32960=CARTESIAN_POINT('Ctrl Pts',(19.5892829417572,-68.3936336378304,31.1101428083714));
#32961=CARTESIAN_POINT('Ctrl Pts',(17.7662643553727,-66.9532027926971,30.9990096903798));
#32962=CARTESIAN_POINT('Ctrl Pts',(17.9876485499293,-64.6403632339913,30.8878765723883));
#32963=CARTESIAN_POINT('Ctrl Pts',(20.0508159969719,-63.5719167583182,30.7767434543967));
#32964=CARTESIAN_POINT('Ctrl Pts',(22.0674746434876,-64.7257476338574,30.6656103364051));
#32965=CARTESIAN_POINT('Ctrl Pts',(22.1918991212745,-67.0458244289748,30.5544772184136));
#32966=CARTESIAN_POINT('Ctrl Pts',(20.3102112509622,-68.4087215434459,30.443344100422));
#32967=CARTESIAN_POINT('Ctrl Pts',(18.1446058339735,-67.5670618949994,30.3322109824305));
#32968=CARTESIAN_POINT('Ctrl Pts',(17.6771301853349,-65.2911655212942,30.2210778644389));
#32969=CARTESIAN_POINT('Ctrl Pts',(19.3356364183429,-63.6640223619538,30.1099447464474));
#32970=CARTESIAN_POINT('Ctrl Pts',(21.6021943503792,-64.1748578801372,29.9988116284558));
#32971=CARTESIAN_POINT('Ctrl Pts',(22.4023609511933,-66.3561353033128,29.8876785104642));
#32972=CARTESIAN_POINT('Ctrl Pts',(21.0037922534698,-68.2114636795477,29.7765453924727));
#32973=CARTESIAN_POINT('Ctrl Pts',(18.6865133764925,-68.0427734538981,29.6654122744811));
#32974=CARTESIAN_POINT('Ctrl Pts',(17.5713891556791,-66.0044565604616,29.5542791564896));
#32975=CARTESIAN_POINT('Ctrl Pts',(18.6790251687795,-63.9620608474818,29.443146038498));
#32976=CARTESIAN_POINT('Ctrl Pts',(20.9956693404756,-63.7848672593903,29.3320129205065));
#32977=CARTESIAN_POINT('Ctrl Pts',(22.4010377426051,-65.6350503422798,29.2208798025149));
#32978=CARTESIAN_POINT('Ctrl Pts',(21.6088818987778,-67.8192497161933,29.1097466845234));
#32979=CARTESIAN_POINT('Ctrl Pts',(19.3442140162146,-68.3384001448757,28.9986135665318));
#32980=CARTESIAN_POINT('Ctrl Pts',(17.6797472774965,-66.717354722435,28.8874804485402));
#32981=CARTESIAN_POINT('Ctrl Pts',(18.1388671546711,-64.439758023215,28.7763473305486));
#32982=CARTESIAN_POINT('Ctrl Pts',(20.3013690653653,-63.5901561916745,28.6652142125571));
#32983=CARTESIAN_POINT('Ctrl Pts',(22.188046145667,-64.9461382640413,28.5540810945655));
#32984=CARTESIAN_POINT('Ctrl Pts',(22.0721372727958,-67.2666560767515,28.442947976574));
#32985=CARTESIAN_POINT('Ctrl Pts',(20.0597268093363,-68.4278803929209,28.3318148585824));
#32986=CARTESIAN_POINT('Ctrl Pts',(17.9926520191425,-67.3670130130489,28.2206817405909));
#32987=CARTESIAN_POINT('Ctrl Pts',(17.7627811094867,-65.0550015185249,28.1095486225993));
#32988=CARTESIAN_POINT('Ctrl Pts',(19.580500984485,-63.6078898290281,27.9984155046077));
#32989=CARTESIAN_POINT('Ctrl Pts',(21.7821628698452,-64.3501315205369,27.8872823866162));
#32990=CARTESIAN_POINT('Ctrl Pts',(22.3527191513918,-66.6023977826542,27.7761492686246));
#32991=CARTESIAN_POINT('Ctrl Pts',(20.7699742636292,-68.3033258839143,27.6650161506331));
#32992=CARTESIAN_POINT('Ctrl Pts',(18.4825186235667,-67.896159478245,27.5538830326415));
#32993=CARTESIAN_POINT('Ctrl Pts',(17.5839216673683,-65.7535532858717,27.44274991465));
#32994=CARTESIAN_POINT('Ctrl Pts',(18.8966146957805,-63.836504826525,27.3316167966584));
#32995=CARTESIAN_POINT('Ctrl Pts',(21.219169386089,-63.8995723038675,27.2204836786668));
#32996=CARTESIAN_POINT('Ctrl Pts',(22.4258922629222,-65.8850338815669,27.1093505606752));
#32997=CARTESIAN_POINT('Ctrl Pts',(21.41234306908,-67.9757169742283,26.9982174426837));
#32998=CARTESIAN_POINT('Ctrl Pts',(19.1061618881228,-68.2581461319033,26.8870843246921));
#32999=CARTESIAN_POINT('Ctrl Pts',(17.6180565701669,-66.4738310633369,26.7759512067006));
#33000=CARTESIAN_POINT('Ctrl Pts',(18.3099995480748,-64.2558471688686,26.664818088709));
#33001=CARTESIAN_POINT('Ctrl Pts',(20.5486976238089,-63.6341805685774,26.5536849707175));
#33002=CARTESIAN_POINT('Ctrl Pts',(22.2852057058799,-65.1778050816215,26.4425518527259));
#33003=CARTESIAN_POINT('Ctrl Pts',(21.9302042425984,-67.4739346416768,26.3314187347344));
#33004=CARTESIAN_POINT('Ctrl Pts',(19.8086025657231,-68.4210614106236,26.2202856167428));
#33005=CARTESIAN_POINT('Ctrl Pts',(17.8621779827765,-67.1523370729513,26.1091524987513));
#33006=CARTESIAN_POINT('Ctrl Pts',(17.8723670134724,-64.8289493110236,25.9980193807597));
#33007=CARTESIAN_POINT('Ctrl Pts',(19.829859942873,-63.5773515961876,25.8868862627681));
#33008=CARTESIAN_POINT('Ctrl Pts',(21.9430509240163,-64.5430603155101,25.7757531447765));
#33009=CARTESIAN_POINT('Ctrl Pts',(22.2779267364902,-66.8422110789462,25.664620026785));
#33010=CARTESIAN_POINT('Ctrl Pts',(20.5278715823273,-68.3705500709468,25.5534869087934));
#33011=CARTESIAN_POINT('Ctrl Pts',(18.2948525586908,-67.7292425039652,25.4423537908019));
#33012=CARTESIAN_POINT('Ctrl Pts',(17.6221226977641,-65.5053156304209,25.3312206728103));
#33013=CARTESIAN_POINT('Ctrl Pts',(19.1263754391461,-63.7340406632385,25.2200875548188));
#33014=CARTESIAN_POINT('Ctrl Pts',(21.4288957812291,-64.0368661589902,25.1089544368272));
#33015=CARTESIAN_POINT('Ctrl Pts',(22.4262529035541,-66.1360124024293,24.9978213188356));
#33016=CARTESIAN_POINT('Ctrl Pts',(21.1976530167761,-68.1115902981272,24.8866882008441));
#33017=CARTESIAN_POINT('Ctrl Pts',(19.656339145916,-68.1379171412778,24.8125994555164));
#33018=CARTESIAN_POINT('Ctrl Pts',(19.0504464477384,-67.8221815534923,24.7755550828525));
#33019=CARTESIAN_POINT('Ctrl Pts',(19.5032651029123,-67.8599788000028,36.0748149723825));
#33020=CARTESIAN_POINT('Ctrl Pts',(18.8848044607623,-67.6948097220376,36.0377705997186));
#33021=CARTESIAN_POINT('Ctrl Pts',(17.8363618040069,-66.7014157307813,35.963681854391));
#33022=CARTESIAN_POINT('Ctrl Pts',(18.2373213319382,-64.558880103346,35.8525487363994));
#33023=CARTESIAN_POINT('Ctrl Pts',(20.254674861246,-63.7393348661546,35.7414156184078));
#33024=CARTESIAN_POINT('Ctrl Pts',(22.03739409682,-64.9868947382407,35.6302825004162));
#33025=CARTESIAN_POINT('Ctrl Pts',(21.9561840352528,-67.1626578550281,35.5191493824247));
#33026=CARTESIAN_POINT('Ctrl Pts',(20.0842092157336,-68.2738249041152,35.4080162644331));
#33027=CARTESIAN_POINT('Ctrl Pts',(18.1353574997526,-67.3041415800863,35.2968831464416));
#33028=CARTESIAN_POINT('Ctrl Pts',(17.8930023281287,-65.1407343181651,35.18575002845));
#33029=CARTESIAN_POINT('Ctrl Pts',(19.5791033476643,-63.763822144746,35.0746169104584));
#33030=CARTESIAN_POINT('Ctrl Pts',(21.6504009740928,-64.4335172013417,34.9634837924669));
#33031=CARTESIAN_POINT('Ctrl Pts',(22.2111989978597,-66.536934400789,34.8523506744753));
#33032=CARTESIAN_POINT('Ctrl Pts',(20.7482144827116,-68.1489203632162,34.7412175564838));
#33033=CARTESIAN_POINT('Ctrl Pts',(18.6004377257187,-67.7941337111346,34.6300844384922));
#33034=CARTESIAN_POINT('Ctrl Pts',(17.7335938922303,-65.7972833225707,34.5189513205007));
#33035=CARTESIAN_POINT('Ctrl Pts',(18.9410549140662,-63.9859681930413,34.4078182025091));
#33036=CARTESIAN_POINT('Ctrl Pts',(21.1177037666367,-64.0179737546636,34.2966850845176));
#33037=CARTESIAN_POINT('Ctrl Pts',(22.2713863360217,-65.8640079936593,34.185551966526));
#33038=CARTESIAN_POINT('Ctrl Pts',(21.3462066312477,-67.8345073461254,34.0744188485344));
#33039=CARTESIAN_POINT('Ctrl Pts',(19.1889256808086,-68.1259934317763,33.9632857305429));
#33040=CARTESIAN_POINT('Ctrl Pts',(17.7739718460721,-66.4716866193462,33.8521526125513));
#33041=CARTESIAN_POINT('Ctrl Pts',(18.3963666058631,-64.3856736630535,33.7410194945598));
#33042=CARTESIAN_POINT('Ctrl Pts',(20.486469760124,-63.7771557017904,33.6298863765682));
#33043=CARTESIAN_POINT('Ctrl Pts',(22.1313366457862,-65.2030723364652,33.5187532585766));
#33044=CARTESIAN_POINT('Ctrl Pts',(21.8255203430619,-67.3583685336091,33.4076201405851));
#33045=CARTESIAN_POINT('Ctrl Pts',(19.8489159713744,-68.2704323849152,33.2964870225935));
#33046=CARTESIAN_POINT('Ctrl Pts',(18.0105896488994,-67.1045071537046,33.185353904602));
#33047=CARTESIAN_POINT('Ctrl Pts',(17.9930499823782,-64.9276935026936,33.0742207866103));
#33048=CARTESIAN_POINT('Ctrl Pts',(19.812349964668,-63.7322969634655,32.9630876686189));
#33049=CARTESIAN_POINT('Ctrl Pts',(21.803394645177,-64.612391499258,32.8519545506273));
#33050=CARTESIAN_POINT('Ctrl Pts',(22.1439015654733,-66.7624799506366,32.7408214326357));
#33051=CARTESIAN_POINT('Ctrl Pts',(20.5222253899178,-68.2147167402899,32.6296883146442));
#33052=CARTESIAN_POINT('Ctrl Pts',(18.4225879829121,-67.6399575988206,32.5185551966526));
#33053=CARTESIAN_POINT('Ctrl Pts',(17.7666601402804,-65.5642447148125,32.4074220786611));
#33054=CARTESIAN_POINT('Ctrl Pts',(19.1547728406628,-63.887352218967,32.2962889606695));
#33055=CARTESIAN_POINT('Ctrl Pts',(21.3164707050882,-64.1440381253301,32.185155842678));
#33056=CARTESIAN_POINT('Ctrl Pts',(22.2732827644345,-66.0993733893383,32.0740227246863));
#33057=CARTESIAN_POINT('Ctrl Pts',(21.1494969622328,-67.9637582161257,31.9628896066948));
#33058=CARTESIAN_POINT('Ctrl Pts',(18.973646296436,-68.0308342307446,31.8517564887032));
#33059=CARTESIAN_POINT('Ctrl Pts',(17.7371549370292,-66.2392108245296,31.7406233707117));
#33060=CARTESIAN_POINT('Ctrl Pts',(18.571708443967,-64.2286522564588,31.6294902527201));
#33061=CARTESIAN_POINT('Ctrl Pts',(20.7134905999941,-63.8393008628447,31.5183571347286));
#33062=CARTESIAN_POINT('Ctrl Pts',(22.2022580761902,-65.4275063638444,31.407224016737));
#33063=CARTESIAN_POINT('Ctrl Pts',(21.6754322810238,-67.5396805737836,31.2960908987455));
#33064=CARTESIAN_POINT('Ctrl Pts',(19.6151849178925,-68.2426785213593,31.1849577807539));
#33065=CARTESIAN_POINT('Ctrl Pts',(17.90713546408,-66.8930888152204,31.0738246627624));
#33066=CARTESIAN_POINT('Ctrl Pts',(18.1145580078869,-64.7261090737586,30.9626915447707));
#33067=CARTESIAN_POINT('Ctrl Pts',(20.0476112731494,-63.7250444478512,30.8515584267792));
#33068=CARTESIAN_POINT('Ctrl Pts',(21.9370888272641,-64.8061086846483,30.7404253087876));
#33069=CARTESIAN_POINT('Ctrl Pts',(22.0536664435935,-66.9798692443596,30.6292921907961));
#33070=CARTESIAN_POINT('Ctrl Pts',(20.2906476992225,-68.2568149043553,30.5181590728045));
#33071=CARTESIAN_POINT('Ctrl Pts',(18.2616167407412,-67.468234736516,30.407025954813));
#33072=CARTESIAN_POINT('Ctrl Pts',(17.8236225632318,-65.3358683486612,30.2958928368214));
#33073=CARTESIAN_POINT('Ctrl Pts',(19.377534677234,-63.8113413880787,30.1847597188299));
#33074=CARTESIAN_POINT('Ctrl Pts',(21.5011515546278,-64.2899609338901,30.0736266008383));
#33075=CARTESIAN_POINT('Ctrl Pts',(22.250855444477,-66.3336755394871,29.9624934828468));
#33076=CARTESIAN_POINT('Ctrl Pts',(20.9404878387337,-68.0719971580043,29.8513603648552));
#33077=CARTESIAN_POINT('Ctrl Pts',(18.7693487457408,-67.9139454245023,29.7402272468636));
#33078=CARTESIAN_POINT('Ctrl Pts',(17.7245501186072,-66.0041755063383,29.6290941288721));
#33079=CARTESIAN_POINT('Ctrl Pts',(18.7623327837589,-64.0905840004269,29.5179610108805));
#33080=CARTESIAN_POINT('Ctrl Pts',(20.9328771993214,-63.9245651712063,29.4068278928889));
#33081=CARTESIAN_POINT('Ctrl Pts',(22.2496156843762,-65.6580659856165,29.2956947748974));
#33082=CARTESIAN_POINT('Ctrl Pts',(21.5074173510794,-67.7045182683821,29.1845616569058));
#33083=CARTESIAN_POINT('Ctrl Pts',(19.385571326706,-68.1909283427392,29.0734285389143));
#33084=CARTESIAN_POINT('Ctrl Pts',(17.8260746078081,-66.6721145637219,28.9622954209227));
#33085=CARTESIAN_POINT('Ctrl Pts',(18.2562399727141,-64.5381550818151,28.8511623029312));
#33086=CARTESIAN_POINT('Ctrl Pts',(20.2823631483176,-63.7421336066862,28.7400291849396));
#33087=CARTESIAN_POINT('Ctrl Pts',(22.0500564568764,-65.0126003234735,28.6288960669481));
#33088=CARTESIAN_POINT('Ctrl Pts',(21.9414574066646,-67.1867740878903,28.5177629489565));
#33089=CARTESIAN_POINT('Ctrl Pts',(20.0559601228571,-68.2747654960968,28.4066298309649));
#33090=CARTESIAN_POINT('Ctrl Pts',(18.1192459320368,-67.2808019883787,28.2954967129734));
#33091=CARTESIAN_POINT('Ctrl Pts',(17.9038718899851,-65.1145980890199,28.1843635949818));
#33092=CARTESIAN_POINT('Ctrl Pts',(19.6069567969976,-63.7587488676727,28.0732304769902));
#33093=CARTESIAN_POINT('Ctrl Pts',(21.6697703134673,-64.4541808974103,27.9620973589987));
#33094=CARTESIAN_POINT('Ctrl Pts',(22.2043443174536,-66.5644074126972,27.8509642410071));
#33095=CARTESIAN_POINT('Ctrl Pts',(20.7214156401169,-68.1580660489999,27.7398311230156));
#33096=CARTESIAN_POINT('Ctrl Pts',(18.5782189739886,-67.7765776966548,27.628698005024));
#33097=CARTESIAN_POINT('Ctrl Pts',(17.7362922642471,-65.7690955108168,27.5175648870325));
#33098=CARTESIAN_POINT('Ctrl Pts',(18.9661999716884,-63.9729462019864,27.4064317690409));
#33099=CARTESIAN_POINT('Ctrl Pts',(21.142282157498,-64.0320363127692,27.2952986510493));
#33100=CARTESIAN_POINT('Ctrl Pts',(22.2729027480241,-65.892284249177,27.1841655330578));
#33101=CARTESIAN_POINT('Ctrl Pts',(21.3232732928534,-67.8511178788426,27.0730324150662));
#33102=CARTESIAN_POINT('Ctrl Pts',(19.1625320168477,-68.1157355695839,26.9618992970746));
#33103=CARTESIAN_POINT('Ctrl Pts',(17.7682744406861,-66.4439487863571,26.8507661790831));
#33104=CARTESIAN_POINT('Ctrl Pts',(18.4165798580372,-64.365842612451,26.7396330610915));
#33105=CARTESIAN_POINT('Ctrl Pts',(20.5140938680794,-63.7833815750203,26.6284999431));
#33106=CARTESIAN_POINT('Ctrl Pts',(22.1410886246193,-65.2296570140577,26.5173668251084));
#33107=CARTESIAN_POINT('Ctrl Pts',(21.8084754192525,-67.3809805771999,26.4062337071169));
#33108=CARTESIAN_POINT('Ctrl Pts',(19.82067309378,-68.2683765546589,26.2951005891253));
#33109=CARTESIAN_POINT('Ctrl Pts',(17.9970002740845,-67.0796646412509,26.1839674711337));
#33110=CARTESIAN_POINT('Ctrl Pts',(18.0065467309583,-64.9028019216962,26.0728343531422));
#33111=CARTESIAN_POINT('Ctrl Pts',(19.840589869013,-63.7301365362829,25.9617012351506));
#33112=CARTESIAN_POINT('Ctrl Pts',(21.8205119214269,-64.634942588673,25.850568117159));
#33113=CARTESIAN_POINT('Ctrl Pts',(22.1342687052924,-66.7890968222338,25.7394349991675));
#33114=CARTESIAN_POINT('Ctrl Pts',(20.4945812262208,-68.2210507255145,25.6283018811759));
#33115=CARTESIAN_POINT('Ctrl Pts',(18.4023881174058,-67.6201873839723,25.5171687631844));
#33116=CARTESIAN_POINT('Ctrl Pts',(17.7720841369082,-65.5365130264827,25.4060356451928));
#33117=CARTESIAN_POINT('Ctrl Pts',(19.1814707951151,-63.876943967317,25.2949025272013));
#33118=CARTESIAN_POINT('Ctrl Pts',(21.3387821039848,-64.1606716958669,25.1837694092097));
#33119=CARTESIAN_POINT('Ctrl Pts',(22.2732406447625,-66.1274347455458,25.0726362912181));
#33120=CARTESIAN_POINT('Ctrl Pts',(21.1221227235089,-67.9784223168809,24.9615031732266));
#33121=CARTESIAN_POINT('Ctrl Pts',(19.6780122054163,-68.003088850947,24.8874144278989));
#33122=CARTESIAN_POINT('Ctrl Pts',(19.1103302849355,-67.7072652086133,24.850370055235));
#33123=CARTESIAN_POINT('Ctrl Pts',(19.5367004230132,-67.7347832743338,36.149629944765));
#33124=CARTESIAN_POINT('Ctrl Pts',(18.9598684839428,-67.5807317583216,36.1125855721011));
#33125=CARTESIAN_POINT('Ctrl Pts',(17.981996701192,-66.6542033049582,36.0384968267734));
#33126=CARTESIAN_POINT('Ctrl Pts',(18.3559675672787,-64.6558821568174,35.9273637087819));
#33127=CARTESIAN_POINT('Ctrl Pts',(20.2375326480507,-63.8915006649221,35.8162305907903));
#33128=CARTESIAN_POINT('Ctrl Pts',(21.9002567138854,-65.0550870454884,35.7050974727987));
#33129=CARTESIAN_POINT('Ctrl Pts',(21.8245129169592,-67.0843991343733,35.5939643548072));
#33130=CARTESIAN_POINT('Ctrl Pts',(20.078541077457,-68.1207733187157,35.4828312368156));
#33131=CARTESIAN_POINT('Ctrl Pts',(18.2608669399692,-67.2163595630733,35.3716981188241));
#33132=CARTESIAN_POINT('Ctrl Pts',(18.0348247408964,-65.1985716541211,35.2605650008325));
#33133=CARTESIAN_POINT('Ctrl Pts',(19.6074339811324,-63.9143397001489,35.149431882841));
#33134=CARTESIAN_POINT('Ctrl Pts',(21.5393121716205,-64.5389574555151,35.0382987648494));
#33135=CARTESIAN_POINT('Ctrl Pts',(22.0623627740838,-66.5007932444724,34.9271656468579));
#33136=CARTESIAN_POINT('Ctrl Pts',(20.6978520240233,-68.0042761261457,34.8160325288663));
#33137=CARTESIAN_POINT('Ctrl Pts',(18.6946425277492,-67.6733702308812,34.7048994108747));
#33138=CARTESIAN_POINT('Ctrl Pts',(17.8861461170412,-65.8109282205623,34.5937662928832));
#33139=CARTESIAN_POINT('Ctrl Pts',(19.01233270857,-64.121533055816,34.4826331748916));
#33140=CARTESIAN_POINT('Ctrl Pts',(21.0424709141944,-64.1513843170174,34.3715000569001));
#33141=CARTESIAN_POINT('Ctrl Pts',(22.1184988911029,-65.8731616413895,34.2603669389085));
#33142=CARTESIAN_POINT('Ctrl Pts',(21.2555932076657,-67.7110263088461,34.1492338209169));
#33143=CARTESIAN_POINT('Ctrl Pts',(19.2435192470082,-67.9828924108079,34.0381007029253));
#33144=CARTESIAN_POINT('Ctrl Pts',(17.9238062231545,-66.4399373035691,33.9269675849338));
#33145=CARTESIAN_POINT('Ctrl Pts',(18.5043074736616,-64.4943342748599,33.8158344669423));
#33146=CARTESIAN_POINT('Ctrl Pts',(20.4537253883383,-63.9267757729409,33.7047013489506));
#33147=CARTESIAN_POINT('Ctrl Pts',(21.9878759720698,-65.2567136885904,33.5935682309591));
#33148=CARTESIAN_POINT('Ctrl Pts',(21.7026442226628,-67.2669364900734,33.4824351129675));
#33149=CARTESIAN_POINT('Ctrl Pts',(19.8590854659858,-68.1176091506262,33.371301994976));
#33150=CARTESIAN_POINT('Ctrl Pts',(18.1444972368122,-67.0301625677809,33.2601688769844));
#33151=CARTESIAN_POINT('Ctrl Pts',(18.12813816857,-64.9998706563301,33.1490357589929));
#33152=CARTESIAN_POINT('Ctrl Pts',(19.8249807241235,-63.8849364847975,33.0379026410013));
#33153=CARTESIAN_POINT('Ctrl Pts',(21.6820078096973,-64.7057916905251,32.9267695230098));
#33154=CARTESIAN_POINT('Ctrl Pts',(21.9995951446305,-66.7111572805976,32.8156364050182));
#33155=CARTESIAN_POINT('Ctrl Pts',(20.4870742999116,-68.0656437366041,32.7045032870267));
#33156=CARTESIAN_POINT('Ctrl Pts',(18.5287638848501,-67.5295717419178,32.5933701690351));
#33157=CARTESIAN_POINT('Ctrl Pts',(17.9169866696659,-65.5935754856751,32.4822370510435));
#33158=CARTESIAN_POINT('Ctrl Pts',(19.2116652410078,-64.0295549416535,32.371103933052));
#33159=CARTESIAN_POINT('Ctrl Pts',(21.2278588123338,-64.2689632709934,32.2599708150604));
#33160=CARTESIAN_POINT('Ctrl Pts',(22.1202676705596,-66.0926845476613,32.1488376970689));
#33161=CARTESIAN_POINT('Ctrl Pts',(21.0721241037672,-67.8315772782816,32.0377045790773));
#33162=CARTESIAN_POINT('Ctrl Pts',(19.0427303588134,-67.8941383936393,31.9265714610858));
#33163=CARTESIAN_POINT('Ctrl Pts',(17.8894674672395,-66.2231094985776,31.8154383430942));
#33164=CARTESIAN_POINT('Ctrl Pts',(18.667847019399,-64.3478820089134,31.7043052251026));
#33165=CARTESIAN_POINT('Ctrl Pts',(20.665465412435,-63.9847379314221,31.5931721071111));
#33166=CARTESIAN_POINT('Ctrl Pts',(22.054023667547,-65.4660410190354,31.4820389891195));
#33167=CARTESIAN_POINT('Ctrl Pts',(21.5626586165363,-67.4360443824481,31.3709058711279));
#33168=CARTESIAN_POINT('Ctrl Pts',(19.6410868940278,-68.0917234048882,31.2597727531364));
#33169=CARTESIAN_POINT('Ctrl Pts',(18.0480065727872,-66.8329748377437,31.1486396351448));
#33170=CARTESIAN_POINT('Ctrl Pts',(18.2414674658445,-64.8118549135259,31.0375065171533));
#33171=CARTESIAN_POINT('Ctrl Pts',(20.0444065493269,-63.8781721373842,30.9263733991617));
#33172=CARTESIAN_POINT('Ctrl Pts',(21.8067030110406,-64.8864697354392,30.8152402811701));
#33173=CARTESIAN_POINT('Ctrl Pts',(21.9154337659124,-66.9139140597444,30.7041071631786));
#33174=CARTESIAN_POINT('Ctrl Pts',(20.2710841474828,-68.1049082652647,30.592974045187));
#33175=CARTESIAN_POINT('Ctrl Pts',(18.3786276475089,-67.3694075780326,30.4818409271955));
#33176=CARTESIAN_POINT('Ctrl Pts',(17.9701149411287,-65.3805711760282,30.3707078092039));
#33177=CARTESIAN_POINT('Ctrl Pts',(19.419432936125,-63.9586604142035,30.2595746912124));
#33178=CARTESIAN_POINT('Ctrl Pts',(21.4001087588765,-64.4050639876431,30.1484415732208));
#33179=CARTESIAN_POINT('Ctrl Pts',(22.0993499377606,-66.3112157756614,30.0373084552292));
#33180=CARTESIAN_POINT('Ctrl Pts',(20.8771834239977,-67.9325306364607,29.9261753372377));
#33181=CARTESIAN_POINT('Ctrl Pts',(18.852184114989,-67.7851173951066,29.8150422192461));
#33182=CARTESIAN_POINT('Ctrl Pts',(17.8777110815354,-66.0038944522149,29.7039091012546));
#33183=CARTESIAN_POINT('Ctrl Pts',(18.8456403987383,-64.2191071533719,29.592775983263));
#33184=CARTESIAN_POINT('Ctrl Pts',(20.8700850581672,-64.0642630830224,29.4816428652715));
#33185=CARTESIAN_POINT('Ctrl Pts',(22.0981936261472,-65.6810816289533,29.3705097472799));
#33186=CARTESIAN_POINT('Ctrl Pts',(21.405952803381,-67.5897868205709,29.2593766292883));
#33187=CARTESIAN_POINT('Ctrl Pts',(19.4269286371974,-68.0434565406025,29.1482435112968));
#33188=CARTESIAN_POINT('Ctrl Pts',(17.9724019381197,-66.626874405009,29.0371103933052));
#33189=CARTESIAN_POINT('Ctrl Pts',(18.3736127907571,-64.636552140415,28.9259772753136));
#33190=CARTESIAN_POINT('Ctrl Pts',(20.26335723127,-63.8941110216982,28.8148441573221));
#33191=CARTESIAN_POINT('Ctrl Pts',(21.9120667680857,-65.0790623829053,28.7037110393305));
#33192=CARTESIAN_POINT('Ctrl Pts',(21.8107775405334,-67.1068920990293,28.592577921339));
#33193=CARTESIAN_POINT('Ctrl Pts',(20.0521934363779,-68.1216505992727,28.4814448033474));
#33194=CARTESIAN_POINT('Ctrl Pts',(18.245839844931,-67.1945909637086,28.3703116853559));
#33195=CARTESIAN_POINT('Ctrl Pts',(18.0449626704835,-65.1741946595148,28.2591785673642));
#33196=CARTESIAN_POINT('Ctrl Pts',(19.6334126095104,-63.9096079063174,28.1480454493728));
#33197=CARTESIAN_POINT('Ctrl Pts',(21.5573777570894,-64.5582302742836,28.0369123313811));
#33198=CARTESIAN_POINT('Ctrl Pts',(22.0559694835154,-66.5264170427403,27.9257792133896));
#33199=CARTESIAN_POINT('Ctrl Pts',(20.6728570166046,-68.0128062140853,27.8146460953981));
#33200=CARTESIAN_POINT('Ctrl Pts',(18.6739193244105,-67.6569959150645,27.7035129774065));
#33201=CARTESIAN_POINT('Ctrl Pts',(17.888662861126,-65.7846377357619,27.5923798594149));
#33202=CARTESIAN_POINT('Ctrl Pts',(19.0357852475963,-64.1093875774479,27.4812467414234));
#33203=CARTESIAN_POINT('Ctrl Pts',(21.065394928907,-64.1645003216707,27.3701136234318));
#33204=CARTESIAN_POINT('Ctrl Pts',(22.1199132331259,-65.8995346167871,27.2589805054402));
#33205=CARTESIAN_POINT('Ctrl Pts',(21.2342035166268,-67.726518783457,27.1478473874487));
#33206=CARTESIAN_POINT('Ctrl Pts',(19.2189021455725,-67.9733250072645,27.0367142694571));
#33207=CARTESIAN_POINT('Ctrl Pts',(17.9184923112052,-66.4140665093775,26.9255811514656));
#33208=CARTESIAN_POINT('Ctrl Pts',(18.5231601679997,-64.4758380560332,26.814448033474));
#33209=CARTESIAN_POINT('Ctrl Pts',(20.4794901123499,-63.9325825814632,26.7033149154825));
#33210=CARTESIAN_POINT('Ctrl Pts',(21.9969715433586,-65.2815089464938,26.5921817974909));
#33211=CARTESIAN_POINT('Ctrl Pts',(21.6867465959066,-67.288026512723,26.4810486794994));
#33212=CARTESIAN_POINT('Ctrl Pts',(19.832743621837,-68.1156916986943,26.3699155615077));
#33213=CARTESIAN_POINT('Ctrl Pts',(18.1318225653926,-67.0069922095504,26.2587824435162));
#33214=CARTESIAN_POINT('Ctrl Pts',(18.1407264484442,-64.9766545323691,26.1476493255247));
#33215=CARTESIAN_POINT('Ctrl Pts',(19.8513197951529,-63.8829214763781,26.0365162075331));
#33216=CARTESIAN_POINT('Ctrl Pts',(21.6979729188376,-64.7268248618362,25.9253830895415));
#33217=CARTESIAN_POINT('Ctrl Pts',(21.9906106740947,-66.7359825655211,25.81424997155));
#33218=CARTESIAN_POINT('Ctrl Pts',(20.4612908701142,-68.0715513800824,25.7031168535584));
#33219=CARTESIAN_POINT('Ctrl Pts',(18.5099236761208,-67.5111322639793,25.5919837355669));
#33220=CARTESIAN_POINT('Ctrl Pts',(17.9220455760523,-65.5677104225445,25.4808506175753));
#33221=CARTESIAN_POINT('Ctrl Pts',(19.2365661510841,-64.0198472713955,25.3697174995837));
#33222=CARTESIAN_POINT('Ctrl Pts',(21.2486684267406,-64.2844772327437,25.2585843815922));
#33223=CARTESIAN_POINT('Ctrl Pts',(22.1202283859708,-66.1188570886621,25.1474512636006));
#33224=CARTESIAN_POINT('Ctrl Pts',(21.0465924302418,-67.8452543356348,25.0363181456091));
#33225=CARTESIAN_POINT('Ctrl Pts',(19.6996852649167,-67.8682605606161,24.9622294002814));
#33226=CARTESIAN_POINT('Ctrl Pts',(19.1702141221325,-67.5923488637343,24.9251850276175));
#33227=CARTESIAN_POINT('Ctrl Pts',(19.5701357431141,-67.6095877486648,36.2244449171475));
#33228=CARTESIAN_POINT('Ctrl Pts',(19.0349325071232,-67.4666537946055,36.1874005444836));
#33229=CARTESIAN_POINT('Ctrl Pts',(18.127631598377,-66.6069908791351,36.1133117991559));
#33230=CARTESIAN_POINT('Ctrl Pts',(18.4746138026192,-64.7528842102888,36.0021786811644));
#33231=CARTESIAN_POINT('Ctrl Pts',(20.2203904348554,-64.0436664636898,35.8910455631728));
#33232=CARTESIAN_POINT('Ctrl Pts',(21.7631193309508,-65.1232793527361,35.7799124451812));
#33233=CARTESIAN_POINT('Ctrl Pts',(21.6928417986657,-67.0061404137184,35.6687793271897));
#33234=CARTESIAN_POINT('Ctrl Pts',(20.0728729391805,-67.9677217333163,35.5576462091981));
#33235=CARTESIAN_POINT('Ctrl Pts',(18.3863763801858,-67.1285775460602,35.4465130912066));
#33236=CARTESIAN_POINT('Ctrl Pts',(18.1766471536642,-65.256408990077,35.335379973215));
#33237=CARTESIAN_POINT('Ctrl Pts',(19.6357646146006,-64.0648572555519,35.2242468552234));
#33238=CARTESIAN_POINT('Ctrl Pts',(21.4282233691483,-64.6443977096884,35.1131137372319));
#33239=CARTESIAN_POINT('Ctrl Pts',(21.9135265503078,-66.4646520881558,35.0019806192403));
#33240=CARTESIAN_POINT('Ctrl Pts',(20.6474895653351,-67.8596318890753,34.8908475012488));
#33241=CARTESIAN_POINT('Ctrl Pts',(18.7888473297796,-67.5526067506278,34.7797143832572));
#33242=CARTESIAN_POINT('Ctrl Pts',(18.0386983418521,-65.8245731185539,34.6685812652657));
#33243=CARTESIAN_POINT('Ctrl Pts',(19.0836105030738,-64.2570979185908,34.5574481472741));
#33244=CARTESIAN_POINT('Ctrl Pts',(20.9672380617522,-64.2847948793711,34.4463150292825));
#33245=CARTESIAN_POINT('Ctrl Pts',(21.9656114461841,-65.8823152891195,34.335181911291));
#33246=CARTESIAN_POINT('Ctrl Pts',(21.1649797840838,-67.5875452715668,34.2240487932994));
#33247=CARTESIAN_POINT('Ctrl Pts',(19.2981128132078,-67.8397913898394,34.1129156753078));
#33248=CARTESIAN_POINT('Ctrl Pts',(18.0736406002369,-66.408187987792,34.0017825573163));
#33249=CARTESIAN_POINT('Ctrl Pts',(18.6122483414602,-64.6029948866662,33.8906494393248));
#33250=CARTESIAN_POINT('Ctrl Pts',(20.4209810165526,-64.0763958440913,33.7795163213331));
#33251=CARTESIAN_POINT('Ctrl Pts',(21.8444152983533,-65.3103550407155,33.6683832033416));
#33252=CARTESIAN_POINT('Ctrl Pts',(21.5797681022636,-67.1755044465377,33.55725008535));
#33253=CARTESIAN_POINT('Ctrl Pts',(19.8692549605973,-67.9647859163373,33.4461169673585));
#33254=CARTESIAN_POINT('Ctrl Pts',(18.278404824725,-66.9558179818571,33.3349838493669));
#33255=CARTESIAN_POINT('Ctrl Pts',(18.2632263547617,-65.0720478099667,33.2238507313754));
#33256=CARTESIAN_POINT('Ctrl Pts',(19.837611483579,-64.0375760061294,33.1127176133838));
#33257=CARTESIAN_POINT('Ctrl Pts',(21.5606209742177,-64.7991918817922,33.0015844953923));
#33258=CARTESIAN_POINT('Ctrl Pts',(21.8552887237877,-66.6598346105587,32.8904513774007));
#33259=CARTESIAN_POINT('Ctrl Pts',(20.4519232099055,-67.9165707329182,32.7793182594091));
#33260=CARTESIAN_POINT('Ctrl Pts',(18.6349397867881,-67.4191858850152,32.6681851414176));
#33261=CARTESIAN_POINT('Ctrl Pts',(18.0673131990514,-65.6229062565376,32.557052023426));
#33262=CARTESIAN_POINT('Ctrl Pts',(19.2685576413527,-64.1717576643402,32.4459189054344));
#33263=CARTESIAN_POINT('Ctrl Pts',(21.1392469195794,-64.3938884166567,32.3347857874429));
#33264=CARTESIAN_POINT('Ctrl Pts',(21.9672525766849,-66.0859957059843,32.2236526694513));
#33265=CARTESIAN_POINT('Ctrl Pts',(20.9947512453016,-67.6993963404374,32.1125195514598));
#33266=CARTESIAN_POINT('Ctrl Pts',(19.1118144211908,-67.757442556534,32.0013864334682));
#33267=CARTESIAN_POINT('Ctrl Pts',(18.0417799974499,-66.2070081726256,31.8902533154767));
#33268=CARTESIAN_POINT('Ctrl Pts',(18.7639855948311,-64.4671117613681,31.7791201974851));
#33269=CARTESIAN_POINT('Ctrl Pts',(20.6174402248758,-64.1301749999996,31.6679870794935));
#33270=CARTESIAN_POINT('Ctrl Pts',(21.9057892589038,-65.5045756742264,31.556853961502));
#33271=CARTESIAN_POINT('Ctrl Pts',(21.4498849520487,-67.3324081911126,31.4457208435104));
#33272=CARTESIAN_POINT('Ctrl Pts',(19.6669888701631,-67.9407682884172,31.3345877255189));
#33273=CARTESIAN_POINT('Ctrl Pts',(18.1888776814945,-66.7728608602669,31.2234546075273));
#33274=CARTESIAN_POINT('Ctrl Pts',(18.368376923802,-64.8976007532933,31.1123214895358));
#33275=CARTESIAN_POINT('Ctrl Pts',(20.0412018255044,-64.0312998269172,31.0011883715442));
#33276=CARTESIAN_POINT('Ctrl Pts',(21.6763171948171,-64.9668307862301,30.8900552535526));
#33277=CARTESIAN_POINT('Ctrl Pts',(21.7772010882313,-66.8479588751294,30.7789221355611));
#33278=CARTESIAN_POINT('Ctrl Pts',(20.2515205957431,-67.9530016261739,30.6677890175695));
#33279=CARTESIAN_POINT('Ctrl Pts',(18.4956385542766,-67.2705804195494,30.556655899578));
#33280=CARTESIAN_POINT('Ctrl Pts',(18.1166073190257,-65.425274003395,30.4455227815864));
#33281=CARTESIAN_POINT('Ctrl Pts',(19.4613311950161,-64.1059794403286,30.3343896635948));
#33282=CARTESIAN_POINT('Ctrl Pts',(21.2990659631253,-64.520167041396,30.2232565456033));
#33283=CARTESIAN_POINT('Ctrl Pts',(21.9478444310442,-66.2887560118356,30.1121234276117));
#33284=CARTESIAN_POINT('Ctrl Pts',(20.8138790092618,-67.7930641149174,30.0009903096202));
#33285=CARTESIAN_POINT('Ctrl Pts',(18.9350194842373,-67.6562893657108,29.8898571916286));
#33286=CARTESIAN_POINT('Ctrl Pts',(18.0308720444635,-66.0036133980917,29.778724073637));
#33287=CARTESIAN_POINT('Ctrl Pts',(18.9289480137178,-64.347630306317,29.6675909556455));
#33288=CARTESIAN_POINT('Ctrl Pts',(20.807292917013,-64.2039609948384,29.5564578376539));
#33289=CARTESIAN_POINT('Ctrl Pts',(21.9467715679183,-65.7040972722901,29.4453247196624));
#33290=CARTESIAN_POINT('Ctrl Pts',(21.3044882556826,-67.4750553727597,29.3341916016708));
#33291=CARTESIAN_POINT('Ctrl Pts',(19.4682859476888,-67.895984738466,29.2230584836793));
#33292=CARTESIAN_POINT('Ctrl Pts',(18.1187292684313,-66.581634246296,29.1119253656877));
#33293=CARTESIAN_POINT('Ctrl Pts',(18.4909856088001,-64.7349491990151,29.0007922476961));
#33294=CARTESIAN_POINT('Ctrl Pts',(20.2443513142224,-64.0460884367099,28.8896591297046));
#33295=CARTESIAN_POINT('Ctrl Pts',(21.774077079295,-65.1455244423375,28.778526011713));
#33296=CARTESIAN_POINT('Ctrl Pts',(21.6800976744022,-67.027010110168,28.6673928937214));
#33297=CARTESIAN_POINT('Ctrl Pts',(20.0484267498987,-67.9685357024486,28.5562597757299));
#33298=CARTESIAN_POINT('Ctrl Pts',(18.3724337578252,-67.1083799390385,28.4451266577383));
#33299=CARTESIAN_POINT('Ctrl Pts',(18.1860534509818,-65.2337912300098,28.3339935397468));
#33300=CARTESIAN_POINT('Ctrl Pts',(19.6598684220231,-64.060466944962,28.2228604217552));
#33301=CARTESIAN_POINT('Ctrl Pts',(21.4449852007115,-64.6622796511569,28.1117273037637));
#33302=CARTESIAN_POINT('Ctrl Pts',(21.9075946495772,-66.4884266727834,28.0005941857721));
#33303=CARTESIAN_POINT('Ctrl Pts',(20.6242983930922,-67.8675463791709,27.8894610677806));
#33304=CARTESIAN_POINT('Ctrl Pts',(18.7696196748325,-67.5374141334743,27.778327949789));
#33305=CARTESIAN_POINT('Ctrl Pts',(18.0410334580049,-65.8001799607068,27.6671948317975));
#33306=CARTESIAN_POINT('Ctrl Pts',(19.1053705235042,-64.2458289529094,27.5560617138058));
#33307=CARTESIAN_POINT('Ctrl Pts',(20.988507700316,-64.2969643305723,27.4449285958143));
#33308=CARTESIAN_POINT('Ctrl Pts',(21.9669237182277,-65.9067849843973,27.3337954778227));
#33309=CARTESIAN_POINT('Ctrl Pts',(21.1451337404002,-67.6019196880712,27.2226623598312));
#33310=CARTESIAN_POINT('Ctrl Pts',(19.2752722742974,-67.8309144449451,27.1115292418396));
#33311=CARTESIAN_POINT('Ctrl Pts',(18.0687101817244,-66.3841842323977,27.0003961238481));
#33312=CARTESIAN_POINT('Ctrl Pts',(18.6297404779621,-64.5858334996156,26.8892630058565));
#33313=CARTESIAN_POINT('Ctrl Pts',(20.4448863566203,-64.081783587906,26.7781298878649));
#33314=CARTESIAN_POINT('Ctrl Pts',(21.852854462098,-65.33336087893,26.6669967698734));
#33315=CARTESIAN_POINT('Ctrl Pts',(21.5650177725607,-67.195072448246,26.5558636518818));
#33316=CARTESIAN_POINT('Ctrl Pts',(19.844814149894,-67.9630068427298,26.4447305338903));
#33317=CARTESIAN_POINT('Ctrl Pts',(18.2666448567006,-66.9343197778498,26.3335974158987));
#33318=CARTESIAN_POINT('Ctrl Pts',(18.2749061659302,-65.0505071430419,26.2224642979072));
#33319=CARTESIAN_POINT('Ctrl Pts',(19.8620497212928,-64.0357064164734,26.1113311799156));
#33320=CARTESIAN_POINT('Ctrl Pts',(21.5754339162483,-64.8187071349992,26.000198061924));
#33321=CARTESIAN_POINT('Ctrl Pts',(21.846952642897,-66.6828683088086,25.8890649439325));
#33322=CARTESIAN_POINT('Ctrl Pts',(20.4280005140077,-67.9220520346501,25.7779318259409));
#33323=CARTESIAN_POINT('Ctrl Pts',(18.6174592348358,-67.4020771439864,25.6667987079494));
#33324=CARTESIAN_POINT('Ctrl Pts',(18.0720070151965,-65.5989078186063,25.5556655899578));
#33325=CARTESIAN_POINT('Ctrl Pts',(19.2916615070531,-64.162750575474,25.4445324719662));
#33326=CARTESIAN_POINT('Ctrl Pts',(21.1585547494963,-64.4082827696205,25.3333993539747));
#33327=CARTESIAN_POINT('Ctrl Pts',(21.9672161271791,-66.1102794317786,25.2222662359831));
#33328=CARTESIAN_POINT('Ctrl Pts',(20.9710621369748,-67.7120863543886,25.1111331179916));
#33329=CARTESIAN_POINT('Ctrl Pts',(19.7213583244171,-67.7334322702853,25.0370443726639));
#33330=CARTESIAN_POINT('Ctrl Pts',(19.2300979593295,-67.4774325188554,25.));
#33331=CARTESIAN_POINT('Ctrl Pts',(18.3361559831984,-65.999055845664,35.3785196366098));
#33332=CARTESIAN_POINT('Ctrl Pts',(18.3350370782603,-65.7833631823591,35.3641397488116));
#33333=CARTESIAN_POINT('Ctrl Pts',(18.3739569960147,-65.5680576617332,35.3497598610133));
#33334=CARTESIAN_POINT('Ctrl Pts',(18.4547882682405,-65.3698451269867,35.335379973215));
#33335=CARTESIAN_POINT('Ctrl Pts',(18.663019640643,-64.8592250785686,35.2983356005511));
#33336=CARTESIAN_POINT('Ctrl Pts',(19.1493921276218,-64.4620411670603,35.2612912278873));
#33337=CARTESIAN_POINT('Ctrl Pts',(19.6913214968691,-64.3600392869955,35.2242468552234));
#33338=CARTESIAN_POINT('Ctrl Pts',(20.2332508661165,-64.2580374069307,35.1872024825596));
#33339=CARTESIAN_POINT('Ctrl Pts',(20.8307371176324,-64.4512175583096,35.1501581098957));
#33340=CARTESIAN_POINT('Ctrl Pts',(21.2103641069169,-64.8511833637436,35.1131137372319));
#33341=CARTESIAN_POINT('Ctrl Pts',(21.5899910962014,-65.2511491691776,35.076069364568));
#33342=CARTESIAN_POINT('Ctrl Pts',(21.7517588232546,-65.8579006286667,35.0390249919042));
#33343=CARTESIAN_POINT('Ctrl Pts',(21.6216365226191,-66.3937729918978,35.0019806192403));
#33344=CARTESIAN_POINT('Ctrl Pts',(21.4915142219835,-66.929645355129,34.9649362465765));
#33345=CARTESIAN_POINT('Ctrl Pts',(21.0695018936593,-67.3946386221021,34.9278918739126));
#33346=CARTESIAN_POINT('Ctrl Pts',(20.5487220235713,-67.5759643991808,34.8908475012488));
#33347=CARTESIAN_POINT('Ctrl Pts',(20.0279421534833,-67.7572901762595,34.8538031285849));
#33348=CARTESIAN_POINT('Ctrl Pts',(19.4083947416314,-67.6549484634436,34.8167587559211));
#33349=CARTESIAN_POINT('Ctrl Pts',(18.9735962043843,-67.3157720016901,34.7797143832572));
#33350=CARTESIAN_POINT('Ctrl Pts',(18.5776806698023,-67.0069272870253,34.7459828010414));
#33351=CARTESIAN_POINT('Ctrl Pts',(18.3349481942213,-66.5017129251968,34.7122512188256));
#33352=CARTESIAN_POINT('Ctrl Pts',(18.3317911996431,-65.9991411289371,34.6785196366098));
#33353=CARTESIAN_POINT('Ctrl Pts',(19.4698297828114,-67.9851743256717,36.));
#33354=CARTESIAN_POINT('Ctrl Pts',(19.4011649893952,-67.9597502983812,36.));
#33355=CARTESIAN_POINT('Ctrl Pts',(19.3342035408141,-67.9304365939153,36.));
#33356=CARTESIAN_POINT('Ctrl Pts',(19.2691343741972,-67.8975272372444,36.));
#33357=CARTESIAN_POINT('Ctrl Pts',(19.2022542736866,-67.8637019833443,36.));
#33358=CARTESIAN_POINT('Ctrl Pts',(19.1373724771277,-67.8260774631159,36.));
#33359=CARTESIAN_POINT('Ctrl Pts',(19.0747253547554,-67.7849282947603,36.));
#33360=CARTESIAN_POINT('Ctrl Pts',(19.0217926342618,-67.7501599391738,36.));
#33361=CARTESIAN_POINT('Ctrl Pts',(18.9704556141999,-67.7128742354079,36.));
#33362=CARTESIAN_POINT('Ctrl Pts',(18.9208796153568,-67.6732188234994,36.));
#33363=CARTESIAN_POINT('Ctrl Pts',(18.8988499701712,-67.6555975011978,36.));
#33364=CARTESIAN_POINT('Ctrl Pts',(18.8771683538016,-67.6375080850151,36.));
#33365=CARTESIAN_POINT('Ctrl Pts',(18.8558508253114,-67.6189628052533,36.));
#33366=CARTESIAN_POINT('Ctrl Pts',(18.844138241103,-67.6087733899569,36.));
#33367=CARTESIAN_POINT('Ctrl Pts',(18.8325355847645,-67.5984463527787,36.));
#33368=CARTESIAN_POINT('Ctrl Pts',(18.8210456541305,-67.5879836806034,36.));
#33369=CARTESIAN_POINT('Ctrl Pts',(18.8104521112012,-67.5783372544957,36.));
#33370=CARTESIAN_POINT('Ctrl Pts',(18.7999529576494,-67.5685740155973,36.));
#33371=CARTESIAN_POINT('Ctrl Pts',(18.7895662739712,-67.5587109766458,36.));
#33372=CARTESIAN_POINT('Ctrl Pts',(18.736481497238,-67.5083024692848,36.));
#33373=CARTESIAN_POINT('Ctrl Pts',(18.6862367142759,-67.45520556261,36.));
#33374=CARTESIAN_POINT('Ctrl Pts',(18.6390505925823,-67.399679719805,36.));
#33375=CARTESIAN_POINT('Ctrl Pts',(18.5922306356017,-67.3445847580211,36.));
#33376=CARTESIAN_POINT('Ctrl Pts',(18.5484215452298,-67.2870975275965,36.));
#33377=CARTESIAN_POINT('Ctrl Pts',(18.507881729457,-67.2274472583178,36.));
#33378=CARTESIAN_POINT('Ctrl Pts',(18.4741932913828,-67.17787810354,36.));
#33379=CARTESIAN_POINT('Ctrl Pts',(18.442763110747,-67.1268145999806,36.));
#33380=CARTESIAN_POINT('Ctrl Pts',(18.4137670774186,-67.0743818157429,36.));
#33381=CARTESIAN_POINT('Ctrl Pts',(18.4016609056866,-67.0524905355397,36.));
#33382=CARTESIAN_POINT('Ctrl Pts',(18.3899793657611,-67.0303605291398,36.));
#33383=CARTESIAN_POINT('Ctrl Pts',(18.3787367001908,-67.0080008158944,36.));
#33384=CARTESIAN_POINT('Ctrl Pts',(18.3735358722236,-66.9976572704731,36.));
#33385=CARTESIAN_POINT('Ctrl Pts',(18.3684289741711,-66.987264568668,36.));
#33386=CARTESIAN_POINT('Ctrl Pts',(18.363417481184,-66.9768236053222,36.));
#33387=CARTESIAN_POINT('Ctrl Pts',(18.3581854927908,-66.9659232610176,36.));
#33388=CARTESIAN_POINT('Ctrl Pts',(18.3530610988599,-66.9549777676102,36.));
#33389=CARTESIAN_POINT('Ctrl Pts',(18.3480473578998,-66.9439924325212,36.));
#33390=CARTESIAN_POINT('Ctrl Pts',(18.3195069605931,-66.8814591204733,36.));
#33391=CARTESIAN_POINT('Ctrl Pts',(18.2945275345026,-66.8175927373651,36.));
#33392=CARTESIAN_POINT('Ctrl Pts',(18.2733325397259,-66.752597734286,36.));
#33393=CARTESIAN_POINT('Ctrl Pts',(18.2541300624259,-66.6937128379039,36.));
#33394=CARTESIAN_POINT('Ctrl Pts',(18.2380342438875,-66.6339009498019,36.));
#33395=CARTESIAN_POINT('Ctrl Pts',(18.2252479596501,-66.5733092869319,36.));
#33396=CARTESIAN_POINT('Ctrl Pts',(18.2101154548975,-66.5015993507748,36.));
#33397=CARTESIAN_POINT('Ctrl Pts',(18.1996178813496,-66.4287956961599,36.));
#33398=CARTESIAN_POINT('Ctrl Pts',(18.1936800996947,-66.3553214263371,36.));
#33399=CARTESIAN_POINT('Ctrl Pts',(18.1923732777051,-66.3391507759068,36.));
#33400=CARTESIAN_POINT('Ctrl Pts',(18.1912875458271,-66.3229477241296,36.));
#33401=CARTESIAN_POINT('Ctrl Pts',(18.1904224723119,-66.3067169458811,36.));
#33402=CARTESIAN_POINT('Ctrl Pts',(18.1895271437582,-66.2899185131946,36.));
#33403=CARTESIAN_POINT('Ctrl Pts',(18.1888681680866,-66.2730841862021,36.));
#33404=CARTESIAN_POINT('Ctrl Pts',(18.1884456276216,-66.256253422113,36.));
#33405=CARTESIAN_POINT('Ctrl Pts',(18.1867243886032,-66.1876924906622,36.));
#33406=CARTESIAN_POINT('Ctrl Pts',(18.1889147565045,-66.1191039788408,36.));
#33407=CARTESIAN_POINT('Ctrl Pts',(18.1948961467264,-66.0508262139634,36.));
#33408=CARTESIAN_POINT('Ctrl Pts',(18.2008763007651,-65.9825625601576,36.));
#33409=CARTESIAN_POINT('Ctrl Pts',(18.2106463639563,-65.9146084532637,36.));
#33410=CARTESIAN_POINT('Ctrl Pts',(18.2241354315071,-65.8473170438901,36.));
#33411=CARTESIAN_POINT('Ctrl Pts',(18.2338954237845,-65.7986284571252,36.));
#33412=CARTESIAN_POINT('Ctrl Pts',(18.2456034473503,-65.7502870727337,36.));
#33413=CARTESIAN_POINT('Ctrl Pts',(18.2592468469421,-65.7024363115996,36.));
#33414=CARTESIAN_POINT('Ctrl Pts',(18.2694831958018,-65.6665349161389,36.));
#33415=CARTESIAN_POINT('Ctrl Pts',(18.2808092514107,-65.630909856111,36.));
#33416=CARTESIAN_POINT('Ctrl Pts',(18.2932235838799,-65.5956258810508,36.));
#33417=CARTESIAN_POINT('Ctrl Pts',(18.297353127888,-65.5838889046042,36.));
#33418=CARTESIAN_POINT('Ctrl Pts',(18.3015998970195,-65.572198863249,36.));
#33419=CARTESIAN_POINT('Ctrl Pts',(18.3059632462308,-65.5605583181236,36.));
#33420=CARTESIAN_POINT('Ctrl Pts',(18.3290871983339,-65.4988682275758,36.));
#33421=CARTESIAN_POINT('Ctrl Pts',(18.3554837360288,-65.4385616710145,36.));
#33422=CARTESIAN_POINT('Ctrl Pts',(18.385102864326,-65.3799727413706,36.));
#33423=CARTESIAN_POINT('Ctrl Pts',(18.4059351916682,-65.338764784515,36.));
#33424=CARTESIAN_POINT('Ctrl Pts',(18.4283625495674,-65.2984070455804,36.));
#33425=CARTESIAN_POINT('Ctrl Pts',(18.4523779441861,-65.2590271139576,36.));
#33426=CARTESIAN_POINT('Ctrl Pts',(18.460090964352,-65.2463794680805,36.));
#33427=CARTESIAN_POINT('Ctrl Pts',(18.4679689477642,-65.233831076664,36.));
#33428=CARTESIAN_POINT('Ctrl Pts',(18.4760083383501,-65.2213918011997,36.));
#33429=CARTESIAN_POINT('Ctrl Pts',(18.5102528434667,-65.1684055918931,36.));
#33430=CARTESIAN_POINT('Ctrl Pts',(18.5473531093338,-65.1175031736617,36.));
#33431=CARTESIAN_POINT('Ctrl Pts',(18.5872748982222,-65.0689997700819,36.));
#33432=CARTESIAN_POINT('Ctrl Pts',(18.6240617329213,-65.0243052125604,36.));
#33433=CARTESIAN_POINT('Ctrl Pts',(18.6632449424928,-64.9816475926941,36.));
#33434=CARTESIAN_POINT('Ctrl Pts',(18.7048191776161,-64.9413064478025,36.));
#33435=CARTESIAN_POINT('Ctrl Pts',(18.7126375272136,-64.9337199901564,36.));
#33436=CARTESIAN_POINT('Ctrl Pts',(18.7205404900226,-64.9262155594354,36.));
#33437=CARTESIAN_POINT('Ctrl Pts',(18.7285264739143,-64.9187938215857,36.));
#33438=CARTESIAN_POINT('Origin',(20.,-66.,30.));
#33439=CARTESIAN_POINT('Origin',(-20.,-66.,25.));
#33440=CARTESIAN_POINT('Ctrl Pts',(-20.7699020406704,-67.4774325188554,
25.));
#33441=CARTESIAN_POINT('Ctrl Pts',(-20.7181608035629,-67.5125051433483,
25.));
#33442=CARTESIAN_POINT('Ctrl Pts',(-20.6644430822213,-67.5443226803472,
25.));
#33443=CARTESIAN_POINT('Ctrl Pts',(-20.6090801759931,-67.5729491720382,
25.));
#33444=CARTESIAN_POINT('Ctrl Pts',(-20.5739700098743,-67.5911035816807,
25.));
#33445=CARTESIAN_POINT('Ctrl Pts',(-20.5381972786393,-67.6079739470072,
25.));
#33446=CARTESIAN_POINT('Ctrl Pts',(-20.5018388806471,-67.6235693893572,
25.));
#33447=CARTESIAN_POINT('Ctrl Pts',(-20.477053808413,-67.6342006103821,25.));
#33448=CARTESIAN_POINT('Ctrl Pts',(-20.4519964598586,-67.6442392598381,
25.));
#33449=CARTESIAN_POINT('Ctrl Pts',(-20.4266899529795,-67.6536866428541,
25.));
#33450=CARTESIAN_POINT('Ctrl Pts',(-20.413200618616,-67.6587224587006,25.));
#33451=CARTESIAN_POINT('Ctrl Pts',(-20.3996405377501,-67.6635901036932,
25.));
#33452=CARTESIAN_POINT('Ctrl Pts',(-20.386026916268,-67.6682852533056,25.));
#33453=CARTESIAN_POINT('Ctrl Pts',(-20.3236625333886,-67.6897938657264,
25.));
#33454=CARTESIAN_POINT('Ctrl Pts',(-20.2601068487493,-67.7077128062917,
25.));
#33455=CARTESIAN_POINT('Ctrl Pts',(-20.1957097546859,-67.7220886184591,
25.));
#33456=CARTESIAN_POINT('Ctrl Pts',(-20.1492572977333,-67.7324585242068,
25.));
#33457=CARTESIAN_POINT('Ctrl Pts',(-20.1023661244431,-67.7409839821677,
25.));
#33458=CARTESIAN_POINT('Ctrl Pts',(-20.0551584518849,-67.7476684316844,
25.));
#33459=CARTESIAN_POINT('Ctrl Pts',(-20.0422593587017,-67.7494949004027,
25.));
#33460=CARTESIAN_POINT('Ctrl Pts',(-20.0293366022274,-67.7511838474356,
25.));
#33461=CARTESIAN_POINT('Ctrl Pts',(-20.0163926091019,-67.7527351822321,
25.));
#33462=CARTESIAN_POINT('Ctrl Pts',(-20.0030616559028,-67.7543328941104,
25.));
#33463=CARTESIAN_POINT('Ctrl Pts',(-19.9897160980323,-67.7557836532261,
25.));
#33464=CARTESIAN_POINT('Ctrl Pts',(-19.9763641937448,-67.7570873827579,
25.));
#33465=CARTESIAN_POINT('Ctrl Pts',(-19.9088330185891,-67.7636813775523,
25.));
#33466=CARTESIAN_POINT('Ctrl Pts',(-19.8410981608417,-67.7665229814955,
25.));
#33467=CARTESIAN_POINT('Ctrl Pts',(-19.7735142959518,-67.7656601451573,
25.));
#33468=CARTESIAN_POINT('Ctrl Pts',(-19.704951841588,-67.7647848152668,25.));
#33469=CARTESIAN_POINT('Ctrl Pts',(-19.63654377446,-67.7600973242924,25.));
#33470=CARTESIAN_POINT('Ctrl Pts',(-19.5686389092575,-67.7515994414432,
25.));
#33471=CARTESIAN_POINT('Ctrl Pts',(-19.5265710026273,-67.7463348975672,
25.));
#33472=CARTESIAN_POINT('Ctrl Pts',(-19.4846958553342,-67.7396069714499,
25.));
#33473=CARTESIAN_POINT('Ctrl Pts',(-19.4430950268279,-67.7314061394558,
25.));
#33474=CARTESIAN_POINT('Ctrl Pts',(-19.4090314673628,-67.7246911403001,
25.));
#33475=CARTESIAN_POINT('Ctrl Pts',(-19.3751517890293,-67.716988473764,25.));
#33476=CARTESIAN_POINT('Ctrl Pts',(-19.3415011106365,-67.7082889292452,
25.));
#33477=CARTESIAN_POINT('Ctrl Pts',(-19.3277178592572,-67.7047256129997,
25.));
#33478=CARTESIAN_POINT('Ctrl Pts',(-19.3139705632122,-67.7009941660984,
25.));
#33479=CARTESIAN_POINT('Ctrl Pts',(-19.3002855806312,-67.6971007967711,
25.));
#33480=CARTESIAN_POINT('Ctrl Pts',(-19.232490274151,-67.6778130727844,25.));
#33481=CARTESIAN_POINT('Ctrl Pts',(-19.1661045678635,-67.6545261552985,
25.));
#33482=CARTESIAN_POINT('Ctrl Pts',(-19.1014911923583,-67.6272587556,25.));
#33483=CARTESIAN_POINT('Ctrl Pts',(-19.0943244150679,-67.6242343139979,
25.));
#33484=CARTESIAN_POINT('Ctrl Pts',(-19.0871794343997,-67.6211608492454,
25.));
#33485=CARTESIAN_POINT('Ctrl Pts',(-19.0800567411892,-67.6180383475084,
25.));
#33486=CARTESIAN_POINT('Ctrl Pts',(-19.0183041427041,-67.5909667623182,
25.));
#33487=CARTESIAN_POINT('Ctrl Pts',(-18.958225984176,-67.5602135819053,25.));
#33488=CARTESIAN_POINT('Ctrl Pts',(-18.8999642015444,-67.5260890069827,
25.));
#33489=CARTESIAN_POINT('Ctrl Pts',(-18.8372883233669,-67.489379047141,25.));
#33490=CARTESIAN_POINT('Ctrl Pts',(-18.7767134702701,-67.4487674765275,
25.));
#33491=CARTESIAN_POINT('Ctrl Pts',(-18.7184362286254,-67.404579398372,25.));
#33492=CARTESIAN_POINT('Ctrl Pts',(-18.7079109252492,-67.3965987027338,
25.));
#33493=CARTESIAN_POINT('Ctrl Pts',(-18.69746064122,-67.3885011964254,25.));
#33494=CARTESIAN_POINT('Ctrl Pts',(-18.6870866397008,-67.3802886058017,
25.));
#33495=CARTESIAN_POINT('Ctrl Pts',(-18.6779106450409,-67.3730244187311,
25.));
#33496=CARTESIAN_POINT('Ctrl Pts',(-18.6688013314437,-67.3656757127138,
25.));
#33497=CARTESIAN_POINT('Ctrl Pts',(-18.6597613497716,-67.3582457843923,
25.));
#33498=CARTESIAN_POINT('Ctrl Pts',(-18.6048581342928,-67.3131210296724,
25.));
#33499=CARTESIAN_POINT('Ctrl Pts',(-18.5524870449414,-67.2649855309608,
25.));
#33500=CARTESIAN_POINT('Ctrl Pts',(-18.5027980990966,-67.2141892911126,
25.));
#33501=CARTESIAN_POINT('Ctrl Pts',(-18.4520613983228,-67.1623219476261,
25.));
#33502=CARTESIAN_POINT('Ctrl Pts',(-18.404120381723,-67.1076799285913,25.));
#33503=CARTESIAN_POINT('Ctrl Pts',(-18.3591549660204,-67.0505845582255,
25.));
#33504=CARTESIAN_POINT('Ctrl Pts',(-18.3139167893624,-66.9931428463985,
25.));
#33505=CARTESIAN_POINT('Ctrl Pts',(-18.2716896355437,-66.9332171999082,
25.));
#33506=CARTESIAN_POINT('Ctrl Pts',(-18.2326886678192,-66.8710932841069,
25.));
#33507=CARTESIAN_POINT('Ctrl Pts',(-18.2230616236579,-66.8557585445919,
25.));
#33508=CARTESIAN_POINT('Ctrl Pts',(-18.21363133674,-66.8402896962556,25.));
#33509=CARTESIAN_POINT('Ctrl Pts',(-18.2044014277785,-66.8246907301826,
25.));
#33510=CARTESIAN_POINT('Ctrl Pts',(-18.1971517956968,-66.8124385221321,
25.));
#33511=CARTESIAN_POINT('Ctrl Pts',(-18.1900250445996,-66.8001044895158,
25.));
#33512=CARTESIAN_POINT('Ctrl Pts',(-18.1830333944425,-66.7877096451503,
25.));
#33513=CARTESIAN_POINT('Ctrl Pts',(-18.1460181911873,-66.7220888441667,
25.));
#33514=CARTESIAN_POINT('Ctrl Pts',(-18.1127170684062,-66.6546510927272,
25.));
#33515=CARTESIAN_POINT('Ctrl Pts',(-18.0833107587068,-66.5857427136206,
25.));
#33516=CARTESIAN_POINT('Ctrl Pts',(-18.0538723748317,-66.5167591744726,
25.));
#33517=CARTESIAN_POINT('Ctrl Pts',(-18.0283365400255,-66.4463009685666,
25.));
#33518=CARTESIAN_POINT('Ctrl Pts',(-18.0069203162448,-66.3746778418095,
25.));
#33519=CARTESIAN_POINT('Ctrl Pts',(-17.9859913237923,-66.3046841821113,
25.));
#33520=CARTESIAN_POINT('Ctrl Pts',(-17.968996070436,-66.2335771265626,25.));
#33521=CARTESIAN_POINT('Ctrl Pts',(-17.956180742014,-66.1616225466294,25.));
#33522=CARTESIAN_POINT('Ctrl Pts',(-17.9534318997022,-66.1461885454602,
25.));
#33523=CARTESIAN_POINT('Ctrl Pts',(-17.9508755507278,-66.1307154913356,
25.));
#33524=CARTESIAN_POINT('Ctrl Pts',(-17.9485144323922,-66.1152059238131,
25.));
#33525=CARTESIAN_POINT('Ctrl Pts',(-17.94650124174,-66.101981802054,25.));
#33526=CARTESIAN_POINT('Ctrl Pts',(-17.9446299860387,-66.0887311345142,
25.));
#33527=CARTESIAN_POINT('Ctrl Pts',(-17.9428998377409,-66.0754556195432,
25.));
#33528=CARTESIAN_POINT('Ctrl Pts',(-18.1825721112406,-65.0413794120407,
25.));
#33529=CARTESIAN_POINT('Ctrl Pts',(-18.2234186022369,-64.9788996288608,
25.));
#33530=CARTESIAN_POINT('Ctrl Pts',(-18.2678617752615,-64.9189705657672,
25.));
#33531=CARTESIAN_POINT('Ctrl Pts',(-18.3155727832729,-64.8617419967287,
25.));
#33532=CARTESIAN_POINT('Ctrl Pts',(-18.3620323341325,-64.8060145299515,
25.));
#33533=CARTESIAN_POINT('Ctrl Pts',(-18.4115915340684,-64.7528475406059,
25.));
#33534=CARTESIAN_POINT('Ctrl Pts',(-18.4639728032933,-64.7024169935917,
25.));
#33535=CARTESIAN_POINT('Ctrl Pts',(-18.4756644727561,-64.6911607316637,
25.));
#33536=CARTESIAN_POINT('Ctrl Pts',(-18.4874984029645,-64.6800395001903,
25.));
#33537=CARTESIAN_POINT('Ctrl Pts',(-18.4994665220206,-64.6690601964525,
25.));
#33538=CARTESIAN_POINT('Ctrl Pts',(-18.5543876810387,-64.6186766663706,
25.));
#33539=CARTESIAN_POINT('Ctrl Pts',(-18.6120225665561,-64.5713776148131,
25.));
#33540=CARTESIAN_POINT('Ctrl Pts',(-18.6720550336875,-64.5273355298405,
25.));
#33541=CARTESIAN_POINT('Ctrl Pts',(-18.7141995014743,-64.4964167567151,
25.));
#33542=CARTESIAN_POINT('Ctrl Pts',(-18.7575262835589,-64.4671040519447,
25.));
#33543=CARTESIAN_POINT('Ctrl Pts',(-18.8019313225172,-64.4394714970494,
25.));
#33544=CARTESIAN_POINT('Ctrl Pts',(-18.8188067446915,-64.4289701881765,
25.));
#33545=CARTESIAN_POINT('Ctrl Pts',(-18.8358379234656,-64.4187116654628,
25.));
#33546=CARTESIAN_POINT('Ctrl Pts',(-18.853019222819,-64.4087004822027,25.));
#33547=CARTESIAN_POINT('Ctrl Pts',(-18.8694039161204,-64.3991534646037,
25.));
#33548=CARTESIAN_POINT('Ctrl Pts',(-18.8859304480109,-64.3898286464703,
25.));
#33549=CARTESIAN_POINT('Ctrl Pts',(-18.9025643388043,-64.3807458845255,
25.));
#33550=CARTESIAN_POINT('Ctrl Pts',(-18.9662812680801,-64.3459539222805,
25.));
#33551=CARTESIAN_POINT('Ctrl Pts',(-19.0316371535594,-64.3146691113732,
25.));
#33552=CARTESIAN_POINT('Ctrl Pts',(-19.0983402957666,-64.2870530879642,
25.));
#33553=CARTESIAN_POINT('Ctrl Pts',(-19.1636110961765,-64.2600300738692,
25.));
#33554=CARTESIAN_POINT('Ctrl Pts',(-19.2301728387105,-64.2365198225598,
25.));
#33555=CARTESIAN_POINT('Ctrl Pts',(-19.2977608179252,-64.216722038388,25.));
#33556=CARTESIAN_POINT('Ctrl Pts',(-19.3638664769608,-64.1973584535415,
25.));
#33557=CARTESIAN_POINT('Ctrl Pts',(-19.4309546138826,-64.1815461688934,
25.));
#33558=CARTESIAN_POINT('Ctrl Pts',(-19.4987736270454,-64.1695206205673,
25.));
#33559=CARTESIAN_POINT('Ctrl Pts',(-19.5208338248684,-64.1656089450263,
25.));
#33560=CARTESIAN_POINT('Ctrl Pts',(-19.5429712759434,-64.162098331058,25.));
#33561=CARTESIAN_POINT('Ctrl Pts',(-19.5651770267509,-64.1589980551018,
25.));
#33562=CARTESIAN_POINT('Ctrl Pts',(-19.5776615166783,-64.1572550217641,
25.));
#33563=CARTESIAN_POINT('Ctrl Pts',(-19.5901688804906,-64.155641648664,25.));
#33564=CARTESIAN_POINT('Ctrl Pts',(-19.6026798229647,-64.1541614637293,
25.));
#33565=CARTESIAN_POINT('Ctrl Pts',(-19.6705104535392,-64.1461363387077,
25.));
#33566=CARTESIAN_POINT('Ctrl Pts',(-19.7385646210674,-64.1420044342446,
25.));
#33567=CARTESIAN_POINT('Ctrl Pts',(-19.8065966031785,-64.1419437913522,
25.));
#33568=CARTESIAN_POINT('Ctrl Pts',(-19.8163935407639,-64.1419350584796,
25.));
#33569=CARTESIAN_POINT('Ctrl Pts',(-19.8261900120765,-64.1420108411578,
25.));
#33570=CARTESIAN_POINT('Ctrl Pts',(-19.8359852738992,-64.1421717610483,
25.));
#33571=CARTESIAN_POINT('Ctrl Pts',(-19.9053495120193,-64.1433113003285,
25.));
#33572=CARTESIAN_POINT('Ctrl Pts',(-19.9746545558373,-64.1487161231621,
25.));
#33573=CARTESIAN_POINT('Ctrl Pts',(-20.0435753974168,-64.1582130010768,
25.));
#33574=CARTESIAN_POINT('Ctrl Pts',(-20.107870675276,-64.1670725040998,25.));
#33575=CARTESIAN_POINT('Ctrl Pts',(-20.1718321045596,-64.1794941475947,
25.));
#33576=CARTESIAN_POINT('Ctrl Pts',(-20.2351753108018,-64.1953717359853,
25.));
#33577=CARTESIAN_POINT('Ctrl Pts',(-20.2490399437352,-64.1988470405675,
25.));
#33578=CARTESIAN_POINT('Ctrl Pts',(-20.2628748598245,-64.2024880266852,
25.));
#33579=CARTESIAN_POINT('Ctrl Pts',(-20.2766768992135,-64.2062937588479,
25.));
#33580=CARTESIAN_POINT('Ctrl Pts',(-20.2877373262727,-64.209343527205,25.));
#33581=CARTESIAN_POINT('Ctrl Pts',(-20.298776094781,-64.2124990316602,25.));
#33582=CARTESIAN_POINT('Ctrl Pts',(-20.309778523466,-64.2157556651497,25.));
#33583=CARTESIAN_POINT('Ctrl Pts',(-20.3753407640279,-64.2351615794598,
25.));
#33584=CARTESIAN_POINT('Ctrl Pts',(-20.4397366338522,-64.2581874947932,
25.));
#33585=CARTESIAN_POINT('Ctrl Pts',(-20.5026636727024,-64.2846513912406,
25.));
#33586=CARTESIAN_POINT('Ctrl Pts',(-20.5652993520049,-64.3109927567531,
25.));
#33587=CARTESIAN_POINT('Ctrl Pts',(-20.6264806629052,-64.3407410428595,
25.));
#33588=CARTESIAN_POINT('Ctrl Pts',(-20.6858795340413,-64.3737582968461,
25.));
#33589=CARTESIAN_POINT('Ctrl Pts',(-20.744005682146,-64.4060680993479,25.));
#33590=CARTESIAN_POINT('Ctrl Pts',(-20.800425628206,-64.4415089864798,25.));
#33591=CARTESIAN_POINT('Ctrl Pts',(-20.8547920034067,-64.4799810839263,
25.));
#33592=CARTESIAN_POINT('Ctrl Pts',(-20.8662884771014,-64.4881165068719,
25.));
#33593=CARTESIAN_POINT('Ctrl Pts',(-20.8776929569316,-64.4963875608038,
25.));
#33594=CARTESIAN_POINT('Ctrl Pts',(-20.8890018799099,-64.5047934300188,
25.));
#33595=CARTESIAN_POINT('Ctrl Pts',(-20.8996330286824,-64.5126955128571,
25.));
#33596=CARTESIAN_POINT('Ctrl Pts',(-20.9101809631529,-64.5207178472751,
25.));
#33597=CARTESIAN_POINT('Ctrl Pts',(-20.9206261440524,-64.5288464944984,
25.));
#33598=CARTESIAN_POINT('Ctrl Pts',(-20.9721935855059,-64.5689773015968,
25.));
#33599=CARTESIAN_POINT('Ctrl Pts',(-21.0213544520126,-64.6117655949196,
25.));
#33600=CARTESIAN_POINT('Ctrl Pts',(-21.067817662843,-64.6570793623473,25.));
#33601=CARTESIAN_POINT('Ctrl Pts',(-21.1133972238304,-64.7015313403558,
25.));
#33602=CARTESIAN_POINT('Ctrl Pts',(-21.1563813453372,-64.7484143078876,
25.));
#33603=CARTESIAN_POINT('Ctrl Pts',(-21.1964527232528,-64.7976294036877,
25.));
#33604=CARTESIAN_POINT('Ctrl Pts',(-21.2352229728486,-64.8452464722117,
25.));
#33605=CARTESIAN_POINT('Ctrl Pts',(-21.2712669040832,-64.8950472509739,
25.));
#33606=CARTESIAN_POINT('Ctrl Pts',(-21.3042504633418,-64.9469575622361,
25.));
#33607=CARTESIAN_POINT('Ctrl Pts',(-21.3097028197845,-64.9555386106862,
25.));
#33608=CARTESIAN_POINT('Ctrl Pts',(-21.3150714360615,-64.9641773281828,
25.));
#33609=CARTESIAN_POINT('Ctrl Pts',(-21.3203546654043,-64.9728734055941,
25.));
#33610=CARTESIAN_POINT('Ctrl Pts',(-21.3260102500976,-64.9821823715897,
25.));
#33611=CARTESIAN_POINT('Ctrl Pts',(-21.3315679871567,-64.9915570687347,
25.));
#33612=CARTESIAN_POINT('Ctrl Pts',(-21.3370274731509,-65.0009958365548,
25.));
#33613=CARTESIAN_POINT('Origin',(-20.,-66.,37.5459252805377));
#33614=CARTESIAN_POINT('Ctrl Pts',(-22.0565720193282,-65.9985037223956,
35.7959252805377));
#33615=CARTESIAN_POINT('Ctrl Pts',(-22.0573889661773,-65.9003307564159,
35.7905876687522));
#33616=CARTESIAN_POINT('Ctrl Pts',(-22.0063638909344,-65.1216410352954,
35.7482056843029));
#33617=CARTESIAN_POINT('Ctrl Pts',(-21.0114092448251,-63.7918186839967,
35.6687793271897));
#33618=CARTESIAN_POINT('Ctrl Pts',(-18.6935440716095,-63.9528112405962,
35.5576462091981));
#33619=CARTESIAN_POINT('Ctrl Pts',(-17.5714219214042,-65.9871397838458,
35.4465130912065));
#33620=CARTESIAN_POINT('Ctrl Pts',(-18.6720184117364,-68.0334048867885,
35.335379973215));
#33621=CARTESIAN_POINT('Ctrl Pts',(-20.9880417410518,-68.218534353231,35.2242468552234));
#33622=CARTESIAN_POINT('Ctrl Pts',(-22.0019739647035,-66.8931862309832,
35.144428624331));
#33623=CARTESIAN_POINT('Ctrl Pts',(-22.0572805505537,-66.1070372200823,
35.1016547661024));
#33624=CARTESIAN_POINT('Ctrl Pts',(-22.0563749241962,-66.0016062120012,
35.0959252805377));
#33625=CARTESIAN_POINT('Ctrl Pts',(-22.0526726878338,-66.0023207051531,
35.8540747194623));
#33626=CARTESIAN_POINT('Ctrl Pts',(-22.0491245215623,-65.5321720585535,
35.8286277343138));
#33627=CARTESIAN_POINT('Ctrl Pts',(-21.656632320464,-64.370597952911,35.7661363765015));
#33628=CARTESIAN_POINT('Ctrl Pts',(-19.7281828815708,-63.5871681688473,
35.6666006460254));
#33629=CARTESIAN_POINT('Ctrl Pts',(-17.825468300226,-64.9187027300962,35.5554675280337));
#33630=CARTESIAN_POINT('Ctrl Pts',(-17.9121446998427,-67.2409164611445,
35.4443344100422));
#33631=CARTESIAN_POINT('Ctrl Pts',(-19.9101226099192,-68.4268768260922,
35.3332012920507));
#33632=CARTESIAN_POINT('Ctrl Pts',(-21.7210101198393,-67.525839720907,35.2364480618573));
#33633=CARTESIAN_POINT('Ctrl Pts',(-22.0499160744514,-66.4181209330382,
35.1767392043279));
#33634=CARTESIAN_POINT('Ctrl Pts',(-22.0520911128174,-65.9988355264336,
35.1540747194623));
#33635=CARTESIAN_POINT('Ctrl Pts',(-18.7309291201477,-64.9206413469514,
36.));
#33636=CARTESIAN_POINT('Ctrl Pts',(-18.372032101712,-65.3426194852432,35.9629556273362));
#33637=CARTESIAN_POINT('Ctrl Pts',(-18.1147588818617,-66.5657419043161,
35.8888668820084));
#33638=CARTESIAN_POINT('Ctrl Pts',(-19.4547380737757,-67.893353926766,35.7777337640169));
#33639=CARTESIAN_POINT('Ctrl Pts',(-21.2940072704514,-67.4836982885462,
35.6666006460253));
#33640=CARTESIAN_POINT('Ctrl Pts',(-21.9488058964948,-65.7182472190985,
35.5554675280338));
#33641=CARTESIAN_POINT('Ctrl Pts',(-20.8200548981038,-64.2095972393422,
35.4443344100422));
#33642=CARTESIAN_POINT('Ctrl Pts',(-18.9407200016067,-64.3401306858903,
35.3332012920506));
#33643=CARTESIAN_POINT('Ctrl Pts',(-18.0308986110522,-65.9895728822909,
35.2220681740591));
#33644=CARTESIAN_POINT('Ctrl Pts',(-18.92326690544,-67.648693291831,35.1109350560675));
#33645=CARTESIAN_POINT('Ctrl Pts',(-20.8011084271042,-67.7987970470776,
34.999801938076));
#33646=CARTESIAN_POINT('Ctrl Pts',(-21.9457416179595,-66.3026048808017,
34.8886688200844));
#33647=CARTESIAN_POINT('Ctrl Pts',(-21.309556683593,-64.5294397965287,34.7775357020928));
#33648=CARTESIAN_POINT('Ctrl Pts',(-19.47481333332,-64.1021978279347,34.6664025841013));
#33649=CARTESIAN_POINT('Ctrl Pts',(-18.12074179018,-65.4118948223318,34.5552694661097));
#33650=CARTESIAN_POINT('Ctrl Pts',(-18.4866411777649,-67.2598509704003,
34.4441363481182));
#33651=CARTESIAN_POINT('Ctrl Pts',(-20.2376261998072,-67.9547408460341,
34.3330032301266));
#33652=CARTESIAN_POINT('Ctrl Pts',(-21.7711263332307,-66.8605755017373,
34.2218701121351));
#33653=CARTESIAN_POINT('Ctrl Pts',(-21.6836219545264,-64.9787773153848,
34.1107369941435));
#33654=CARTESIAN_POINT('Ctrl Pts',(-20.0552004868468,-64.0316424608183,
33.999603876152));
#33655=CARTESIAN_POINT('Ctrl Pts',(-18.3762573656889,-64.886025831751,33.8884707581604));
#33656=CARTESIAN_POINT('Ctrl Pts',(-18.1834274109556,-66.7599622412461,
33.7773376401689));
#33657=CARTESIAN_POINT('Ctrl Pts',(-19.6531961905118,-67.9383512785846,
33.6662045221772));
#33658=CARTESIAN_POINT('Ctrl Pts',(-21.4403734659769,-67.3426849415994,
33.5550714041857));
#33659=CARTESIAN_POINT('Ctrl Pts',(-21.9092642531335,-65.5181404941846,
33.4439382861941));
#33660=CARTESIAN_POINT('Ctrl Pts',(-20.6307212477628,-64.134612834461,33.3328051682026));
#33661=CARTESIAN_POINT('Ctrl Pts',(-18.7749173315688,-64.4583609284768,
33.221672050211));
#33662=CARTESIAN_POINT('Ctrl Pts',(-18.0403572922691,-66.1930777796175,
33.1105389322195));
#33663=CARTESIAN_POINT('Ctrl Pts',(-19.0993393898891,-67.751082247112,32.9994058142279));
#33664=CARTESIAN_POINT('Ctrl Pts',(-20.9826415275293,-67.7064273202608,
32.8882726962363));
#33665=CARTESIAN_POINT('Ctrl Pts',(-21.9665914627858,-66.0999829455134,
32.7771395782448));
#33666=CARTESIAN_POINT('Ctrl Pts',(-21.1506394870126,-64.4020302437763,
32.6660064602533));
#33667=CARTESIAN_POINT('Ctrl Pts',(-19.2815769639979,-64.1666023583945,
32.5548733422617));
#33668=CARTESIAN_POINT('Ctrl Pts',(-18.0700434803867,-65.6091721564467,
32.4437402242701));
#33669=CARTESIAN_POINT('Ctrl Pts',(-18.6248821658744,-67.4094429797487,
32.3326071062786));
#33670=CARTESIAN_POINT('Ctrl Pts',(-20.4382828172642,-67.9197361128516,
32.221473988287));
#33671=CARTESIAN_POINT('Ctrl Pts',(-21.8505497836503,-66.6730111953947,
32.1103408702955));
#33672=CARTESIAN_POINT('Ctrl Pts',(-21.5691207511098,-64.8103199424505,
31.9992077523039));
#33673=CARTESIAN_POINT('Ctrl Pts',(-19.8515706471628,-64.0364707035261,
31.8880746343123));
#33674=CARTESIAN_POINT('Ctrl Pts',(-18.2698689290547,-65.0597207604948,
31.7769415163207));
#33675=CARTESIAN_POINT('Ctrl Pts',(-18.2716512643712,-66.9435513864888,
31.6658083983292));
#33676=CARTESIAN_POINT('Ctrl Pts',(-19.8552863896784,-67.9638066457476,
31.5546752803376));
#33677=CARTESIAN_POINT('Ctrl Pts',(-21.5713691070242,-67.1867087681419,
31.4435421623461));
#33678=CARTESIAN_POINT('Ctrl Pts',(-21.8492729691361,-65.3234883175307,
31.3324090443545));
#33679=CARTESIAN_POINT('Ctrl Pts',(-20.4346494232198,-64.0794379859558,
31.221275926363));
#33680=CARTESIAN_POINT('Ctrl Pts',(-18.6222176175382,-64.5931616022184,
31.1101428083714));
#33681=CARTESIAN_POINT('Ctrl Pts',(-18.0707864772717,-66.3944790927504,
30.9990096903798));
#33682=CARTESIAN_POINT('Ctrl Pts',(-19.2850474861105,-67.8347537910515,
30.8878765723883));
#33683=CARTESIAN_POINT('Ctrl Pts',(-21.1536611759177,-67.5957896045767,
30.7767434543967));
#33684=CARTESIAN_POINT('Ctrl Pts',(-21.9663987498635,-65.8962959623265,
30.6656103364051));
#33685=CARTESIAN_POINT('Ctrl Pts',(-20.9794107912338,-64.2917163371063,
30.5544772184136));
#33686=CARTESIAN_POINT('Ctrl Pts',(-19.0960275272337,-64.2506251575561,
30.443344100422));
#33687=CARTESIAN_POINT('Ctrl Pts',(-18.0399954503192,-65.8106306885334,
30.3322109824305));
#33688=CARTESIAN_POINT('Ctrl Pts',(-18.7778366822999,-67.5439544668685,
30.2210778644389));
#33689=CARTESIAN_POINT('Ctrl Pts',(-20.6342498865192,-67.8641903476697,
30.1099447464474));
#33690=CARTESIAN_POINT('Ctrl Pts',(-21.9101726307638,-66.4782458484667,
29.9988116284558));
#33691=CARTESIAN_POINT('Ctrl Pts',(-21.4378301996713,-64.6545919251736,
29.8876785104643));
#33692=CARTESIAN_POINT('Ctrl Pts',(-19.6495289773944,-64.0623084267076,
29.7765453924727));
#33693=CARTESIAN_POINT('Ctrl Pts',(-18.1819926294112,-65.2434765229158,
29.6654122744811));
#33694=CARTESIAN_POINT('Ctrl Pts',(-18.3783681830636,-67.1170446818255,
29.5542791564896));
#33695=CARTESIAN_POINT('Ctrl Pts',(-20.0589250023826,-67.9682495814781,
29.443146038498));
#33696=CARTESIAN_POINT('Ctrl Pts',(-21.6855513402555,-67.0180349946135,
29.3320129205065));
#33697=CARTESIAN_POINT('Ctrl Pts',(-21.7694947488723,-65.1360747112116,
29.2208798025149));
#33698=CARTESIAN_POINT('Ctrl Pts',(-20.2339269166865,-64.0448128558769,
29.1097466845233));
#33699=CARTESIAN_POINT('Ctrl Pts',(-18.4842599630755,-64.7430152302597,
28.9986135665318));
#33700=CARTESIAN_POINT('Ctrl Pts',(-18.1218579502043,-66.5916595403474,
28.8874804485402));
#33701=CARTESIAN_POINT('Ctrl Pts',(-19.4784054642569,-67.8987937516163,
28.7763473305487));
#33702=CARTESIAN_POINT('Ctrl Pts',(-21.3123368271822,-67.4680771856126,
28.6652142125571));
#33703=CARTESIAN_POINT('Ctrl Pts',(-21.9451658727967,-65.6937185963808,
28.5540810945656));
#33704=CARTESIAN_POINT('Ctrl Pts',(-20.797702550644,-64.1996808028605,28.4429479765739));
#33705=CARTESIAN_POINT('Ctrl Pts',(-18.9201504568774,-64.3533659984344,
28.3318148585824));
#33706=CARTESIAN_POINT('Ctrl Pts',(-18.0309191674365,-66.0141154431258,
28.2206817405908));
#33707=CARTESIAN_POINT('Ctrl Pts',(-18.943868158232,-67.6619458786863,28.1095486225993));
#33708=CARTESIAN_POINT('Ctrl Pts',(-20.8234305795421,-67.7886980325282,
27.9984155046077));
#33709=CARTESIAN_POINT('Ctrl Pts',(-21.9493569245747,-66.278363344517,27.8872823866162));
#33710=CARTESIAN_POINT('Ctrl Pts',(-21.2911550862336,-64.513259567359,27.7761492686246));
#33711=CARTESIAN_POINT('Ctrl Pts',(-19.4512372937262,-64.1088791516278,
27.6650161506331));
#33712=CARTESIAN_POINT('Ctrl Pts',(-18.1135687288438,-65.4353269702371,
27.5538830326415));
#33713=CARTESIAN_POINT('Ctrl Pts',(-18.5024363130261,-67.2785857707618,
27.4427499146499));
#33714=CARTESIAN_POINT('Ctrl Pts',(-20.26193312608,-67.9516325497133,27.3316167966584));
#33715=CARTESIAN_POINT('Ctrl Pts',(-21.7816984345104,-66.8384684027146,
27.2204836786668));
#33716=CARTESIAN_POINT('Ctrl Pts',(-21.6707832048173,-64.9579049736386,
27.1093505606753));
#33717=CARTESIAN_POINT('Ctrl Pts',(-20.0307014324503,-64.0311079253974,
26.9982174426837));
#33718=CARTESIAN_POINT('Ctrl Pts',(-18.3625204852342,-64.9063184061494,
26.8870843246922));
#33719=CARTESIAN_POINT('Ctrl Pts',(-18.1930252713496,-66.782509313568,26.7759512067006));
#33720=CARTESIAN_POINT('Ctrl Pts',(-19.6773443894448,-67.9425169276774,
26.6648180887091));
#33721=CARTESIAN_POINT('Ctrl Pts',(-21.4569707445669,-67.32465653357,26.5536849707174));
#33722=CARTESIAN_POINT('Ctrl Pts',(-21.90311988392,-65.4944184601696,26.4425518527259));
#33723=CARTESIAN_POINT('Ctrl Pts',(-20.6074592869896,-64.1269082758429,
26.3314187347343));
#33724=CARTESIAN_POINT('Ctrl Pts',(-18.7558270691641,-64.473725831526,26.2202856167428));
#33725=CARTESIAN_POINT('Ctrl Pts',(-18.0429128259432,-66.2174486428944,
26.1091524987512));
#33726=CARTESIAN_POINT('Ctrl Pts',(-19.1211979303562,-67.7621557655232,
25.9980193807597));
#33727=CARTESIAN_POINT('Ctrl Pts',(-21.0038049828108,-67.6940648494755,
25.8868862627682));
#33728=CARTESIAN_POINT('Ctrl Pts',(-21.9676748441585,-66.0755065309653,
25.7757531447765));
#33729=CARTESIAN_POINT('Ctrl Pts',(-21.1306818689754,-64.3878268583619,
25.664620026785));
#33730=CARTESIAN_POINT('Ctrl Pts',(-19.2587832782431,-64.1757010178898,
25.5534869087934));
#33731=CARTESIAN_POINT('Ctrl Pts',(-18.0653971591218,-65.6331865556109,
25.4423537908019));
#33732=CARTESIAN_POINT('Ctrl Pts',(-18.6423929466843,-67.4265115387061,
25.3312206728103));
#33733=CARTESIAN_POINT('Ctrl Pts',(-20.4624082215941,-67.9140030533836,
25.2200875548188));
#33734=CARTESIAN_POINT('Ctrl Pts',(-21.8582433164759,-66.650190129261,25.1089544368272));
#33735=CARTESIAN_POINT('Ctrl Pts',(-21.5552776423771,-64.7903673634893,
24.9978213188357));
#33736=CARTESIAN_POINT('Ctrl Pts',(-19.8248705803293,-64.0395083111156,
24.8866882008441));
#33737=CARTESIAN_POINT('Ctrl Pts',(-18.7848659979775,-64.7327675918889,
24.8125994555164));
#33738=CARTESIAN_POINT('Ctrl Pts',(-18.5264217726374,-65.2227463683951,
24.7755550828525));
#33739=CARTESIAN_POINT('Ctrl Pts',(-18.6322193753412,-64.8366876301902,
36.0748149723825));
#33740=CARTESIAN_POINT('Ctrl Pts',(-18.2454069475584,-65.2914876975057,
36.0377705997186));
#33741=CARTESIAN_POINT('Ctrl Pts',(-17.9681227304658,-66.6097459389905,
35.9636818543909));
#33742=CARTESIAN_POINT('Ctrl Pts',(-19.4123269945801,-68.040621101442,35.8525487363994));
#33743=CARTESIAN_POINT('Ctrl Pts',(-21.3946565954591,-67.599101991962,35.7414156184078));
#33744=CARTESIAN_POINT('Ctrl Pts',(-22.1003861870635,-65.6963321743655,
35.6302825004162));
#33745=CARTESIAN_POINT('Ctrl Pts',(-20.8838396803442,-64.0703377208937,
35.5191493824247));
#33746=CARTESIAN_POINT('Ctrl Pts',(-18.858328024941,-64.2110242041256,35.4080162644331));
#33747=CARTESIAN_POINT('Ctrl Pts',(-17.8777397145028,-65.9887618494759,
35.2968831464416));
#33748=CARTESIAN_POINT('Ctrl Pts',(-18.8395174075388,-67.7769304901502,
35.18575002845));
#33749=CARTESIAN_POINT('Ctrl Pts',(-20.8634195317534,-67.9387094824621,
35.0746169104584));
#33750=CARTESIAN_POINT('Ctrl Pts',(-22.0970835655348,-66.3261418250617,
34.963483792467));
#33751=CARTESIAN_POINT('Ctrl Pts',(-21.4114154592526,-64.4150579879853,
34.8523506744753));
#33752=CARTESIAN_POINT('Ctrl Pts',(-19.4339637301444,-63.954584663791,34.7412175564838));
#33753=CARTESIAN_POINT('Ctrl Pts',(-17.9745709960488,-65.3661513473781,
34.6300844384922));
#33754=CARTESIAN_POINT('Ctrl Pts',(-18.368930445043,-67.3578435803929,34.5189513205007));
#33755=CARTESIAN_POINT('Ctrl Pts',(-20.2561090299742,-68.1067827635803,
34.4078182025091));
#33756=CARTESIAN_POINT('Ctrl Pts',(-21.90888650971,-66.9275120216053,34.2966850845175));
#33757=CARTESIAN_POINT('Ctrl Pts',(-21.8145759430863,-64.8993454789214,
34.185551966526));
#33758=CARTESIAN_POINT('Ctrl Pts',(-20.0594940421212,-63.8785414217313,
34.0744188485344));
#33759=CARTESIAN_POINT('Ctrl Pts',(-18.2499608572679,-64.7993796817096,
33.9632857305429));
#33760=CARTESIAN_POINT('Ctrl Pts',(-18.0421323741426,-66.8190729497863,
33.8521526125513));
#33761=CARTESIAN_POINT('Ctrl Pts',(-19.6262214044097,-68.0891183973422,
33.7410194945598));
#33762=CARTESIAN_POINT('Ctrl Pts',(-21.5524073164968,-67.44712047002,33.6298863765682));
#33763=CARTESIAN_POINT('Ctrl Pts',(-22.0577689506937,-65.4806609257802,
33.5187532585766));
#33764=CARTESIAN_POINT('Ctrl Pts',(-20.6797794480564,-63.9895209455846,
33.4076201405851));
#33765=CARTESIAN_POINT('Ctrl Pts',(-18.6796290387811,-64.3384505265051,
33.2964870225935));
#33766=CARTESIAN_POINT('Ctrl Pts',(-17.8879341024671,-66.2080955841046,
33.185353904602));
#33767=CARTESIAN_POINT('Ctrl Pts',(-19.0292850056993,-67.887283372275,33.0742207866104));
#33768=CARTESIAN_POINT('Ctrl Pts',(-21.0590724786751,-67.8391551355372,
32.9630876686189));
#33769=CARTESIAN_POINT('Ctrl Pts',(-22.1195551344861,-66.107759730241,32.8519545506273));
#33770=CARTESIAN_POINT('Ctrl Pts',(-21.2401375063356,-64.2777383784837,
32.7408214326358));
#33771=CARTESIAN_POINT('Ctrl Pts',(-19.2256972210515,-64.0239986502764,
32.6296883146441));
#33772=CARTESIAN_POINT('Ctrl Pts',(-17.9199293153208,-65.5787731320006,
32.5185551966526));
#33773=CARTESIAN_POINT('Ctrl Pts',(-18.5179239709932,-67.5190710226412,
32.407422078661));
#33774=CARTESIAN_POINT('Ctrl Pts',(-20.4723729423565,-68.06905532331,32.2962889606695));
#33775=CARTESIAN_POINT('Ctrl Pts',(-21.9944876044574,-66.7253587548605,
32.1851558426779));
#33776=CARTESIAN_POINT('Ctrl Pts',(-21.6911687086917,-64.7177853041207,
32.0740227246864));
#33777=CARTESIAN_POINT('Ctrl Pts',(-19.8400256469796,-63.883745210528,31.9628896066948));
#33778=CARTESIAN_POINT('Ctrl Pts',(-18.135297409681,-64.9865847952371,31.8517564887032));
#33779=CARTESIAN_POINT('Ctrl Pts',(-18.1372183770211,-67.0169418629789,
31.7406233707117));
#33780=CARTESIAN_POINT('Ctrl Pts',(-19.8440304040817,-68.1165537112807,
31.6294902527201));
#33781=CARTESIAN_POINT('Ctrl Pts',(-21.6935919442302,-67.2790122962762,
31.5183571347286));
#33782=CARTESIAN_POINT('Ctrl Pts',(-21.9931114778899,-65.2708684862861,
31.407224016737));
#33783=CARTESIAN_POINT('Ctrl Pts',(-20.4684569388814,-63.9300545359839,
31.2960908987454));
#33784=CARTESIAN_POINT('Ctrl Pts',(-18.5150521711233,-64.4837361466086,
31.1849577807539));
#33785=CARTESIAN_POINT('Ctrl Pts',(-17.92073010333,-66.4251621154209,31.0738246627623));
#33786=CARTESIAN_POINT('Ctrl Pts',(-19.2294376842349,-67.9774629819821,
30.9626915447708));
#33787=CARTESIAN_POINT('Ctrl Pts',(-21.2433942255651,-67.7199118952488,
30.8515584267792));
#33788=CARTESIAN_POINT('Ctrl Pts',(-22.1193474321384,-65.8882297469111,
30.7404253087876));
#33789=CARTESIAN_POINT('Ctrl Pts',(-21.0555904521165,-64.1588441334349,
30.6292921907961));
#33790=CARTESIAN_POINT('Ctrl Pts',(-19.0257155426823,-64.1145568362275,
30.5181590728046));
#33791=CARTESIAN_POINT('Ctrl Pts',(-17.8875441160478,-65.7959013328247,
30.407025954813));
#33792=CARTESIAN_POINT('Ctrl Pts',(-18.6827754598598,-67.6640449628659,
30.2958928368214));
#33793=CARTESIAN_POINT('Ctrl Pts',(-20.6835825482607,-68.0091891467207,
30.1847597188298));
#33794=CARTESIAN_POINT('Ctrl Pts',(-22.0587479829466,-66.5154443425826,
30.0736266008383));
#33795=CARTESIAN_POINT('Ctrl Pts',(-21.5496662321087,-64.5499445884212,
29.9624934828467));
#33796=CARTESIAN_POINT('Ctrl Pts',(-19.6222689513765,-63.9115926205616,
29.8513603648552));
#33797=CARTESIAN_POINT('Ctrl Pts',(-18.0405859936936,-65.1846332852775,
29.7402272468636));
#33798=CARTESIAN_POINT('Ctrl Pts',(-18.2522358563662,-67.2039296598285,
29.6290941288721));
#33799=CARTESIAN_POINT('Ctrl Pts',(-20.0635082546187,-68.1213422234949,
29.5179610108805));
#33800=CARTESIAN_POINT('Ctrl Pts',(-21.8166553985837,-67.0972188890024,
29.406827892889));
#33801=CARTESIAN_POINT('Ctrl Pts',(-21.9071280189051,-65.0688776411803,
29.2956947748974));
#33802=CARTESIAN_POINT('Ctrl Pts',(-20.2521220124972,-63.8927362247689,
29.1845616569058));
#33803=CARTESIAN_POINT('Ctrl Pts',(-18.3663640168262,-64.645245556543,29.0734285389143));
#33804=CARTESIAN_POINT('Ctrl Pts',(-17.9757739722415,-66.6376794775842,
28.9622954209227));
#33805=CARTESIAN_POINT('Ctrl Pts',(-19.4378352610216,-68.0464840419207,
28.8511623029311));
#33806=CARTESIAN_POINT('Ctrl Pts',(-21.414411845503,-67.5822658622644,28.7400291849396));
#33807=CARTESIAN_POINT('Ctrl Pts',(-22.0964630382728,-65.6698956880862,
28.628896066948));
#33808=CARTESIAN_POINT('Ctrl Pts',(-20.8597487424332,-64.0596499729509,
28.5177629489565));
#33809=CARTESIAN_POINT('Ctrl Pts',(-18.8361585581401,-64.225288974003,28.4066298309649));
#33810=CARTESIAN_POINT('Ctrl Pts',(-17.8777618697857,-66.0152133579947,
28.2954967129733));
#33811=CARTESIAN_POINT('Ctrl Pts',(-18.8617210486907,-67.7912138779539,
28.1843635949818));
#33812=CARTESIAN_POINT('Ctrl Pts',(-20.8874779260401,-67.9278249553264,
28.0732304769902));
#33813=CARTESIAN_POINT('Ctrl Pts',(-22.1009800747204,-66.3000147551173,
27.9620973589987));
#33814=CARTESIAN_POINT('Ctrl Pts',(-21.3915825651798,-64.3976192425913,
27.8509642410071));
#33815=CARTESIAN_POINT('Ctrl Pts',(-19.4085539199639,-63.9617856682735,
27.7398311230155));
#33816=CARTESIAN_POINT('Ctrl Pts',(-17.9668400060223,-65.3914060738144,
27.628698005024));
#33817=CARTESIAN_POINT('Ctrl Pts',(-18.3859541434961,-67.378035594368,27.5175648870324));
#33818=CARTESIAN_POINT('Ctrl Pts',(-20.2823065760127,-68.1034327005137,
27.4064317690409));
#33819=CARTESIAN_POINT('Ctrl Pts',(-21.9202809207881,-66.9036854078278,
27.2952986510493));
#33820=CARTESIAN_POINT('Ctrl Pts',(-21.8007385811424,-64.8768496632148,
27.1841655330578));
#33821=CARTESIAN_POINT('Ctrl Pts',(-20.0330894240199,-63.8779653095508,
27.0730324150662));
#33822=CARTESIAN_POINT('Ctrl Pts',(-18.2351555069698,-64.821250635119,26.9618992970747));
#33823=CARTESIAN_POINT('Ctrl Pts',(-18.0524767667952,-66.8433737584758,
26.8507661790831));
#33824=CARTESIAN_POINT('Ctrl Pts',(-19.6522478771192,-68.0936080552553,
26.7396330610915));
#33825=CARTESIAN_POINT('Ctrl Pts',(-21.5702955498791,-67.4276897923586,
26.6284999431));
#33826=CARTESIAN_POINT('Ctrl Pts',(-22.0511466656074,-65.4550937655699,
26.5173668251084));
#33827=CARTESIAN_POINT('Ctrl Pts',(-20.6547081460967,-63.9812171178266,
26.4062337071169));
#33828=CARTESIAN_POINT('Ctrl Pts',(-18.6590539145297,-64.3550105288059,
26.2951005891253));
#33829=CARTESIAN_POINT('Ctrl Pts',(-17.8906884083933,-66.2343620402385,
26.1839674711337));
#33830=CARTESIAN_POINT('Ctrl Pts',(-19.0528437277604,-67.8992182012669,
26.0728343531422));
#33831=CARTESIAN_POINT('Ctrl Pts',(-21.0818820510516,-67.8258310980217,
25.9617012351506));
#33832=CARTESIAN_POINT('Ctrl Pts',(-22.1207227824672,-66.0813795129406,
25.850568117159));
#33833=CARTESIAN_POINT('Ctrl Pts',(-21.2186275625656,-64.2624302379513,
25.7394349991675));
#33834=CARTESIAN_POINT('Ctrl Pts',(-19.201130617062,-64.033805013629,25.6283018811759));
#33835=CARTESIAN_POINT('Ctrl Pts',(-17.914921598019,-65.6046553978465,25.5171687631844));
#33836=CARTESIAN_POINT('Ctrl Pts',(-18.5367967598142,-67.5374671931023,
25.4060356451928));
#33837=CARTESIAN_POINT('Ctrl Pts',(-20.4983748474734,-68.0628763400987,
25.2949025272013));
#33838=CARTESIAN_POINT('Ctrl Pts',(-22.0027795488249,-66.7007626408157,
25.1837694092097));
#33839=CARTESIAN_POINT('Ctrl Pts',(-21.676248867562,-64.6962807913717,25.0726362912181));
#33840=CARTESIAN_POINT('Ctrl Pts',(-19.8112488192455,-63.8870190866151,
24.9615031732266));
#33841=CARTESIAN_POINT('Ctrl Pts',(-18.6903515235305,-64.6342008454597,
24.8874144278989));
#33842=CARTESIAN_POINT('Ctrl Pts',(-18.4118052188385,-65.162290716277,24.850370055235));
#33843=CARTESIAN_POINT('Ctrl Pts',(-18.5335096305348,-64.7527339134289,
36.149629944765));
#33844=CARTESIAN_POINT('Ctrl Pts',(-18.1187817934049,-65.2403559097683,
36.1125855721011));
#33845=CARTESIAN_POINT('Ctrl Pts',(-17.82148657907,-66.6537499736649,36.0384968267734));
#33846=CARTESIAN_POINT('Ctrl Pts',(-19.3699159153844,-68.1878882761179,
35.9273637087819));
#33847=CARTESIAN_POINT('Ctrl Pts',(-21.4953059204666,-67.7145056953778,
35.8162305907903));
#33848=CARTESIAN_POINT('Ctrl Pts',(-22.2519664776322,-65.6744171296325,
35.7050974727987));
#33849=CARTESIAN_POINT('Ctrl Pts',(-20.9476244625846,-63.9310782024452,
35.5939643548072));
#33850=CARTESIAN_POINT('Ctrl Pts',(-18.7759360482752,-64.0819177223609,
35.4828312368156));
#33851=CARTESIAN_POINT('Ctrl Pts',(-17.7245808179535,-65.9879508166608,
35.3716981188241));
#33852=CARTESIAN_POINT('Ctrl Pts',(-18.7557679096376,-67.9051676884693,
35.2605650008325));
#33853=CARTESIAN_POINT('Ctrl Pts',(-20.9257306364026,-68.0786219178465,
35.149431882841));
#33854=CARTESIAN_POINT('Ctrl Pts',(-22.2484255131102,-66.3496787693217,
35.0382987648494));
#33855=CARTESIAN_POINT('Ctrl Pts',(-21.5132742349122,-64.300676179442,34.9271656468578));
#33856=CARTESIAN_POINT('Ctrl Pts',(-19.3931141269688,-63.8069714996472,
34.8160325288663));
#33857=CARTESIAN_POINT('Ctrl Pts',(-17.8284002019177,-65.3204078724244,
34.7048994108747));
#33858=CARTESIAN_POINT('Ctrl Pts',(-18.2512197123211,-67.4558361903855,
34.5937662928832));
#33859=CARTESIAN_POINT('Ctrl Pts',(-20.2745918601413,-68.2588246811265,
34.4826331748916));
#33860=CARTESIAN_POINT('Ctrl Pts',(-22.0466466861892,-66.9944485414733,
34.3715000569001));
#33861=CARTESIAN_POINT('Ctrl Pts',(-21.9455299316461,-64.819913642458,34.2603669389084));
#33862=CARTESIAN_POINT('Ctrl Pts',(-20.0637875973957,-63.7254403826442,
34.149233820917));
#33863=CARTESIAN_POINT('Ctrl Pts',(-18.1236643488468,-64.7127335316683,
34.0381007029253));
#33864=CARTESIAN_POINT('Ctrl Pts',(-17.9008373373297,-66.8781836583265,
33.9269675849339));
#33865=CARTESIAN_POINT('Ctrl Pts',(-19.5992466183076,-68.2398855160997,
33.8158344669422));
#33866=CARTESIAN_POINT('Ctrl Pts',(-21.6644411670167,-67.5515559984407,
33.7047013489507));
#33867=CARTESIAN_POINT('Ctrl Pts',(-22.2062736482538,-65.4431813573757,
33.5935682309591));
#33868=CARTESIAN_POINT('Ctrl Pts',(-20.7288376483501,-63.8444290567085,
33.4824351129676));
#33869=CARTESIAN_POINT('Ctrl Pts',(-18.5843407459935,-64.2185401245333,
33.371301994976));
#33870=CARTESIAN_POINT('Ctrl Pts',(-17.7355109126651,-66.2231133885917,
33.2601688769844));
#33871=CARTESIAN_POINT('Ctrl Pts',(-18.9592306215095,-68.023484497438,33.1490357589929));
#33872=CARTESIAN_POINT('Ctrl Pts',(-21.135503429821,-67.9718829508136,33.0379026410013));
#33873=CARTESIAN_POINT('Ctrl Pts',(-22.2725188061863,-66.1155365149686,
32.9267695230097));
#33874=CARTESIAN_POINT('Ctrl Pts',(-21.3296355256586,-64.1534465131912,
32.8156364050182));
#33875=CARTESIAN_POINT('Ctrl Pts',(-19.1698174781052,-63.8813949421583,
32.7045032870266));
#33876=CARTESIAN_POINT('Ctrl Pts',(-17.7698151502549,-65.5483741075547,
32.5933701690351));
#33877=CARTESIAN_POINT('Ctrl Pts',(-18.410965776112,-67.6286990655338,32.4822370510435));
#33878=CARTESIAN_POINT('Ctrl Pts',(-20.5064630674488,-68.2183745337685,
32.371103933052));
#33879=CARTESIAN_POINT('Ctrl Pts',(-22.1384254252645,-66.7777063143262,
32.2599708150604));
#33880=CARTESIAN_POINT('Ctrl Pts',(-21.8132166662735,-64.6252506657909,
32.1488376970689));
#33881=CARTESIAN_POINT('Ctrl Pts',(-19.8284806467965,-63.73101971753,32.0377045790773));
#33882=CARTESIAN_POINT('Ctrl Pts',(-18.0007258903072,-64.9134488299795,
31.9265714610857));
#33883=CARTESIAN_POINT('Ctrl Pts',(-18.002785489671,-67.090332339469,31.8154383430942));
#33884=CARTESIAN_POINT('Ctrl Pts',(-19.8327744184849,-68.2693007768138,
31.7043052251026));
#33885=CARTESIAN_POINT('Ctrl Pts',(-21.8158147814363,-67.3713158244104,
31.5931721071111));
#33886=CARTESIAN_POINT('Ctrl Pts',(-22.1369499866437,-65.2182486550417,
31.4820389891195));
#33887=CARTESIAN_POINT('Ctrl Pts',(-20.502264454543,-63.780671086012,31.3709058711279));
#33888=CARTESIAN_POINT('Ctrl Pts',(-18.4078867247083,-64.3743106909989,
31.2597727531364));
#33889=CARTESIAN_POINT('Ctrl Pts',(-17.7706737293884,-66.4558451380913,
31.1486396351448));
#33890=CARTESIAN_POINT('Ctrl Pts',(-19.1738278823592,-68.1201721729128,
31.0375065171533));
#33891=CARTESIAN_POINT('Ctrl Pts',(-21.3331272752126,-67.8440341859209,
30.9263733991617));
#33892=CARTESIAN_POINT('Ctrl Pts',(-22.2722961144131,-65.8801635314959,
30.8152402811701));
#33893=CARTESIAN_POINT('Ctrl Pts',(-21.1317701129993,-64.0259719297634,
30.7041071631786));
#33894=CARTESIAN_POINT('Ctrl Pts',(-18.9554035581309,-63.978488514899,30.592974045187));
#33895=CARTESIAN_POINT('Ctrl Pts',(-17.7350927817764,-65.7811719771159,
30.4818409271955));
#33896=CARTESIAN_POINT('Ctrl Pts',(-18.5877142374196,-67.7841354588633,
30.3707078092039));
#33897=CARTESIAN_POINT('Ctrl Pts',(-20.7329152100023,-68.1541879457717,
30.2595746912124));
#33898=CARTESIAN_POINT('Ctrl Pts',(-22.2073233351293,-66.5526428366984,
30.1484415732208));
#33899=CARTESIAN_POINT('Ctrl Pts',(-21.6615022645462,-64.4452972516688,
30.0373084552293));
#33900=CARTESIAN_POINT('Ctrl Pts',(-19.5950089253585,-63.7608768144156,
29.9261753372376));
#33901=CARTESIAN_POINT('Ctrl Pts',(-17.8991793579761,-65.1257900476391,
29.8150422192461));
#33902=CARTESIAN_POINT('Ctrl Pts',(-18.1261035296687,-67.2908146378317,
29.7039091012545));
#33903=CARTESIAN_POINT('Ctrl Pts',(-20.0680915068549,-68.2744348655116,
29.592775983263));
#33904=CARTESIAN_POINT('Ctrl Pts',(-21.9477594569119,-67.1764027833913,
29.4816428652714));
#33905=CARTESIAN_POINT('Ctrl Pts',(-22.044761288938,-65.001680571149,29.3705097472799));
#33906=CARTESIAN_POINT('Ctrl Pts',(-20.2703171083079,-63.7406595936608,
29.2593766292883));
#33907=CARTESIAN_POINT('Ctrl Pts',(-18.2484680705768,-64.5474758828262,
29.1482435112968));
#33908=CARTESIAN_POINT('Ctrl Pts',(-17.8296899942787,-66.683699414821,29.0371103933052));
#33909=CARTESIAN_POINT('Ctrl Pts',(-19.3972650577863,-68.1941743322251,
28.9259772753137));
#33910=CARTESIAN_POINT('Ctrl Pts',(-21.5164868638238,-67.6964545389165,
28.8148441573221));
#33911=CARTESIAN_POINT('Ctrl Pts',(-22.247760203749,-65.6460727797915,28.7037110393305));
#33912=CARTESIAN_POINT('Ctrl Pts',(-20.9217949342225,-63.9196191430413,
28.592577921339));
#33913=CARTESIAN_POINT('Ctrl Pts',(-18.7521666594028,-64.0972119495715,
28.4814448033474));
#33914=CARTESIAN_POINT('Ctrl Pts',(-17.7246045721348,-66.0163112728636,
28.3703116853558));
#33915=CARTESIAN_POINT('Ctrl Pts',(-18.7795739391494,-67.9204818772215,
28.2591785673643));
#33916=CARTESIAN_POINT('Ctrl Pts',(-20.9515252725381,-68.0669518781245,
28.1480454493727));
#33917=CARTESIAN_POINT('Ctrl Pts',(-22.2526032248661,-66.3216661657179,
28.0369123313812));
#33918=CARTESIAN_POINT('Ctrl Pts',(-21.492010044126,-64.2819789178235,27.9257792133896));
#33919=CARTESIAN_POINT('Ctrl Pts',(-19.3658705462016,-63.8146921849193,
27.8146460953981));
#33920=CARTESIAN_POINT('Ctrl Pts',(-17.8201112832008,-65.3474851773918,
27.7035129774065));
#33921=CARTESIAN_POINT('Ctrl Pts',(-18.2694719739661,-67.4774854179741,
27.5923798594149));
#33922=CARTESIAN_POINT('Ctrl Pts',(-20.3026800259454,-68.2552328513142,
27.4812467414234));
#33923=CARTESIAN_POINT('Ctrl Pts',(-22.0588634070658,-66.9689024129409,
27.3701136234318));
#33924=CARTESIAN_POINT('Ctrl Pts',(-21.9306939574675,-64.7957943527911,
27.2589805054402));
#33925=CARTESIAN_POINT('Ctrl Pts',(-20.0354774155896,-63.724822693704,27.1478473874487));
#33926=CARTESIAN_POINT('Ctrl Pts',(-18.1077905287054,-64.7361828640888,
27.0367142694571));
#33927=CARTESIAN_POINT('Ctrl Pts',(-17.9119282622408,-66.9042382033836,
26.9255811514656));
#33928=CARTESIAN_POINT('Ctrl Pts',(-19.6271513647936,-68.2446991828334,
26.814448033474));
#33929=CARTESIAN_POINT('Ctrl Pts',(-21.6836203551913,-67.530723051147,26.7033149154825));
#33930=CARTESIAN_POINT('Ctrl Pts',(-22.1991734472949,-65.4157690709703,
26.5921817974909));
#33931=CARTESIAN_POINT('Ctrl Pts',(-20.7019570052038,-63.8355259598101,
26.4810486794993));
#33932=CARTESIAN_POINT('Ctrl Pts',(-18.5622807598954,-64.236295226086,26.3699155615078));
#33933=CARTESIAN_POINT('Ctrl Pts',(-17.7384639908433,-66.2512754375824,
26.2587824435162));
#33934=CARTESIAN_POINT('Ctrl Pts',(-18.9844895251645,-68.0362806370106,
26.1476493255246));
#33935=CARTESIAN_POINT('Ctrl Pts',(-21.1599591192924,-67.9575973465678,
26.0365162075331));
#33936=CARTESIAN_POINT('Ctrl Pts',(-22.2737707207758,-66.087252494916,25.9253830895415));
#33937=CARTESIAN_POINT('Ctrl Pts',(-21.3065732561559,-64.1370336175406,
25.81424997155));
#33938=CARTESIAN_POINT('Ctrl Pts',(-19.143477955881,-63.8919090093683,25.7031168535584));
#33939=CARTESIAN_POINT('Ctrl Pts',(-17.7644460369163,-65.5761242400821,
25.5919837355669));
#33940=CARTESIAN_POINT('Ctrl Pts',(-18.4312005729442,-67.6484228474986,
25.4808506175753));
#33941=CARTESIAN_POINT('Ctrl Pts',(-20.5343414733527,-68.2117496268139,
25.3697174995837));
#33942=CARTESIAN_POINT('Ctrl Pts',(-22.1473157811738,-66.7513351523705,
25.2585843815922));
#33943=CARTESIAN_POINT('Ctrl Pts',(-21.7972200927469,-64.6021942192541,
25.1474512636006));
#33944=CARTESIAN_POINT('Ctrl Pts',(-19.7976270581616,-63.7345298621146,
25.0363181456091));
#33945=CARTESIAN_POINT('Ctrl Pts',(-18.5958370490835,-64.5356340990305,
24.9622294002814));
#33946=CARTESIAN_POINT('Ctrl Pts',(-18.2971886650395,-65.1018350641589,
24.9251850276175));
#33947=CARTESIAN_POINT('Ctrl Pts',(-18.4347998857283,-64.6687801966677,
36.2244449171475));
#33948=CARTESIAN_POINT('Ctrl Pts',(-17.9921566392513,-65.1892241220309,
36.1874005444836));
#33949=CARTESIAN_POINT('Ctrl Pts',(-17.6748504276742,-66.6977540083394,
36.1133117991559));
#33950=CARTESIAN_POINT('Ctrl Pts',(-19.3275048361888,-68.3351554507938,
36.0021786811644));
#33951=CARTESIAN_POINT('Ctrl Pts',(-21.5959552454742,-67.8299093987937,
35.8910455631728));
#33952=CARTESIAN_POINT('Ctrl Pts',(-22.4035467682009,-65.6525020848995,
35.7799124451812));
#33953=CARTESIAN_POINT('Ctrl Pts',(-21.0114092448251,-63.7918186839967,
35.6687793271897));
#33954=CARTESIAN_POINT('Ctrl Pts',(-18.6935440716095,-63.9528112405962,
35.5576462091981));
#33955=CARTESIAN_POINT('Ctrl Pts',(-17.5714219214042,-65.9871397838458,
35.4465130912065));
#33956=CARTESIAN_POINT('Ctrl Pts',(-18.6720184117364,-68.0334048867885,
35.335379973215));
#33957=CARTESIAN_POINT('Ctrl Pts',(-20.9880417410518,-68.218534353231,35.2242468552234));
#33958=CARTESIAN_POINT('Ctrl Pts',(-22.3997674606856,-66.3732157135816,
35.1131137372319));
#33959=CARTESIAN_POINT('Ctrl Pts',(-21.6151330105718,-64.1862943708987,
35.0019806192403));
#33960=CARTESIAN_POINT('Ctrl Pts',(-19.3522645237931,-63.6593583355034,
34.8908475012488));
#33961=CARTESIAN_POINT('Ctrl Pts',(-17.6822294077865,-65.2746643974708,
34.7797143832572));
#33962=CARTESIAN_POINT('Ctrl Pts',(-18.1335089795993,-67.5538288003781,
34.6685812652656));
#33963=CARTESIAN_POINT('Ctrl Pts',(-20.2930746903084,-68.4108665986726,
34.5574481472741));
#33964=CARTESIAN_POINT('Ctrl Pts',(-22.1844068626685,-67.0613850613413,
34.4463150292825));
#33965=CARTESIAN_POINT('Ctrl Pts',(-22.076483920206,-64.7404818059946,34.3351819112909));
#33966=CARTESIAN_POINT('Ctrl Pts',(-20.0680811526701,-63.5723393435572,
34.2240487932995));
#33967=CARTESIAN_POINT('Ctrl Pts',(-17.9973678404257,-64.6260873816269,
34.1129156753078));
#33968=CARTESIAN_POINT('Ctrl Pts',(-17.7595423005167,-66.9372943668669,
34.0017825573163));
#33969=CARTESIAN_POINT('Ctrl Pts',(-19.5722718322054,-68.3906526348572,
33.8906494393247));
#33970=CARTESIAN_POINT('Ctrl Pts',(-21.7764750175367,-67.6559915268615,
33.7795163213332));
#33971=CARTESIAN_POINT('Ctrl Pts',(-22.354778345814,-65.4057017889712,33.6683832033416));
#33972=CARTESIAN_POINT('Ctrl Pts',(-20.7778958486438,-63.6993371678323,
33.5572500853501));
#33973=CARTESIAN_POINT('Ctrl Pts',(-18.4890524532058,-64.0986297225616,
33.4461169673585));
#33974=CARTESIAN_POINT('Ctrl Pts',(-17.5830877228631,-66.2381311930787,
33.334983849367));
#33975=CARTESIAN_POINT('Ctrl Pts',(-18.8891762373197,-68.159685622601,33.2238507313753));
#33976=CARTESIAN_POINT('Ctrl Pts',(-21.2119343809668,-68.1046107660899,
33.1127176133838));
#33977=CARTESIAN_POINT('Ctrl Pts',(-22.4254824778866,-66.1233132996962,
33.0015844953923));
#33978=CARTESIAN_POINT('Ctrl Pts',(-21.4191335449815,-64.0291546478987,
32.8904513774007));
#33979=CARTESIAN_POINT('Ctrl Pts',(-19.1139377351588,-63.7387912340402,
32.7793182594091));
#33980=CARTESIAN_POINT('Ctrl Pts',(-17.6197009851889,-65.5179750831086,
32.6681851414176));
#33981=CARTESIAN_POINT('Ctrl Pts',(-18.3040075812308,-67.7383271084264,
32.557052023426));
#33982=CARTESIAN_POINT('Ctrl Pts',(-20.5405531925411,-68.3676937442268,
32.4459189054345));
#33983=CARTESIAN_POINT('Ctrl Pts',(-22.2823632460717,-66.8300538737919,
32.3347857874429));
#33984=CARTESIAN_POINT('Ctrl Pts',(-21.9352646238553,-64.532716027461,32.2236526694514));
#33985=CARTESIAN_POINT('Ctrl Pts',(-19.8169356466133,-63.578294224532,32.1125195514598));
#33986=CARTESIAN_POINT('Ctrl Pts',(-17.8661543709335,-64.8403128647219,
32.0013864334682));
#33987=CARTESIAN_POINT('Ctrl Pts',(-17.8683526023209,-67.163722815959,31.8902533154767));
#33988=CARTESIAN_POINT('Ctrl Pts',(-19.8215184328882,-68.4220478423468,
31.7791201974851));
#33989=CARTESIAN_POINT('Ctrl Pts',(-21.9380376186423,-67.4636193525447,
31.6679870794936));
#33990=CARTESIAN_POINT('Ctrl Pts',(-22.2807884953976,-65.1656288237973,
31.556853961502));
#33991=CARTESIAN_POINT('Ctrl Pts',(-20.5360719702046,-63.63128763604,31.4457208435104));
#33992=CARTESIAN_POINT('Ctrl Pts',(-18.3007212782933,-64.2648852353891,
31.3345877255189));
#33993=CARTESIAN_POINT('Ctrl Pts',(-17.6206173554466,-66.4865281607617,
31.2234546075273));
#33994=CARTESIAN_POINT('Ctrl Pts',(-19.1182180804836,-68.2628813638435,
31.1123214895358));
#33995=CARTESIAN_POINT('Ctrl Pts',(-21.42286032486,-67.9681564765929,31.0011883715442));
#33996=CARTESIAN_POINT('Ctrl Pts',(-22.425244796688,-65.8720973160807,30.8900552535526));
#33997=CARTESIAN_POINT('Ctrl Pts',(-21.207949773882,-63.8930997260919,30.778922135561));
#33998=CARTESIAN_POINT('Ctrl Pts',(-18.8850915735795,-63.8424201935705,
30.6677890175695));
#33999=CARTESIAN_POINT('Ctrl Pts',(-17.582641447505,-65.766442621407,30.556655899578));
#34000=CARTESIAN_POINT('Ctrl Pts',(-18.4926530149794,-67.9042259548608,
30.4455227815864));
#34001=CARTESIAN_POINT('Ctrl Pts',(-20.7822478717438,-68.2991867448226,
30.3343896635948));
#34002=CARTESIAN_POINT('Ctrl Pts',(-22.3558986873121,-66.5898413308144,
30.2232565456033));
#34003=CARTESIAN_POINT('Ctrl Pts',(-21.7733382969836,-64.3406499149163,
30.1121234276117));
#34004=CARTESIAN_POINT('Ctrl Pts',(-19.5677488993405,-63.6101610082697,
30.0009903096201));
#34005=CARTESIAN_POINT('Ctrl Pts',(-17.7577727222585,-65.0669468100008,
29.8898571916286));
#34006=CARTESIAN_POINT('Ctrl Pts',(-17.9999712029712,-67.3776996158348,
29.7787240736371));
#34007=CARTESIAN_POINT('Ctrl Pts',(-20.072674759091,-68.4275275075284,29.6675909556455));
#34008=CARTESIAN_POINT('Ctrl Pts',(-22.0788635152401,-67.2555866777803,
29.5564578376539));
#34009=CARTESIAN_POINT('Ctrl Pts',(-22.1823945589708,-64.9344835011177,
29.4453247196624));
#34010=CARTESIAN_POINT('Ctrl Pts',(-20.2885122041186,-63.5885829625528,
29.3341916016708));
#34011=CARTESIAN_POINT('Ctrl Pts',(-18.1305721243274,-64.4497062091094,
29.2230584836793));
#34012=CARTESIAN_POINT('Ctrl Pts',(-17.6836060163159,-66.729719352058,29.1119253656877));
#34013=CARTESIAN_POINT('Ctrl Pts',(-19.3566948545509,-68.3418646225293,
29.0007922476961));
#34014=CARTESIAN_POINT('Ctrl Pts',(-21.6185618821445,-67.8106432155685,
28.8896591297046));
#34015=CARTESIAN_POINT('Ctrl Pts',(-22.3990573692251,-65.6222498714967,
28.778526011713));
#34016=CARTESIAN_POINT('Ctrl Pts',(-20.9838411260118,-63.7795883131318,
28.6673928937215));
#34017=CARTESIAN_POINT('Ctrl Pts',(-18.6681747606656,-63.9691349251399,
28.5562597757299));
#34018=CARTESIAN_POINT('Ctrl Pts',(-17.5714472744839,-66.0174091877327,
28.4451266577383));
#34019=CARTESIAN_POINT('Ctrl Pts',(-18.6974268296081,-68.0497498764889,
28.3339935397468));
#34020=CARTESIAN_POINT('Ctrl Pts',(-21.0155726190361,-68.2060788009229,
28.2228604217552));
#34021=CARTESIAN_POINT('Ctrl Pts',(-22.4042263750118,-66.3433175763181,
28.1117273037637));
#34022=CARTESIAN_POINT('Ctrl Pts',(-21.5924375230723,-64.1663385930559,
28.0005941857721));
#34023=CARTESIAN_POINT('Ctrl Pts',(-19.3231871724393,-63.667598701565,27.8894610677806));
#34024=CARTESIAN_POINT('Ctrl Pts',(-17.6733825603793,-65.3035642809691,
27.778327949789));
#34025=CARTESIAN_POINT('Ctrl Pts',(-18.152989804436,-67.5769352415803,27.6671948317974));
#34026=CARTESIAN_POINT('Ctrl Pts',(-20.3230534758781,-68.4070330021147,
27.5560617138059));
#34027=CARTESIAN_POINT('Ctrl Pts',(-22.1974458933435,-67.034119418054,27.4449285958143));
#34028=CARTESIAN_POINT('Ctrl Pts',(-22.0606493337925,-64.7147390423673,
27.3337954778227));
#34029=CARTESIAN_POINT('Ctrl Pts',(-20.0378654071592,-63.5716800778574,
27.2226623598312));
#34030=CARTESIAN_POINT('Ctrl Pts',(-17.9804255504411,-64.6511150930585,
27.1115292418396));
#34031=CARTESIAN_POINT('Ctrl Pts',(-17.7713797576864,-66.9651026482916,
27.0003961238481));
#34032=CARTESIAN_POINT('Ctrl Pts',(-19.602054852468,-68.3957903104112,26.8892630058565));
#34033=CARTESIAN_POINT('Ctrl Pts',(-21.7969451605035,-67.6337563099357,
26.7781298878649));
#34034=CARTESIAN_POINT('Ctrl Pts',(-22.3472002289823,-65.3764443763705,
26.6669967698734));
#34035=CARTESIAN_POINT('Ctrl Pts',(-20.7492058643109,-63.6898348017937,
26.5558636518818));
#34036=CARTESIAN_POINT('Ctrl Pts',(-18.465507605261,-64.1175799233661,26.4447305338903));
#34037=CARTESIAN_POINT('Ctrl Pts',(-17.5862395732934,-66.2681888349264,
26.3335974158987));
#34038=CARTESIAN_POINT('Ctrl Pts',(-18.9161353225687,-68.1733430727544,
26.2224642979071));
#34039=CARTESIAN_POINT('Ctrl Pts',(-21.2380361875332,-68.089363595114,26.1113311799156));
#34040=CARTESIAN_POINT('Ctrl Pts',(-22.4268186590844,-66.0931254768914,
26.000198061924));
#34041=CARTESIAN_POINT('Ctrl Pts',(-21.3945189497461,-64.0116369971301,
25.8890649439325));
#34042=CARTESIAN_POINT('Ctrl Pts',(-19.0858252946999,-63.7500130051076,
25.7779318259409));
#34043=CARTESIAN_POINT('Ctrl Pts',(-17.6139704758136,-65.5475930823177,
25.6667987079494));
#34044=CARTESIAN_POINT('Ctrl Pts',(-18.3256043860741,-67.7593785018947,
25.5556655899578));
#34045=CARTESIAN_POINT('Ctrl Pts',(-20.570308099232,-68.3606229135291,25.4445324719662));
#34046=CARTESIAN_POINT('Ctrl Pts',(-22.2918520135227,-66.8019076639252,
25.3333993539747));
#34047=CARTESIAN_POINT('Ctrl Pts',(-21.9181913179318,-64.5081076471365,
25.2222662359831));
#34048=CARTESIAN_POINT('Ctrl Pts',(-19.7840052970778,-63.5820406376141,
25.1111331179915));
#34049=CARTESIAN_POINT('Ctrl Pts',(-18.5013225746365,-64.4370673526013,
25.0370443726639));
#34050=CARTESIAN_POINT('Ctrl Pts',(-18.1825721112405,-65.0413794120407,
25.));
#34051=CARTESIAN_POINT('Ctrl Pts',(-18.7309291201477,-64.9206413469514,
36.));
#34052=CARTESIAN_POINT('Ctrl Pts',(-18.6855998945711,-64.9629287034795,
36.));
#34053=CARTESIAN_POINT('Ctrl Pts',(-18.6430006729863,-65.0077851737201,
36.));
#34054=CARTESIAN_POINT('Ctrl Pts',(-18.6031299766235,-65.0548657336984,
36.));
#34055=CARTESIAN_POINT('Ctrl Pts',(-18.5606276998918,-65.105053745733,36.));
#34056=CARTESIAN_POINT('Ctrl Pts',(-18.5212252911969,-65.157769362507,36.));
#34057=CARTESIAN_POINT('Ctrl Pts',(-18.48494979168,-65.2126493493662,36.));
#34058=CARTESIAN_POINT('Ctrl Pts',(-18.4532087296026,-65.2606693378681,
36.));
#34059=CARTESIAN_POINT('Ctrl Pts',(-18.4238619507797,-65.3103476478189,
36.));
#34060=CARTESIAN_POINT('Ctrl Pts',(-18.3969504636413,-65.3614684945306,
36.));
#34061=CARTESIAN_POINT('Ctrl Pts',(-18.3834501843084,-65.3871135176685,
36.));
#34062=CARTESIAN_POINT('Ctrl Pts',(-18.3705631253762,-65.4131219219355,
36.));
#34063=CARTESIAN_POINT('Ctrl Pts',(-18.3582968052852,-65.4394683065982,
36.));
#34064=CARTESIAN_POINT('Ctrl Pts',(-18.3526878548587,-65.4515155680748,
36.));
#34065=CARTESIAN_POINT('Ctrl Pts',(-18.3472081170408,-65.4636351822643,
36.));
#34066=CARTESIAN_POINT('Ctrl Pts',(-18.3418668232121,-65.4758047617324,
36.));
#34067=CARTESIAN_POINT('Ctrl Pts',(-18.3149478587099,-65.5371368075278,
36.));
#34068=CARTESIAN_POINT('Ctrl Pts',(-18.2914900585818,-65.5998443155028,
36.));
#34069=CARTESIAN_POINT('Ctrl Pts',(-18.2715169288168,-65.6635695192081,
36.));
#34070=CARTESIAN_POINT('Ctrl Pts',(-18.2511894863638,-65.728425174099,36.));
#34071=CARTESIAN_POINT('Ctrl Pts',(-18.2344708858127,-65.7943357931695,
36.));
#34072=CARTESIAN_POINT('Ctrl Pts',(-18.2214252225953,-65.8609607427827,
36.));
#34073=CARTESIAN_POINT('Ctrl Pts',(-18.2105139769834,-65.916685099375,36.));
#34074=CARTESIAN_POINT('Ctrl Pts',(-18.2021726753615,-65.9729101042603,
36.));
#34075=CARTESIAN_POINT('Ctrl Pts',(-18.1964636437841,-66.0294487409383,
36.));
#34076=CARTESIAN_POINT('Ctrl Pts',(-18.1938340141056,-66.0554909295261,
36.));
#34077=CARTESIAN_POINT('Ctrl Pts',(-18.1917631829515,-66.081599771445,36.));
#34078=CARTESIAN_POINT('Ctrl Pts',(-18.1902590427239,-66.1077573920335,
36.));
#34079=CARTESIAN_POINT('Ctrl Pts',(-18.18960167741,-66.119189246694,36.));
#34080=CARTESIAN_POINT('Ctrl Pts',(-18.189052668073,-66.1306302131104,36.));
#34081=CARTESIAN_POINT('Ctrl Pts',(-18.1886130081778,-66.14206466439,36.));
#34082=CARTESIAN_POINT('Ctrl Pts',(-18.1859166238465,-66.2121908587719,
36.));
#34083=CARTESIAN_POINT('Ctrl Pts',(-18.187320978683,-66.2822033640486,36.));
#34084=CARTESIAN_POINT('Ctrl Pts',(-18.1928807035668,-66.3517413797487,
36.));
#34085=CARTESIAN_POINT('Ctrl Pts',(-18.1978502575643,-66.4138978589117,
36.));
#34086=CARTESIAN_POINT('Ctrl Pts',(-18.2061401607249,-66.4756762006059,
36.));
#34087=CARTESIAN_POINT('Ctrl Pts',(-18.2178225373334,-66.5368308666899,
36.));
#34088=CARTESIAN_POINT('Ctrl Pts',(-18.2305529842617,-66.6034719498439,
36.));
#34089=CARTESIAN_POINT('Ctrl Pts',(-18.2473108243593,-66.6693732662793,
36.));
#34090=CARTESIAN_POINT('Ctrl Pts',(-18.2678508258431,-66.7343212384354,
36.));
#34091=CARTESIAN_POINT('Ctrl Pts',(-18.2757801894081,-66.7593940742109,
36.));
#34092=CARTESIAN_POINT('Ctrl Pts',(-18.2842737653242,-66.784324785242,36.));
#34093=CARTESIAN_POINT('Ctrl Pts',(-18.2933194547362,-66.8091007633723,
36.));
#34094=CARTESIAN_POINT('Ctrl Pts',(-18.2972868318851,-66.8199673369411,
36.));
#34095=CARTESIAN_POINT('Ctrl Pts',(-18.3013603141585,-66.8308035780201,
36.));
#34096=CARTESIAN_POINT('Ctrl Pts',(-18.3055337954211,-66.8415958863165,
36.));
#34097=CARTESIAN_POINT('Ctrl Pts',(-18.3307566163043,-66.9068202019305,
36.));
#34098=CARTESIAN_POINT('Ctrl Pts',(-18.3596702577605,-66.9705591095508,
36.));
#34099=CARTESIAN_POINT('Ctrl Pts',(-18.3919620622396,-67.0325938038885,
36.));
#34100=CARTESIAN_POINT('Ctrl Pts',(-18.4250018795219,-67.0960654803447,
36.));
#34101=CARTESIAN_POINT('Ctrl Pts',(-18.4615784793499,-67.1577538950259,
36.));
#34102=CARTESIAN_POINT('Ctrl Pts',(-18.5014131074424,-67.2174209687524,
36.));
#34103=CARTESIAN_POINT('Ctrl Pts',(-18.5319058104575,-67.2630950580072,
36.));
#34104=CARTESIAN_POINT('Ctrl Pts',(-18.5643088135805,-67.3075847482202,
36.));
#34105=CARTESIAN_POINT('Ctrl Pts',(-18.598516631454,-67.3507771468078,36.));
#34106=CARTESIAN_POINT('Ctrl Pts',(-18.6198131995129,-67.3776671945607,
36.));
#34107=CARTESIAN_POINT('Ctrl Pts',(-18.641809612871,-67.4040543069109,36.));
#34108=CARTESIAN_POINT('Ctrl Pts',(-18.6644833259196,-67.4299095535707,
36.));
#34109=CARTESIAN_POINT('Ctrl Pts',(-18.677161402459,-67.4443665944354,36.));
#34110=CARTESIAN_POINT('Ctrl Pts',(-18.6900557042991,-67.4586618783781,
36.));
#34111=CARTESIAN_POINT('Ctrl Pts',(-18.7031386066276,-67.4727649428971,
36.));
#34112=CARTESIAN_POINT('Ctrl Pts',(-18.7540098725322,-67.5276029847322,
36.));
#34113=CARTESIAN_POINT('Ctrl Pts',(-18.8077776801803,-67.5795960840031,
36.));
#34114=CARTESIAN_POINT('Ctrl Pts',(-18.8641570822702,-67.6284803205922,
36.));
#34115=CARTESIAN_POINT('Ctrl Pts',(-18.9063166745294,-67.6650351510109,
36.));
#34116=CARTESIAN_POINT('Ctrl Pts',(-18.9499377755388,-67.6998513681333,
36.));
#34117=CARTESIAN_POINT('Ctrl Pts',(-18.9949176240316,-67.7328088704017,
36.));
#34118=CARTESIAN_POINT('Ctrl Pts',(-19.0089812695787,-67.7431135433954,
36.));
#34119=CARTESIAN_POINT('Ctrl Pts',(-19.0231778384453,-67.7532364320782,
36.));
#34120=CARTESIAN_POINT('Ctrl Pts',(-19.0375044310318,-67.7631736385769,
36.));
#34121=CARTESIAN_POINT('Ctrl Pts',(-19.0512937947226,-67.7727382125433,
36.));
#34122=CARTESIAN_POINT('Ctrl Pts',(-19.0651965725833,-67.7821258221753,
36.));
#34123=CARTESIAN_POINT('Ctrl Pts',(-19.0792048052933,-67.7913302509702,
36.));
#34124=CARTESIAN_POINT('Ctrl Pts',(-19.1421585203574,-67.8326954252703,
36.));
#34125=CARTESIAN_POINT('Ctrl Pts',(-19.2072696868205,-67.870384921608,36.));
#34126=CARTESIAN_POINT('Ctrl Pts',(-19.2742770195005,-67.9041195716521,
36.));
#34127=CARTESIAN_POINT('Ctrl Pts',(-19.3255044410234,-67.9299098705436,
36.));
#34128=CARTESIAN_POINT('Ctrl Pts',(-19.3778410840131,-67.9533882828924,
36.));
#34129=CARTESIAN_POINT('Ctrl Pts',(-19.431184066025,-67.9744148140802,36.));
#34130=CARTESIAN_POINT('Ctrl Pts',(-19.4436313126694,-67.9793212218193,
36.));
#34131=CARTESIAN_POINT('Ctrl Pts',(-19.4561333979725,-67.9840940592263,
36.));
#34132=CARTESIAN_POINT('Ctrl Pts',(-19.4686883835207,-67.9887339150381,
36.));
#34133=CARTESIAN_POINT('Ctrl Pts',(-21.6673174954184,-66.0013023234915,
34.8714803633902));
#34134=CARTESIAN_POINT('Ctrl Pts',(-21.6680517811035,-66.0867862312482,
34.8772098489549));
#34135=CARTESIAN_POINT('Ctrl Pts',(-21.6620451624345,-66.1721666114135,
34.8829393345197));
#34136=CARTESIAN_POINT('Ctrl Pts',(-21.6489385970892,-66.2564427278022,
34.8886688200844));
#34137=CARTESIAN_POINT('Ctrl Pts',(-21.5641972210077,-66.8013356028936,
34.9257131927483));
#34138=CARTESIAN_POINT('Ctrl Pts',(-21.1826528240559,-67.3000663249856,
34.9627575654121));
#34139=CARTESIAN_POINT('Ctrl Pts',(-20.678907038636,-67.5244143934905,34.999801938076));
#34140=CARTESIAN_POINT('Ctrl Pts',(-20.1751612532161,-67.7487624619954,
35.0368463107398));
#34141=CARTESIAN_POINT('Ctrl Pts',(-19.549214079328,-67.6987278769132,35.0738906834037));
#34142=CARTESIAN_POINT('Ctrl Pts',(-19.0875124433194,-67.3971905161154,
35.1109350560675));
#34143=CARTESIAN_POINT('Ctrl Pts',(-18.6258108073107,-67.0956531553176,
35.1479794287314));
#34144=CARTESIAN_POINT('Ctrl Pts',(-18.3283547091814,-66.5426130188043,
35.1850238013952));
#34145=CARTESIAN_POINT('Ctrl Pts',(-18.3312635585425,-65.9911859178142,
35.2220681740591));
#34146=CARTESIAN_POINT('Ctrl Pts',(-18.3341724079037,-65.4397588168241,
35.2591125467229));
#34147=CARTESIAN_POINT('Ctrl Pts',(-18.6374462047552,-64.8899447513572,
35.2961569193868));
#34148=CARTESIAN_POINT('Ctrl Pts',(-19.1023055859304,-64.5932821441991,
35.3332012920506));
#34149=CARTESIAN_POINT('Ctrl Pts',(-19.5671649671057,-64.296619537041,35.3702456647145));
#34150=CARTESIAN_POINT('Ctrl Pts',(-20.1936099326047,-64.2531083881916,
35.4072900373783));
#34151=CARTESIAN_POINT('Ctrl Pts',(-20.6949575817528,-64.4827944770596,
35.4443344100422));
#34152=CARTESIAN_POINT('Ctrl Pts',(-21.1963052309008,-64.7124805659277,
35.4813787827061));
#34153=CARTESIAN_POINT('Ctrl Pts',(-21.5725555636978,-65.2153638925131,
35.5184231553699));
#34154=CARTESIAN_POINT('Ctrl Pts',(-21.6515476257557,-65.7610474007137,
35.5554675280338));
#34155=CARTESIAN_POINT('Ctrl Pts',(-21.6629293534267,-65.8396732894808,
35.5608051398192));
#34156=CARTESIAN_POINT('Ctrl Pts',(-21.6681396849502,-65.9191877552933,
35.5661427516047));
#34157=CARTESIAN_POINT('Ctrl Pts',(-21.6674773009859,-65.998786811783,35.5714803633902));
#34158=CARTESIAN_POINT('Ctrl Pts',(-20.5301702171885,-67.9851743256717,
36.));
#34159=CARTESIAN_POINT('Ctrl Pts',(-21.190259562418,-67.8088876857537,35.9629556273362));
#34160=CARTESIAN_POINT('Ctrl Pts',(-22.3092726893092,-66.7486255815858,
35.8888668820085));
#34161=CARTESIAN_POINT('Ctrl Pts',(-21.8813252557512,-64.4618791315732,
35.7777337640169));
#34162=CARTESIAN_POINT('Ctrl Pts',(-19.7281828815708,-63.5871681688473,
35.6666006460254));
#34163=CARTESIAN_POINT('Ctrl Pts',(-17.825468300226,-64.9187027300962,35.5554675280337));
#34164=CARTESIAN_POINT('Ctrl Pts',(-17.9121446998427,-67.2409164611445,
35.4443344100422));
#34165=CARTESIAN_POINT('Ctrl Pts',(-19.9101226099192,-68.4268768260922,
35.3332012920507));
#34166=CARTESIAN_POINT('Ctrl Pts',(-21.9901521335571,-67.3919236495908,
35.2220681740591));
#34167=CARTESIAN_POINT('Ctrl Pts',(-22.2488202686706,-65.0828969400198,
35.1109350560676));
#34168=CARTESIAN_POINT('Ctrl Pts',(-20.4492273324997,-63.61330436034,34.9998019380759));
#34169=CARTESIAN_POINT('Ctrl Pts',(-18.2385100652431,-64.3280768123671,
34.8886688200844));
#34170=CARTESIAN_POINT('Ctrl Pts',(-17.6399645748577,-66.5730756011264,
34.7775357020929));
#34171=CARTESIAN_POINT('Ctrl Pts',(-19.2014229874425,-68.2935648037488,
34.6664025841013));
#34172=CARTESIAN_POINT('Ctrl Pts',(-21.4937672075293,-67.9148973568499,
34.5552694661097));
#34173=CARTESIAN_POINT('Ctrl Pts',(-22.4189585433245,-65.7836384066037,
34.4441363481182));
#34174=CARTESIAN_POINT('Ctrl Pts',(-21.1302229793561,-63.8504031421106,
34.3330032301266));
#34175=CARTESIAN_POINT('Ctrl Pts',(-18.8070632766386,-63.8845630078765,
34.221870112135));
#34176=CARTESIAN_POINT('Ctrl Pts',(-17.5757260074789,-65.8548543331223,
34.1107369941435));
#34177=CARTESIAN_POINT('Ctrl Pts',(-18.5631798196893,-67.9579885544186,
33.9996038761519));
#34178=CARTESIAN_POINT('Ctrl Pts',(-20.8656679609891,-68.2690946508119,
33.8884707581604));
#34179=CARTESIAN_POINT('Ctrl Pts',(-22.3758627384251,-66.5034359790957,
33.7773376401688));
#34180=CARTESIAN_POINT('Ctrl Pts',(-21.7115744113714,-64.2770129008106,
33.6662045221773));
#34181=CARTESIAN_POINT('Ctrl Pts',(-19.4807858227571,-63.6275354235162,
33.5550714041857));
#34182=CARTESIAN_POINT('Ctrl Pts',(-17.7252024818967,-65.1494309100778,
33.4439382861942));
#34183=CARTESIAN_POINT('Ctrl Pts',(-18.0516033664323,-67.4498007037218,
33.3328051682026));
#34184=CARTESIAN_POINT('Ctrl Pts',(-20.1612535373157,-68.4232558307668,
33.221672050211));
#34185=CARTESIAN_POINT('Ctrl Pts',(-22.1233181243905,-67.1788518425491,
33.1105389322194));
#34186=CARTESIAN_POINT('Ctrl Pts',(-22.1420383908254,-64.8555162491372,
32.9994058142279));
#34187=CARTESIAN_POINT('Ctrl Pts',(-20.2002808122731,-63.5796572308245,
32.8882726962363));
#34188=CARTESIAN_POINT('Ctrl Pts',(-18.0752183512995,-64.5189911786904,
32.7771395782448));
#34189=CARTESIAN_POINT('Ctrl Pts',(-17.7117918139106,-66.8138026917249,
32.6660064602532));
#34190=CARTESIAN_POINT('Ctrl Pts',(-19.442623471414,-68.3637899503476,32.5548733422617));
#34191=CARTESIAN_POINT('Ctrl Pts',(-21.6835880660123,-67.7503436085379,
32.4437402242701));
#34192=CARTESIAN_POINT('Ctrl Pts',(-22.3836665972123,-65.5349139033455,
32.3326071062786));
#34193=CARTESIAN_POINT('Ctrl Pts',(-20.9021196384422,-63.7451492994194,
32.221473988287));
#34194=CARTESIAN_POINT('Ctrl Pts',(-18.594917279486,-64.0191128067246,32.1103408702954));
#34195=CARTESIAN_POINT('Ctrl Pts',(-17.5737019298616,-66.106062240275,31.9992077523039));
#34196=CARTESIAN_POINT('Ctrl Pts',(-18.7731300721891,-68.0959393369569,
31.8880746343123));
#34197=CARTESIAN_POINT('Ctrl Pts',(-21.095437861579,-68.1675302570873,31.7769415163208));
#34198=CARTESIAN_POINT('Ctrl Pts',(-22.4151578040377,-66.2553121727719,
31.6658083983292));
#34199=CARTESIAN_POINT('Ctrl Pts',(-21.5244302645563,-64.1094223389464,
31.5546752803376));
#34200=CARTESIAN_POINT('Ctrl Pts',(-19.2384841459624,-63.6938635929289,
31.4435421623461));
#34201=CARTESIAN_POINT('Ctrl Pts',(-17.6495073099557,-65.3889716553072,
31.3324090443545));
#34202=CARTESIAN_POINT('Ctrl Pts',(-18.2117938983683,-67.6433169085898,
31.221275926363));
#34203=CARTESIAN_POINT('Ctrl Pts',(-20.4107170941006,-68.3936338468077,
31.1101428083714));
#34204=CARTESIAN_POINT('Ctrl Pts',(-22.2337358396447,-66.9532028759171,
30.9990096903798));
#34205=CARTESIAN_POINT('Ctrl Pts',(-22.0123516257601,-64.6403631152875,
30.8878765723883));
#34206=CARTESIAN_POINT('Ctrl Pts',(-19.9491839985917,-63.5719165463332,
30.7767434543967));
#34207=CARTESIAN_POINT('Ctrl Pts',(-17.9325251760105,-64.7257475226081,
30.6656103364052));
#34208=CARTESIAN_POINT('Ctrl Pts',(-17.8081006873606,-67.0458245202808,
30.5544772184136));
#34209=CARTESIAN_POINT('Ctrl Pts',(-19.6897887219546,-68.4087217537406,
30.443344100422));
#34210=CARTESIAN_POINT('Ctrl Pts',(-21.8553943280126,-67.5670620318125,
30.3322109824305));
#34211=CARTESIAN_POINT('Ctrl Pts',(-22.3228700174644,-65.2911654594091,
30.221077864439));
#34212=CARTESIAN_POINT('Ctrl Pts',(-20.6643636396598,-63.6640221580101,
30.1099447464473));
#34213=CARTESIAN_POINT('Ctrl Pts',(-18.3978055097405,-64.1748577207922,
29.9988116284558));
#34214=CARTESIAN_POINT('Ctrl Pts',(-17.5976388390673,-66.3561353344053,
29.8876785104642));
#34215=CARTESIAN_POINT('Ctrl Pts',(-18.9962076588936,-68.2114638726205,
29.7765453924727));
#34216=CARTESIAN_POINT('Ctrl Pts',(-21.313486738182,-68.0427736322436,29.6654122744811));
#34217=CARTESIAN_POINT('Ctrl Pts',(-22.4286110563519,-66.0044565608507,
29.5542791564895));
#34218=CARTESIAN_POINT('Ctrl Pts',(-21.320974946549,-63.9620606695586,29.4431460384981));
#34219=CARTESIAN_POINT('Ctrl Pts',(-19.004330572597,-63.784867065997,29.3320129205064));
#34220=CARTESIAN_POINT('Ctrl Pts',(-17.5989620477711,-65.6350503104176,
29.2208798025149));
#34221=CARTESIAN_POINT('Ctrl Pts',(-18.391117960758,-67.8192498750237,29.1097466845233));
#34222=CARTESIAN_POINT('Ctrl Pts',(-20.6557860410391,-68.3384003490309,
28.9986135665318));
#34223=CARTESIAN_POINT('Ctrl Pts',(-22.3202529250742,-66.7173547850641,
28.8874804485402));
#34224=CARTESIAN_POINT('Ctrl Pts',(-21.8611330078161,-64.4397578869974,
28.7763473305487));
#34225=CARTESIAN_POINT('Ctrl Pts',(-19.6986309083236,-63.5901559812818,
28.6652142125571));
#34226=CARTESIAN_POINT('Ctrl Pts',(-17.8119536633046,-64.9461381720334,
28.5540810945656));
#34227=CARTESIAN_POINT('Ctrl Pts',(-17.9278625462951,-67.2666561873374,
28.4429479765739));
#34228=CARTESIAN_POINT('Ctrl Pts',(-19.9402731854491,-68.4278806048883,
28.3318148585824));
#34229=CARTESIAN_POINT('Ctrl Pts',(-22.0073481561099,-67.3670131323966,
28.2206817405908));
#34230=CARTESIAN_POINT('Ctrl Pts',(-22.2372190858348,-65.0550014360215,
28.1095486225993));
#34231=CARTESIAN_POINT('Ctrl Pts',(-20.4194990521396,-63.6078896201836,
27.9984155046077));
#34232=CARTESIAN_POINT('Ctrl Pts',(-18.2178369745624,-64.3501313764944,
27.8872823866162));
#34233=CARTESIAN_POINT('Ctrl Pts',(-17.6472806432027,-66.6023978352466,
27.7761492686246));
#34234=CARTESIAN_POINT('Ctrl Pts',(-19.2300256691482,-68.3033260850074,
27.665016150633));
#34235=CARTESIAN_POINT('Ctrl Pts',(-21.5174815089169,-67.89615964379,27.5538830326415));
#34236=CARTESIAN_POINT('Ctrl Pts',(-22.4160785435702,-65.7535532643562,
27.4427499146499));
#34237=CARTESIAN_POINT('Ctrl Pts',(-21.1033854005481,-63.836504637639,27.3316167966584));
#34238=CARTESIAN_POINT('Ctrl Pts',(-18.7808305074767,-63.8995721204905,
27.2204836786668));
#34239=CARTESIAN_POINT('Ctrl Pts',(-17.5741075252728,-65.8850338715259,
27.1093505606753));
#34240=CARTESIAN_POINT('Ctrl Pts',(-18.5876568076359,-67.9757171467262,
26.9982174426837));
#34241=CARTESIAN_POINT('Ctrl Pts',(-20.8938381898737,-68.2581463290383,
26.8870843246921));
#34242=CARTESIAN_POINT('Ctrl Pts',(-22.3819436378662,-66.4738311047313,
26.7759512067006));
#34243=CARTESIAN_POINT('Ctrl Pts',(-21.6900005993275,-64.2558470165435,
26.664818088709));
#34244=CARTESIAN_POINT('Ctrl Pts',(-19.4513023285576,-63.6341803621276,
26.5536849707175));
#34245=CARTESIAN_POINT('Ctrl Pts',(-17.7147940941022,-65.1778050096466,
26.4425518527259));
#34246=CARTESIAN_POINT('Ctrl Pts',(-18.0697955898292,-67.4739347707333,
26.3314187347343));
#34247=CARTESIAN_POINT('Ctrl Pts',(-20.1913974492333,-68.4210616212703,
26.2202856167428));
#34248=CARTESIAN_POINT('Ctrl Pts',(-22.1378222071026,-67.1523371749621,
26.1091524987513));
#34249=CARTESIAN_POINT('Ctrl Pts',(-22.1276331663505,-64.8289492060639,
25.9980193807597));
#34250=CARTESIAN_POINT('Ctrl Pts',(-20.1701400827706,-63.5773513899392,
25.8868862627681));
#34251=CARTESIAN_POINT('Ctrl Pts',(-18.0569488868988,-64.5430601781429,
25.7757531447766));
#34252=CARTESIAN_POINT('Ctrl Pts',(-17.7220730992874,-66.842211172105,25.664620026785));
#34253=CARTESIAN_POINT('Ctrl Pts',(-19.4721283107045,-68.3705502400566,
25.5534869087934));
#34254=CARTESIAN_POINT('Ctrl Pts',(-21.7051476952021,-67.7292427278489,
25.4423537908019));
#34255=CARTESIAN_POINT('Ctrl Pts',(-22.3778773330212,-65.5053154469377,
25.3312206728103));
#34256=CARTESIAN_POINT('Ctrl Pts',(-20.8736249251117,-63.7340407352631,
25.2200875548188));
#34257=CARTESIAN_POINT('Ctrl Pts',(-18.5711036444345,-64.0368654665697,
25.1089544368272));
#34258=CARTESIAN_POINT('Ctrl Pts',(-17.573747567038,-66.1360134381725,24.9978213188356));
#34259=CARTESIAN_POINT('Ctrl Pts',(-18.8023455421979,-68.1115881261982,
24.8866882008441));
#34260=CARTESIAN_POINT('Ctrl Pts',(-20.343660854084,-68.1379171412778,24.8125994555164));
#34261=CARTESIAN_POINT('Ctrl Pts',(-20.9495535522615,-67.8221815534923,
24.7755550828525));
#34262=CARTESIAN_POINT('Ctrl Pts',(-20.4967348970876,-67.8599788000028,
36.0748149723825));
#34263=CARTESIAN_POINT('Ctrl Pts',(-21.1151955392376,-67.6948097220377,
36.0377705997186));
#34264=CARTESIAN_POINT('Ctrl Pts',(-22.1636378175943,-66.7014133181569,
35.9636818543909));
#34265=CARTESIAN_POINT('Ctrl Pts',(-21.7626789981897,-64.5588811168271,
35.8525487363994));
#34266=CARTESIAN_POINT('Ctrl Pts',(-19.7453250975402,-63.7393340242815,
35.7414156184078));
#34267=CARTESIAN_POINT('Ctrl Pts',(-17.9626056970361,-64.9868950184809,
35.6302825004163));
#34268=CARTESIAN_POINT('Ctrl Pts',(-18.0438158273823,-67.162657747713,35.5191493824247));
#34269=CARTESIAN_POINT('Ctrl Pts',(-19.9157907504706,-68.2738252194664,
35.4080162644331));
#34270=CARTESIAN_POINT('Ctrl Pts',(-21.864642681163,-67.3041416292674,35.2968831464415));
#34271=CARTESIAN_POINT('Ctrl Pts',(-22.1069978442969,-65.1407342786364,
35.1857500284501));
#34272=CARTESIAN_POINT('Ctrl Pts',(-20.4208966960866,-63.763821930185,35.0746169104584));
#34273=CARTESIAN_POINT('Ctrl Pts',(-18.3495988776918,-64.4335170750418,
34.9634837924669));
#34274=CARTESIAN_POINT('Ctrl Pts',(-17.7888008114678,-66.5369344420336,
34.8523506744753));
#34275=CARTESIAN_POINT('Ctrl Pts',(-19.2517854506183,-68.148920553847,34.7412175564838));
#34276=CARTESIAN_POINT('Ctrl Pts',(-21.3995623972236,-67.7941338661616,
34.6300844384922));
#34277=CARTESIAN_POINT('Ctrl Pts',(-22.266406305223,-65.797283305729,34.5189513205006));
#34278=CARTESIAN_POINT('Ctrl Pts',(-21.0589451786139,-63.9859680167513,
34.4078182025091));
#34279=CARTESIAN_POINT('Ctrl Pts',(-18.8822961356574,-64.0179735818617,
34.2966850845175));
#34280=CARTESIAN_POINT('Ctrl Pts',(-17.7286134657411,-65.86400798166,34.185551966526));
#34281=CARTESIAN_POINT('Ctrl Pts',(-18.6537932511848,-67.8345075063544,
34.0744188485344));
#34282=CARTESIAN_POINT('Ctrl Pts',(-20.811074390022,-68.1259936173523,33.9632857305429));
#34283=CARTESIAN_POINT('Ctrl Pts',(-22.226028348262,-66.4716866605454,33.8521526125513));
#34284=CARTESIAN_POINT('Ctrl Pts',(-21.6036335341486,-64.3856735221044,
33.7410194945598));
#34285=CARTESIAN_POINT('Ctrl Pts',(-19.5135301974017,-63.7771555077289,
33.6298863765682));
#34286=CARTESIAN_POINT('Ctrl Pts',(-17.868663168138,-65.2030722668864,33.5187532585766));
#34287=CARTESIAN_POINT('Ctrl Pts',(-18.1744794975593,-67.3583686522034,
33.4076201405851));
#34288=CARTESIAN_POINT('Ctrl Pts',(-20.1510840418164,-68.2704325831357,
33.2964870225935));
#34289=CARTESIAN_POINT('Ctrl Pts',(-21.9894105247868,-67.1045072501346,
33.185353904602));
#34290=CARTESIAN_POINT('Ctrl Pts',(-22.0069501928397,-64.9276934090752,
33.0742207866104));
#34291=CARTESIAN_POINT('Ctrl Pts',(-20.1876500517149,-63.7322967654826,
32.9630876686188));
#34292=CARTESIAN_POINT('Ctrl Pts',(-18.1966051973769,-64.612391378112,32.8519545506273));
#34293=CARTESIAN_POINT('Ctrl Pts',(-17.8560982473522,-66.7624800172052,
32.7408214326357));
#34294=CARTESIAN_POINT('Ctrl Pts',(-19.477774564489,-68.2147169336469,32.6296883146442));
#34295=CARTESIAN_POINT('Ctrl Pts',(-21.5774121548046,-67.6399577419979,
32.5185551966526));
#34296=CARTESIAN_POINT('Ctrl Pts',(-22.2333400547025,-65.5642446767688,
32.4074220786611));
#34297=CARTESIAN_POINT('Ctrl Pts',(-20.8452272331302,-63.8873520345212,
32.2962889606695));
#34298=CARTESIAN_POINT('Ctrl Pts',(-18.6835291799767,-64.1440379632945,
32.1851558426779));
#34299=CARTESIAN_POINT('Ctrl Pts',(-17.7267170370955,-66.0993733980141,
32.0740227246864));
#34300=CARTESIAN_POINT('Ctrl Pts',(-18.8505029374097,-67.9637583875726,
31.9628896066948));
#34301=CARTESIAN_POINT('Ctrl Pts',(-21.0263537931702,-68.0308344080476,
31.8517564887032));
#34302=CARTESIAN_POINT('Ctrl Pts',(-22.2628452605296,-66.2392108454141,
31.7406233707117));
#34303=CARTESIAN_POINT('Ctrl Pts',(-21.4282916807308,-64.2286521018105,
31.6294902527201));
#34304=CARTESIAN_POINT('Ctrl Pts',(-19.2865093377144,-63.8393006742038,
31.5183571347286));
#34305=CARTESIAN_POINT('Ctrl Pts',(-17.7977417315406,-65.4275063138625,
31.407224016737));
#34306=CARTESIAN_POINT('Ctrl Pts',(-18.3245675727016,-67.5396807082061,
31.2960908987455));
#34307=CARTESIAN_POINT('Ctrl Pts',(-20.3848151157039,-68.2426787171575,
31.1849577807539));
#34308=CARTESIAN_POINT('Ctrl Pts',(-22.0928647186386,-66.893088893192,31.0738246627623));
#34309=CARTESIAN_POINT('Ctrl Pts',(-21.8854421567226,-64.726108962541,30.9626915447708));
#34310=CARTESIAN_POINT('Ctrl Pts',(-19.952388722694,-63.725044249235,30.8515584267792));
#34311=CARTESIAN_POINT('Ctrl Pts',(-18.0629110036174,-64.806108580415,30.7404253087877));
#34312=CARTESIAN_POINT('Ctrl Pts',(-17.9463333771102,-66.9798693299075,
30.6292921907961));
#34313=CARTESIAN_POINT('Ctrl Pts',(-19.7093522754023,-68.2568151013876,
30.5181590728045));
#34314=CARTESIAN_POINT('Ctrl Pts',(-21.7383834110292,-67.468234864701,30.407025954813));
#34315=CARTESIAN_POINT('Ctrl Pts',(-22.1763776267779,-65.3358682906789,
30.2958928368214));
#34316=CARTESIAN_POINT('Ctrl Pts',(-20.6224653771108,-63.8113411969967,
30.1847597188298));
#34317=CARTESIAN_POINT('Ctrl Pts',(-18.4988483143134,-64.2899607845943,
30.0736266008383));
#34318=CARTESIAN_POINT('Ctrl Pts',(-17.749144359011,-66.3336755686187,29.9624934828467));
#34319=CARTESIAN_POINT('Ctrl Pts',(-19.0595120791564,-68.071997338901,29.8513603648552));
#34320=CARTESIAN_POINT('Ctrl Pts',(-21.2306513617017,-67.9139455916004,
29.7402272468636));
#34321=CARTESIAN_POINT('Ctrl Pts',(-22.275450080052,-66.0041755067028,29.6290941288721));
#34322=CARTESIAN_POINT('Ctrl Pts',(-21.2376673242963,-64.0905838337245,
29.5179610108805));
#34323=CARTESIAN_POINT('Ctrl Pts',(-19.0671227192333,-63.9245649900093,
29.406827892889));
#34324=CARTESIAN_POINT('Ctrl Pts',(-17.75038411922,-65.6580659557638,29.2956947748974));
#34325=CARTESIAN_POINT('Ctrl Pts',(-18.4925825173148,-67.7045184171959,
29.1845616569058));
#34326=CARTESIAN_POINT('Ctrl Pts',(-20.6144287269369,-68.1909285340192,
29.0734285389143));
#34327=CARTESIAN_POINT('Ctrl Pts',(-22.1739255819875,-66.6721146224013,
28.9622954209227));
#34328=CARTESIAN_POINT('Ctrl Pts',(-21.7437601795258,-64.5381549541881,
28.8511623029312));
#34329=CARTESIAN_POINT('Ctrl Pts',(-19.7176368270306,-63.7421334095621,
28.7400291849396));
#34330=CARTESIAN_POINT('Ctrl Pts',(-17.9499433641425,-65.0126002372679,
28.6288960669481));
#34331=CARTESIAN_POINT('Ctrl Pts',(-18.0585424238354,-67.1867741915022,
28.5177629489565));
#34332=CARTESIAN_POINT('Ctrl Pts',(-19.9440398722572,-68.2747656946963,
28.4066298309649));
#34333=CARTESIAN_POINT('Ctrl Pts',(-21.8807542321633,-67.2808021001998,
28.2954967129733));
#34334=CARTESIAN_POINT('Ctrl Pts',(-22.0961282930185,-65.1145980117196,
28.1843635949818));
#34335=CARTESIAN_POINT('Ctrl Pts',(-20.3930432373172,-63.7587486719991,
28.0732304769902));
#34336=CARTESIAN_POINT('Ctrl Pts',(-18.3302295407528,-64.4541807624518,
27.9620973589987));
#34337=CARTESIAN_POINT('Ctrl Pts',(-17.7956554900948,-66.564407461973,27.8509642410071));
#34338=CARTESIAN_POINT('Ctrl Pts',(-19.2785842968999,-68.1580662374109,
27.7398311230155));
#34339=CARTESIAN_POINT('Ctrl Pts',(-21.4217811501398,-67.7765778517597,
27.628698005024));
#34340=CARTESIAN_POINT('Ctrl Pts',(-22.2637079333885,-65.769095490658,27.5175648870324));
#34341=CARTESIAN_POINT('Ctrl Pts',(-21.0338001185652,-63.9729460250127,
27.4064317690409));
#34342=CARTESIAN_POINT('Ctrl Pts',(-18.85771774278,-64.0320361409567,27.2952986510493));
#34343=CARTESIAN_POINT('Ctrl Pts',(-17.7270970535285,-65.8922842397695,
27.1841655330578));
#34344=CARTESIAN_POINT('Ctrl Pts',(-18.6767265916375,-67.8511180404618,
27.0730324150662));
#34345=CARTESIAN_POINT('Ctrl Pts',(-20.8374680562299,-68.1157357542866,
26.9618992970746));
#34346=CARTESIAN_POINT('Ctrl Pts',(-22.2317257542274,-66.4439488251411,
26.8507661790831));
#34347=CARTESIAN_POINT('Ctrl Pts',(-21.5834202800691,-64.3658424697322,
26.7396330610915));
#34348=CARTESIAN_POINT('Ctrl Pts',(-19.4859060872912,-63.7833813815903,
26.6284999431));
#34349=CARTESIAN_POINT('Ctrl Pts',(-17.858911187977,-65.2296569466219,26.5173668251084));
#34350=CARTESIAN_POINT('Ctrl Pts',(-18.1915244237431,-67.3809806981174,
26.4062337071169));
#34351=CARTESIAN_POINT('Ctrl Pts',(-20.1793269202331,-68.2683767520211,
26.2951005891253));
#34352=CARTESIAN_POINT('Ctrl Pts',(-22.0029999038198,-67.0796647368282,
26.1839674711337));
#34353=CARTESIAN_POINT('Ctrl Pts',(-21.993453437524,-64.902801823356,26.0728343531422));
#34354=CARTESIAN_POINT('Ctrl Pts',(-20.1594101550134,-63.7301363430416,
25.9617012351506));
#34355=CARTESIAN_POINT('Ctrl Pts',(-18.1794879014128,-64.634942459969,25.8505681171591));
#34356=CARTESIAN_POINT('Ctrl Pts',(-17.8657311408418,-66.7890969095174,
25.7394349991675));
#34357=CARTESIAN_POINT('Ctrl Pts',(-19.5054186735571,-68.2210508839594,
25.6283018811759));
#34358=CARTESIAN_POINT('Ctrl Pts',(-21.5976121204752,-67.6201875937367,
25.5171687631844));
#34359=CARTESIAN_POINT('Ctrl Pts',(-22.2279158919356,-65.5365128545709,
25.4060356451928));
#34360=CARTESIAN_POINT('Ctrl Pts',(-20.8185295461707,-63.8769440347993,
25.2949025272013));
#34361=CARTESIAN_POINT('Ctrl Pts',(-18.6612173578994,-64.1606710471141,
25.1837694092097));
#34362=CARTESIAN_POINT('Ctrl Pts',(-17.7267597961517,-66.1274357159696,
25.0726362912181));
#34363=CARTESIAN_POINT('Ctrl Pts',(-18.8778759263437,-67.9784202819252,
24.9615031732266));
#34364=CARTESIAN_POINT('Ctrl Pts',(-20.3219877945836,-68.003088850947,24.8874144278989));
#34365=CARTESIAN_POINT('Ctrl Pts',(-20.8896697150645,-67.7072652086133,
24.850370055235));
#34366=CARTESIAN_POINT('Ctrl Pts',(-20.4632995769867,-67.7347832743338,
36.149629944765));
#34367=CARTESIAN_POINT('Ctrl Pts',(-21.0401315160572,-67.5807317583216,
36.1125855721011));
#34368=CARTESIAN_POINT('Ctrl Pts',(-22.0180029458793,-66.654201054728,36.0384968267735));
#34369=CARTESIAN_POINT('Ctrl Pts',(-21.6440327406283,-64.6558831020808,
35.9273637087818));
#34370=CARTESIAN_POINT('Ctrl Pts',(-19.7624673135096,-63.8914998797159,
35.8162305907903));
#34371=CARTESIAN_POINT('Ctrl Pts',(-18.0997430938463,-65.0550873068655,
35.7050974727987));
#34372=CARTESIAN_POINT('Ctrl Pts',(-18.1754869549219,-67.0843990342815,
35.5939643548072));
#34373=CARTESIAN_POINT('Ctrl Pts',(-19.921458891022,-68.1207736128406,35.4828312368156));
#34374=CARTESIAN_POINT('Ctrl Pts',(-21.7391332287689,-67.2163596089439,
35.3716981188241));
#34375=CARTESIAN_POINT('Ctrl Pts',(-21.9651754199231,-65.198571617253,35.2605650008325));
#34376=CARTESIAN_POINT('Ctrl Pts',(-20.3925660596736,-63.9143395000302,
35.149431882841));
#34377=CARTESIAN_POINT('Ctrl Pts',(-18.4606876901404,-64.5389573377165,
35.0382987648494));
#34378=CARTESIAN_POINT('Ctrl Pts',(-17.937637048078,-66.5007932829407,34.9271656468579));
#34379=CARTESIAN_POINT('Ctrl Pts',(-19.3021479137942,-68.0042763039452,
34.8160325288662));
#34380=CARTESIAN_POINT('Ctrl Pts',(-21.3053575869179,-67.6733703754733,
34.7048994108748));
#34381=CARTESIAN_POINT('Ctrl Pts',(-22.1138540671214,-65.8109282048542,
34.5937662928831));
#34382=CARTESIAN_POINT('Ctrl Pts',(-20.9876673778718,-64.1215328913922,
34.4826331748916));
#34383=CARTESIAN_POINT('Ctrl Pts',(-18.9575289946762,-64.1513841558468,
34.3715000569001));
#34384=CARTESIAN_POINT('Ctrl Pts',(-17.8815009240032,-65.8731616301978,
34.2603669389085));
#34385=CARTESIAN_POINT('Ctrl Pts',(-18.7444066826802,-67.71102645829,34.1492338209169));
#34386=CARTESIAN_POINT('Ctrl Pts',(-20.7564808190548,-67.9828925838928,
34.0381007029253));
#34387=CARTESIAN_POINT('Ctrl Pts',(-22.0761939580989,-66.4399373419952,
33.9269675849338));
#34388=CARTESIAN_POINT('Ctrl Pts',(-21.4956926569258,-64.4943341433981,
33.8158344669422));
#34389=CARTESIAN_POINT('Ctrl Pts',(-19.5462745720463,-63.9267755919416,
33.7047013489507));
#34390=CARTESIAN_POINT('Ctrl Pts',(-18.0121238543792,-65.2567136236949,
33.5935682309591));
#34391=CARTESIAN_POINT('Ctrl Pts',(-18.2973556286862,-67.2669366006852,
33.4824351129676));
#34392=CARTESIAN_POINT('Ctrl Pts',(-20.1409145463171,-68.1176093355045,
33.371301994976));
#34393=CARTESIAN_POINT('Ctrl Pts',(-21.8555029251832,-67.0301626577201,
33.2601688769845));
#34394=CARTESIAN_POINT('Ctrl Pts',(-21.871861994854,-64.9998705690132,33.1490357589928));
#34395=CARTESIAN_POINT('Ctrl Pts',(-20.1750192911566,-63.8849363001409,
33.0379026410013));
#34396=CARTESIAN_POINT('Ctrl Pts',(-18.3179920434542,-64.7057915775334,
32.9267695230098));
#34397=CARTESIAN_POINT('Ctrl Pts',(-18.0004046807938,-66.7111573426855,
32.8156364050182));
#34398=CARTESIAN_POINT('Ctrl Pts',(-19.5129256575641,-68.065643916946,32.7045032870266));
#34399=CARTESIAN_POINT('Ctrl Pts',(-21.4712362435969,-67.529571875458,32.5933701690351));
#34400=CARTESIAN_POINT('Ctrl Pts',(-22.0830135121926,-65.5935754501919,
32.4822370510435));
#34401=CARTESIAN_POINT('Ctrl Pts',(-20.7883348278182,-64.029554769623,32.3711039330519));
#34402=CARTESIAN_POINT('Ctrl Pts',(-18.7721410804674,-64.2689631198643,
32.2599708150604));
#34403=CARTESIAN_POINT('Ctrl Pts',(-17.8797321443293,-66.0926845557532,
32.1488376970689));
#34404=CARTESIAN_POINT('Ctrl Pts',(-18.9278758026304,-67.8315774381883,
32.0377045790773));
#34405=CARTESIAN_POINT('Ctrl Pts',(-20.9572697247615,-67.894138559008,31.9265714610857));
#34406=CARTESIAN_POINT('Ctrl Pts',(-22.1105327170215,-66.2231095180563,
31.8154383430942));
#34407=CARTESIAN_POINT('Ctrl Pts',(-21.3321530969053,-64.3478818646744,
31.7043052251026));
#34408=CARTESIAN_POINT('Ctrl Pts',(-19.3345345294663,-63.9847377554787,
31.593172107111));
#34409=CARTESIAN_POINT('Ctrl Pts',(-17.9459761531255,-65.4660409724177,
31.4820389891195));
#34410=CARTESIAN_POINT('Ctrl Pts',(-18.437341247035,-67.4360445078226,31.3709058711279));
#34411=CARTESIAN_POINT('Ctrl Pts',(-20.3589131373073,-68.0917235875072,
31.2597727531364));
#34412=CARTESIAN_POINT('Ctrl Pts',(-21.9519935976325,-66.832974910467,31.1486396351448));
#34413=CARTESIAN_POINT('Ctrl Pts',(-21.7585326876851,-64.8118548097944,
31.0375065171533));
#34414=CARTESIAN_POINT('Ctrl Pts',(-19.9555934467963,-63.8781719521369,
30.9263733991617));
#34415=CARTESIAN_POINT('Ctrl Pts',(-18.1932968312243,-64.8864696382219,
30.8152402811701));
#34416=CARTESIAN_POINT('Ctrl Pts',(-18.0845660668597,-66.913914139534,30.7041071631786));
#34417=CARTESIAN_POINT('Ctrl Pts',(-19.72891582885,-68.1049084490347,30.592974045187));
#34418=CARTESIAN_POINT('Ctrl Pts',(-21.6213724940458,-67.3694076975895,
30.4818409271954));
#34419=CARTESIAN_POINT('Ctrl Pts',(-22.0298852360914,-65.3805711219487,
30.3707078092039));
#34420=CARTESIAN_POINT('Ctrl Pts',(-20.5805671145618,-63.9586602359834,
30.2595746912123));
#34421=CARTESIAN_POINT('Ctrl Pts',(-18.5998911188863,-64.4050638483964,
30.1484415732208));
#34422=CARTESIAN_POINT('Ctrl Pts',(-17.9006498789546,-66.3112158028321,
30.0373084552292));
#34423=CARTESIAN_POINT('Ctrl Pts',(-19.1228164994193,-67.9325308051813,
29.9261753372377));
#34424=CARTESIAN_POINT('Ctrl Pts',(-21.1478159852215,-67.7851175509572,
29.8150422192461));
#34425=CARTESIAN_POINT('Ctrl Pts',(-22.1222891037521,-66.003894452555,29.7039091012546));
#34426=CARTESIAN_POINT('Ctrl Pts',(-21.1543597020436,-64.2191069978902,
29.592775983263));
#34427=CARTESIAN_POINT('Ctrl Pts',(-19.1299148658697,-64.0642629140219,
29.4816428652715));
#34428=CARTESIAN_POINT('Ctrl Pts',(-17.9018061906689,-65.68108160111,29.3705097472798));
#34429=CARTESIAN_POINT('Ctrl Pts',(-18.5940470738716,-67.589786959368,29.2593766292883));
#34430=CARTESIAN_POINT('Ctrl Pts',(-20.5730714128348,-68.0434567190076,
29.1482435112967));
#34431=CARTESIAN_POINT('Ctrl Pts',(-22.0275982389007,-66.6268744597386,
29.0371103933052));
#34432=CARTESIAN_POINT('Ctrl Pts',(-21.6263873512355,-64.6365520213787,
28.9259772753136));
#34433=CARTESIAN_POINT('Ctrl Pts',(-19.7366427457375,-63.8941108378424,
28.8148441573221));
#34434=CARTESIAN_POINT('Ctrl Pts',(-18.0879330649805,-65.0790623025024,
28.7037110393305));
#34435=CARTESIAN_POINT('Ctrl Pts',(-18.1892223013757,-67.106892195667,28.592577921339));
#34436=CARTESIAN_POINT('Ctrl Pts',(-19.9478065590653,-68.1216507845045,
28.4814448033474));
#34437=CARTESIAN_POINT('Ctrl Pts',(-21.7541603082167,-67.194591068003,28.3703116853558));
#34438=CARTESIAN_POINT('Ctrl Pts',(-21.9550375002021,-65.1741945874176,
28.2591785673643));
#34439=CARTESIAN_POINT('Ctrl Pts',(-20.3665874224948,-63.9096077238146,
28.1480454493727));
#34440=CARTESIAN_POINT('Ctrl Pts',(-18.4426221069431,-64.5582301484091,
28.0369123313812));
#34441=CARTESIAN_POINT('Ctrl Pts',(-17.9440303369869,-66.5264170886993,
27.9257792133896));
#34442=CARTESIAN_POINT('Ctrl Pts',(-19.3271429246517,-68.0128063898144,
27.814646095398));
#34443=CARTESIAN_POINT('Ctrl Pts',(-21.3260807913628,-67.6569960597292,
27.7035129774065));
#34444=CARTESIAN_POINT('Ctrl Pts',(-22.1113373232067,-65.78463771696,27.5923798594149));
#34445=CARTESIAN_POINT('Ctrl Pts',(-20.9642148365823,-64.1093874123863,
27.4812467414234));
#34446=CARTESIAN_POINT('Ctrl Pts',(-18.9346049780834,-64.164500161423,27.3701136234318));
#34447=CARTESIAN_POINT('Ctrl Pts',(-17.8800865817842,-65.8995346080128,
27.2589805054402));
#34448=CARTESIAN_POINT('Ctrl Pts',(-18.765796375639,-67.7265189341975,27.1478473874487));
#34449=CARTESIAN_POINT('Ctrl Pts',(-20.7810979225862,-67.9733251795348,
27.0367142694571));
#34450=CARTESIAN_POINT('Ctrl Pts',(-22.0815078705886,-66.4140665455509,
26.9255811514656));
#34451=CARTESIAN_POINT('Ctrl Pts',(-21.4768399608107,-64.4758379229209,
26.814448033474));
#34452=CARTESIAN_POINT('Ctrl Pts',(-19.5205098460247,-63.932582401053,26.7033149154824));
#34453=CARTESIAN_POINT('Ctrl Pts',(-18.0030282818518,-65.2815088835971,
26.5921817974909));
#34454=CARTESIAN_POINT('Ctrl Pts',(-18.313253257657,-67.2880266255015,26.4810486794993));
#34455=CARTESIAN_POINT('Ctrl Pts',(-20.1672563912329,-68.115691882772,26.3699155615078));
#34456=CARTESIAN_POINT('Ctrl Pts',(-21.868177600537,-67.0069922986945,26.2587824435162));
#34457=CARTESIAN_POINT('Ctrl Pts',(-21.8592737086975,-64.976654440648,26.1476493255247));
#34458=CARTESIAN_POINT('Ctrl Pts',(-20.1486802272563,-63.882921296144,26.0365162075331));
#34459=CARTESIAN_POINT('Ctrl Pts',(-18.3020269159268,-64.7268247417951,
25.9253830895415));
#34460=CARTESIAN_POINT('Ctrl Pts',(-18.0093891823963,-66.7359826469298,
25.81424997155));
#34461=CARTESIAN_POINT('Ctrl Pts',(-19.5387090364096,-68.0715515278622,
25.7031168535584));
#34462=CARTESIAN_POINT('Ctrl Pts',(-21.4900765457484,-67.5111324596245,
25.5919837355669));
#34463=CARTESIAN_POINT('Ctrl Pts',(-22.07795445085,-65.5677102622041,25.4808506175753));
#34464=CARTESIAN_POINT('Ctrl Pts',(-20.7634341672297,-64.0198473343356,
25.3697174995838));
#34465=CARTESIAN_POINT('Ctrl Pts',(-18.7513310713643,-64.2844766276586,
25.2585843815922));
#34466=CARTESIAN_POINT('Ctrl Pts',(-17.8797720252654,-66.1188579937667,
25.1474512636006));
#34467=CARTESIAN_POINT('Ctrl Pts',(-18.9534063104895,-67.8452524376522,
25.0363181456091));
#34468=CARTESIAN_POINT('Ctrl Pts',(-20.3003147350832,-67.8682605606162,
24.9622294002814));
#34469=CARTESIAN_POINT('Ctrl Pts',(-20.8297858778675,-67.5923488637344,
24.9251850276175));
#34470=CARTESIAN_POINT('Ctrl Pts',(-20.4298642568858,-67.6095877486649,
36.2244449171475));
#34471=CARTESIAN_POINT('Ctrl Pts',(-20.9650674928767,-67.4666537946055,
36.1874005444836));
#34472=CARTESIAN_POINT('Ctrl Pts',(-21.8723680741644,-66.6069887912992,
36.113311799156));
#34473=CARTESIAN_POINT('Ctrl Pts',(-21.5253864830668,-64.7528850873347,
36.0021786811643));
#34474=CARTESIAN_POINT('Ctrl Pts',(-19.779609529479,-64.04366573515,35.8910455631728));
#34475=CARTESIAN_POINT('Ctrl Pts',(-18.2368804906565,-65.1232795952502,
35.7799124451812));
#34476=CARTESIAN_POINT('Ctrl Pts',(-18.3071580824616,-67.0061403208501,
35.6687793271897));
#34477=CARTESIAN_POINT('Ctrl Pts',(-19.9271270315734,-67.9677220062147,
35.5576462091981));
#34478=CARTESIAN_POINT('Ctrl Pts',(-21.6136237763748,-67.1285775886206,
35.4465130912065));
#34479=CARTESIAN_POINT('Ctrl Pts',(-21.8233529955495,-65.2564089558696,
35.335379973215));
#34480=CARTESIAN_POINT('Ctrl Pts',(-20.3642354232605,-64.0648570698753,
35.2242468552234));
#34481=CARTESIAN_POINT('Ctrl Pts',(-18.5717765025891,-64.6443976003911,
35.1131137372319));
#34482=CARTESIAN_POINT('Ctrl Pts',(-18.0864732846881,-66.4646521238479,
35.0019806192403));
#34483=CARTESIAN_POINT('Ctrl Pts',(-19.35251037697,-67.8596320540434,34.8908475012488));
#34484=CARTESIAN_POINT('Ctrl Pts',(-21.2111527766122,-67.552606884785,34.7797143832572));
#34485=CARTESIAN_POINT('Ctrl Pts',(-21.9613018290199,-65.8245731039795,
34.6685812652656));
#34486=CARTESIAN_POINT('Ctrl Pts',(-20.9163895771297,-64.2570977660329,
34.5574481472741));
#34487=CARTESIAN_POINT('Ctrl Pts',(-19.0327618536951,-64.284794729832,34.4463150292825));
#34488=CARTESIAN_POINT('Ctrl Pts',(-18.0343883822654,-65.8823152787355,
34.335181911291));
#34489=CARTESIAN_POINT('Ctrl Pts',(-18.8350201141757,-67.5875454102258,
34.2240487932994));
#34490=CARTESIAN_POINT('Ctrl Pts',(-20.7018872480875,-67.8397915504332,
34.1129156753078));
#34491=CARTESIAN_POINT('Ctrl Pts',(-21.9263595679359,-66.4081880234449,
34.0017825573163));
#34492=CARTESIAN_POINT('Ctrl Pts',(-21.387751779703,-64.6029947646918,33.8906494393247));
#34493=CARTESIAN_POINT('Ctrl Pts',(-19.579018946691,-64.0763956761543,33.7795163213332));
#34494=CARTESIAN_POINT('Ctrl Pts',(-18.1555845406205,-65.3103549805034,
33.6683832033416));
#34495=CARTESIAN_POINT('Ctrl Pts',(-18.4202317598132,-67.1755045491668,
33.5572500853501));
#34496=CARTESIAN_POINT('Ctrl Pts',(-20.1307450508178,-67.9647860878732,
33.4461169673584));
#34497=CARTESIAN_POINT('Ctrl Pts',(-21.7215953255795,-66.9558180653057,
33.334983849367));
#34498=CARTESIAN_POINT('Ctrl Pts',(-21.7367737968683,-65.0720477289512,
33.2238507313753));
#34499=CARTESIAN_POINT('Ctrl Pts',(-20.1623885305984,-64.0375758347992,
33.1127176133839));
#34500=CARTESIAN_POINT('Ctrl Pts',(-18.4393788895316,-64.7991917769549,
33.0015844953922));
#34501=CARTESIAN_POINT('Ctrl Pts',(-18.1447111142353,-66.6598346681659,
32.8904513774007));
#34502=CARTESIAN_POINT('Ctrl Pts',(-19.5480767506391,-67.9165709002453,
32.7793182594091));
#34503=CARTESIAN_POINT('Ctrl Pts',(-21.3650603323891,-67.419186008918,32.6681851414176));
#34504=CARTESIAN_POINT('Ctrl Pts',(-21.9326869696828,-65.6229062236153,
32.557052023426));
#34505=CARTESIAN_POINT('Ctrl Pts',(-20.7314424225063,-64.1717575047246,
32.4459189054345));
#34506=CARTESIAN_POINT('Ctrl Pts',(-18.8607529809581,-64.3938882764342,
32.3347857874429));
#34507=CARTESIAN_POINT('Ctrl Pts',(-18.0327472515632,-66.0859957134922,
32.2236526694514));
#34508=CARTESIAN_POINT('Ctrl Pts',(-19.0052486678511,-67.699396488804,32.1125195514597));
#34509=CARTESIAN_POINT('Ctrl Pts',(-20.8881856563527,-67.7574427099684,
32.0013864334682));
#34510=CARTESIAN_POINT('Ctrl Pts',(-21.9582201735135,-66.2070081906986,
31.8902533154767));
#34511=CARTESIAN_POINT('Ctrl Pts',(-21.2360145130798,-64.4671116275385,
31.7791201974851));
#34512=CARTESIAN_POINT('Ctrl Pts',(-19.3825597212183,-64.1301748367536,
31.6679870794935));
#34513=CARTESIAN_POINT('Ctrl Pts',(-18.0942105747104,-65.5045756309731,
31.556853961502));
#34514=CARTESIAN_POINT('Ctrl Pts',(-18.5501149213683,-67.3324083074391,
31.4457208435104));
#34515=CARTESIAN_POINT('Ctrl Pts',(-20.3330111589106,-67.940768457857,31.3345877255189));
#34516=CARTESIAN_POINT('Ctrl Pts',(-21.8111224766264,-66.772860927742,31.2234546075273));
#34517=CARTESIAN_POINT('Ctrl Pts',(-21.6316232186476,-64.8976006570478,
31.1123214895357));
#34518=CARTESIAN_POINT('Ctrl Pts',(-19.9587981708986,-64.0312996550389,
31.0011883715442));
#34519=CARTESIAN_POINT('Ctrl Pts',(-18.3236826588312,-64.9668306960287,
30.8900552535526));
#34520=CARTESIAN_POINT('Ctrl Pts',(-18.2227987566092,-66.8479589491607,
30.7789221355611));
#34521=CARTESIAN_POINT('Ctrl Pts',(-19.7484793822977,-67.9530017966818,
30.6677890175695));
#34522=CARTESIAN_POINT('Ctrl Pts',(-21.5043615770624,-67.2705805304779,
30.5566558995779));
#34523=CARTESIAN_POINT('Ctrl Pts',(-21.8833928454049,-65.4252739532185,
30.4455227815864));
#34524=CARTESIAN_POINT('Ctrl Pts',(-20.5386688520128,-64.1059792749701,
30.3343896635948));
#34525=CARTESIAN_POINT('Ctrl Pts',(-18.7009339234592,-64.5201669121985,
30.2232565456033));
#34526=CARTESIAN_POINT('Ctrl Pts',(-18.0521553988983,-66.2887560370454,
30.1121234276117));
#34527=CARTESIAN_POINT('Ctrl Pts',(-19.186120919682,-67.7930642714616,30.0009903096201));
#34528=CARTESIAN_POINT('Ctrl Pts',(-21.0649806087413,-67.6562895103141,
29.8898571916286));
#34529=CARTESIAN_POINT('Ctrl Pts',(-21.9691281274522,-66.0036133984072,
29.778724073637));
#34530=CARTESIAN_POINT('Ctrl Pts',(-21.071052079791,-64.347630162056,29.6675909556455));
#34531=CARTESIAN_POINT('Ctrl Pts',(-19.192707012506,-64.2039608380343,29.5564578376539));
#34532=CARTESIAN_POINT('Ctrl Pts',(-18.0532282621179,-65.704097246456,29.4453247196623));
#34533=CARTESIAN_POINT('Ctrl Pts',(-18.6955116304284,-67.4750555015402,
29.3341916016708));
#34534=CARTESIAN_POINT('Ctrl Pts',(-20.5317140987327,-67.8959849039958,
29.2230584836792));
#34535=CARTESIAN_POINT('Ctrl Pts',(-21.8812708958139,-66.581634297076,29.1119253656877));
#34536=CARTESIAN_POINT('Ctrl Pts',(-21.5090145229452,-64.7349490885693,
29.0007922476961));
#34537=CARTESIAN_POINT('Ctrl Pts',(-19.7556486644444,-64.0460882661226,
28.8896591297046));
#34538=CARTESIAN_POINT('Ctrl Pts',(-18.2259227658184,-65.145524367737,28.778526011713));
#34539=CARTESIAN_POINT('Ctrl Pts',(-18.319902178916,-67.0270101998317,28.6673928937214));
#34540=CARTESIAN_POINT('Ctrl Pts',(-19.9515732458733,-67.9685358743126,
28.5562597757299));
#34541=CARTESIAN_POINT('Ctrl Pts',(-21.6275663842701,-67.1083800358061,
28.4451266577383));
#34542=CARTESIAN_POINT('Ctrl Pts',(-21.8139467073857,-65.2337911631157,
28.3339935397468));
#34543=CARTESIAN_POINT('Ctrl Pts',(-20.3401316076723,-64.0604667756301,
28.2228604217552));
#34544=CARTESIAN_POINT('Ctrl Pts',(-18.5550146731335,-64.6622795343665,
28.1117273037637));
#34545=CARTESIAN_POINT('Ctrl Pts',(-18.0924051838791,-66.4884267154256,
28.0005941857721));
#34546=CARTESIAN_POINT('Ctrl Pts',(-19.3757015524034,-67.867546542218,27.8894610677805));
#34547=CARTESIAN_POINT('Ctrl Pts',(-21.2303804325857,-67.5374142676988,
27.778327949789));
#34548=CARTESIAN_POINT('Ctrl Pts',(-21.958966713025,-65.8001799432619,27.6671948317974));
#34549=CARTESIAN_POINT('Ctrl Pts',(-20.8946295545994,-64.2458287997599,
27.5560617138058));
#34550=CARTESIAN_POINT('Ctrl Pts',(-19.0114922133866,-64.2969641818893,
27.4449285958143));
#34551=CARTESIAN_POINT('Ctrl Pts',(-18.03307611004,-65.9067849762562,27.3337954778227));
#34552=CARTESIAN_POINT('Ctrl Pts',(-18.8548661596405,-67.6019198279331,
27.2226623598312));
#34553=CARTESIAN_POINT('Ctrl Pts',(-20.7247277889425,-67.830914604783,27.1115292418396));
#34554=CARTESIAN_POINT('Ctrl Pts',(-21.9312899869498,-66.3841842659606,
27.0003961238481));
#34555=CARTESIAN_POINT('Ctrl Pts',(-21.3702596415523,-64.5858333761097,
26.8892630058565));
#34556=CARTESIAN_POINT('Ctrl Pts',(-19.5551136047582,-64.0817834205157,
26.7781298878649));
#34557=CARTESIAN_POINT('Ctrl Pts',(-18.1471453757266,-65.3333608205724,
26.6669967698734));
#34558=CARTESIAN_POINT('Ctrl Pts',(-18.4349820915709,-67.1950725528856,
26.5558636518818));
#34559=CARTESIAN_POINT('Ctrl Pts',(-20.1551858622327,-67.9630070135229,
26.4447305338903));
#34560=CARTESIAN_POINT('Ctrl Pts',(-21.7333552972541,-66.9343198605606,
26.3335974158987));
#34561=CARTESIAN_POINT('Ctrl Pts',(-21.725093979871,-65.0505070579402,26.2224642979072));
#34562=CARTESIAN_POINT('Ctrl Pts',(-20.1379502994991,-64.0357062492462,
26.1113311799156));
#34563=CARTESIAN_POINT('Ctrl Pts',(-18.4245659304409,-64.8187070236213,
26.000198061924));
#34564=CARTESIAN_POINT('Ctrl Pts',(-18.1530472239507,-66.6828683843421,
25.8890649439325));
#34565=CARTESIAN_POINT('Ctrl Pts',(-19.5719993992621,-67.922052171765,25.7779318259409));
#34566=CARTESIAN_POINT('Ctrl Pts',(-21.3825409710216,-67.4020773255123,
25.6667987079494));
#34567=CARTESIAN_POINT('Ctrl Pts',(-21.9279930097644,-65.5989076698373,
25.5556655899578));
#34568=CARTESIAN_POINT('Ctrl Pts',(-20.7083387882887,-64.162750633872,25.4445324719662));
#34569=CARTESIAN_POINT('Ctrl Pts',(-18.8414447848292,-64.408282208203,25.3333993539747));
#34570=CARTESIAN_POINT('Ctrl Pts',(-18.032784254379,-66.1102802715637,25.2222662359831));
#34571=CARTESIAN_POINT('Ctrl Pts',(-19.0289366946352,-67.7120845933793,
25.1111331179916));
#34572=CARTESIAN_POINT('Ctrl Pts',(-20.2786416755829,-67.7334322702853,
25.0370443726639));
#34573=CARTESIAN_POINT('Ctrl Pts',(-20.7699020406705,-67.4774325188554,
25.));
#34574=CARTESIAN_POINT('Ctrl Pts',(-21.6638441630143,-65.999055839902,35.3785196366098));
#34575=CARTESIAN_POINT('Ctrl Pts',(-21.664963066366,-65.7833631633576,35.3641397488116));
#34576=CARTESIAN_POINT('Ctrl Pts',(-21.6260431435441,-65.5680576298417,
35.3497598610133));
#34577=CARTESIAN_POINT('Ctrl Pts',(-21.5452118636389,-65.369845080329,35.335379973215));
#34578=CARTESIAN_POINT('Ctrl Pts',(-21.3369804714531,-64.8592249938715,
35.2983356005512));
#34579=CARTESIAN_POINT('Ctrl Pts',(-20.8506079473568,-64.4620410318734,
35.2612912278873));
#34580=CARTESIAN_POINT('Ctrl Pts',(-20.3086785318634,-64.3600391392936,
35.2242468552234));
#34581=CARTESIAN_POINT('Ctrl Pts',(-19.76674911637,-64.2580372467139,35.1872024825596));
#34582=CARTESIAN_POINT('Ctrl Pts',(-19.1692628094796,-64.4512174235525,
35.1501581098957));
#34583=CARTESIAN_POINT('Ctrl Pts',(-18.7896357863842,-64.8511832658813,
35.1131137372319));
#34584=CARTESIAN_POINT('Ctrl Pts',(-18.4100087632888,-65.2511491082101,
35.076069364568));
#34585=CARTESIAN_POINT('Ctrl Pts',(-18.2482410239884,-65.857900616029,35.0390249919042));
#34586=CARTESIAN_POINT('Ctrl Pts',(-18.3783633363853,-66.393773024971,35.0019806192403));
#34587=CARTESIAN_POINT('Ctrl Pts',(-18.5084856487821,-66.9296454339131,
34.9649362465765));
#34588=CARTESIAN_POINT('Ctrl Pts',(-18.9304980128761,-67.3946387439782,
34.9278918739126));
#34589=CARTESIAN_POINT('Ctrl Pts',(-19.4512779281967,-67.5759645374677,
34.8908475012488));
#34590=CARTESIAN_POINT('Ctrl Pts',(-19.9720578435174,-67.7572903309572,
34.8538031285849));
#34591=CARTESIAN_POINT('Ctrl Pts',(-20.5916053100648,-67.6549486078711,
34.8167587559211));
#34592=CARTESIAN_POINT('Ctrl Pts',(-21.0264038854064,-67.3157721161938,
34.7797143832572));
#34593=CARTESIAN_POINT('Ctrl Pts',(-21.4223194546762,-67.0069273742812,
34.7459828010414));
#34594=CARTESIAN_POINT('Ctrl Pts',(-21.6650519511804,-66.5017129689095,
34.7122512188256));
#34595=CARTESIAN_POINT('Ctrl Pts',(-21.668208945928,-65.9991411290017,34.6785196366098));
#34596=CARTESIAN_POINT('Ctrl Pts',(-20.5301702171885,-67.9851743256717,
36.));
#34597=CARTESIAN_POINT('Ctrl Pts',(-20.5988349568115,-67.9597503182989,
36.));
#34598=CARTESIAN_POINT('Ctrl Pts',(-20.6657963519685,-67.9304366251968,
36.));
#34599=CARTESIAN_POINT('Ctrl Pts',(-20.7308654665295,-67.8975272739048,
36.));
#34600=CARTESIAN_POINT('Ctrl Pts',(-20.7977455609987,-67.8637020015282,
36.));
#34601=CARTESIAN_POINT('Ctrl Pts',(-20.8626273501256,-67.8260774511082,
36.));
#34602=CARTESIAN_POINT('Ctrl Pts',(-20.9252744643285,-67.7849282442006,
36.));
#34603=CARTESIAN_POINT('Ctrl Pts',(-20.978207188369,-67.7501598491764,36.));
#34604=CARTESIAN_POINT('Ctrl Pts',(-21.0295442108216,-67.712874099006,36.));
#34605=CARTESIAN_POINT('Ctrl Pts',(-21.0791202112029,-67.6732186358219,
36.));
#34606=CARTESIAN_POINT('Ctrl Pts',(-21.1011498844546,-67.6555972688324,
36.));
#34607=CARTESIAN_POINT('Ctrl Pts',(-21.122831527857,-67.6375078058363,36.));
#34608=CARTESIAN_POINT('Ctrl Pts',(-21.1441490823126,-67.6189624773662,
36.));
#34609=CARTESIAN_POINT('Ctrl Pts',(-21.155861650937,-67.6087730612763,36.));
#34610=CARTESIAN_POINT('Ctrl Pts',(-21.1674642919294,-67.5984460234341,
36.));
#34611=CARTESIAN_POINT('Ctrl Pts',(-21.1789542074706,-67.5879833507474,
36.));
#34612=CARTESIAN_POINT('Ctrl Pts',(-21.1895477678368,-67.5783368956189,
36.));
#34613=CARTESIAN_POINT('Ctrl Pts',(-21.2000469385075,-67.5685736271126,
36.));
#34614=CARTESIAN_POINT('Ctrl Pts',(-21.2104336389044,-67.558710558091,36.));
#34615=CARTESIAN_POINT('Ctrl Pts',(-21.2635184075268,-67.5083019858866,
36.));
#34616=CARTESIAN_POINT('Ctrl Pts',(-21.3137631820402,-67.4552050116029,
36.));
#34617=CARTESIAN_POINT('Ctrl Pts',(-21.3609492954881,-67.3996791016713,
36.));
#34618=CARTESIAN_POINT('Ctrl Pts',(-21.4077692547296,-67.3445840609934,
36.));
#34619=CARTESIAN_POINT('Ctrl Pts',(-21.4515783462198,-67.2870967510757,
36.));
#34620=CARTESIAN_POINT('Ctrl Pts',(-21.492118162325,-67.227446405065,36.));
#34621=CARTESIAN_POINT('Ctrl Pts',(-21.5258065913802,-67.1778772002002,
36.));
#34622=CARTESIAN_POINT('Ctrl Pts',(-21.5572367636985,-67.1268136492829,
36.));
#34623=CARTESIAN_POINT('Ctrl Pts',(-21.5862327897514,-67.0743808223096,
36.));
#34624=CARTESIAN_POINT('Ctrl Pts',(-21.5983389541644,-67.0524895320059,
36.));
#34625=CARTESIAN_POINT('Ctrl Pts',(-21.6100204872529,-67.0303595164811,
36.));
#34626=CARTESIAN_POINT('Ctrl Pts',(-21.6212631465098,-67.00799979522,36.));
#34627=CARTESIAN_POINT('Ctrl Pts',(-21.6264639667105,-66.9976562557281,
36.));
#34628=CARTESIAN_POINT('Ctrl Pts',(-21.6315708572837,-66.9872635601815,
36.));
#34629=CARTESIAN_POINT('Ctrl Pts',(-21.6365823430867,-66.9768226034342,
36.));
#34630=CARTESIAN_POINT('Ctrl Pts',(-21.6418143363506,-66.9659222402453,
36.));
#34631=CARTESIAN_POINT('Ctrl Pts',(-21.646938735,-66.9549767280432,36.));
#34632=CARTESIAN_POINT('Ctrl Pts',(-21.6519524804853,-66.9439913743558,
36.));
#34633=CARTESIAN_POINT('Ctrl Pts',(-21.6804928809327,-66.8814580059955,
36.));
#34634=CARTESIAN_POINT('Ctrl Pts',(-21.7054723099544,-66.8175915741647,
36.));
#34635=CARTESIAN_POINT('Ctrl Pts',(-21.7266673077709,-66.75259653298,36.));
#34636=CARTESIAN_POINT('Ctrl Pts',(-21.745869779544,-66.6937116274686,36.));
#34637=CARTESIAN_POINT('Ctrl Pts',(-21.7619655953208,-66.6338997397485,
36.));
#34638=CARTESIAN_POINT('Ctrl Pts',(-21.7747518800532,-66.5733080889475,
36.));
#34639=CARTESIAN_POINT('Ctrl Pts',(-21.7898843881512,-66.5015981539972,
36.));
#34640=CARTESIAN_POINT('Ctrl Pts',(-21.800381967919,-66.4287945165716,36.));
#34641=CARTESIAN_POINT('Ctrl Pts',(-21.8063197580553,-66.3553202766994,
36.));
#34642=CARTESIAN_POINT('Ctrl Pts',(-21.8076265822748,-66.3391496283656,
36.));
#34643=CARTESIAN_POINT('Ctrl Pts',(-21.8087123163694,-66.3229465792852,
36.));
#34644=CARTESIAN_POINT('Ctrl Pts',(-21.8095773920817,-66.3067158043034,
36.));
#34645=CARTESIAN_POINT('Ctrl Pts',(-21.8104727224283,-66.2899173840217,
36.));
#34646=CARTESIAN_POINT('Ctrl Pts',(-21.8111317001266,-66.273083070086,36.));
#34647=CARTESIAN_POINT('Ctrl Pts',(-21.8115542428401,-66.2562523196269,
36.));
#34648=CARTESIAN_POINT('Ctrl Pts',(-21.8132754914067,-66.1876914281915,
36.));
#34649=CARTESIAN_POINT('Ctrl Pts',(-21.8110851349638,-66.1191029658962,
36.));
#34650=CARTESIAN_POINT('Ctrl Pts',(-21.8051037575689,-66.0508252572189,
36.));
#34651=CARTESIAN_POINT('Ctrl Pts',(-21.7991236159828,-65.982561655357,36.));
#34652=CARTESIAN_POINT('Ctrl Pts',(-21.7893535661429,-65.9146076071237,
36.));
#34653=CARTESIAN_POINT('Ctrl Pts',(-21.775864512327,-65.8473162604127,36.));
#34654=CARTESIAN_POINT('Ctrl Pts',(-21.7661045201055,-65.7986276696904,
36.));
#34655=CARTESIAN_POINT('Ctrl Pts',(-21.7543964928538,-65.7502862841395,
36.));
#34656=CARTESIAN_POINT('Ctrl Pts',(-21.7407530856673,-65.7024355240451,
36.));
#34657=CARTESIAN_POINT('Ctrl Pts',(-21.730516731348,-65.6665341302011,36.));
#34658=CARTESIAN_POINT('Ctrl Pts',(-21.7191906681288,-65.6309090730154,
36.));
#34659=CARTESIAN_POINT('Ctrl Pts',(-21.7067763258098,-65.5956251017723,
36.));
#34660=CARTESIAN_POINT('Ctrl Pts',(-21.7026468040941,-65.5838881992669,
36.));
#34661=CARTESIAN_POINT('Ctrl Pts',(-21.6984000585611,-65.5721982316542,
36.));
#34662=CARTESIAN_POINT('Ctrl Pts',(-21.694036734101,-65.5605577596171,36.));
#34663=CARTESIAN_POINT('Ctrl Pts',(-21.6709127863924,-65.4988677181932,
36.));
#34664=CARTESIAN_POINT('Ctrl Pts',(-21.644516250875,-65.4385612113467,36.));
#34665=CARTESIAN_POINT('Ctrl Pts',(-21.6148971220792,-65.3799723297871,
36.));
#34666=CARTESIAN_POINT('Ctrl Pts',(-21.5940647872686,-65.3387643926717,
36.));
#34667=CARTESIAN_POINT('Ctrl Pts',(-21.5716374194864,-65.2984066732515,
36.));
#34668=CARTESIAN_POINT('Ctrl Pts',(-21.5476220123981,-65.2590267602619,
36.));
#34669=CARTESIAN_POINT('Ctrl Pts',(-21.5399089963368,-65.2463791336669,
36.));
#34670=CARTESIAN_POINT('Ctrl Pts',(-21.5320310170669,-65.2338307611699,
36.));
#34671=CARTESIAN_POINT('Ctrl Pts',(-21.5239916307924,-65.2213915044329,
36.));
#34672=CARTESIAN_POINT('Ctrl Pts',(-21.4897471128518,-65.1684053266386,
36.));
#34673=CARTESIAN_POINT('Ctrl Pts',(-21.4526468301773,-65.117502937192,36.));
#34674=CARTESIAN_POINT('Ctrl Pts',(-21.4127250200562,-65.0689995578316,
36.));
#34675=CARTESIAN_POINT('Ctrl Pts',(-21.3759382490648,-65.024305123801,36.));
#34676=CARTESIAN_POINT('Ctrl Pts',(-21.3367551102847,-64.9816476143428,
36.));
#34677=CARTESIAN_POINT('Ctrl Pts',(-21.2951809526149,-64.9413065633649,
36.));
#34678=CARTESIAN_POINT('Ctrl Pts',(-21.2873626038736,-64.9337201100773,
36.));
#34679=CARTESIAN_POINT('Ctrl Pts',(-21.2794596418601,-64.9262156834178,
36.));
#34680=CARTESIAN_POINT('Ctrl Pts',(-21.2714736587043,-64.9187939493416,
36.));
#34681=CARTESIAN_POINT('Origin',(-20.,-66.,30.));
#34682=CARTESIAN_POINT('Origin',(20.,-66.,24.));
#34683=CARTESIAN_POINT('Origin',(-20.,-66.,24.));
#34684=CARTESIAN_POINT('Origin',(-20.,66.,24.));
#34685=CARTESIAN_POINT('Origin',(20.,66.,24.));
#34686=CARTESIAN_POINT('Origin',(20.,50.,0.));
#34687=CARTESIAN_POINT('',(24.,45.,6.12323399573677E-16));
#34688=CARTESIAN_POINT('Origin',(24.,50.,0.));
#34689=CARTESIAN_POINT('',(16.,45.,6.12323399573677E-16));
#34690=CARTESIAN_POINT('',(20.,45.,6.12323399573677E-16));
#34691=CARTESIAN_POINT('Origin',(16.,50.,0.));
#34692=CARTESIAN_POINT('Origin',(20.,30.,20.));
#34693=CARTESIAN_POINT('',(24.,25.,20.));
#34694=CARTESIAN_POINT('Origin',(24.,30.,20.));
#34695=CARTESIAN_POINT('',(16.,25.,20.));
#34696=CARTESIAN_POINT('',(20.,25.,20.));
#34697=CARTESIAN_POINT('Origin',(16.,30.,20.));
#34698=CARTESIAN_POINT('Origin',(20.,30.,-20.));
#34699=CARTESIAN_POINT('',(24.,25.,-20.));
#34700=CARTESIAN_POINT('Origin',(24.,30.,-20.));
#34701=CARTESIAN_POINT('',(16.,25.,-20.));
#34702=CARTESIAN_POINT('',(20.,25.,-20.));
#34703=CARTESIAN_POINT('Origin',(16.,30.,-20.));
#34704=CARTESIAN_POINT('Origin',(20.,10.,0.));
#34705=CARTESIAN_POINT('',(24.,5.,6.12323399573677E-16));
#34706=CARTESIAN_POINT('Origin',(24.,10.,0.));
#34707=CARTESIAN_POINT('',(16.,5.,6.12323399573677E-16));
#34708=CARTESIAN_POINT('',(20.,5.,6.12323399573677E-16));
#34709=CARTESIAN_POINT('Origin',(16.,10.,0.));
#34710=CARTESIAN_POINT('Origin',(20.,-10.,20.));
#34711=CARTESIAN_POINT('',(24.,-15.,20.));
#34712=CARTESIAN_POINT('Origin',(24.,-10.,20.));
#34713=CARTESIAN_POINT('',(16.,-15.,20.));
#34714=CARTESIAN_POINT('',(20.,-15.,20.));
#34715=CARTESIAN_POINT('Origin',(16.,-10.,20.));
#34716=CARTESIAN_POINT('Origin',(20.,-10.,-20.));
#34717=CARTESIAN_POINT('',(24.,-15.,-20.));
#34718=CARTESIAN_POINT('Origin',(24.,-10.,-20.));
#34719=CARTESIAN_POINT('',(16.,-15.,-20.));
#34720=CARTESIAN_POINT('',(20.,-15.,-20.));
#34721=CARTESIAN_POINT('Origin',(16.,-10.,-20.));
#34722=CARTESIAN_POINT('Origin',(20.,-30.,0.));
#34723=CARTESIAN_POINT('',(24.,-35.,6.12323399573677E-16));
#34724=CARTESIAN_POINT('Origin',(24.,-30.,0.));
#34725=CARTESIAN_POINT('',(16.,-35.,6.12323399573677E-16));
#34726=CARTESIAN_POINT('',(20.,-35.,6.12323399573677E-16));
#34727=CARTESIAN_POINT('Origin',(16.,-30.,0.));
#34728=CARTESIAN_POINT('Origin',(20.,-50.,20.));
#34729=CARTESIAN_POINT('',(24.,-55.,20.));
#34730=CARTESIAN_POINT('Origin',(24.,-50.,20.));
#34731=CARTESIAN_POINT('',(16.,-55.,20.));
#34732=CARTESIAN_POINT('',(20.,-55.,20.));
#34733=CARTESIAN_POINT('Origin',(16.,-50.,20.));
#34734=CARTESIAN_POINT('Origin',(20.,-50.,-20.));
#34735=CARTESIAN_POINT('',(24.,-50.,-25.));
#34736=CARTESIAN_POINT('Origin',(24.,-50.,-20.));
#34737=CARTESIAN_POINT('',(20.,-50.,-25.));
#34738=CARTESIAN_POINT('',(16.,-50.,-25.));
#34739=CARTESIAN_POINT('',(20.,-50.,-25.));
#34740=CARTESIAN_POINT('Origin',(16.,-50.,-20.));
#34741=CARTESIAN_POINT('Origin',(20.,-50.,0.));
#34742=CARTESIAN_POINT('',(24.,-55.,6.12323399573677E-16));
#34743=CARTESIAN_POINT('Origin',(24.,-50.,0.));
#34744=CARTESIAN_POINT('',(16.,-55.,6.12323399573677E-16));
#34745=CARTESIAN_POINT('',(20.,-55.,6.12323399573677E-16));
#34746=CARTESIAN_POINT('Origin',(16.,-50.,0.));
#34747=CARTESIAN_POINT('Origin',(20.,-30.,-20.));
#34748=CARTESIAN_POINT('',(24.,-35.,-20.));
#34749=CARTESIAN_POINT('Origin',(24.,-30.,-20.));
#34750=CARTESIAN_POINT('',(16.,-35.,-20.));
#34751=CARTESIAN_POINT('',(20.,-35.,-20.));
#34752=CARTESIAN_POINT('Origin',(16.,-30.,-20.));
#34753=CARTESIAN_POINT('Origin',(20.,-30.,20.));
#34754=CARTESIAN_POINT('',(24.,-35.,20.));
#34755=CARTESIAN_POINT('Origin',(24.,-30.,20.));
#34756=CARTESIAN_POINT('',(16.,-35.,20.));
#34757=CARTESIAN_POINT('',(20.,-35.,20.));
#34758=CARTESIAN_POINT('Origin',(16.,-30.,20.));
#34759=CARTESIAN_POINT('Origin',(20.,-10.,0.));
#34760=CARTESIAN_POINT('',(24.,-15.,6.12323399573677E-16));
#34761=CARTESIAN_POINT('Origin',(24.,-10.,0.));
#34762=CARTESIAN_POINT('',(16.,-15.,6.12323399573677E-16));
#34763=CARTESIAN_POINT('',(20.,-15.,6.12323399573677E-16));
#34764=CARTESIAN_POINT('Origin',(16.,-10.,0.));
#34765=CARTESIAN_POINT('Origin',(20.,10.,-20.));
#34766=CARTESIAN_POINT('',(24.,5.,-20.));
#34767=CARTESIAN_POINT('Origin',(24.,10.,-20.));
#34768=CARTESIAN_POINT('',(16.,5.,-20.));
#34769=CARTESIAN_POINT('',(20.,5.,-20.));
#34770=CARTESIAN_POINT('Origin',(16.,10.,-20.));
#34771=CARTESIAN_POINT('Origin',(20.,10.,20.));
#34772=CARTESIAN_POINT('',(24.,5.,20.));
#34773=CARTESIAN_POINT('Origin',(24.,10.,20.));
#34774=CARTESIAN_POINT('',(16.,5.,20.));
#34775=CARTESIAN_POINT('',(20.,5.,20.));
#34776=CARTESIAN_POINT('Origin',(16.,10.,20.));
#34777=CARTESIAN_POINT('Origin',(20.,30.,0.));
#34778=CARTESIAN_POINT('',(24.,25.,6.12323399573677E-16));
#34779=CARTESIAN_POINT('Origin',(24.,30.,0.));
#34780=CARTESIAN_POINT('',(16.,25.,6.12323399573677E-16));
#34781=CARTESIAN_POINT('',(20.,25.,6.12323399573677E-16));
#34782=CARTESIAN_POINT('Origin',(16.,30.,0.));
#34783=CARTESIAN_POINT('Origin',(20.,50.,-20.));
#34784=CARTESIAN_POINT('',(24.,50.,-25.));
#34785=CARTESIAN_POINT('Origin',(24.,50.,-20.));
#34786=CARTESIAN_POINT('',(20.,50.,-25.));
#34787=CARTESIAN_POINT('',(16.,50.,-25.));
#34788=CARTESIAN_POINT('',(20.,50.,-25.));
#34789=CARTESIAN_POINT('Origin',(16.,50.,-20.));
#34790=CARTESIAN_POINT('Origin',(20.,50.,20.));
#34791=CARTESIAN_POINT('',(24.,45.,20.));
#34792=CARTESIAN_POINT('Origin',(24.,50.,20.));
#34793=CARTESIAN_POINT('',(16.,45.,20.));
#34794=CARTESIAN_POINT('',(20.,45.,20.));
#34795=CARTESIAN_POINT('Origin',(16.,50.,20.));
#34796=CARTESIAN_POINT('Origin',(16.,-62.,36.));
#34797=CARTESIAN_POINT('',(16.,-62.,36.));
#34798=CARTESIAN_POINT('',(-16.,-62.,36.));
#34799=CARTESIAN_POINT('',(8.,-62.,36.));
#34800=CARTESIAN_POINT('',(16.,-62.,-36.));
#34801=CARTESIAN_POINT('',(16.,-62.,36.));
#34802=CARTESIAN_POINT('',(-16.,-62.,-36.));
#34803=CARTESIAN_POINT('',(-16.,-62.,-36.));
#34804=CARTESIAN_POINT('',(-16.,-62.,36.));
#34805=CARTESIAN_POINT('Origin',(16.,62.,36.));
#34806=CARTESIAN_POINT('',(16.,62.,36.));
#34807=CARTESIAN_POINT('',(16.,31.,36.));
#34808=CARTESIAN_POINT('',(16.,62.,-36.));
#34809=CARTESIAN_POINT('',(16.,62.,36.));
#34810=CARTESIAN_POINT('',(16.,-62.,-36.));
#34811=CARTESIAN_POINT('Origin',(-16.,62.,36.));
#34812=CARTESIAN_POINT('',(-16.,62.,36.));
#34813=CARTESIAN_POINT('',(-8.,62.,36.));
#34814=CARTESIAN_POINT('',(-16.,62.,-36.));
#34815=CARTESIAN_POINT('',(-16.,62.,36.));
#34816=CARTESIAN_POINT('',(16.,62.,-36.));
#34817=CARTESIAN_POINT('Origin',(-16.,-62.,36.));
#34818=CARTESIAN_POINT('',(-16.,-31.,36.));
#34819=CARTESIAN_POINT('',(-16.,62.,-36.));
#34820=CARTESIAN_POINT('Origin',(0.,0.,-36.));
#34821=CARTESIAN_POINT('Origin',(24.,75.,-40.));
#34822=CARTESIAN_POINT('',(-29.,75.,36.));
#34823=CARTESIAN_POINT('',(-29.,75.,-40.));
#34824=CARTESIAN_POINT('',(24.,75.,36.));
#34825=CARTESIAN_POINT('',(12.,75.,36.));
#34826=CARTESIAN_POINT('',(24.,75.,-40.));
#34827=CARTESIAN_POINT('Origin',(24.,-70.,-40.));
#34828=CARTESIAN_POINT('',(24.,-75.,36.));
#34829=CARTESIAN_POINT('',(24.,-70.,36.));
#34830=CARTESIAN_POINT('',(24.,-75.,-40.));
#34831=CARTESIAN_POINT('Origin',(-24.,-75.,-40.));
#34832=CARTESIAN_POINT('',(-29.,-75.,36.));
#34833=CARTESIAN_POINT('',(-12.,-75.,36.));
#34834=CARTESIAN_POINT('',(-29.,-75.,-40.));
#34835=CARTESIAN_POINT('Origin',(-29.,70.,-40.));
#34836=CARTESIAN_POINT('',(-29.,35.,36.));
#34837=CARTESIAN_POINT('Origin',(0.,0.,36.));
#42598=UNCERTAINTY_MEASURE_WITH_UNIT(LENGTH_MEASURE(0.01),#42621,
'DISTANCE_ACCURACY_VALUE',
'Maximum model space distance between geometric entities at asserted c
onnectivities');
#42608=UNCERTAINTY_MEASURE_WITH_UNIT(LENGTH_MEASURE(0.01),#42621,
'DISTANCE_ACCURACY_VALUE',
'Maximum model space distance between geometric entities at asserted c
onnectivities');
#42610=(
GEOMETRIC_REPRESENTATION_CONTEXT(3)
GLOBAL_UNCERTAINTY_ASSIGNED_CONTEXT((#42598))
GLOBAL_UNIT_ASSIGNED_CONTEXT((#42621,#42623,#42624))
REPRESENTATION_CONTEXT('','3D')
);
#42620=(
GEOMETRIC_REPRESENTATION_CONTEXT(3)
GLOBAL_UNCERTAINTY_ASSIGNED_CONTEXT((#42608))
GLOBAL_UNIT_ASSIGNED_CONTEXT((#42621,#42623,#42624))
REPRESENTATION_CONTEXT('','3D')
);
#42621=(
LENGTH_UNIT()
NAMED_UNIT(*)
SI_UNIT(.MILLI.,.METRE.)
);
#42623=(
NAMED_UNIT(*)
PLANE_ANGLE_UNIT()
SI_UNIT($,.RADIAN.)
);
#42624=(
NAMED_UNIT(*)
SI_UNIT($,.STERADIAN.)
SOLID_ANGLE_UNIT()
);
#42626=SHAPE_DEFINITION_REPRESENTATION(#42637,#42723);
#42637=PRODUCT_DEFINITION_SHAPE('',$,#42735);
#42723=SHAPE_REPRESENTATION('',(#10505),#42610);
#42733=PRODUCT_DEFINITION_CONTEXT('part definition',#42768,'design');
#42735=PRODUCT_DEFINITION('Fluid header','Fluid header',#42746,#42733);
#42746=PRODUCT_DEFINITION_FORMATION('',$,#42771);
#42768=APPLICATION_CONTEXT(
'Core Data for Automotive Mechanical Design Process');
#42769=PRODUCT_CONTEXT('part definition',#42768,'mechanical');
#42771=PRODUCT('Fluid header','Fluid header',$,(#42769));
#42782=PRESENTATION_STYLE_ASSIGNMENT((#42790));
#42790=SURFACE_STYLE_USAGE(.BOTH.,#42798);
#42798=SURFACE_SIDE_STYLE('',(#42806));
#42806=SURFACE_STYLE_FILL_AREA(#42814);
#42814=FILL_AREA_STYLE('Dark blue',(#42822));
#42822=FILL_AREA_STYLE_COLOUR('Dark blue',#42830);
#42830=COLOUR_RGB('Dark blue',0.0901960784313725,0.270588235294118,0.513725490196078);
ENDSEC;
END-ISO-10303-21;
